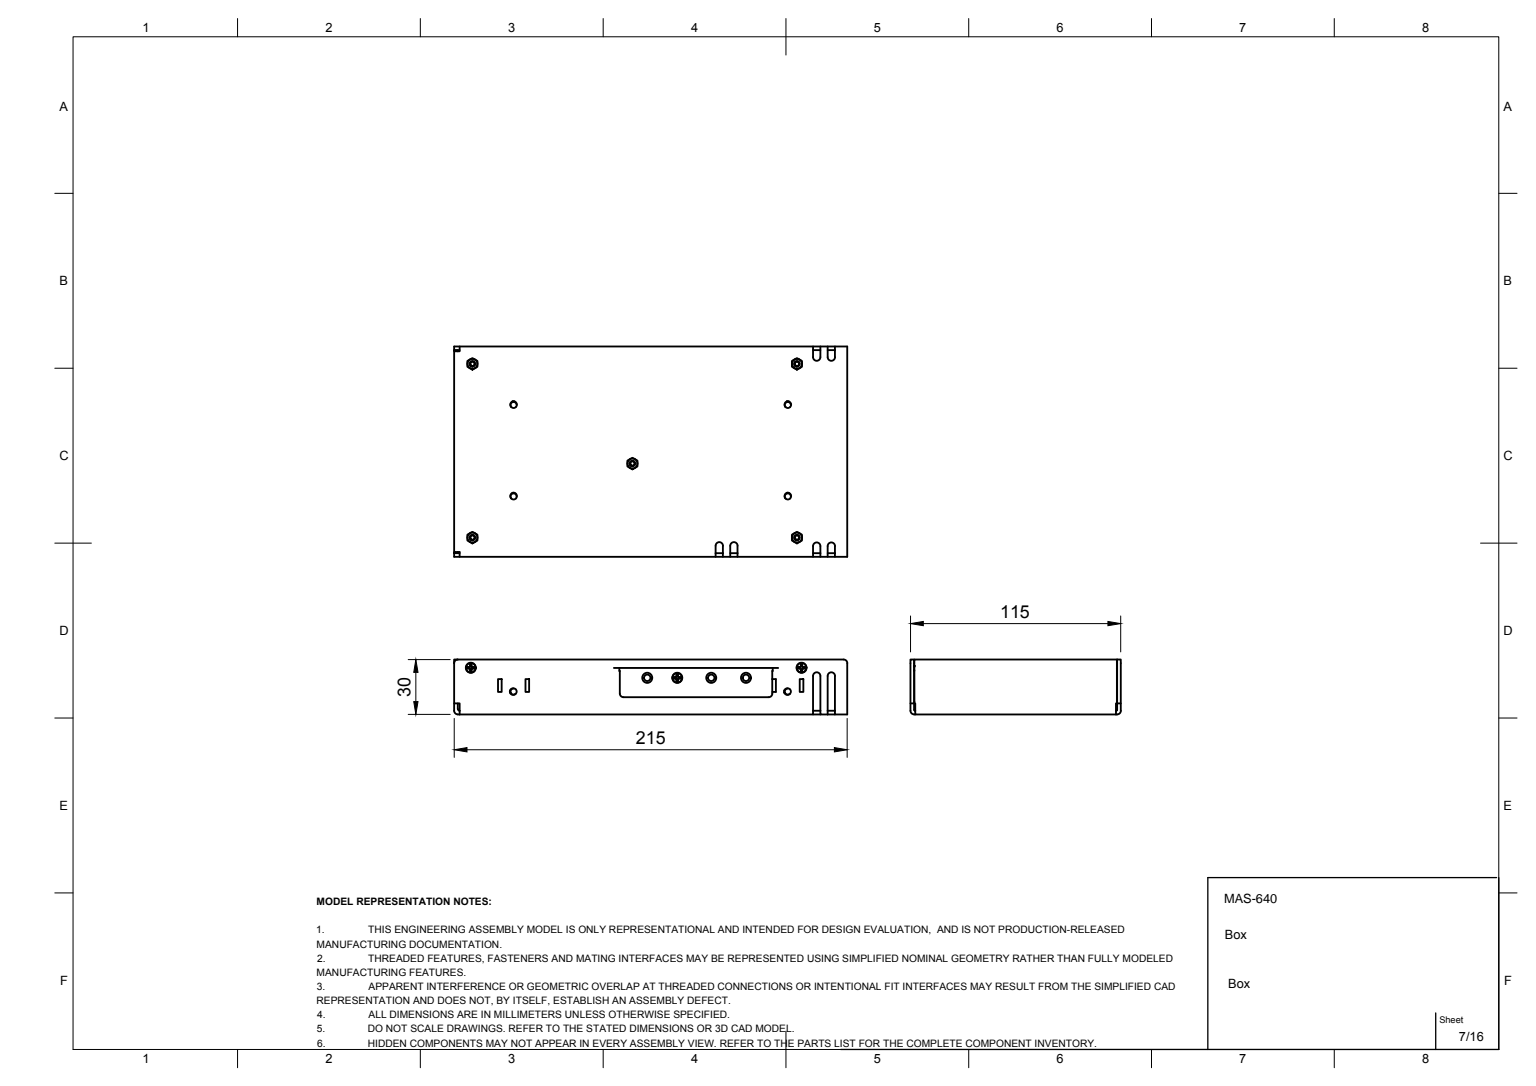
ISO-10303-21;
HEADER;
FILE_DESCRIPTION((''),'2;1');
FILE_NAME('Box.step','2026-10-09T10:33:02-07:00',(''),(''),'','','');
FILE_SCHEMA (('AUTOMOTIVE_DESIGN { 1 0 10303 214 3 1 1 }'));
ENDSEC;
DATA;
#10=MECHANICAL_DESIGN_GEOMETRIC_PRESENTATION_REPRESENTATION('',(#841),#86330);
#227=TOROIDAL_SURFACE('',#33403,5.,1.) ;
#228=TOROIDAL_SURFACE('',#33408,5.,1.) ;
#229=TOROIDAL_SURFACE('',#33423,5.,1.) ;
#230=TOROIDAL_SURFACE('',#33428,5.,1.) ;
#231=TOROIDAL_SURFACE('',#33506,5.25,3.25) ;
#232=TOROIDAL_SURFACE('',#33549,5.25,3.25) ;
#233=TOROIDAL_SURFACE('',#33614,5.25,3.25) ;
#234=TOROIDAL_SURFACE('',#33619,5.25,3.25) ;
#235=TOROIDAL_SURFACE('',#33657,0.250000000000004,0.124999999999957) ;
#236=TOROIDAL_SURFACE('',#33661,0.250000000000004,0.125000000000002) ;
#237=TOROIDAL_SURFACE('',#33662,0.250000000000004,0.125000000000002) ;
#238=TOROIDAL_SURFACE('',#33663,0.250000000000004,0.125000000000011) ;
#740=(
BOUNDED_SURFACE()
B_SPLINE_SURFACE(2,2,((#67035,#67036,#67037),(#67038,#67039,#67040),(#67041,
#67042,#67043)),.UNSPECIFIED.,.F.,.F.,.F.)
B_SPLINE_SURFACE_WITH_KNOTS((3,3),(3,3),(-1.5707963267962,1.31181440870059E-14),
(-1.57079632679766,2.95313754417746E-12),.UNSPECIFIED.)
GEOMETRIC_REPRESENTATION_ITEM()
RATIONAL_B_SPLINE_SURFACE(((1.,0.707106781184525,1.),(0.707106781186029,
0.499999999998204,0.707106781186029),(1.,0.707106781184525,1.)))
REPRESENTATION_ITEM('')
SURFACE()
) ;
#741=(
BOUNDED_SURFACE()
B_SPLINE_SURFACE(2,2,((#67047,#67048,#67049),(#67050,#67051,#67052),(#67053,
#67054,#67055)),.UNSPECIFIED.,.F.,.F.,.F.)
B_SPLINE_SURFACE_WITH_KNOTS((3,3),(3,3),(-1.38839876682605E-15,1.57079632679588),
(1.57079632679424,3.14159265359081),.UNSPECIFIED.)
GEOMETRIC_REPRESENTATION_ITEM()
RATIONAL_B_SPLINE_SURFACE(((1.,0.707106781185957,1.),(0.707106781186211,
0.499999999999345,0.707106781186211),(1.,0.707106781185957,1.)))
REPRESENTATION_ITEM('')
SURFACE()
) ;
#742=(
BOUNDED_SURFACE()
B_SPLINE_SURFACE(2,2,((#67066,#67067,#67068),(#67069,#67070,#67071),(#67072,
#67073,#67074)),.UNSPECIFIED.,.F.,.F.,.F.)
B_SPLINE_SURFACE_WITH_KNOTS((3,3),(3,3),(-3.21499456677232E-13,1.57079632679539),
(-7.36310365920222E-13,1.57079632679562),.UNSPECIFIED.)
GEOMETRIC_REPRESENTATION_ITEM()
RATIONAL_B_SPLINE_SURFACE(((1.,0.707106781186032,1.),(0.707106781186293,
0.499999999999455,0.707106781186293),(1.,0.707106781186032,1.)))
REPRESENTATION_ITEM('')
SURFACE()
) ;
#743=(
BOUNDED_SURFACE()
B_SPLINE_SURFACE(2,2,((#67078,#67079,#67080),(#67081,#67082,#67083),(#67084,
#67085,#67086)),.UNSPECIFIED.,.F.,.F.,.F.)
B_SPLINE_SURFACE_WITH_KNOTS((3,3),(3,3),(-1.57079632679451,6.78283756875461E-13),
(-3.14159265358933,-1.57079632679533),.UNSPECIFIED.)
GEOMETRIC_REPRESENTATION_ITEM()
RATIONAL_B_SPLINE_SURFACE(((1.,0.707106781186867,1.),(0.70710678118647,
0.500000000000171,0.70710678118647),(1.,0.707106781186867,1.)))
REPRESENTATION_ITEM('')
SURFACE()
) ;
#817=SHAPE_REPRESENTATION_RELATIONSHIP('SRR','None',#86454,#829) ;
#829=ADVANCED_BREP_SHAPE_REPRESENTATION('',(#853),#86308) ;
#841=STYLED_ITEM('',(#86581),#853) ;
#853=MANIFOLD_SOLID_BREP('Body1',#32640) ;
#883=CONICAL_SURFACE('',#33469,2.20000000000002,0.785398163397472) ;
#884=CONICAL_SURFACE('',#33472,2.2,0.78539816339745) ;
#885=CONICAL_SURFACE('',#33475,2.2,0.785398163397451) ;
#886=CONICAL_SURFACE('',#33486,2.25,0.785398163397448) ;
#887=CONICAL_SURFACE('',#33571,2.25,0.785398163397448) ;
#888=CONICAL_SURFACE('',#33576,2.25,0.785398163397448) ;
#889=CONICAL_SURFACE('',#33581,2.25,0.785398163397448) ;
#890=CONICAL_SURFACE('',#33586,2.25,0.785398163397448) ;
#891=CONICAL_SURFACE('',#33635,2.2,0.78539816339745) ;
#905=B_SPLINE_SURFACE_WITH_KNOTS('',3,1,((#65564,#65565),(#65566,#65567),
(#65568,#65569),(#65570,#65571),(#65572,#65573),(#65574,#65575),(#65576,
#65577),(#65578,#65579),(#65580,#65581),(#65582,#65583),(#65584,#65585),
(#65586,#65587),(#65588,#65589),(#65590,#65591),(#65592,#65593),(#65594,
#65595),(#65596,#65597),(#65598,#65599),(#65600,#65601),(#65602,#65603),
(#65604,#65605),(#65606,#65607)),.UNSPECIFIED.,.F.,.F.,.F.,(4,3,3,3,3,3,
3,4),(2,2),(0.136589431488165,0.1402592459748,0.143851356976514,0.2091154250925,
0.346827783328,0.4845401415634,0.990211404581674,0.997547219258416),(0.,
0.297000000002801),.UNSPECIFIED.) ;
#906=B_SPLINE_SURFACE_WITH_KNOTS('',3,3,((#66221,#66222,#66223,#66224,#66225,
#66226,#66227,#66228,#66229,#66230,#66231,#66232,#66233,#66234,#66235,#66236,
#66237,#66238,#66239,#66240,#66241,#66242,#66243),(#66244,#66245,#66246,
#66247,#66248,#66249,#66250,#66251,#66252,#66253,#66254,#66255,#66256,#66257,
#66258,#66259,#66260,#66261,#66262,#66263,#66264,#66265,#66266),(#66267,
#66268,#66269,#66270,#66271,#66272,#66273,#66274,#66275,#66276,#66277,#66278,
#66279,#66280,#66281,#66282,#66283,#66284,#66285,#66286,#66287,#66288,#66289),
(#66290,#66291,#66292,#66293,#66294,#66295,#66296,#66297,#66298,#66299,
#66300,#66301,#66302,#66303,#66304,#66305,#66306,#66307,#66308,#66309,#66310,
#66311,#66312)),.UNSPECIFIED.,.F.,.F.,.F.,(4,4),(4,1,1,1,1,1,1,1,1,1,1,
1,1,1,1,1,1,1,1,1,4),(-0.000643685928907995,0.0452738098722425),(14.3976860695295,
15.3964695570642,16.3947981013537,17.3931266456432,18.3914551899327,19.3897837342222,
20.3881122785118,21.3864408228013,22.3847693670908,23.3830979113803,24.3814264556698,
25.3797549999593,26.3780835442488,27.3764120885383,28.3747406328278,29.3730691771173,
30.3713977214068,31.3697262656963,32.3680548099858,33.3663833542754,34.3650967250075),
 .UNSPECIFIED.) ;
#907=B_SPLINE_SURFACE_WITH_KNOTS('',3,3,((#66313,#66314,#66315,#66316,#66317,
#66318,#66319,#66320,#66321,#66322,#66323,#66324,#66325,#66326,#66327,#66328,
#66329,#66330,#66331,#66332,#66333,#66334,#66335),(#66336,#66337,#66338,
#66339,#66340,#66341,#66342,#66343,#66344,#66345,#66346,#66347,#66348,#66349,
#66350,#66351,#66352,#66353,#66354,#66355,#66356,#66357,#66358),(#66359,
#66360,#66361,#66362,#66363,#66364,#66365,#66366,#66367,#66368,#66369,#66370,
#66371,#66372,#66373,#66374,#66375,#66376,#66377,#66378,#66379,#66380,#66381),
(#66382,#66383,#66384,#66385,#66386,#66387,#66388,#66389,#66390,#66391,
#66392,#66393,#66394,#66395,#66396,#66397,#66398,#66399,#66400,#66401,#66402,
#66403,#66404)),.UNSPECIFIED.,.F.,.F.,.F.,(4,4),(4,1,1,1,1,1,1,1,1,1,1,
1,1,1,1,1,1,1,1,1,4),(-0.000384825361838686,0.0458091503480694),(11.8611951788935,
12.8599085485448,13.8582370928343,14.8565656371238,15.8548941814133,16.8532227257028,
17.8515512699923,18.8498798142818,19.8482083585713,20.8465369028608,21.8448654471503,
22.8431939914399,23.8415225357294,24.8398510800189,25.8381796243084,26.8365081685979,
27.8348367128874,28.8331652571769,29.8314938014664,30.8298223457559,31.8285783647924),
 .UNSPECIFIED.) ;
#908=B_SPLINE_SURFACE_WITH_KNOTS('',3,3,((#66405,#66406,#66407,#66408,#66409,
#66410,#66411,#66412,#66413,#66414,#66415,#66416,#66417,#66418,#66419,#66420,
#66421,#66422,#66423,#66424,#66425,#66426,#66427),(#66428,#66429,#66430,
#66431,#66432,#66433,#66434,#66435,#66436,#66437,#66438,#66439,#66440,#66441,
#66442,#66443,#66444,#66445,#66446,#66447,#66448,#66449,#66450),(#66451,
#66452,#66453,#66454,#66455,#66456,#66457,#66458,#66459,#66460,#66461,#66462,
#66463,#66464,#66465,#66466,#66467,#66468,#66469,#66470,#66471,#66472,#66473),
(#66474,#66475,#66476,#66477,#66478,#66479,#66480,#66481,#66482,#66483,
#66484,#66485,#66486,#66487,#66488,#66489,#66490,#66491,#66492,#66493,#66494,
#66495,#66496)),.UNSPECIFIED.,.F.,.F.,.F.,(4,4),(4,1,1,1,1,1,1,1,1,1,1,
1,1,1,1,1,1,1,1,1,4),(-0.000647263935840991,0.0452759437895929),(14.3976836084423,
15.3964695570666,16.394798101356,17.3931266456453,18.3914551899347,19.389783734224,
20.3881122785134,21.3864408228027,22.384769367092,23.3830979113814,24.3814264556707,
25.3797549999601,26.3780835442494,27.3764120885388,28.3747406328281,29.3730691771175,
30.3713977214068,31.3697262656962,32.3680548099855,33.3663833542749,34.3650988589243),
 .UNSPECIFIED.) ;
#909=B_SPLINE_SURFACE_WITH_KNOTS('',3,3,((#66497,#66498,#66499,#66500,#66501,
#66502,#66503,#66504,#66505,#66506,#66507,#66508,#66509,#66510,#66511,#66512,
#66513,#66514,#66515,#66516,#66517,#66518,#66519),(#66520,#66521,#66522,
#66523,#66524,#66525,#66526,#66527,#66528,#66529,#66530,#66531,#66532,#66533,
#66534,#66535,#66536,#66537,#66538,#66539,#66540,#66541,#66542),(#66543,
#66544,#66545,#66546,#66547,#66548,#66549,#66550,#66551,#66552,#66553,#66554,
#66555,#66556,#66557,#66558,#66559,#66560,#66561,#66562,#66563,#66564,#66565),
(#66566,#66567,#66568,#66569,#66570,#66571,#66572,#66573,#66574,#66575,
#66576,#66577,#66578,#66579,#66580,#66581,#66582,#66583,#66584,#66585,#66586,
#66587,#66588)),.UNSPECIFIED.,.F.,.F.,.F.,(4,4),(4,1,1,1,1,1,1,1,1,1,1,
1,1,1,1,1,1,1,1,1,4),(-0.00038695950106726,0.0458188085461498),(11.8611930447567,
12.8599085485472,13.8582370928365,14.8565656371259,15.8548941814152,16.8532227257046,
17.8515512699939,18.8498798142833,19.8482083585726,20.846536902862,21.8448654471513,
22.8431939914407,23.84152253573,24.8398510800194,25.8381796243087,26.8365081685981,
27.8348367128874,28.8331652571768,29.8314938014661,30.8298223457555,31.8285876047897),
 .UNSPECIFIED.) ;
#910=B_SPLINE_SURFACE_WITH_KNOTS('',3,3,((#66589,#66590,#66591,#66592,#66593,
#66594,#66595,#66596,#66597,#66598,#66599,#66600,#66601,#66602,#66603,#66604,
#66605,#66606,#66607,#66608,#66609,#66610,#66611),(#66612,#66613,#66614,
#66615,#66616,#66617,#66618,#66619,#66620,#66621,#66622,#66623,#66624,#66625,
#66626,#66627,#66628,#66629,#66630,#66631,#66632,#66633,#66634),(#66635,
#66636,#66637,#66638,#66639,#66640,#66641,#66642,#66643,#66644,#66645,#66646,
#66647,#66648,#66649,#66650,#66651,#66652,#66653,#66654,#66655,#66656,#66657),
(#66658,#66659,#66660,#66661,#66662,#66663,#66664,#66665,#66666,#66667,
#66668,#66669,#66670,#66671,#66672,#66673,#66674,#66675,#66676,#66677,#66678,
#66679,#66680)),.UNSPECIFIED.,.F.,.F.,.F.,(4,4),(4,1,1,1,1,1,1,1,1,1,1,
1,1,1,1,1,1,1,1,1,4),(-0.000640464694106941,0.0452718121575805),(14.3976883946163,
15.3964695570665,16.394798101356,17.3931266456454,18.3914551899348,19.3897837342242,
20.3881122785137,21.3864408228031,22.3847693670925,23.3830979113819,24.3814264556714,
25.3797549999608,26.3780835442502,27.3764120885396,28.3747406328291,29.3730691771185,
30.3713977214079,31.3697262656973,32.3680548099868,33.3663833542762,34.3650947272934),
 .UNSPECIFIED.) ;
#911=B_SPLINE_SURFACE_WITH_KNOTS('',3,3,((#66681,#66682,#66683,#66684,#66685,
#66686,#66687,#66688,#66689,#66690,#66691,#66692,#66693,#66694,#66695,#66696,
#66697,#66698,#66699,#66700,#66701,#66702,#66703),(#66704,#66705,#66706,
#66707,#66708,#66709,#66710,#66711,#66712,#66713,#66714,#66715,#66716,#66717,
#66718,#66719,#66720,#66721,#66722,#66723,#66724,#66725,#66726),(#66727,
#66728,#66729,#66730,#66731,#66732,#66733,#66734,#66735,#66736,#66737,#66738,
#66739,#66740,#66741,#66742,#66743,#66744,#66745,#66746,#66747,#66748,#66749),
(#66750,#66751,#66752,#66753,#66754,#66755,#66756,#66757,#66758,#66759,
#66760,#66761,#66762,#66763,#66764,#66765,#66766,#66767,#66768,#66769,#66770,
#66771,#66772)),.UNSPECIFIED.,.F.,.F.,.F.,(4,4),(4,1,1,1,1,1,1,1,1,1,1,
1,1,1,1,1,1,1,1,1,4),(-0.000382830284004954,0.0458008767222032),(11.8611971739735,
12.8599085485469,13.8582370928364,14.8565656371258,15.8548941814152,16.8532227257047,
17.8515512699941,18.8498798142835,19.848208358573,20.8465369028624,21.8448654471518,
22.8431939914413,23.8415225357307,24.8398510800201,25.8381796243096,26.836508168599,
27.8348367128884,28.8331652571779,29.8314938014673,30.8298223457568,31.8285705594706),
 .UNSPECIFIED.) ;
#912=B_SPLINE_SURFACE_WITH_KNOTS('',3,3,((#66773,#66774,#66775,#66776,#66777,
#66778,#66779,#66780,#66781,#66782,#66783,#66784,#66785,#66786,#66787,#66788,
#66789,#66790,#66791,#66792,#66793,#66794,#66795),(#66796,#66797,#66798,
#66799,#66800,#66801,#66802,#66803,#66804,#66805,#66806,#66807,#66808,#66809,
#66810,#66811,#66812,#66813,#66814,#66815,#66816,#66817,#66818),(#66819,
#66820,#66821,#66822,#66823,#66824,#66825,#66826,#66827,#66828,#66829,#66830,
#66831,#66832,#66833,#66834,#66835,#66836,#66837,#66838,#66839,#66840,#66841),
(#66842,#66843,#66844,#66845,#66846,#66847,#66848,#66849,#66850,#66851,
#66852,#66853,#66854,#66855,#66856,#66857,#66858,#66859,#66860,#66861,#66862,
#66863,#66864)),.UNSPECIFIED.,.F.,.F.,.F.,(4,4),(4,1,1,1,1,1,1,1,1,1,1,
1,1,1,1,1,1,1,1,1,4),(-0.000644632360233455,0.0452743831442753),(14.3976854059706,
15.3964695570646,16.394798101354,17.3931266456435,18.3914551899329,19.3897837342223,
20.3881122785117,21.3864408228012,22.3847693670906,23.38309791138,24.3814264556694,
25.3797549999589,26.3780835442483,27.3764120885377,28.3747406328271,29.3730691771166,
30.371397721406,31.3697262656954,32.3680548099849,33.3663833542743,34.3650972982779),
 .UNSPECIFIED.) ;
#913=B_SPLINE_SURFACE_WITH_KNOTS('',3,3,((#66865,#66866,#66867,#66868,#66869,
#66870,#66871,#66872,#66873,#66874,#66875,#66876,#66877,#66878,#66879,#66880,
#66881,#66882,#66883,#66884,#66885,#66886,#66887),(#66888,#66889,#66890,
#66891,#66892,#66893,#66894,#66895,#66896,#66897,#66898,#66899,#66900,#66901,
#66902,#66903,#66904,#66905,#66906,#66907,#66908,#66909,#66910),(#66911,
#66912,#66913,#66914,#66915,#66916,#66917,#66918,#66919,#66920,#66921,#66922,
#66923,#66924,#66925,#66926,#66927,#66928,#66929,#66930,#66931,#66932,#66933),
(#66934,#66935,#66936,#66937,#66938,#66939,#66940,#66941,#66942,#66943,
#66944,#66945,#66946,#66947,#66948,#66949,#66950,#66951,#66952,#66953,#66954,
#66955,#66956)),.UNSPECIFIED.,.F.,.F.,.F.,(4,4),(4,1,1,1,1,1,1,1,1,1,1,
1,1,1,1,1,1,1,1,1,4),(-0.000385400908840022,0.045811671314961),(11.8611946033468,
12.859908548545,13.8582370928345,14.8565656371239,15.8548941814133,16.8532227257028,
17.8515512699922,18.8498798142816,19.8482083585711,20.8465369028605,21.8448654471499,
22.8431939914394,23.8415225357288,24.8398510800182,25.8381796243077,26.8365081685971,
27.8348367128865,28.833165257176,29.8314938014654,30.8298223457548,31.8285807653119),
 .UNSPECIFIED.) ;
#914=B_SPLINE_SURFACE_WITH_KNOTS('',3,3,((#67087,#67088,#67089,#67090,#67091,
#67092,#67093,#67094,#67095,#67096,#67097,#67098,#67099,#67100,#67101,#67102,
#67103,#67104,#67105,#67106,#67107,#67108,#67109),(#67110,#67111,#67112,
#67113,#67114,#67115,#67116,#67117,#67118,#67119,#67120,#67121,#67122,#67123,
#67124,#67125,#67126,#67127,#67128,#67129,#67130,#67131,#67132),(#67133,
#67134,#67135,#67136,#67137,#67138,#67139,#67140,#67141,#67142,#67143,#67144,
#67145,#67146,#67147,#67148,#67149,#67150,#67151,#67152,#67153,#67154,#67155),
(#67156,#67157,#67158,#67159,#67160,#67161,#67162,#67163,#67164,#67165,
#67166,#67167,#67168,#67169,#67170,#67171,#67172,#67173,#67174,#67175,#67176,
#67177,#67178)),.UNSPECIFIED.,.F.,.F.,.F.,(4,4),(4,1,1,1,1,1,1,1,1,1,1,
1,1,1,1,1,1,1,1,1,4),(-0.000645665255431383,0.0452750015650409),(14.3976846920928,
15.3964695570661,16.3947981013555,17.3931266456449,18.3914551899343,19.3897837342237,
20.3881122785131,21.3864408228024,22.3847693670918,23.3830979113812,24.3814264556706,
25.37975499996,26.3780835442494,27.3764120885388,28.3747406328282,29.3730691771176,
30.3713977214069,31.3697262656963,32.3680548099857,33.3663833542751,34.3650979167),
 .UNSPECIFIED.) ;
#915=B_SPLINE_SURFACE_WITH_KNOTS('',3,3,((#67354,#67355,#67356,#67357,#67358,
#67359,#67360,#67361,#67362,#67363,#67364,#67365,#67366,#67367,#67368,#67369,
#67370,#67371,#67372,#67373,#67374,#67375,#67376),(#67377,#67378,#67379,
#67380,#67381,#67382,#67383,#67384,#67385,#67386,#67387,#67388,#67389,#67390,
#67391,#67392,#67393,#67394,#67395,#67396,#67397,#67398,#67399),(#67400,
#67401,#67402,#67403,#67404,#67405,#67406,#67407,#67408,#67409,#67410,#67411,
#67412,#67413,#67414,#67415,#67416,#67417,#67418,#67419,#67420,#67421,#67422),
(#67423,#67424,#67425,#67426,#67427,#67428,#67429,#67430,#67431,#67432,
#67433,#67434,#67435,#67436,#67437,#67438,#67439,#67440,#67441,#67442,#67443,
#67444,#67445)),.UNSPECIFIED.,.F.,.F.,.F.,(4,4),(4,1,1,1,1,1,1,1,1,1,1,
1,1,1,1,1,1,1,1,1,4),(-0.000386017183284365,0.0458144387691291),(11.8611939870731,
12.8599085485457,13.8582370928351,14.8565656371245,15.8548941814139,16.8532227257033,
17.8515512699927,18.8498798142821,19.8482083585714,20.8465369028608,21.8448654471502,
22.8431939914396,23.841522535729,24.8398510800184,25.8381796243078,26.8365081685971,
27.8348367128865,28.8331652571759,29.8314938014653,30.8298223457547,31.8285834103066),
 .UNSPECIFIED.) ;
#916=B_SPLINE_SURFACE_WITH_KNOTS('',3,3,((#67621,#67622,#67623,#67624,#67625,
#67626,#67627,#67628,#67629,#67630,#67631,#67632,#67633,#67634,#67635,#67636,
#67637,#67638,#67639,#67640,#67641,#67642,#67643),(#67644,#67645,#67646,
#67647,#67648,#67649,#67650,#67651,#67652,#67653,#67654,#67655,#67656,#67657,
#67658,#67659,#67660,#67661,#67662,#67663,#67664,#67665,#67666),(#67667,
#67668,#67669,#67670,#67671,#67672,#67673,#67674,#67675,#67676,#67677,#67678,
#67679,#67680,#67681,#67682,#67683,#67684,#67685,#67686,#67687,#67688,#67689),
(#67690,#67691,#67692,#67693,#67694,#67695,#67696,#67697,#67698,#67699,
#67700,#67701,#67702,#67703,#67704,#67705,#67706,#67707,#67708,#67709,#67710,
#67711,#67712)),.UNSPECIFIED.,.F.,.F.,.F.,(4,4),(4,1,1,1,1,1,1,1,1,1,1,
1,1,1,1,1,1,1,1,1,4),(-0.000641741025930388,0.0452726121833519),(14.3976874611935,
15.3964695570662,16.3947981013556,17.393126645645,18.3914551899344,19.3897837342237,
20.3881122785131,21.3864408228025,22.3847693670919,23.3830979113813,24.3814264556707,
25.37975499996,26.3780835442494,27.3764120885388,28.3747406328282,29.3730691771176,
30.371397721407,31.3697262656963,32.3680548099857,33.3663833542751,34.3650955273184),
 .UNSPECIFIED.) ;
#917=B_SPLINE_SURFACE_WITH_KNOTS('',3,3,((#67888,#67889,#67890,#67891,#67892,
#67893,#67894,#67895,#67896,#67897,#67898,#67899,#67900,#67901,#67902,#67903,
#67904,#67905,#67906,#67907,#67908,#67909,#67910),(#67911,#67912,#67913,
#67914,#67915,#67916,#67917,#67918,#67919,#67920,#67921,#67922,#67923,#67924,
#67925,#67926,#67927,#67928,#67929,#67930,#67931,#67932,#67933),(#67934,
#67935,#67936,#67937,#67938,#67939,#67940,#67941,#67942,#67943,#67944,#67945,
#67946,#67947,#67948,#67949,#67950,#67951,#67952,#67953,#67954,#67955,#67956),
(#67957,#67958,#67959,#67960,#67961,#67962,#67963,#67964,#67965,#67966,
#67967,#67968,#67969,#67970,#67971,#67972,#67973,#67974,#67975,#67976,#67977,
#67978,#67979)),.UNSPECIFIED.,.F.,.F.,.F.,(4,4),(4,1,1,1,1,1,1,1,1,1,1,
1,1,1,1,1,1,1,1,1,4),(-0.000383627530710749,0.0458040974015815),(11.8611963767258,
12.8599085485459,13.8582370928353,14.8565656371247,15.8548941814141,16.8532227257035,
17.8515512699929,18.8498798142822,19.8482083585716,20.846536902861,21.8448654471504,
22.8431939914398,23.8415225357292,24.8398510800186,25.8381796243079,26.8365081685973,
27.8348367128867,28.8331652571761,29.8314938014655,30.8298223457549,31.8285735830159),
 .UNSPECIFIED.) ;
#918=B_SPLINE_SURFACE_WITH_KNOTS('',3,3,((#68155,#68156,#68157,#68158,#68159,
#68160,#68161,#68162,#68163,#68164,#68165,#68166,#68167,#68168,#68169,#68170,
#68171,#68172,#68173,#68174,#68175,#68176,#68177),(#68178,#68179,#68180,
#68181,#68182,#68183,#68184,#68185,#68186,#68187,#68188,#68189,#68190,#68191,
#68192,#68193,#68194,#68195,#68196,#68197,#68198,#68199,#68200),(#68201,
#68202,#68203,#68204,#68205,#68206,#68207,#68208,#68209,#68210,#68211,#68212,
#68213,#68214,#68215,#68216,#68217,#68218,#68219,#68220,#68221,#68222,#68223),
(#68224,#68225,#68226,#68227,#68228,#68229,#68230,#68231,#68232,#68233,
#68234,#68235,#68236,#68237,#68238,#68239,#68240,#68241,#68242,#68243,#68244,
#68245,#68246)),.UNSPECIFIED.,.F.,.F.,.F.,(4,4),(4,1,1,1,1,1,1,1,1,1,1,
1,1,1,1,1,1,1,1,1,4),(-0.000643140498361754,0.0452734766386899),(14.3976864560211,
15.3964695570662,16.3947981013556,17.3931266456449,18.3914551899343,19.3897837342237,
20.3881122785131,21.3864408228024,22.3847693670918,23.3830979113812,24.3814264556706,
25.3797549999599,26.3780835442493,27.3764120885387,28.3747406328281,29.3730691771174,
30.3713977214068,31.3697262656962,32.3680548099856,33.3663833542749,34.3650963917735),
 .UNSPECIFIED.) ;
#919=B_SPLINE_SURFACE_WITH_KNOTS('',3,3,((#68422,#68423,#68424,#68425,#68426,
#68427,#68428,#68429,#68430,#68431,#68432,#68433,#68434,#68435,#68436,#68437,
#68438,#68439,#68440,#68441,#68442,#68443,#68444),(#68445,#68446,#68447,
#68448,#68449,#68450,#68451,#68452,#68453,#68454,#68455,#68456,#68457,#68458,
#68459,#68460,#68461,#68462,#68463,#68464,#68465,#68466,#68467),(#68468,
#68469,#68470,#68471,#68472,#68473,#68474,#68475,#68476,#68477,#68478,#68479,
#68480,#68481,#68482,#68483,#68484,#68485,#68486,#68487,#68488,#68489,#68490),
(#68491,#68492,#68493,#68494,#68495,#68496,#68497,#68498,#68499,#68500,
#68501,#68502,#68503,#68504,#68505,#68506,#68507,#68508,#68509,#68510,#68511,
#68512,#68513)),.UNSPECIFIED.,.F.,.F.,.F.,(4,4),(4,1,1,1,1,1,1,1,1,1,1,
1,1,1,1,1,1,1,1,1,4),(-0.000384492090036841,0.0458077183624923),(11.8611955121666,
12.859908548546,13.8582370928354,14.8565656371247,15.8548941814141,16.8532227257035,
17.8515512699929,18.8498798142823,19.8482083585716,20.846536902861,21.8448654471504,
22.8431939914398,23.8415225357292,24.8398510800185,25.8381796243079,26.8365081685973,
27.8348367128867,28.833165257176,29.8314938014654,30.8298223457548,31.8285770053882),
 .UNSPECIFIED.) ;
#920=B_SPLINE_SURFACE_WITH_KNOTS('',3,3,((#68901,#68902,#68903,#68904,#68905,
#68906,#68907,#68908,#68909,#68910,#68911,#68912,#68913,#68914,#68915,#68916,
#68917,#68918,#68919,#68920,#68921,#68922,#68923),(#68924,#68925,#68926,
#68927,#68928,#68929,#68930,#68931,#68932,#68933,#68934,#68935,#68936,#68937,
#68938,#68939,#68940,#68941,#68942,#68943,#68944,#68945,#68946),(#68947,
#68948,#68949,#68950,#68951,#68952,#68953,#68954,#68955,#68956,#68957,#68958,
#68959,#68960,#68961,#68962,#68963,#68964,#68965,#68966,#68967,#68968,#68969),
(#68970,#68971,#68972,#68973,#68974,#68975,#68976,#68977,#68978,#68979,
#68980,#68981,#68982,#68983,#68984,#68985,#68986,#68987,#68988,#68989,#68990,
#68991,#68992)),.UNSPECIFIED.,.F.,.F.,.F.,(4,4),(4,1,1,1,1,1,1,1,1,1,1,
1,1,1,1,1,1,1,1,1,4),(-0.000646812714374105,0.0452756796923178),(14.3976839116802,
15.3964695570661,16.3947981013555,17.3931266456449,18.3914551899343,19.3897837342237,
20.3881122785131,21.3864408228024,22.3847693670918,23.3830979113812,24.3814264556706,
25.37975499996,26.3780835442494,27.3764120885387,28.3747406328281,29.3730691771175,
30.3713977214069,31.3697262656963,32.3680548099857,33.3663833542751,34.3650985948273),
 .UNSPECIFIED.) ;
#921=B_SPLINE_SURFACE_WITH_KNOTS('',3,3,((#69075,#69076,#69077,#69078,#69079,
#69080,#69081,#69082,#69083,#69084,#69085,#69086,#69087,#69088,#69089,#69090,
#69091,#69092,#69093,#69094,#69095,#69096,#69097),(#69098,#69099,#69100,
#69101,#69102,#69103,#69104,#69105,#69106,#69107,#69108,#69109,#69110,#69111,
#69112,#69113,#69114,#69115,#69116,#69117,#69118,#69119,#69120),(#69121,
#69122,#69123,#69124,#69125,#69126,#69127,#69128,#69129,#69130,#69131,#69132,
#69133,#69134,#69135,#69136,#69137,#69138,#69139,#69140,#69141,#69142,#69143),
(#69144,#69145,#69146,#69147,#69148,#69149,#69150,#69151,#69152,#69153,
#69154,#69155,#69156,#69157,#69158,#69159,#69160,#69161,#69162,#69163,#69164,
#69165,#69166)),.UNSPECIFIED.,.F.,.F.,.F.,(4,4),(4,1,1,1,1,1,1,1,1,1,1,
1,1,1,1,1,1,1,1,1,4),(-0.000386695378374584,0.0458175667348162),(11.861193308878,
12.8599085485458,13.8582370928352,14.8565656371246,15.854894181414,16.8532227257034,
17.8515512699928,18.8498798142822,19.8482083585716,20.846536902861,21.8448654471503,
22.8431939914397,23.8415225357291,24.8398510800185,25.8381796243079,26.8365081685973,
27.8348367128867,28.8331652571761,29.8314938014655,30.8298223457549,31.8285864107338),
 .UNSPECIFIED.) ;
#1051=FACE_BOUND('',#4491,.T.) ;
#1052=FACE_BOUND('',#4492,.T.) ;
#1053=FACE_BOUND('',#4493,.T.) ;
#1054=FACE_BOUND('',#4494,.T.) ;
#1055=FACE_BOUND('',#4495,.T.) ;
#1056=FACE_BOUND('',#4496,.T.) ;
#1057=FACE_BOUND('',#4497,.T.) ;
#1058=FACE_BOUND('',#4498,.T.) ;
#1059=FACE_BOUND('',#4501,.T.) ;
#1060=FACE_BOUND('',#4502,.T.) ;
#1061=FACE_BOUND('',#4503,.T.) ;
#1062=FACE_BOUND('',#4504,.T.) ;
#1063=FACE_BOUND('',#4505,.T.) ;
#1064=FACE_BOUND('',#4506,.T.) ;
#1065=FACE_BOUND('',#4507,.T.) ;
#1066=FACE_BOUND('',#4508,.T.) ;
#1067=FACE_BOUND('',#4509,.T.) ;
#1068=FACE_BOUND('',#4510,.T.) ;
#1069=FACE_BOUND('',#4512,.T.) ;
#1070=FACE_BOUND('',#4513,.T.) ;
#1071=FACE_BOUND('',#4514,.T.) ;
#1072=FACE_BOUND('',#4515,.T.) ;
#1073=FACE_BOUND('',#4516,.T.) ;
#1074=FACE_BOUND('',#4517,.T.) ;
#1075=FACE_BOUND('',#4518,.T.) ;
#1076=FACE_BOUND('',#4519,.T.) ;
#1077=FACE_BOUND('',#4521,.T.) ;
#1078=FACE_BOUND('',#4522,.T.) ;
#1079=FACE_BOUND('',#4523,.T.) ;
#1080=FACE_BOUND('',#4524,.T.) ;
#1081=FACE_BOUND('',#4525,.T.) ;
#1082=FACE_BOUND('',#4526,.T.) ;
#1083=FACE_BOUND('',#4527,.T.) ;
#1084=FACE_BOUND('',#4528,.T.) ;
#1085=FACE_BOUND('',#4529,.T.) ;
#1086=FACE_BOUND('',#4530,.T.) ;
#1087=FACE_BOUND('',#4644,.T.) ;
#1088=FACE_BOUND('',#4645,.T.) ;
#1089=FACE_BOUND('',#4646,.T.) ;
#1090=FACE_BOUND('',#4647,.T.) ;
#1091=FACE_BOUND('',#4689,.T.) ;
#1092=FACE_BOUND('',#4724,.T.) ;
#1093=FACE_BOUND('',#4725,.T.) ;
#1094=FACE_BOUND('',#4726,.T.) ;
#1095=FACE_BOUND('',#4727,.T.) ;
#1096=FACE_BOUND('',#4732,.T.) ;
#1097=FACE_BOUND('',#4744,.T.) ;
#1098=FACE_BOUND('',#4745,.T.) ;
#1099=FACE_BOUND('',#4746,.T.) ;
#1100=FACE_BOUND('',#4747,.T.) ;
#1101=FACE_BOUND('',#4748,.T.) ;
#1102=FACE_BOUND('',#4749,.T.) ;
#1103=FACE_BOUND('',#4750,.T.) ;
#1104=FACE_BOUND('',#4751,.T.) ;
#1105=FACE_BOUND('',#4752,.T.) ;
#1106=FACE_BOUND('',#4768,.T.) ;
#1107=FACE_BOUND('',#4769,.T.) ;
#1108=FACE_BOUND('',#4770,.T.) ;
#1109=FACE_BOUND('',#4771,.T.) ;
#1110=FACE_BOUND('',#4772,.T.) ;
#1111=FACE_BOUND('',#4773,.T.) ;
#1112=FACE_BOUND('',#4774,.T.) ;
#1113=FACE_BOUND('',#4775,.T.) ;
#1114=FACE_BOUND('',#4776,.T.) ;
#1256=B_SPLINE_CURVE_WITH_KNOTS('',3,(#50230,#50231,#50232,#50233,#50234,
#50235,#50236,#50237,#50238,#50239,#50240,#50241,#50242,#50243,#50244,#50245,
#50246,#50247,#50248,#50249,#50250,#50251,#50252,#50253,#50254,#50255,#50256,
#50257),.UNSPECIFIED.,.F.,.F.,(4,2,2,2,2,2,2,2,2,2,2,2,2,4),(0.459093916516044,
0.46455562735916,0.505821881594587,0.520988271639936,0.529970590367133,
0.542578350982259,0.575709939682203,0.614672647551458,0.632542444852366,
0.649281677754947,0.689464111786888,0.720032267469635,0.726902083818049,
0.732437476861398),.UNSPECIFIED.) ;
#1257=B_SPLINE_CURVE_WITH_KNOTS('',3,(#50260,#50261,#50262,#50263,#50264,
#50265,#50266,#50267,#50268,#50269,#50270,#50271,#50272,#50273,#50274,#50275,
#50276,#50277,#50278,#50279,#50280,#50281,#50282,#50283,#50284,#50285,#50286,
#50287,#50288,#50289,#50290,#50291,#50292,#50293,#50294,#50295),
 .UNSPECIFIED.,.F.,.F.,(4,2,2,2,2,2,2,2,2,2,2,2,2,2,2,2,2,4),(0.000332701134793292,
0.00532995658148356,0.0119825509393597,0.0487188803356833,0.0844089965964979,
0.100361879460944,0.116282468689568,0.149629266254007,0.178290336895723,
0.190733178272163,0.201074425783365,0.210399404436054,0.232074117560219,
0.28208000915706,0.30011450772679,0.315087246273823,0.336912777571983,0.381141457942968),
 .UNSPECIFIED.) ;
#1258=B_SPLINE_CURVE_WITH_KNOTS('',3,(#50301,#50302,#50303,#50304,#50305,
#50306,#50307,#50308,#50309,#50310,#50311,#50312,#50313,#50314,#50315,#50316,
#50317,#50318,#50319,#50320,#50321,#50322,#50323,#50324,#50325,#50326,#50327,
#50328,#50329,#50330,#50331,#50332,#50333,#50334,#50335,#50336,#50337,#50338,
#50339,#50340,#50341,#50342,#50343,#50344,#50345,#50346,#50347,#50348,#50349,
#50350,#50351,#50352,#50353,#50354,#50355,#50356,#50357,#50358,#50359,#50360,
#50361,#50362,#50363,#50364,#50365,#50366,#50367,#50368,#50369,#50370,#50371,
#50372,#50373,#50374,#50375,#50376,#50377,#50378),.UNSPECIFIED.,.F.,.F.,
(4,2,2,2,2,2,2,2,2,2,2,2,2,2,2,2,2,2,2,2,2,2,2,2,2,2,2,2,2,2,2,2,2,2,2,
2,2,2,4),(1.29365561641325,1.30113546894178,1.31756663056678,1.33312830280463,
1.36194319812924,1.40306001798898,1.41707239726473,1.42583345144023,1.438907235276,
1.4567472055773,1.50742443095404,1.52367565736048,1.53936823703037,1.57015419556187,
1.61065266245251,1.62355132522206,1.63233056992128,1.64662569486736,1.66730671714928,
1.71296324961579,1.72915479064639,1.74486354159992,1.77604692182362,1.81647765873443,
1.82921296125272,1.83797276770033,1.85234265187279,1.87321966665841,1.91832818857784,
1.93450511617934,1.95007856425548,1.97985222672331,2.02092117751393,2.03443886875799,
2.04322587270968,2.05689828304459,2.07604574726155,2.11487866906583,2.12885059658721),
 .UNSPECIFIED.) ;
#1259=B_SPLINE_CURVE_WITH_KNOTS('',3,(#50379,#50380,#50381,#50382,#50383,
#50384,#50385,#50386,#50387,#50388,#50389,#50390,#50391,#50392,#50393,#50394,
#50395,#50396,#50397,#50398,#50399,#50400,#50401,#50402,#50403,#50404,#50405,
#50406,#50407,#50408,#50409,#50410,#50411,#50412,#50413,#50414,#50415,#50416,
#50417,#50418,#50419,#50420),.UNSPECIFIED.,.F.,.F.,(4,2,2,2,2,2,2,2,2,2,
2,2,2,2,2,2,2,2,2,2,4),(0.000735163267886744,0.0138746955681923,0.0296423865919577,
0.0801063196227826,0.106649689626277,0.116363467174073,0.126486258322458,
0.164825866697053,0.201303399889853,0.217473147550887,0.233580681855967,
0.267585305229778,0.296202685786829,0.313253112284756,0.322102080649573,
0.33246197481545,0.366409709031667,0.408171648460054,0.424893469175312,
0.43988857479256,0.459093916516044),.UNSPECIFIED.) ;
#1260=B_SPLINE_CURVE_WITH_KNOTS('',3,(#50421,#50422,#50423,#50424,#50425,
#50426,#50427,#50428,#50429,#50430,#50431,#50432,#50433,#50434,#50435,#50436,
#50437,#50438,#50439,#50440,#50441,#50442,#50443,#50444,#50445,#50446,#50447,
#50448,#50449,#50450,#50451,#50452,#50453,#50454,#50455,#50456,#50457,#50458,
#50459,#50460,#50461,#50462,#50463,#50464,#50465,#50466,#50467,#50468,#50469,
#50470,#50471,#50472,#50473,#50474,#50475,#50476,#50477,#50478,#50479,#50480,
#50481,#50482,#50483,#50484,#50485,#50486,#50487,#50488,#50489,#50490,#50491,
#50492,#50493,#50494,#50495,#50496,#50497,#50498,#50499,#50500,#50501,#50502,
#50503,#50504,#50505,#50506,#50507,#50508,#50509,#50510,#50511,#50512,#50513,
#50514,#50515,#50516,#50517,#50518,#50519,#50520,#50521,#50522,#50523,#50524,
#50525,#50526,#50527,#50528,#50529,#50530,#50531,#50532,#50533,#50534),
 .UNSPECIFIED.,.F.,.F.,(4,2,2,2,2,2,2,2,2,2,2,2,2,2,2,2,2,2,2,2,2,2,2,2,
2,2,2,2,2,2,2,2,2,2,2,2,2,2,2,2,2,2,2,2,2,2,2,2,2,2,2,2,2,2,2,2,4),(9.99999991669717E-7,
0.0184447153223968,0.0263230505661795,0.036124778687421,0.0777207405050378,
0.102193231964045,0.121768138081197,0.136562874516093,0.155835590898569,
0.200176795636776,0.223236930617453,0.232676101620211,0.242768076763171,
0.281244235113264,0.318133316641436,0.334188540648712,0.349821365894987,
0.404181271018304,0.421248051626733,0.433948239560394,0.442676632303089,
0.45695402708308,0.498123802940828,0.526459180733287,0.541922825721667,
0.558274678127576,0.608828260701387,0.626375137247475,0.639298848005466,
0.648006132300929,0.661936527802842,0.702985516242036,0.731840841610424,
0.747335614023785,0.763614463819922,0.813238739648188,0.83939123519187,
0.849033315152608,0.858910393837397,0.899917598632736,0.935729657832649,
0.951576711293341,0.96742262672389,1.01680549308803,1.03610593709597,1.04980856829621,
1.05851147029703,1.07163514017831,1.11229204645002,1.14255802948317,1.1581480745398,
1.17429114011009,1.22532712172044,1.25069491457693,1.26029683909567,1.27022952044346,
1.29379821101641),.UNSPECIFIED.) ;
#1261=B_SPLINE_CURVE_WITH_KNOTS('',3,(#50540,#50541,#50542,#50543,#50544,
#50545,#50546,#50547,#50548,#50549,#50550,#50551,#50552,#50553,#50554,#50555,
#50556,#50557,#50558,#50559,#50560,#50561,#50562,#50563,#50564,#50565,#50566,
#50567,#50568,#50569,#50570,#50571,#50572,#50573,#50574,#50575,#50576,#50577,
#50578,#50579,#50580,#50581,#50582,#50583,#50584,#50585,#50586,#50587,#50588,
#50589,#50590,#50591,#50592,#50593,#50594,#50595,#50596,#50597,#50598,#50599,
#50600,#50601,#50602,#50603,#50604,#50605,#50606,#50607,#50608,#50609,#50610,
#50611,#50612,#50613,#50614,#50615,#50616,#50617,#50618,#50619,#50620,#50621,
#50622,#50623,#50624,#50625,#50626,#50627,#50628,#50629,#50630),
 .UNSPECIFIED.,.F.,.F.,(4,3,3,3,3,3,3,3,3,3,3,3,3,3,3,3,3,3,3,3,3,3,3,3,
3,3,3,3,3,3,4),(15.707963267949,15.8113162289403,15.9146430055769,16.0179789766908,
16.1214346358621,16.2249545823278,16.3224671580076,16.3286700874657,16.3947464669144,
16.3947981013555,16.489367670122,16.4989544967138,16.6029510560627,16.706819180176,
16.8106179355233,16.9143822485449,17.0181469982565,17.1220156832995,17.2259403207901,
17.3243464907781,17.3300437451009,17.3930767925987,17.3931266456449,17.488158788607,
17.4974450344715,17.6010532740212,17.606557916941,17.7106004897465,17.8145739596521,
17.9185190132978,17.9338965643494),.UNSPECIFIED.) ;
#1262=B_SPLINE_CURVE_WITH_KNOTS('',3,(#50632,#50633,#50634,#50635,#50636,
#50637,#50638,#50639,#50640,#50641,#50642,#50643,#50644,#50645,#50646,#50647,
#50648,#50649,#50650,#50651,#50652,#50653,#50654,#50655,#50656,#50657,#50658,
#50659,#50660,#50661,#50662,#50663,#50664,#50665,#50666,#50667,#50668,#50669,
#50670,#50671),.UNSPECIFIED.,.F.,.F.,(4,3,3,3,3,3,3,3,3,3,3,3,3,4),(14.3981410127767,
14.5041304628989,14.6100344213185,14.7159061169048,14.8217654368488,14.9276423442954,
15.0335668127656,15.1396478264459,15.2458169541302,15.3521882187467,15.3964695570661,
15.5190017212959,15.6402256956334,15.7079554188088),.UNSPECIFIED.) ;
#1263=B_SPLINE_CURVE_WITH_KNOTS('',3,(#50674,#50675,#50676,#50677,#50678,
#50679,#50680,#50681,#50682,#50683,#50684,#50685,#50686,#50687,#50688,#50689,
#50690,#50691,#50692,#50693,#50694,#50695,#50696,#50697,#50698,#50699,#50700,
#50701,#50702,#50703,#50704,#50705,#50706,#50707,#50708,#50709,#50710,#50711,
#50712,#50713,#50714,#50715,#50716,#50717,#50718,#50719,#50720,#50721,#50722,
#50723,#50724,#50725,#50726,#50727,#50728,#50729,#50730,#50731,#50732,#50733,
#50734,#50735,#50736,#50737,#50738,#50739,#50740,#50741,#50742,#50743,#50744,
#50745,#50746,#50747),.UNSPECIFIED.,.F.,.F.,(4,2,2,2,2,2,2,2,2,2,2,2,2,
2,2,2,2,2,2,2,2,2,2,2,2,2,2,2,2,2,2,2,2,2,2,2,4),(9.08164939039677E-5,0.00964446188066229,
0.0631727038946699,0.0833213424346721,0.0995270112478277,0.11521076241323,
0.168160574823218,0.192914913994012,0.202483681644903,0.212472572657854,
0.25229975169802,0.277505378195093,0.297440690943511,0.312324763000316,
0.331569412660729,0.375644072231997,0.398570725096213,0.408027582384325,
0.418068765141332,0.451392820401004,0.491734973859357,0.508171201472686,
0.52328080899074,0.548904583706971,0.592593255836169,0.607623400269449,
0.616321082217894,0.62824029431287,0.661333455958532,0.699795498757593,
0.715650850691533,0.731252650752003,0.763193487628226,0.808059994616459,
0.818142249781261,0.826085801679224,0.835754501023224),.UNSPECIFIED.) ;
#1264=B_SPLINE_CURVE_WITH_KNOTS('',3,(#50753,#50754,#50755,#50756,#50757,
#50758),.UNSPECIFIED.,.F.,.F.,(4,2,4),(0.688175935048327,0.722528389859189,
0.732483913740625),.UNSPECIFIED.) ;
#1265=B_SPLINE_CURVE_WITH_KNOTS('',3,(#50761,#50762,#50763,#50764,#50765,
#50766,#50767,#50768,#50769,#50770,#50771,#50772,#50773,#50774,#50775,#50776,
#50777,#50778),.UNSPECIFIED.,.F.,.F.,(4,2,2,2,2,2,2,2,4),(0.000326322779117739,
0.0053095587093796,0.0119345202360929,0.0491915472726964,0.0845062818898445,
0.100433841269843,0.116331511114054,0.149505453170145,0.152028373115396),
 .UNSPECIFIED.) ;
#1266=B_SPLINE_CURVE_WITH_KNOTS('',3,(#50784,#50785,#50786,#50787,#50788,
#50789,#50790,#50791,#50792,#50793,#50794,#50795,#50796,#50797,#50798,#50799,
#50800,#50801,#50802,#50803,#50804,#50805,#50806,#50807,#50808,#50809,#50810,
#50811,#50812,#50813,#50814,#50815,#50816,#50817,#50818,#50819,#50820,#50821,
#50822,#50823,#50824,#50825,#50826,#50827,#50828,#50829,#50830,#50831,#50832,
#50833,#50834,#50835,#50836,#50837,#50838,#50839),.UNSPECIFIED.,.F.,.F.,
(4,2,2,2,2,2,2,2,2,2,2,2,2,2,2,2,2,2,2,2,2,2,2,2,2,2,2,4),(1.98102711455768,
1.98958188275697,2.00867262502161,2.03197282727063,2.07443930051198,2.08480989656363,
2.09422631816803,2.11636340346817,2.16057507188391,2.18055526267638,2.19552374775884,
2.21498613387434,2.23909906769021,2.28155745479864,2.29133239102646,2.3011688929944,
2.33194922685791,2.37661912184551,2.39284432220525,2.40839273375275,2.43776671592168,
2.47890861126898,2.49264355354582,2.5014268582012,2.51487424116833,2.53350674094852,
2.5735412222785,2.58730157653673),.UNSPECIFIED.) ;
#1267=B_SPLINE_CURVE_WITH_KNOTS('',3,(#50840,#50841,#50842,#50843,#50844,
#50845,#50846,#50847,#50848,#50849,#50850,#50851,#50852,#50853,#50854,#50855,
#50856,#50857,#50858,#50859,#50860,#50861,#50862,#50863,#50864,#50865,#50866,
#50867,#50868,#50869,#50870,#50871,#50872,#50873,#50874,#50875,#50876,#50877,
#50878,#50879,#50880,#50881,#50882,#50883,#50884,#50885,#50886,#50887,#50888,
#50889,#50890,#50891,#50892,#50893,#50894,#50895,#50896,#50897,#50898,#50899,
#50900,#50901),.UNSPECIFIED.,.F.,.F.,(4,2,2,2,2,2,2,2,2,2,2,2,2,2,2,2,2,
2,2,2,2,2,2,2,2,2,2,2,2,2,4),(0.000740443363498194,0.0138349862975699,0.0295154725943613,
0.0790451299155813,0.106523846021425,0.116283064754404,0.126365470374231,
0.165172536751136,0.201324346128904,0.217457679525018,0.233551669346709,
0.267457400749719,0.296225634265475,0.313321898958139,0.322168521883493,
0.332525058471953,0.366431274633955,0.408017845899989,0.424714758522178,
0.439696860657482,0.4643168630784,0.505291340570378,0.520968983786635,0.529935246689459,
0.542398396489085,0.575204404091594,0.614943460595965,0.632807529475108,
0.649590886610583,0.66732217651446,0.688175935048327),.UNSPECIFIED.) ;
#1268=B_SPLINE_CURVE_WITH_KNOTS('',3,(#50903,#50904,#50905,#50906,#50907,
#50908,#50909,#50910,#50911,#50912,#50913,#50914,#50915,#50916,#50917,#50918,
#50919,#50920,#50921,#50922,#50923,#50924),.UNSPECIFIED.,.F.,.F.,(4,2,2,
2,2,2,2,2,2,2,4),(0.152028373115396,0.178271254198615,0.190732100705371,
0.201082878473419,0.210411761708287,0.232100824336856,0.282188910937535,
0.300143539111472,0.315112949643421,0.337038683452346,0.38114427299709),
 .UNSPECIFIED.) ;
#1269=B_SPLINE_CURVE_WITH_KNOTS('',3,(#50925,#50926,#50927,#50928,#50929,
#50930,#50931,#50932,#50933,#50934,#50935,#50936,#50937,#50938,#50939,#50940,
#50941,#50942,#50943,#50944,#50945,#50946,#50947,#50948,#50949,#50950,#50951,
#50952,#50953,#50954,#50955,#50956,#50957,#50958,#50959,#50960,#50961,#50962,
#50963,#50964,#50965,#50966,#50967,#50968,#50969,#50970,#50971,#50972,#50973,
#50974,#50975,#50976,#50977,#50978,#50979,#50980,#50981,#50982,#50983,#50984,
#50985,#50986,#50987,#50988,#50989,#50990,#50991,#50992,#50993,#50994,#50995,
#50996,#50997,#50998,#50999,#51000,#51001,#51002,#51003,#51004,#51005,#51006,
#51007,#51008,#51009,#51010,#51011,#51012,#51013,#51014,#51015,#51016,#51017,
#51018,#51019,#51020),.UNSPECIFIED.,.F.,.F.,(4,2,2,2,2,2,2,2,2,2,2,2,2,
2,2,2,2,2,2,2,2,2,2,2,2,2,2,2,2,2,2,2,2,2,2,2,2,2,2,2,2,2,2,2,2,2,2,4),
(9.99999998689338E-7,0.0174292635150208,0.0254334249445552,0.034789333326389,
0.0508440411265439,0.0912843741617236,0.111367032937248,0.127643504238079,
0.142995575497015,0.170701023554272,0.20580631807345,0.219337663136388,
0.230262195740999,0.239264644851289,0.257288082646908,0.297769585088541,
0.317929655952516,0.334037200357709,0.349643368751472,0.404845134658746,
0.428697831040931,0.438205956602896,0.448279237366973,0.487071365345615,
0.523692736645848,0.539737861694203,0.555412355415605,0.60929867965605,
0.634103560413446,0.643671473439017,0.653641438561538,0.69361372217156,
0.729510278592592,0.745504798507947,0.76120034152742,0.814297588916916,
0.839633215522294,0.849230500429995,0.859158345347323,0.899622697096617,
0.935800805641872,0.951658023515114,0.967490300857546,1.01703691034612,
1.03627966855327,1.04995760843149,1.05865975920911,1.06478356715028),
 .UNSPECIFIED.) ;
#1270=B_SPLINE_CURVE_WITH_KNOTS('',3,(#51026,#51027,#51028,#51029,#51030,
#51031,#51032,#51033,#51034,#51035,#51036,#51037,#51038,#51039,#51040,#51041,
#51042,#51043,#51044,#51045,#51046,#51047,#51048,#51049),.UNSPECIFIED.,
 .F.,.F.,(4,2,2,2,2,2,2,2,2,2,2,4),(2.35872509297639,2.36454743071151,2.38374966573916,
2.39854959804016,2.41821532462426,2.44290115786587,2.48383265586654,2.49371083602286,
2.50342578994992,2.52999234611409,2.57237232063052,2.58784193793521),
 .UNSPECIFIED.) ;
#1271=B_SPLINE_CURVE_WITH_KNOTS('',3,(#51051,#51052,#51053,#51054,#51055,
#51056,#51057,#51058,#51059,#51060,#51061,#51062,#51063,#51064,#51065,#51066,
#51067,#51068,#51069,#51070,#51071,#51072,#51073,#51074,#51075,#51076,#51077,
#51078,#51079,#51080,#51081,#51082,#51083,#51084,#51085,#51086,#51087,#51088,
#51089,#51090,#51091,#51092,#51093,#51094,#51095,#51096,#51097,#51098,#51099,
#51100,#51101,#51102,#51103,#51104,#51105,#51106,#51107,#51108,#51109,#51110,
#51111,#51112,#51113,#51114,#51115,#51116,#51117,#51118,#51119,#51120,#51121,
#51122,#51123,#51124,#51125,#51126,#51127,#51128,#51129,#51130,#51131,#51132,
#51133,#51134,#51135,#51136,#51137,#51138,#51139,#51140,#51141),
 .UNSPECIFIED.,.F.,.F.,(4,3,3,3,3,3,3,3,3,3,3,3,3,3,3,3,3,3,3,3,3,3,3,3,
3,3,3,3,3,3,4),(15.707963267949,15.8112952063224,15.9146002263953,16.0179137372553,
16.1213459971886,16.2248419869704,16.322362584987,16.3285328702908,16.394747429185,
16.3947981013556,16.4893602620961,16.4989462658854,16.6029345449639,16.7067943250266,
16.8105846969145,16.9143405893863,17.0180968837363,17.1219570901659,17.2258732220661,
17.3242843261941,17.3299681660503,17.3930783662191,17.3931266456449,17.4881614419572,
17.4974411081676,17.6010539690716,17.606553977256,17.710593186314,17.8145634851322,
17.9185056328178,17.9338925845213),.UNSPECIFIED.) ;
#1272=B_SPLINE_CURVE_WITH_KNOTS('',3,(#51143,#51144,#51145,#51146,#51147,
#51148,#51149,#51150,#51151,#51152,#51153,#51154,#51155,#51156,#51157,#51158,
#51159,#51160,#51161,#51162,#51163,#51164,#51165,#51166,#51167,#51168,#51169,
#51170,#51171,#51172,#51173,#51174,#51175,#51176,#51177,#51178,#51179,#51180,
#51181,#51182),.UNSPECIFIED.,.F.,.F.,(4,3,3,3,3,3,3,3,3,3,3,3,3,4),(14.3981410127768,
14.5041552849212,14.610085034542,14.7159837761904,14.8218708833437,14.9277762546341,
15.0337297999276,15.1398405743496,15.246039878247,15.3524416189491,15.3964695570662,
15.5190178529893,15.6402487977518,15.7079553869838),.UNSPECIFIED.) ;
#1273=B_SPLINE_CURVE_WITH_KNOTS('',3,(#51186,#51187,#51188,#51189,#51190,
#51191,#51192,#51193,#51194,#51195,#51196,#51197,#51198,#51199,#51200,#51201,
#51202,#51203,#51204,#51205,#51206,#51207,#51208,#51209,#51210,#51211,#51212,
#51213,#51214,#51215,#51216,#51217,#51218,#51219,#51220,#51221,#51222,#51223),
 .UNSPECIFIED.,.F.,.F.,(4,2,2,2,2,2,2,2,2,2,2,2,2,2,2,2,2,2,4),(0.000124769152405228,
0.00530283650978471,0.0119163883522527,0.0412949498779639,0.0805290761834309,
0.0975098147518704,0.112590970716538,0.1376147116016,0.175122950526936,
0.188971300360272,0.200067436032103,0.209050888113163,0.226868360620307,
0.258115591573283,0.289449081113609,0.305266632561115,0.321115120108506,
0.358122798341047,0.377579306682493),.UNSPECIFIED.) ;
#1274=B_SPLINE_CURVE_WITH_KNOTS('',3,(#51224,#51225,#51226,#51227,#51228,
#51229,#51230,#51231,#51232,#51233,#51234,#51235,#51236,#51237,#51238,#51239,
#51240,#51241,#51242,#51243,#51244,#51245,#51246,#51247,#51248,#51249,#51250,
#51251,#51252,#51253,#51254,#51255,#51256,#51257,#51258,#51259,#51260,#51261,
#51262,#51263,#51264,#51265,#51266,#51267,#51268,#51269,#51270,#51271,#51272,
#51273,#51274,#51275,#51276,#51277,#51278,#51279,#51280,#51281,#51282,#51283,
#51284,#51285),.UNSPECIFIED.,.F.,.F.,(4,2,2,2,2,2,2,2,2,2,2,2,2,2,2,2,2,
2,2,2,2,2,2,2,2,2,2,2,2,2,4),(9.999999931312E-7,0.0195843476304998,0.0296126220572481,
0.039313713778823,0.087896979280459,0.109292353934291,0.127460709263585,
0.142411374670944,0.163896663152293,0.207090939979833,0.227594924564628,
0.236857837595574,0.247394214498245,0.288505026781035,0.322917817070159,
0.338779331894746,0.354790271445652,0.392049970295044,0.427641430355377,
0.438989063679899,0.447877993643495,0.465017643283455,0.506415288618611,
0.526589770247727,0.542852862564029,0.558535544036832,0.614023558862245,
0.637818889649371,0.647353831033265,0.657516966897515,0.687313624506759),
 .UNSPECIFIED.) ;
#1275=B_SPLINE_CURVE_WITH_KNOTS('',3,(#51291,#51292,#51293,#51294,#51295,
#51296,#51297,#51298,#51299,#51300,#51301,#51302,#51303,#51304,#51305,#51306,
#51307,#51308,#51309,#51310,#51311,#51312,#51313,#51314,#51315,#51316,#51317,
#51318),.UNSPECIFIED.,.F.,.F.,(4,2,2,2,2,2,2,2,2,2,2,2,2,4),(0.459106433511841,
0.46421803988814,0.505059886921481,0.52089212016626,0.529860094088288,0.542206609381327,
0.57500566722291,0.615055906254151,0.632916344569532,0.649718573849782,
0.687670392249843,0.719981615275833,0.726884172836083,0.732443895036435),
 .UNSPECIFIED.) ;
#1276=B_SPLINE_CURVE_WITH_KNOTS('',3,(#51321,#51322,#51323,#51324,#51325,
#51326,#51327,#51328,#51329,#51330,#51331,#51332,#51333,#51334,#51335,#51336,
#51337,#51338,#51339,#51340,#51341,#51342,#51343,#51344,#51345,#51346,#51347,
#51348,#51349,#51350,#51351,#51352,#51353,#51354,#51355,#51356),
 .UNSPECIFIED.,.F.,.F.,(4,2,2,2,2,2,2,2,2,2,2,2,2,2,2,2,2,4),(0.000323627366430275,
0.00530468234356636,0.0119236929644194,0.0492443118740968,0.0845209544914468,
0.100443254054711,0.116328626559381,0.149319629535501,0.178221238025312,
0.190706602926174,0.2010706929436,0.210395000645647,0.232013989441357,0.281746612914986,
0.299850090908258,0.314796919879222,0.33640350897614,0.381145592574581),
 .UNSPECIFIED.) ;
#1277=B_SPLINE_CURVE_WITH_KNOTS('',3,(#51362,#51363,#51364,#51365,#51366,
#51367,#51368,#51369,#51370,#51371,#51372,#51373,#51374,#51375,#51376,#51377,
#51378,#51379,#51380,#51381,#51382,#51383,#51384,#51385,#51386,#51387,#51388,
#51389,#51390,#51391,#51392,#51393,#51394,#51395,#51396,#51397,#51398,#51399,
#51400,#51401,#51402,#51403,#51404,#51405,#51406,#51407,#51408,#51409,#51410,
#51411,#51412,#51413,#51414,#51415,#51416,#51417,#51418,#51419,#51420,#51421,
#51422,#51423,#51424,#51425,#51426,#51427,#51428,#51429,#51430,#51431,#51432,
#51433,#51434,#51435,#51436,#51437,#51438,#51439),.UNSPECIFIED.,.F.,.F.,
(4,2,2,2,2,2,2,2,2,2,2,2,2,2,2,2,2,2,2,2,2,2,2,2,2,2,2,2,2,2,2,2,2,2,2,
2,2,2,4),(0.458634629932413,0.468300840510139,0.484196861274041,0.50016509288339,
0.548723419503458,0.568340131710824,0.582191837596508,0.59094604609867,
0.604144741830108,0.64702296667436,0.675665519837222,0.691218868871637,
0.70767490065704,0.72781583866651,0.771167490136565,0.786448567224049,0.795305947097795,
0.807310050431355,0.840575503830774,0.87876863269993,0.894763994595969,
0.910638413268068,0.945390278369844,0.985953035480812,0.996560194075815,
1.0057826482125,1.0258531736437,1.06679615831433,1.08978974441653,1.1048418048654,
1.12234040877952,1.14239095099251,1.18372609071405,1.19842596399046,1.20722957825154,
1.21990039351384,1.23683119570789,1.28103441539912,1.29379172823382),
 .UNSPECIFIED.) ;
#1278=B_SPLINE_CURVE_WITH_KNOTS('',3,(#51440,#51441,#51442,#51443,#51444,
#51445,#51446,#51447,#51448,#51449,#51450,#51451,#51452,#51453,#51454,#51455,
#51456,#51457,#51458,#51459,#51460,#51461,#51462,#51463,#51464,#51465,#51466,
#51467,#51468,#51469,#51470,#51471,#51472,#51473,#51474,#51475,#51476,#51477,
#51478,#51479,#51480,#51481),.UNSPECIFIED.,.F.,.F.,(4,2,2,2,2,2,2,2,2,2,
2,2,2,2,2,2,2,2,2,2,4),(0.000743070825158928,0.0138183874138461,0.0294632506701812,
0.078638337800008,0.106479908835764,0.116255202249531,0.12632377121154,
0.165286117290309,0.201331912606227,0.217452660851885,0.233541178068994,
0.267395556774417,0.296229585496045,0.31334574782802,0.322192112681112,
0.332547173019449,0.366439965368885,0.407958097916761,0.424645227747565,
0.439621348066991,0.459106433511841),.UNSPECIFIED.) ;
#1279=B_SPLINE_CURVE_WITH_KNOTS('',3,(#51482,#51483,#51484,#51485,#51486,
#51487,#51488,#51489,#51490,#51491,#51492,#51493,#51494,#51495,#51496,#51497,
#51498,#51499,#51500,#51501,#51502,#51503,#51504,#51505,#51506,#51507,#51508,
#51509,#51510,#51511,#51512,#51513,#51514,#51515,#51516,#51517,#51518,#51519,
#51520,#51521,#51522,#51523,#51524,#51525,#51526,#51527,#51528,#51529,#51530,
#51531,#51532,#51533,#51534,#51535,#51536,#51537,#51538,#51539,#51540,#51541,
#51542,#51543,#51544,#51545,#51546,#51547,#51548,#51549,#51550,#51551,#51552,
#51553,#51554,#51555,#51556,#51557,#51558,#51559,#51560,#51561,#51562,#51563,
#51564,#51565,#51566,#51567,#51568,#51569,#51570,#51571,#51572,#51573,#51574,
#51575,#51576,#51577,#51578,#51579,#51580,#51581,#51582,#51583,#51584,#51585,
#51586,#51587,#51588,#51589,#51590,#51591,#51592,#51593,#51594,#51595,#51596,
#51597),.UNSPECIFIED.,.F.,.F.,(4,2,2,2,2,2,2,2,2,2,2,2,2,2,2,2,2,2,2,2,
2,2,2,2,2,2,2,2,2,2,2,2,2,2,2,2,2,2,2,2,2,2,2,2,2,2,2,2,2,2,2,2,2,2,2,2,
2,4),(1.00000002227832E-6,0.0112238415242,0.0192301303887427,0.0272771137891719,
0.0376302766663001,0.0801259453598099,0.103386439221757,0.122405930723958,
0.137206159944638,0.157073182616755,0.201283797023069,0.223466584261481,
0.232832546780453,0.243009558461636,0.286600593259539,0.319563822681232,
0.335294199052886,0.351238688388344,0.387813790697272,0.421429964250173,
0.433991334059334,0.442723428560765,0.457173786303744,0.499600153131827,
0.526857736851706,0.542239034458496,0.558729495818835,0.606205000027797,
0.625114473075408,0.638646897705653,0.647343441333917,0.660607608104126,
0.701332032884221,0.731305251402524,0.746867883638596,0.763022205076203,
0.813861763041297,0.839335603509961,0.848938126424361,0.858852205273181,
0.899417192833346,0.935509224651299,0.951358618903697,0.967186436715782,
1.01669943243797,1.03594198043776,1.04961797458601,1.05831696692786,1.07145231923964,
1.11210924043534,1.1423381118637,1.15792046651988,1.17405768397425,1.22508146764573,
1.25044280360822,1.26004140506794,1.26996816855601,1.29353464663662),
 .UNSPECIFIED.) ;
#1280=B_SPLINE_CURVE_WITH_KNOTS('',3,(#51603,#51604,#51605,#51606,#51607,
#51608,#51609,#51610,#51611,#51612,#51613,#51614,#51615,#51616,#51617,#51618,
#51619,#51620,#51621,#51622,#51623,#51624,#51625,#51626,#51627,#51628,#51629,
#51630,#51631,#51632,#51633,#51634,#51635,#51636,#51637,#51638,#51639,#51640,
#51641,#51642,#51643,#51644,#51645,#51646,#51647,#51648,#51649,#51650,#51651,
#51652,#51653,#51654,#51655,#51656,#51657,#51658,#51659,#51660,#51661,#51662,
#51663,#51664,#51665,#51666,#51667,#51668,#51669,#51670,#51671,#51672,#51673,
#51674,#51675,#51676,#51677,#51678,#51679,#51680,#51681,#51682,#51683,#51684,
#51685,#51686,#51687,#51688,#51689,#51690,#51691,#51692,#51693),
 .UNSPECIFIED.,.F.,.F.,(4,3,3,3,3,3,3,3,3,3,3,3,3,3,3,3,3,3,3,3,3,3,3,3,
3,3,3,3,3,3,4),(15.7079632679489,15.8112862145918,15.9145819569287,16.0178859166035,
16.1213082644554,16.2247941267765,16.3223176520483,16.328474632555,16.3947477954893,
16.3947981013556,16.489357726852,16.4989433816516,16.6029287721312,16.7067856596915,
16.8105731365216,16.9143261318643,17.0180795274943,17.1219368421535,17.2258500814329,
17.3242629549208,17.3299421537631,17.3930789381131,17.393126645645,17.4881627074684,
17.4974400050297,17.6010549229789,17.6065527859347,17.7105911054467,17.8145605873424,
17.9185020171076,17.9338911286497),.UNSPECIFIED.) ;
#1281=B_SPLINE_CURVE_WITH_KNOTS('',3,(#51695,#51696,#51697,#51698,#51699,
#51700,#51701,#51702,#51703,#51704,#51705,#51706,#51707,#51708,#51709,#51710,
#51711,#51712,#51713,#51714,#51715,#51716,#51717,#51718,#51719,#51720,#51721,
#51722,#51723,#51724,#51725,#51726,#51727,#51728,#51729,#51730,#51731,#51732,
#51733,#51734),.UNSPECIFIED.,.F.,.F.,(4,3,3,3,3,3,3,3,3,3,3,3,3,4),(14.3981410127768,
14.504165380809,14.6101056089343,14.716015321525,14.8219136896749,14.9278305855172,
15.0337958927558,15.1399186889816,15.2461301728942,15.3525441995258,15.3964695570662,
15.5190228063118,15.640255155241,15.7079553729118),.UNSPECIFIED.) ;
#1282=B_SPLINE_CURVE_WITH_KNOTS('',3,(#51738,#51739,#51740,#51741,#51742,
#51743,#51744,#51745,#51746,#51747,#51748,#51749,#51750,#51751,#51752,#51753,
#51754,#51755,#51756,#51757,#51758,#51759,#51760,#51761,#51762,#51763,#51764,
#51765,#51766,#51767,#51768,#51769,#51770,#51771,#51772,#51773,#51774,#51775),
 .UNSPECIFIED.,.F.,.F.,(4,2,2,2,2,2,2,2,2,2,2,2,2,2,2,2,2,2,4),(0.000123888491208429,
0.00530097158793175,0.0119135358149671,0.0413087913729525,0.0805378612701992,
0.0975159189419682,0.112586285557099,0.137553323954031,0.175117088689359,
0.188972222625648,0.200071653519827,0.209056561170478,0.22687817831067,
0.25814390936283,0.289431712038232,0.305242605840278,0.321088767321622,
0.358043788409661,0.377582389026477),.UNSPECIFIED.) ;
#1283=B_SPLINE_CURVE_WITH_KNOTS('',3,(#51776,#51777,#51778,#51779,#51780,
#51781,#51782,#51783,#51784,#51785,#51786,#51787,#51788,#51789,#51790,#51791,
#51792,#51793,#51794,#51795,#51796,#51797,#51798,#51799,#51800,#51801,#51802,
#51803,#51804,#51805,#51806,#51807,#51808,#51809,#51810,#51811,#51812,#51813,
#51814,#51815,#51816,#51817,#51818,#51819,#51820,#51821),.UNSPECIFIED.,
 .F.,.F.,(4,2,2,2,2,2,2,2,2,2,2,2,2,2,2,2,2,2,2,2,2,2,4),(9.62132622118833E-5,
0.0151686805222011,0.0250764405871821,0.0338681801368411,0.0468910424127618,
0.090942954515606,0.119087295147558,0.134543854258273,0.150904946987846,
0.199684592076087,0.218150734757442,0.231497901566788,0.240231336528935,
0.253830368051126,0.294788211242235,0.324295440911908,0.339901492363877,
0.356248065950247,0.405673464097533,0.423906443126347,0.437155718637114,
0.445919717201807,0.458255991027476),.UNSPECIFIED.) ;
#1284=B_SPLINE_CURVE_WITH_KNOTS('',3,(#51827,#51828,#51829,#51830,#51831,
#51832,#51833,#51834,#51835,#51836,#51837,#51838,#51839,#51840,#51841,#51842,
#51843,#51844,#51845,#51846,#51847,#51848,#51849,#51850,#51851,#51852),
 .UNSPECIFIED.,.F.,.F.,(4,2,2,2,2,2,2,2,2,2,2,2,4),(0.459096610162116,0.464484342986074,
0.505668080579649,0.520933833493707,0.529915992349492,0.54243499630205,
0.575250236487497,0.614798671012523,0.632654644680522,0.649413835000852,
0.667105487768125,0.722540336011944,0.73248042541764),.UNSPECIFIED.) ;
#1285=B_SPLINE_CURVE_WITH_KNOTS('',3,(#51855,#51856,#51857,#51858,#51859,
#51860,#51861,#51862,#51863,#51864,#51865,#51866,#51867,#51868,#51869,#51870,
#51871,#51872,#51873,#51874,#51875,#51876,#51877,#51878,#51879,#51880,#51881,
#51882,#51883,#51884,#51885,#51886,#51887,#51888,#51889,#51890),
 .UNSPECIFIED.,.F.,.F.,(4,2,2,2,2,2,2,2,2,2,2,2,2,2,2,2,2,4),(0.000330659804311743,
0.00532268279890478,0.0119652393155716,0.0489137712862508,0.0844466789380679,
0.100390177495993,0.116304718668483,0.149639300369354,0.178299187759877,
0.190741385079452,0.201082178857332,0.210410580183121,0.232117158451284,
0.282288937876845,0.300234024157747,0.315213791978961,0.337203182451053,
0.381142147507287),.UNSPECIFIED.) ;
#1286=B_SPLINE_CURVE_WITH_KNOTS('',3,(#51896,#51897,#51898,#51899,#51900,
#51901,#51902,#51903,#51904,#51905,#51906,#51907,#51908,#51909,#51910,#51911,
#51912,#51913,#51914,#51915,#51916,#51917,#51918,#51919,#51920,#51921,#51922,
#51923,#51924,#51925,#51926,#51927,#51928,#51929,#51930,#51931,#51932,#51933,
#51934,#51935,#51936,#51937,#51938,#51939,#51940,#51941,#51942,#51943,#51944,
#51945,#51946,#51947,#51948,#51949,#51950,#51951,#51952,#51953,#51954,#51955,
#51956,#51957,#51958,#51959,#51960,#51961,#51962,#51963,#51964,#51965,#51966,
#51967,#51968,#51969,#51970,#51971,#51972,#51973),.UNSPECIFIED.,.F.,.F.,
(4,2,2,2,2,2,2,2,2,2,2,2,2,2,2,2,2,2,2,2,2,2,2,2,2,2,2,2,2,2,2,2,2,2,2,
2,2,2,4),(1.29358094859399,1.30102621768796,1.31746349241148,1.33301830687605,
1.36175265660975,1.40289178715733,1.41695745330526,1.42571909490168,1.43874559827101,
1.4564822236342,1.50745376612977,1.52367647047814,1.53938760067812,1.57050924037248,
1.61088197490208,1.62361971586095,1.63240634535552,1.64691310392657,1.66812039125473,
1.71247092468887,1.72876553219963,1.74440242333882,1.77438578117767,1.81523711670643,
1.82858191899148,1.83732061561392,1.8509484004107,1.87005073834989,1.91688275202948,
1.93342514886333,1.94878576328709,1.97562922446084,2.02433805715359,2.035934070784,
2.04486283448474,2.0610646819781,2.08687744711799,2.11459664905666,2.12877604277013),
 .UNSPECIFIED.) ;
#1287=B_SPLINE_CURVE_WITH_KNOTS('',3,(#51974,#51975,#51976,#51977,#51978,
#51979,#51980,#51981,#51982,#51983,#51984,#51985,#51986,#51987,#51988,#51989,
#51990,#51991,#51992,#51993,#51994,#51995,#51996,#51997,#51998,#51999,#52000,
#52001,#52002,#52003,#52004,#52005,#52006,#52007,#52008,#52009,#52010,#52011,
#52012,#52013,#52014,#52015),.UNSPECIFIED.,.F.,.F.,(4,2,2,2,2,2,2,2,2,2,
2,2,2,2,2,2,2,2,2,2,4),(0.000736727244597652,0.0138630500639099,0.0296047208355221,
0.0797774319646349,0.10660912375222,0.116337527341353,0.12644712976289,
0.164941777871912,0.201310185331325,0.217468062584905,0.233571497463829,
0.267550915715147,0.296211966738743,0.313275697185141,0.322123670998576,
0.332482592175531,0.366416413504128,0.408124252474692,0.424838409521503,
0.439829856362813,0.459096610162116),.UNSPECIFIED.) ;
#1288=B_SPLINE_CURVE_WITH_KNOTS('',3,(#52016,#52017,#52018,#52019,#52020,
#52021,#52022,#52023,#52024,#52025,#52026,#52027,#52028,#52029,#52030,#52031,
#52032,#52033,#52034,#52035,#52036,#52037,#52038,#52039,#52040,#52041,#52042,
#52043,#52044,#52045,#52046,#52047,#52048,#52049,#52050,#52051,#52052,#52053,
#52054,#52055,#52056,#52057,#52058,#52059,#52060,#52061,#52062,#52063,#52064,
#52065,#52066,#52067,#52068,#52069,#52070,#52071,#52072,#52073,#52074,#52075,
#52076,#52077,#52078,#52079,#52080,#52081,#52082,#52083,#52084,#52085,#52086,
#52087,#52088,#52089,#52090,#52091,#52092,#52093,#52094,#52095,#52096,#52097,
#52098,#52099,#52100,#52101,#52102,#52103,#52104,#52105,#52106,#52107,#52108,
#52109,#52110,#52111,#52112,#52113,#52114,#52115,#52116,#52117,#52118,#52119,
#52120,#52121,#52122,#52123,#52124,#52125,#52126,#52127,#52128,#52129),
 .UNSPECIFIED.,.F.,.F.,(4,2,2,2,2,2,2,2,2,2,2,2,2,2,2,2,2,2,2,2,2,2,2,2,
2,2,2,2,2,2,2,2,2,2,2,2,2,2,2,2,2,2,2,2,2,2,2,2,2,2,2,2,2,2,2,2,4),(9.99999992887031E-7,
0.0186616073847396,0.0265145648287108,0.0364172205219696,0.0768552188462689,
0.101753994768879,0.121515268481445,0.136312633376872,0.155416829288432,
0.199810777329292,0.223169469646049,0.23262884996062,0.242689125040078,
0.281562678656109,0.31632308573852,0.33284556735728,0.348192875678435,0.375112560596473,
0.411072223212628,0.424735680902339,0.435735995351809,0.44475699666495,
0.462801730928076,0.503187277361918,0.523359270112846,0.53945352867169,
0.555087724667914,0.609993057856924,0.63412073326911,0.643643996789702,
0.653668525480734,0.702347086434316,0.731644458141428,0.747167476314061,
0.763395866290607,0.813517561529774,0.839394244676013,0.849020882378051,
0.858913106669476,0.899745295132745,0.935668108620726,0.951516768444482,
0.967356614754378,1.01678695434003,1.036066749431,1.04975998469544,1.05846175303386,
1.07159052398353,1.11224828740261,1.14249992235587,1.15808752367891,1.17422930654474,
1.22525639840622,1.25062473160401,1.26022582485268,1.27015675728782,1.29372477504308),
 .UNSPECIFIED.) ;
#1289=B_SPLINE_CURVE_WITH_KNOTS('',3,(#52135,#52136,#52137,#52138,#52139,
#52140,#52141,#52142,#52143,#52144,#52145,#52146,#52147,#52148,#52149,#52150,
#52151,#52152,#52153,#52154,#52155,#52156,#52157,#52158,#52159,#52160,#52161,
#52162,#52163,#52164,#52165,#52166,#52167,#52168,#52169,#52170,#52171,#52172,
#52173,#52174,#52175,#52176,#52177,#52178,#52179,#52180,#52181,#52182,#52183,
#52184,#52185,#52186,#52187,#52188,#52189,#52190,#52191,#52192,#52193,#52194,
#52195,#52196,#52197,#52198,#52199,#52200,#52201,#52202,#52203,#52204,#52205,
#52206,#52207,#52208,#52209,#52210,#52211,#52212,#52213,#52214,#52215,#52216,
#52217,#52218,#52219,#52220,#52221,#52222,#52223,#52224,#52225),
 .UNSPECIFIED.,.F.,.F.,(4,3,3,3,3,3,3,3,3,3,3,3,3,3,3,3,3,3,3,3,3,3,3,3,
3,3,3,3,3,3,4),(15.7079632679489,15.8113100481548,15.9146304174514,16.0179597637145,
16.121408506256,16.224921363305,16.3224364904957,16.3286295701974,16.3947467672854,
16.3947981013555,16.4893652458264,16.4989518365239,16.6029457144663,16.7068111290688,
16.8106071575924,16.9143687273476,17.0181307182028,17.1219966306611,17.2259184833068,
17.3243262425669,17.3300191259139,17.3930772951172,17.3931266456449,17.4881595111779,
17.4974436459181,17.6010532040285,17.6065565589844,17.7105979188205,17.8145702361085,
17.918514220579,17.9338952981833),.UNSPECIFIED.) ;
#1290=B_SPLINE_CURVE_WITH_KNOTS('',3,(#52227,#52228,#52229,#52230,#52231,
#52232,#52233,#52234,#52235,#52236,#52237,#52238,#52239,#52240,#52241,#52242,
#52243,#52244,#52245,#52246,#52247,#52248,#52249,#52250,#52251,#52252,#52253,
#52254,#52255,#52256,#52257,#52258,#52259,#52260,#52261,#52262,#52263,#52264,
#52265,#52266),.UNSPECIFIED.,.F.,.F.,(4,3,3,3,3,3,3,3,3,3,3,3,3,4),(14.3981410127767,
14.504137960918,14.61004971469,14.7159295917658,14.8217973215678,14.9276828478524,
15.0336161250156,15.1397061611793,15.2458844410812,15.3522649548022,15.3964695570661,
15.5190072170087,15.6402338511171,15.7079554096739),.UNSPECIFIED.) ;
#1291=B_SPLINE_CURVE_WITH_KNOTS('',3,(#52269,#52270,#52271,#52272,#52273,
#52274,#52275,#52276,#52277,#52278,#52279,#52280,#52281,#52282,#52283,#52284,
#52285,#52286,#52287,#52288,#52289,#52290,#52291,#52292,#52293,#52294,#52295,
#52296,#52297,#52298,#52299,#52300,#52301,#52302,#52303,#52304,#52305,#52306,
#52307,#52308,#52309,#52310,#52311,#52312,#52313,#52314,#52315,#52316,#52317,
#52318,#52319,#52320,#52321,#52322,#52323,#52324,#52325,#52326,#52327,#52328,
#52329,#52330,#52331,#52332,#52333,#52334,#52335,#52336,#52337,#52338,#52339,
#52340,#52341,#52342,#52343,#52344),.UNSPECIFIED.,.F.,.F.,(4,2,2,2,2,2,
2,2,2,2,2,2,2,2,2,2,2,2,2,2,2,2,2,2,2,2,2,2,2,2,2,2,2,2,2,2,2,4),(9.03212379660126E-5,
0.00957464539286387,0.063316634352145,0.083467899230563,0.0996371287737807,
0.115333995030373,0.167738796060251,0.192855728715468,0.202445810461218,
0.212412273542816,0.252486125819501,0.277582644409014,0.297467528730337,
0.312346809846427,0.331622833295928,0.375708714755005,0.39859634760076,
0.408047640128789,0.418091316914522,0.430056519706791,0.456400850306449,
0.494030306038328,0.509859880561215,0.525330099484413,0.555914229040669,
0.596369402008556,0.609242891445144,0.617871076698452,0.631503317897237,
0.65068604789205,0.700307170737338,0.716050896621134,0.731757816929863,
0.765959715718328,0.808239304508462,0.818258387720161,0.826154683199369,
0.835771767811734),.UNSPECIFIED.) ;
#1292=B_SPLINE_CURVE_WITH_KNOTS('',3,(#52351,#52352,#52353,#52354,#52355,
#52356,#52357,#52358,#52359,#52360,#52361,#52362,#52363,#52364,#52365,#52366,
#52367,#52368,#52369,#52370,#52371,#52372,#52373,#52374,#52375,#52376,#52377,
#52378,#52379,#52380,#52381,#52382,#52383,#52384,#52385,#52386,#52387,#52388,
#52389,#52390,#52391,#52392,#52393),.UNSPECIFIED.,.F.,.F.,(4,3,3,3,3,3,
3,3,3,3,3,3,3,3,4),(-17.9381921786934,-17.84255119842,-17.733347647525,
-17.6242554309927,-17.5152330417418,-17.4062390702213,-17.297153285934,
-17.1880265338616,-17.078692513265,-16.9804446462392,-16.9716447107412,
-16.9715852529195,-16.8695603658721,-16.8587108864595,-16.7648968801594),
 .UNSPECIFIED.) ;
#1293=B_SPLINE_CURVE_WITH_KNOTS('',3,(#52399,#52400,#52401,#52402,#52403,
#52404,#52405,#52406,#52407,#52408,#52409,#52410,#52411,#52412,#52413,#52414,
#52415,#52416,#52417,#52418,#52419,#52420,#52421,#52422,#52423,#52424,#52425,
#52426,#52427,#52428,#52429,#52430,#52431,#52432,#52433,#52434,#52435,#52436,
#52437,#52438,#52439,#52440,#52441,#52442,#52443,#52444,#52445,#52446,#52447,
#52448,#52449,#52450,#52451,#52452,#52453,#52454,#52455,#52456,#52457,#52458,
#52459,#52460,#52461,#52462,#52463,#52464,#52465,#52466,#52467,#52468,#52469,
#52470,#52471,#52472,#52473,#52474,#52475,#52476,#52477,#52478,#52479,#52480,
#52481,#52482,#52483,#52484,#52485,#52486,#52487,#52488,#52489,#52490,#52491,
#52492,#52493,#52494,#52495,#52496,#52497,#52498,#52499,#52500,#52501,#52502,
#52503,#52504,#52505,#52506,#52507,#52508,#52509,#52510,#52511,#52512,#52513,
#52514,#52515,#52516,#52517,#52518,#52519,#52520,#52521,#52522,#52523,#52524,
#52525,#52526,#52527,#52528,#52529,#52530,#52531,#52532,#52533,#52534,#52535,
#52536,#52537,#52538,#52539,#52540,#52541,#52542,#52543,#52544,#52545,#52546,
#52547,#52548,#52549,#52550,#52551,#52552,#52553,#52554,#52555,#52556,#52557,
#52558,#52559,#52560,#52561,#52562,#52563,#52564,#52565,#52566,#52567,#52568,
#52569,#52570,#52571,#52572,#52573,#52574,#52575,#52576,#52577,#52578,#52579,
#52580,#52581,#52582,#52583,#52584,#52585,#52586,#52587,#52588,#52589,#52590,
#52591,#52592,#52593,#52594,#52595,#52596,#52597),.UNSPECIFIED.,.F.,.F.,
(4,3,3,3,3,3,3,3,3,3,3,3,3,3,3,3,3,3,3,3,3,3,3,3,3,3,3,3,3,3,3,3,3,3,3,
3,3,3,3,3,3,3,3,3,3,3,3,3,3,3,3,3,3,3,3,3,3,3,3,3,3,3,3,3,3,3,4),(14.2294985582914,
14.3389460551526,14.4483384046449,14.5577163080432,14.6671996455868,14.7767350734239,
14.8864771704765,14.9748740828937,14.9749281643406,15.0752586873661,15.0846380345985,
15.1957153688525,15.3051222524056,15.414462240541,15.5237761597846,15.6361462969959,
15.7456017222214,15.8594292154257,15.9579697000886,15.9732013864772,15.97325670863,
16.0738005094969,16.0831956290521,16.1942443320355,16.3038817778961,16.4134522833054,
16.5229963245652,16.6351435566538,16.7448256020604,16.8582054274899,16.9568838883179,
16.9715259416915,16.9715852529194,17.0721629157137,17.0813044812162,17.1923806457152,
17.3018057577008,17.4111673178708,17.5205061818026,17.6328580856542,17.7423468637998,
17.8561303305043,17.9543267491162,17.9698505499765,17.9699137972087,18.0695586486444,
18.0792692192989,18.1903908595738,18.299435457365,18.4084113055606,18.5173598834856,
18.6300804979887,18.7391721543765,18.8537072479373,18.9524124448144,18.9682083299824,
18.9682423414981,19.0701276240468,19.0803889423434,19.1922977544505,19.3040678221704,
19.4157344265348,19.5273327084527,19.6389407654977,19.7505444309161,19.8622587312217,
19.9665708857875),.UNSPECIFIED.) ;
#1294=B_SPLINE_CURVE_WITH_KNOTS('',3,(#52599,#52600,#52601,#52602,#52603,
#52604,#52605,#52606,#52607,#52608,#52609,#52610,#52611,#52612,#52613,#52614,
#52615,#52616,#52617,#52618,#52619,#52620,#52621,#52622,#52623,#52624,#52625,
#52626,#52627,#52628,#52629,#52630,#52631,#52632,#52633,#52634,#52635,#52636,
#52637,#52638,#52639,#52640,#52641,#52642,#52643,#52644,#52645,#52646,#52647,
#52648,#52649,#52650,#52651,#52652,#52653,#52654,#52655,#52656,#52657,#52658,
#52659,#52660,#52661,#52662,#52663,#52664,#52665,#52666,#52667,#52668,#52669,
#52670,#52671,#52672,#52673,#52674,#52675,#52676,#52677,#52678,#52679,#52680,
#52681,#52682,#52683,#52684,#52685,#52686,#52687,#52688,#52689,#52690,#52691,
#52692,#52693,#52694,#52695,#52696,#52697,#52698,#52699,#52700,#52701,#52702),
 .UNSPECIFIED.,.F.,.F.,(4,2,2,2,2,2,2,2,2,2,2,2,2,2,2,2,2,2,2,2,2,2,2,2,
2,2,2,2,2,2,2,2,2,2,2,2,2,2,2,2,2,2,2,2,2,2,2,2,2,2,2,4),(1.10906469945444,
1.11644179379854,1.13767404484332,1.16925937097399,1.18614807304508,1.19521787211305,
1.2079746259431,1.22628467027725,1.26313703689709,1.27862570307869,1.29601903027109,
1.31662312511589,1.35083366981395,1.36044435318284,1.37150334131016,1.40310804188015,
1.4311789832774,1.44633688717477,1.46421088555474,1.4859701109504,1.5186366830229,
1.52796710429679,1.53967142713642,1.55546837692492,1.59652752283311,1.61207491358455,
1.62932310833252,1.64959144102805,1.68487769212845,1.69438184985283,1.70570010383403,
1.72064458309577,1.76585042140126,1.78102778991588,1.7996551503634,1.84829086317497,
1.85912184122804,1.86883008853204,1.88048923002279,1.90864659496912,1.93331757477378,
1.94837534891107,1.96720425580469,2.00360604212628,2.0205483517595,2.02963733862127,
2.04245354220867,2.06087185016348,2.0972058647788,2.11276529158488,2.13033849194594,
2.1591307752799),.UNSPECIFIED.) ;
#1295=B_SPLINE_CURVE_WITH_KNOTS('',3,(#52708,#52709,#52710,#52711,#52712,
#52713,#52714,#52715,#52716,#52717),.UNSPECIFIED.,.F.,.F.,(4,2,2,2,4),(0.000104814392196666,
0.0139942526189345,0.0233080874743996,0.0329393031166841,0.0589549240516137),
 .UNSPECIFIED.) ;
#1296=B_SPLINE_CURVE_WITH_KNOTS('',3,(#52719,#52720,#52721,#52722,#52723,
#52724,#52725,#52726,#52727,#52728,#52729,#52730,#52731,#52732,#52733,#52734,
#52735,#52736,#52737,#52738,#52739,#52740,#52741,#52742,#52743,#52744,#52745,
#52746,#52747,#52748,#52749,#52750,#52751,#52752,#52753,#52754,#52755,#52756,
#52757,#52758,#52759,#52760,#52761,#52762,#52763,#52764,#52765,#52766,#52767,
#52768,#52769,#52770,#52771,#52772,#52773,#52774,#52775,#52776,#52777,#52778,
#52779,#52780,#52781,#52782,#52783,#52784,#52785,#52786,#52787,#52788,#52789,
#52790,#52791,#52792,#52793,#52794,#52795,#52796,#52797,#52798,#52799,#52800,
#52801,#52802,#52803,#52804,#52805,#52806,#52807,#52808,#52809,#52810,#52811,
#52812,#52813,#52814,#52815,#52816,#52817,#52818,#52819,#52820,#52821,#52822,
#52823,#52824,#52825,#52826,#52827,#52828,#52829,#52830,#52831,#52832,#52833,
#52834,#52835,#52836,#52837,#52838,#52839,#52840,#52841,#52842,#52843,#52844,
#52845,#52846,#52847,#52848),.UNSPECIFIED.,.F.,.F.,(4,3,3,3,3,3,3,3,3,3,
3,3,3,3,3,3,3,3,3,3,3,3,3,3,3,3,3,3,3,3,3,3,3,3,3,3,3,3,3,3,3,3,3,4),(-3.84638257448865,
-3.73820981375279,-3.63015427375729,-3.52217346020946,-3.41422462150895,
-3.30618883650797,-3.19811283732308,-3.0898366058282,-2.99504494316089,
-2.99498563286816,-2.89440797106735,-2.88526640865405,-2.77419024364464,
-2.66476513576646,-2.55540357970902,-2.44606471989407,-2.33371281206525,
-2.22422403802765,-2.11044056330321,-2.01224414737772,-1.996720335184,-1.99665708857877,
-1.89701223877746,-1.887301676346,-1.77618003483892,-1.66713544615312,-1.55815960676097,
-1.44921103732509,-1.33649041406617,-1.22739876529517,-1.11286365479228,
-1.01415847169605,-0.998362556174536,-0.998328544289387,-0.896443265106951,
-0.886181926854384,-0.774273098472086,-0.662503014698027,-0.550836394538628,
-0.439238097123404,-0.327630025180105,-0.216026345188961,-0.10431203103316,
-1.15547111670624E-13),.UNSPECIFIED.) ;
#1297=B_SPLINE_CURVE_WITH_KNOTS('',3,(#52852,#52853,#52854,#52855,#52856,
#52857,#52858,#52859,#52860,#52861,#52862,#52863,#52864,#52865,#52866,#52867,
#52868,#52869,#52870,#52871,#52872,#52873,#52874,#52875,#52876,#52877,#52878,
#52879,#52880,#52881,#52882,#52883,#52884,#52885,#52886,#52887,#52888,#52889,
#52890,#52891,#52892,#52893,#52894,#52895,#52896,#52897,#52898,#52899,#52900,
#52901,#52902,#52903,#52904,#52905,#52906,#52907,#52908,#52909,#52910,#52911,
#52912,#52913,#52914,#52915,#52916,#52917,#52918,#52919,#52920,#52921,#52922,
#52923,#52924,#52925,#52926,#52927,#52928,#52929,#52930,#52931,#52932,#52933,
#52934,#52935,#52936,#52937,#52938,#52939,#52940,#52941,#52942,#52943,#52944,
#52945,#52946,#52947,#52948,#52949,#52950,#52951,#52952,#52953,#52954,#52955,
#52956,#52957,#52958,#52959,#52960,#52961,#52962,#52963,#52964,#52965,#52966,
#52967,#52968,#52969,#52970,#52971,#52972,#52973,#52974,#52975,#52976,#52977,
#52978,#52979,#52980,#52981,#52982,#52983,#52984,#52985,#52986,#52987,#52988,
#52989,#52990,#52991,#52992,#52993,#52994,#52995,#52996,#52997,#52998,#52999,
#53000,#53001,#53002,#53003,#53004,#53005,#53006,#53007,#53008,#53009,#53010,
#53011,#53012,#53013,#53014,#53015,#53016,#53017,#53018,#53019,#53020,#53021,
#53022,#53023,#53024,#53025,#53026,#53027,#53028,#53029,#53030,#53031,#53032,
#53033,#53034,#53035,#53036,#53037,#53038,#53039,#53040,#53041,#53042,#53043,
#53044,#53045,#53046,#53047,#53048,#53049,#53050),.UNSPECIFIED.,.F.,.F.,
(4,3,3,3,3,3,3,3,3,3,3,3,3,3,3,3,3,3,3,3,3,3,3,3,3,3,3,3,3,3,3,3,3,3,3,
3,3,3,3,3,3,3,3,3,3,3,3,3,3,3,3,3,3,3,3,3,3,3,3,3,3,3,3,3,3,3,4),(2.02837884434118,
2.1240196911459,2.23322324616186,2.34231546682411,2.45133786021298,2.56033183587889,
2.66941762430942,2.77854438053048,2.88787840524992,2.98612627157822,2.99492617411531,
2.99498563286811,3.095559170198,3.10492126614826,3.21597038002441,3.32560646520527,
3.43517633163416,3.54472045447418,3.65686888514501,3.76655278708082,3.87993348211915,
3.9785834862159,3.99325866988823,3.99331417715749,4.0937196533305,4.10302861870553,
4.2141053815482,4.32351415904549,4.43285503962457,4.54216885140771,4.6545373189175,
4.76399016764901,4.87781644454794,4.97628313139962,4.99158865070613,4.99164272144687,
5.09203035032617,5.10141775971842,5.21248694797065,5.32195859236235,5.43136300708735,
5.54074091187526,5.6530485003405,5.7625660676359,5.87626866668607,5.97482553317191,
5.98991776896683,5.98997126573624,6.09040645084578,6.09976781763968,6.21083431668792,
6.32032871950448,6.42975630058055,6.53915774670571,6.65144326253569,6.76098505495927,
6.87464243249244,6.97319341710015,6.98824593552854,6.98829981002562,7.08940621512439,
7.09951479840276,7.21054371655544,7.32140209163783,7.43216080950087,7.54286222160147,
7.59300756235177),.UNSPECIFIED.) ;
#1298=B_SPLINE_CURVE_WITH_KNOTS('',3,(#53051,#53052,#53053,#53054,#53055,
#53056,#53057,#53058),.UNSPECIFIED.,.F.,.F.,(4,2,2,4),(-1.10892786928915,
-1.08701579877003,-1.05545668530014,-1.05009726896819),.UNSPECIFIED.) ;
#1299=B_SPLINE_CURVE_WITH_KNOTS('',3,(#53065,#53066,#53067,#53068,#53069,
#53070,#53071,#53072,#53073,#53074,#53075,#53076,#53077,#53078,#53079,#53080,
#53081,#53082,#53083,#53084,#53085,#53086,#53087,#53088,#53089,#53090,#53091,
#53092,#53093,#53094,#53095,#53096,#53097,#53098,#53099,#53100,#53101,#53102,
#53103,#53104,#53105,#53106,#53107),.UNSPECIFIED.,.F.,.F.,(4,3,3,3,3,3,
3,3,3,3,3,3,3,3,4),(-17.9382970979382,-17.8425540308235,-17.7333535479141,
-17.6242644024251,-17.5152450868105,-17.4062541910623,-17.2971714758685,
-17.1880477943208,-17.0787168207789,-16.9804683437631,-16.9716440068398,
-16.9715852529196,-16.8695599004832,-16.8587139242793,-16.7649015929075),
 .UNSPECIFIED.) ;
#1300=B_SPLINE_CURVE_WITH_KNOTS('',3,(#53113,#53114,#53115,#53116,#53117,
#53118,#53119,#53120,#53121,#53122,#53123,#53124,#53125,#53126,#53127,#53128,
#53129,#53130,#53131,#53132,#53133,#53134,#53135,#53136,#53137,#53138,#53139,
#53140,#53141,#53142,#53143,#53144,#53145,#53146,#53147,#53148,#53149,#53150,
#53151,#53152,#53153,#53154,#53155,#53156,#53157,#53158,#53159,#53160,#53161,
#53162,#53163,#53164,#53165,#53166,#53167,#53168,#53169,#53170,#53171,#53172,
#53173,#53174,#53175,#53176,#53177,#53178,#53179,#53180,#53181,#53182,#53183,
#53184,#53185,#53186,#53187,#53188,#53189,#53190,#53191,#53192,#53193,#53194,
#53195,#53196,#53197,#53198,#53199,#53200,#53201,#53202,#53203,#53204,#53205,
#53206,#53207,#53208,#53209,#53210,#53211,#53212,#53213,#53214,#53215,#53216,
#53217,#53218,#53219,#53220,#53221,#53222,#53223,#53224,#53225,#53226,#53227,
#53228,#53229,#53230,#53231,#53232,#53233,#53234,#53235,#53236,#53237,#53238,
#53239,#53240,#53241,#53242,#53243,#53244,#53245,#53246,#53247,#53248,#53249,
#53250,#53251,#53252,#53253,#53254,#53255,#53256,#53257,#53258,#53259,#53260,
#53261,#53262,#53263,#53264,#53265,#53266,#53267,#53268,#53269,#53270,#53271,
#53272,#53273,#53274,#53275,#53276,#53277,#53278,#53279,#53280,#53281,#53282,
#53283,#53284,#53285,#53286,#53287,#53288,#53289,#53290,#53291,#53292,#53293,
#53294,#53295,#53296,#53297,#53298,#53299,#53300,#53301,#53302,#53303,#53304,
#53305,#53306,#53307,#53308,#53309,#53310,#53311),.UNSPECIFIED.,.F.,.F.,
(4,3,3,3,3,3,3,3,3,3,3,3,3,3,3,3,3,3,3,3,3,3,3,3,3,3,3,3,3,3,3,3,3,3,3,
3,3,3,3,3,3,3,3,3,3,3,3,3,3,3,3,3,3,3,3,3,3,3,3,3,3,3,3,3,3,3,4),(14.2295041962807,
14.3389527740686,14.4483462151971,14.5577252201524,14.6672096681762,14.7767462138682,
14.8864894271704,14.9748742139681,14.9749281643407,15.0752586275347,15.084638833907,
15.1957160682474,15.3051236621828,15.4144643261432,15.5237788860543,15.6361483416983,
15.7456043152617,15.8594305119459,15.9579714051649,15.973201766293,15.9732567086301,
16.0737983632465,16.0831953062282,16.1942440495646,16.303880929867,16.4134507779162,
16.5229940690511,16.6351418650182,16.744822928944,16.8582040909317,16.9568843065312,
16.9715266399014,16.9715852529195,17.07216214021,17.081301466679,17.1923780079952,
17.3018000786669,17.411158590375,17.5204943992678,17.6328492487531,17.7423349694877,
17.8561243833483,17.9543186908075,17.9698510293629,17.9699137972089,18.0695572552717,
18.0792613911935,18.1903840099816,18.2994213549179,18.4083901820114,18.5173319801007,
18.6300595704501,18.7391451195388,18.8536937305186,18.9523880995745,18.9682080461121,
18.9682423414983,19.0701250867853,19.080401850269,19.1923233312894,19.3041058992852,
19.415784805444,19.5273951605258,19.6390148289136,19.7506298546352,19.8623549565011,
19.9665708857876),.UNSPECIFIED.) ;
#1301=B_SPLINE_CURVE_WITH_KNOTS('',3,(#53313,#53314,#53315,#53316,#53317,
#53318,#53319,#53320,#53321,#53322,#53323,#53324,#53325,#53326,#53327,#53328,
#53329,#53330,#53331,#53332,#53333,#53334,#53335,#53336,#53337,#53338,#53339,
#53340,#53341,#53342,#53343,#53344,#53345,#53346,#53347,#53348,#53349,#53350,
#53351,#53352,#53353,#53354,#53355,#53356,#53357,#53358,#53359,#53360,#53361,
#53362,#53363,#53364,#53365,#53366,#53367,#53368,#53369,#53370,#53371,#53372,
#53373,#53374,#53375,#53376,#53377,#53378,#53379,#53380,#53381,#53382,#53383,
#53384,#53385,#53386,#53387,#53388,#53389,#53390,#53391,#53392,#53393,#53394,
#53395,#53396,#53397,#53398,#53399,#53400,#53401,#53402,#53403,#53404,#53405,
#53406,#53407,#53408,#53409,#53410,#53411,#53412,#53413,#53414,#53415,#53416),
 .UNSPECIFIED.,.F.,.F.,(4,2,2,2,2,2,2,2,2,2,2,2,2,2,2,2,2,2,2,2,2,2,2,2,
2,2,2,2,2,2,2,2,2,2,2,2,2,2,2,2,2,2,2,2,2,2,2,2,2,2,2,4),(1.10921089576887,
1.1165407497641,1.1377191197715,1.16909543804062,1.18618906391538,1.19528608214462,
1.20790932058952,1.22587909147871,1.26360125462676,1.2790532194091,1.29656844924673,
1.31745268685726,1.35276232031494,1.36183513301177,1.37401990875906,1.39092675320549,
1.43145123251076,1.44661521359877,1.46448147982816,1.48621574539827,1.5189855364488,
1.52831265082856,1.54003542102944,1.5558706418114,1.59684321214082,1.61240079929573,
1.62963855734371,1.64987657864815,1.68530409836741,1.69479824642061,1.70614484450102,
1.72114792974254,1.76623728942954,1.78142302429321,1.80004020942435,1.84859367092729,
1.85948803106446,1.86915885371709,1.88073863170467,1.9083848327913,1.93384705100083,
1.94890686995806,1.9677744135678,2.00274590059768,2.02036028629064,2.02949399608927,
2.04158020440638,2.05821101212464,2.09925252968438,2.11460315827409,2.13296303919467,
2.15968734072935),.UNSPECIFIED.) ;
#1302=B_SPLINE_CURVE_WITH_KNOTS('',3,(#53422,#53423,#53424,#53425,#53426,
#53427,#53428,#53429,#53430,#53431),.UNSPECIFIED.,.F.,.F.,(4,2,2,2,4),(0.000104517902925009,
0.0138899081821579,0.0231300525877348,0.0326747507448214,0.0589272293900401),
 .UNSPECIFIED.) ;
#1303=B_SPLINE_CURVE_WITH_KNOTS('',3,(#53433,#53434,#53435,#53436,#53437,
#53438,#53439,#53440,#53441,#53442,#53443,#53444,#53445,#53446,#53447,#53448,
#53449,#53450,#53451,#53452,#53453,#53454,#53455,#53456,#53457,#53458,#53459,
#53460,#53461,#53462,#53463,#53464,#53465,#53466,#53467,#53468,#53469,#53470,
#53471,#53472,#53473,#53474,#53475,#53476,#53477,#53478,#53479,#53480,#53481,
#53482,#53483,#53484,#53485,#53486,#53487,#53488,#53489,#53490,#53491,#53492,
#53493,#53494,#53495,#53496,#53497,#53498,#53499,#53500,#53501,#53502,#53503,
#53504,#53505,#53506,#53507,#53508,#53509,#53510,#53511,#53512,#53513,#53514,
#53515,#53516,#53517,#53518,#53519,#53520,#53521,#53522,#53523,#53524,#53525,
#53526,#53527,#53528,#53529,#53530,#53531,#53532,#53533,#53534,#53535,#53536,
#53537,#53538,#53539,#53540,#53541,#53542,#53543,#53544,#53545,#53546,#53547,
#53548,#53549,#53550,#53551,#53552,#53553,#53554,#53555,#53556,#53557,#53558,
#53559,#53560,#53561,#53562),.UNSPECIFIED.,.F.,.F.,(4,3,3,3,3,3,3,3,3,3,
3,3,3,3,3,3,3,3,3,3,3,3,3,3,3,3,3,3,3,3,3,3,3,3,3,3,3,3,3,3,3,3,3,4),(-3.84638258138888,
-3.73821081936309,-3.63015636590979,-3.52217672366053,-3.41422914122735,
-3.30619474264527,-3.19812020357506,-3.08984554459139,-2.99504424490879,
-2.99498563286818,-2.89440874631802,-2.88526942317335,-2.77419288134903,
-2.6647708147905,-2.55541230721001,-2.44607650245855,-2.33372164898861,
-2.22423593241171,-2.11044651049525,-2.01225220580641,-1.9967198557535,
-1.99665708857879,-1.89701363271621,-1.88730950597383,-1.77618688576327,
-1.66714955140073,-1.55818073455541,-1.44923894637485,-1.33651134585349,
-1.22742580572388,-1.11287717500664,-1.01418282151687,-0.998362840074688,
-0.998328544289396,-0.896445802515984,-0.886169017124272,-0.774247518042122,
-0.662464932220208,-0.550786008513675,-0.439175636205823,-0.327555951244137,
-0.215940909303158,-0.104215792009426,-1.01437695921273E-13),
 .UNSPECIFIED.) ;
#1304=B_SPLINE_CURVE_WITH_KNOTS('',3,(#53566,#53567,#53568,#53569,#53570,
#53571,#53572,#53573,#53574,#53575,#53576,#53577,#53578,#53579,#53580,#53581,
#53582,#53583,#53584,#53585,#53586,#53587,#53588,#53589,#53590,#53591,#53592,
#53593,#53594,#53595,#53596,#53597,#53598,#53599,#53600,#53601,#53602,#53603,
#53604,#53605,#53606,#53607,#53608,#53609,#53610,#53611,#53612,#53613,#53614,
#53615,#53616,#53617,#53618,#53619,#53620,#53621,#53622,#53623,#53624,#53625,
#53626,#53627,#53628,#53629,#53630,#53631,#53632,#53633,#53634,#53635,#53636,
#53637,#53638,#53639,#53640,#53641,#53642,#53643,#53644,#53645,#53646,#53647,
#53648,#53649,#53650,#53651,#53652,#53653,#53654,#53655,#53656,#53657,#53658,
#53659,#53660,#53661,#53662,#53663,#53664,#53665,#53666,#53667,#53668,#53669,
#53670,#53671,#53672,#53673,#53674,#53675,#53676,#53677,#53678,#53679,#53680,
#53681,#53682,#53683,#53684,#53685,#53686,#53687,#53688,#53689,#53690,#53691,
#53692,#53693,#53694,#53695,#53696,#53697,#53698,#53699,#53700,#53701,#53702,
#53703,#53704,#53705,#53706,#53707,#53708,#53709,#53710,#53711,#53712,#53713,
#53714,#53715,#53716,#53717,#53718,#53719,#53720,#53721,#53722,#53723,#53724,
#53725,#53726,#53727,#53728,#53729,#53730,#53731,#53732,#53733,#53734,#53735,
#53736,#53737,#53738,#53739,#53740,#53741,#53742,#53743,#53744,#53745,#53746,
#53747,#53748,#53749,#53750,#53751,#53752,#53753,#53754,#53755,#53756,#53757,
#53758,#53759,#53760,#53761,#53762,#53763,#53764),.UNSPECIFIED.,.F.,.F.,
(4,3,3,3,3,3,3,3,3,3,3,3,3,3,3,3,3,3,3,3,3,3,3,3,3,3,3,3,3,3,3,3,3,3,3,
3,3,3,3,3,3,3,3,3,3,3,3,3,3,3,3,3,3,3,3,3,3,3,3,3,3,3,3,3,3,3,4),(2.02827393470618,
2.12401685884403,2.2332173459281,2.34230649559061,2.45132581537725,2.5603167152955,
2.66939943464312,2.77852312034262,2.88785409799839,2.98610257413192,2.99492687797345,
2.99498563286815,3.09556048440326,3.10492009829771,3.21596935815519,3.32560452798313,
3.43517357277873,3.54471696644991,3.65686626912681,3.76654966682786,3.87993192199269,
3.97857994078247,3.9932590621024,3.99331417715753,4.09372001119541,4.10302908632675,
4.21410579071677,4.32351514116986,4.43285663280961,4.54217109304234,4.65453900014349,
4.76399258414707,4.877817652797,4.97628416232411,4.99158878638053,4.99164272144692,
5.09203073599517,5.10141887365017,5.21248792266094,5.32196067405111,5.43136619139733,
5.54074519366075,5.65305171167964,5.76257035608005,5.87627081090818,5.97482854624451,
5.98991786319383,5.9899712657363,6.0904065550125,6.09976804010903,6.21083451134862,
6.32032909358392,6.4297568381361,6.53915843204149,6.65144377653754,6.76098567858234,
6.87464274430401,6.97319398049008,6.9882460799675,6.98829981002569,7.08940605201705,
7.09951457708467,7.2105432634816,7.32140139284322,7.43215985716547,7.54286100567203,
7.59300756235177),.UNSPECIFIED.) ;
#1305=B_SPLINE_CURVE_WITH_KNOTS('',3,(#53765,#53766,#53767,#53768,#53769,
#53770,#53771,#53772),.UNSPECIFIED.,.F.,.F.,(4,2,2,4),(-1.10892889037454,
-1.08702947025092,-1.0554688082652,-1.05009743737373),.UNSPECIFIED.) ;
#1306=B_SPLINE_CURVE_WITH_KNOTS('',3,(#53779,#53780,#53781,#53782,#53783,
#53784,#53785,#53786,#53787,#53788,#53789,#53790,#53791,#53792,#53793,#53794,
#53795,#53796,#53797,#53798,#53799,#53800,#53801,#53802,#53803,#53804,#53805,
#53806,#53807,#53808,#53809,#53810,#53811,#53812,#53813,#53814,#53815,#53816,
#53817,#53818,#53819,#53820,#53821),.UNSPECIFIED.,.F.,.F.,(4,3,3,3,3,3,
3,3,3,3,3,3,3,3,4),(-17.9379151410847,-17.8425432679218,-17.7333309013929,
-17.6242298257075,-17.5151985361325,-17.4061956253956,-17.29710087273,-17.1879651215466,
-17.0786221284184,-16.9803757539028,-16.9716466477506,-16.9715852529197,
-16.8695608598858,-16.8587017272605,-16.7648831157624),.UNSPECIFIED.) ;
#1307=B_SPLINE_CURVE_WITH_KNOTS('',3,(#53827,#53828,#53829,#53830,#53831,
#53832,#53833,#53834,#53835,#53836,#53837,#53838,#53839,#53840,#53841,#53842,
#53843,#53844,#53845,#53846,#53847,#53848,#53849,#53850,#53851,#53852,#53853,
#53854,#53855,#53856,#53857,#53858,#53859,#53860,#53861,#53862,#53863,#53864,
#53865,#53866,#53867,#53868,#53869,#53870,#53871,#53872,#53873,#53874,#53875,
#53876,#53877,#53878,#53879,#53880,#53881,#53882,#53883,#53884,#53885,#53886,
#53887,#53888,#53889,#53890,#53891,#53892,#53893,#53894,#53895,#53896,#53897,
#53898,#53899,#53900,#53901,#53902,#53903,#53904,#53905,#53906,#53907,#53908,
#53909,#53910,#53911,#53912,#53913,#53914,#53915,#53916,#53917,#53918,#53919,
#53920,#53921,#53922,#53923,#53924,#53925,#53926,#53927,#53928,#53929,#53930,
#53931,#53932,#53933,#53934,#53935,#53936,#53937,#53938,#53939,#53940,#53941,
#53942,#53943,#53944,#53945,#53946,#53947,#53948,#53949,#53950,#53951,#53952,
#53953,#53954,#53955,#53956,#53957,#53958,#53959,#53960,#53961,#53962,#53963,
#53964,#53965,#53966,#53967,#53968,#53969,#53970,#53971,#53972,#53973,#53974,
#53975,#53976,#53977,#53978,#53979,#53980,#53981,#53982,#53983,#53984,#53985,
#53986,#53987,#53988,#53989,#53990,#53991,#53992,#53993,#53994,#53995,#53996,
#53997,#53998,#53999,#54000,#54001,#54002,#54003,#54004,#54005,#54006,#54007,
#54008,#54009,#54010,#54011,#54012,#54013,#54014,#54015,#54016,#54017,#54018,
#54019,#54020,#54021,#54022,#54023,#54024,#54025),.UNSPECIFIED.,.F.,.F.,
(4,3,3,3,3,3,3,3,3,3,3,3,3,3,3,3,3,3,3,3,3,3,3,3,3,3,3,3,3,3,3,3,3,3,3,
3,3,3,3,3,3,3,3,3,3,3,3,3,3,3,3,3,3,3,3,3,3,3,3,3,3,3,3,3,3,3,4),(14.2294810629657,
14.3389251840774,14.4483141319448,14.5576886102697,14.6671685063617,14.77670047614,
14.8864391301828,14.9748737855452,14.9749281643408,15.075258940077,15.0846355867601,
15.1957132269939,15.3051179526876,15.414455895575,15.523767884172,15.6361400902866,
15.745593885446,15.8594252970381,15.9579642345869,15.9732003327611,15.9732567086302,
16.0738069045067,16.0831975064353,16.1942459747458,16.3038859647742,16.413459264328,
16.523006351189,16.6351510766217,16.7448367857224,16.858211019321,16.9568853997338,
16.9715240189252,16.9715852529196,17.0721654154571,17.0813133909945,17.1923884417713,
17.3018224587493,17.4111929125193,17.520540656044,17.6328839413352,17.742381519234,
17.8561476582214,17.9543503381828,17.9698492848388,17.9699137972089,18.0695607358278,
18.0792872295431,18.1904066185375,18.2994677125777,18.408459452567,18.5174232958139,
18.630128057235,18.7392332550938,18.853737798296,18.9524694433536,18.9682090697805,
18.9682423414983,19.0701346353313,19.0803569178244,19.1922343498211,19.3039734858659,
19.4156096794738,19.5271781448262,19.6387575696301,19.7503332460084,19.8620209741044,
19.9665708857877),.UNSPECIFIED.) ;
#1308=B_SPLINE_CURVE_WITH_KNOTS('',3,(#54027,#54028,#54029,#54030,#54031,
#54032,#54033,#54034,#54035,#54036,#54037,#54038,#54039,#54040,#54041,#54042,
#54043,#54044,#54045,#54046,#54047,#54048,#54049,#54050,#54051,#54052,#54053,
#54054,#54055,#54056,#54057,#54058,#54059,#54060,#54061,#54062,#54063,#54064,
#54065,#54066,#54067,#54068,#54069,#54070,#54071,#54072,#54073,#54074,#54075,
#54076,#54077,#54078,#54079,#54080,#54081,#54082,#54083,#54084,#54085,#54086,
#54087,#54088,#54089,#54090,#54091,#54092,#54093,#54094,#54095,#54096,#54097,
#54098,#54099,#54100,#54101,#54102,#54103,#54104,#54105,#54106,#54107,#54108,
#54109,#54110,#54111,#54112,#54113,#54114,#54115,#54116,#54117,#54118,#54119,
#54120,#54121,#54122,#54123,#54124,#54125,#54126,#54127,#54128,#54129,#54130),
 .UNSPECIFIED.,.F.,.F.,(4,2,2,2,2,2,2,2,2,2,2,2,2,2,2,2,2,2,2,2,2,2,2,2,
2,2,2,2,2,2,2,2,2,2,2,2,2,2,2,2,2,2,2,2,2,2,2,2,2,2,2,4),(1.10923317368641,
1.11666256443331,1.13796698671944,1.16979398628159,1.18648633306866,1.1955363052136,
1.20845641506686,1.2271779298195,1.26308344394781,1.27862643423749,1.29591470288027,
1.31626339855425,1.35135219608917,1.36087907748399,1.37211876799907,1.40422601455767,
1.43154479013796,1.44684981283533,1.46488734764193,1.48703666194828,1.51867416145164,
1.52807467181166,1.53961320413495,1.55503553052287,1.59723041441357,1.61272025648597,
1.63014776357057,1.65082730757719,1.68477650100827,1.69442112195966,1.70548341908458,
1.73711202265563,1.76510278197234,1.78025690052183,1.79814050897969,1.81991228390051,
1.85264425634999,1.86196800051899,1.87362972720979,1.88934043318008,1.93049967303983,
1.94596068848039,1.9630644315494,1.98305552649924,2.01952385790263,2.02892042589877,
2.04057198294345,2.05620240023131,2.09741648348771,2.11299416773319,2.13056123103445,
2.15945093591691),.UNSPECIFIED.) ;
#1309=B_SPLINE_CURVE_WITH_KNOTS('',3,(#54136,#54137,#54138,#54139,#54140,
#54141,#54142,#54143,#54144,#54145),.UNSPECIFIED.,.F.,.F.,(4,2,2,2,4),(0.000105573133753892,
0.0138955038549731,0.0231490164641212,0.0327225726684864,0.0589305428466179),
 .UNSPECIFIED.) ;
#1310=B_SPLINE_CURVE_WITH_KNOTS('',3,(#54147,#54148,#54149,#54150,#54151,
#54152,#54153,#54154,#54155,#54156,#54157,#54158,#54159,#54160,#54161,#54162,
#54163,#54164,#54165,#54166,#54167,#54168,#54169,#54170,#54171,#54172,#54173,
#54174,#54175,#54176,#54177,#54178,#54179,#54180,#54181,#54182,#54183,#54184,
#54185,#54186,#54187,#54188,#54189,#54190,#54191,#54192,#54193,#54194,#54195,
#54196,#54197,#54198,#54199,#54200,#54201,#54202,#54203,#54204,#54205,#54206,
#54207,#54208,#54209,#54210,#54211,#54212,#54213,#54214,#54215,#54216,#54217,
#54218,#54219,#54220,#54221,#54222,#54223,#54224,#54225,#54226,#54227,#54228,
#54229,#54230,#54231,#54232,#54233,#54234,#54235,#54236,#54237,#54238,#54239,
#54240,#54241,#54242,#54243,#54244,#54245,#54246,#54247,#54248,#54249,#54250,
#54251,#54252,#54253,#54254,#54255,#54256,#54257,#54258,#54259,#54260,#54261,
#54262,#54263,#54264,#54265,#54266,#54267,#54268,#54269,#54270,#54271,#54272,
#54273,#54274,#54275,#54276),.UNSPECIFIED.,.F.,.F.,(4,3,3,3,3,3,3,3,3,3,
3,3,3,3,3,3,3,3,3,3,3,3,3,3,3,3,3,3,3,3,3,3,3,3,3,3,3,3,3,3,3,3,3,4),(-3.84638255852685,
-3.73820615619476,-3.63014673992374,-3.5221618213571,-3.41420864885417,
-3.30616818381397,-3.19808730684748,-3.08980590461576,-2.99504686603603,
-2.99498563286819,-2.8944054715389,-2.88525749870731,-2.77418244744124,
-2.66474843435285,-2.55537798445871,-2.44603024479486,-2.33368695574084,
-2.22418938164505,-2.11042323511192,-2.01222055801228,-1.99672160042913,
-1.99665708857879,-1.89701015027871,-1.88728366291615,-1.7761642730878,
-1.66710318509831,-1.55811145091343,-1.4491476132164,-1.33644284598465,
-1.22733765298158,-1.11283309863549,-1.01410146365423,-0.998361816309247,
-0.998328544289396,-0.89643625326683,-0.886213955367558,-0.774336511044062,
-0.662597362857677,-0.550961157321703,-0.439392680283066,-0.327813244270253,
-0.21623755694208,-0.104549818462726,-8.74178244858098E-13),
 .UNSPECIFIED.) ;
#1311=B_SPLINE_CURVE_WITH_KNOTS('',3,(#54280,#54281,#54282,#54283,#54284,
#54285,#54286,#54287,#54288,#54289,#54290,#54291,#54292,#54293,#54294,#54295,
#54296,#54297,#54298,#54299,#54300,#54301,#54302,#54303,#54304,#54305,#54306,
#54307,#54308,#54309,#54310,#54311,#54312,#54313,#54314,#54315,#54316,#54317,
#54318,#54319,#54320,#54321,#54322,#54323,#54324,#54325,#54326,#54327,#54328,
#54329,#54330,#54331,#54332,#54333,#54334,#54335,#54336,#54337,#54338,#54339,
#54340,#54341,#54342,#54343,#54344,#54345,#54346,#54347,#54348,#54349,#54350,
#54351,#54352,#54353,#54354,#54355,#54356,#54357,#54358,#54359,#54360,#54361,
#54362,#54363,#54364,#54365,#54366,#54367,#54368,#54369,#54370,#54371,#54372,
#54373,#54374,#54375,#54376,#54377,#54378,#54379,#54380,#54381,#54382,#54383,
#54384,#54385,#54386,#54387,#54388,#54389,#54390,#54391,#54392,#54393,#54394,
#54395,#54396,#54397,#54398,#54399,#54400,#54401,#54402,#54403,#54404,#54405,
#54406,#54407,#54408,#54409,#54410,#54411,#54412,#54413,#54414,#54415,#54416,
#54417,#54418,#54419,#54420,#54421,#54422,#54423,#54424,#54425,#54426,#54427,
#54428,#54429,#54430,#54431,#54432,#54433,#54434,#54435,#54436,#54437,#54438,
#54439,#54440,#54441,#54442,#54443,#54444,#54445,#54446,#54447,#54448,#54449,
#54450,#54451,#54452,#54453,#54454,#54455,#54456,#54457,#54458,#54459,#54460,
#54461,#54462,#54463,#54464,#54465,#54466,#54467,#54468,#54469,#54470,#54471,
#54472,#54473,#54474,#54475,#54476,#54477,#54478),.UNSPECIFIED.,.F.,.F.,
(4,3,3,3,3,3,3,3,3,3,3,3,3,3,3,3,3,3,3,3,3,3,3,3,3,3,3,3,3,3,3,3,3,3,3,
3,3,3,3,3,3,3,3,3,3,3,3,3,3,3,3,3,3,3,3,3,3,3,3,3,3,3,3,3,3,3,4),(2.02865585856489,
2.12402762122252,2.23323999155846,2.34234107107911,2.45137236451629,2.56037527914099,
2.66947003572026,2.77860579083783,2.88794878790004,2.9861951620001,2.99492423721753,
2.99498563286815,3.09555643554825,3.10492541786507,3.21597401277663,3.32561358356885,
3.43518668625693,3.54473379827187,3.65687889299329,3.76656517412907,3.8799396756433,
3.97859548600955,3.99325757945939,3.99331417715754,4.09371825155224,4.10302725066695,
4.21410418451445,4.32351125154536,4.43285029772412,4.54216215354018,4.65453229551687,
4.76398290563599,4.87781281354146,4.97628013227034,4.9915883385075,4.99164272144692,
5.09202893482422,5.10141432669419,5.21248394407445,5.32195215739788,5.43135314730772,
5.54072763591608,5.65303854337114,5.76255273957561,5.87626200265596,5.97481642665783,
5.98991760907827,5.98997126573631,6.09040615425878,6.09976697233783,6.21083357704881,
6.32032727182328,6.42975419592545,6.53915503546805,6.65144122910747,6.76098253848876,
6.87464117425723,6.97319126496119,6.98824561473473,6.9882998100257,7.08940671165733,
7.09951538805716,7.21054493226041,7.32140398308574,7.43216340464187,7.54286555752923,
7.59300756235177),.UNSPECIFIED.) ;
#1312=B_SPLINE_CURVE_WITH_KNOTS('',3,(#54479,#54480,#54481,#54482,#54483,
#54484,#54485,#54486),.UNSPECIFIED.,.F.,.F.,(4,2,2,4),(-1.10884496276699,
-1.08689879128658,-1.05535201010488,-1.05003008412879),.UNSPECIFIED.) ;
#1313=B_SPLINE_CURVE_WITH_KNOTS('',3,(#54493,#54494,#54495,#54496,#54497,
#54498,#54499,#54500,#54501,#54502,#54503,#54504,#54505,#54506,#54507,#54508,
#54509,#54510,#54511,#54512,#54513,#54514,#54515,#54516,#54517,#54518,#54519,
#54520,#54521,#54522,#54523,#54524,#54525,#54526,#54527,#54528,#54529,#54530,
#54531,#54532,#54533,#54534,#54535),.UNSPECIFIED.,.F.,.F.,(4,3,3,3,3,3,
3,3,3,3,3,3,3,3,4),(-17.9380018385438,-17.8425458057697,-17.7333362973642,
-17.6242380988214,-17.5152097045172,-17.4062097063169,-17.2971178825619,
-17.1879850740603,-17.0786450208909,-16.9803981893995,-16.9716460291613,
-16.9715852529196,-16.8695608211846,-16.8587047742622,-16.7648876345291),
 .UNSPECIFIED.) ;
#1314=B_SPLINE_CURVE_WITH_KNOTS('',3,(#54541,#54542,#54543,#54544,#54545,
#54546,#54547,#54548,#54549,#54550,#54551,#54552,#54553,#54554,#54555,#54556,
#54557,#54558,#54559,#54560,#54561,#54562,#54563,#54564,#54565,#54566,#54567,
#54568,#54569,#54570,#54571,#54572,#54573,#54574,#54575,#54576,#54577,#54578,
#54579,#54580,#54581,#54582,#54583,#54584,#54585,#54586,#54587,#54588,#54589,
#54590,#54591,#54592,#54593,#54594,#54595,#54596,#54597,#54598,#54599,#54600,
#54601,#54602,#54603,#54604,#54605,#54606,#54607,#54608,#54609,#54610,#54611,
#54612,#54613,#54614,#54615,#54616,#54617,#54618,#54619,#54620,#54621,#54622,
#54623,#54624,#54625,#54626,#54627,#54628,#54629,#54630,#54631,#54632,#54633,
#54634,#54635,#54636,#54637,#54638,#54639,#54640,#54641,#54642,#54643,#54644,
#54645,#54646,#54647,#54648,#54649,#54650,#54651,#54652,#54653,#54654,#54655,
#54656,#54657,#54658,#54659,#54660,#54661,#54662,#54663,#54664,#54665,#54666,
#54667,#54668,#54669,#54670,#54671,#54672,#54673,#54674,#54675,#54676,#54677,
#54678,#54679,#54680,#54681,#54682,#54683,#54684,#54685,#54686,#54687,#54688,
#54689,#54690,#54691,#54692,#54693,#54694,#54695,#54696,#54697,#54698,#54699,
#54700,#54701,#54702,#54703,#54704,#54705,#54706,#54707,#54708,#54709,#54710,
#54711,#54712,#54713,#54714,#54715,#54716,#54717,#54718,#54719,#54720,#54721,
#54722,#54723,#54724,#54725,#54726,#54727,#54728,#54729,#54730,#54731,#54732,
#54733,#54734,#54735,#54736,#54737,#54738,#54739),.UNSPECIFIED.,.F.,.F.,
(4,3,3,3,3,3,3,3,3,3,3,3,3,3,3,3,3,3,3,3,3,3,3,3,3,3,3,3,3,3,3,3,3,3,3,
3,3,3,3,3,3,3,3,3,3,3,3,3,3,3,3,3,3,3,3,3,3,3,3,3,3,3,3,3,3,3,4),(14.2294869669467,
14.3389322308676,14.4483223291313,14.5576979646225,14.6671790216403,14.7767121569683,
14.8864519699031,14.9748738708372,14.9749281643408,15.0752588397667,15.0846363989758,
15.1957139376826,15.3051193758575,15.4144579925258,15.5237706155259,15.636142138802,
15.7455964652154,15.8594265869228,15.9579660798332,15.9732006708539,15.9732567086302,
16.0738047882785,16.0831967562974,16.1942453183752,16.3038843458098,16.4134566034534,
16.5230025687912,16.6351482398233,16.744832633098,16.8582089430088,16.9568845136797,
16.9715246332023,16.9715852529196,17.0721645754056,17.081310467377,17.192385883606,
17.3018169902679,17.4111845419844,17.5205293926883,17.6328754938185,17.742370217053,
17.856142007131,17.9543426244737,17.9698496806575,17.969913797209,18.0695603136759,
18.0792819826719,18.1904020275252,18.299458347709,18.4084455018845,18.5174049537962,
18.6301143007217,18.7392156390599,18.8537289902791,18.9524526707438,18.968208839462,
18.9682423414984,19.0701323904312,19.0803666377335,19.192253585914,19.3040020972769,
19.4156475035808,19.5272249970061,19.6388130843005,19.7503972247079,19.8620929819371,
19.9665708857877),.UNSPECIFIED.) ;
#1315=B_SPLINE_CURVE_WITH_KNOTS('',3,(#54741,#54742,#54743,#54744,#54745,
#54746,#54747,#54748,#54749,#54750,#54751,#54752,#54753,#54754,#54755,#54756,
#54757,#54758,#54759,#54760,#54761,#54762,#54763,#54764,#54765,#54766,#54767,
#54768,#54769,#54770,#54771,#54772,#54773,#54774,#54775,#54776,#54777,#54778,
#54779,#54780,#54781,#54782,#54783,#54784,#54785,#54786,#54787,#54788,#54789,
#54790,#54791,#54792,#54793,#54794,#54795,#54796,#54797,#54798,#54799,#54800,
#54801,#54802,#54803,#54804,#54805,#54806,#54807,#54808,#54809,#54810,#54811,
#54812,#54813,#54814,#54815,#54816,#54817,#54818,#54819,#54820,#54821,#54822,
#54823,#54824,#54825,#54826,#54827,#54828,#54829,#54830,#54831,#54832,#54833,
#54834,#54835,#54836,#54837,#54838,#54839,#54840,#54841,#54842,#54843,#54844),
 .UNSPECIFIED.,.F.,.F.,(4,2,2,2,2,2,2,2,2,2,2,2,2,2,2,2,2,2,2,2,2,2,2,2,
2,2,2,2,2,2,2,2,2,2,2,2,2,2,2,2,2,2,2,2,2,2,2,2,2,2,2,4),(1.10920453594835,
1.1166320815093,1.13793450121648,1.16974966156749,1.18645799264353,1.19551033122356,
1.20841878766804,1.22710875477439,1.26309690717015,1.27863717849374,1.29593413862243,
1.31630153851001,1.35134179362724,1.36087497196007,1.3721034776389,1.40414323734612,
1.43154792730153,1.4467050506917,1.46463919801635,1.48653286711609,1.51886748686928,
1.52822543273842,1.53987769753952,1.5555523588918,1.59701777933286,1.61255121200086,
1.62986742642601,1.65028403353202,1.68511285067916,1.69466952558485,1.70590048122777,
1.73794741238401,1.76525899060161,1.78040499829536,1.79833960200703,1.82023252238522,
1.85263795723406,1.86198361343096,1.87358284299029,1.88915308158601,1.93075092780285,
1.94618976202995,1.96335684506068,1.98349276395793,2.01944550510397,2.0288905106591,
2.04041875376629,2.05577463402855,2.09782802978038,2.11336056920194,2.13105185822123,
2.15957942398687),.UNSPECIFIED.) ;
#1316=B_SPLINE_CURVE_WITH_KNOTS('',3,(#54850,#54851,#54852,#54853,#54854,
#54855,#54856,#54857,#54858,#54859),.UNSPECIFIED.,.F.,.F.,(4,2,2,2,4),(0.00010533907809324,
0.013377535183783,0.022284006867853,0.0315331293986908,0.0589297775460328),
 .UNSPECIFIED.) ;
#1317=B_SPLINE_CURVE_WITH_KNOTS('',3,(#54861,#54862,#54863,#54864,#54865,
#54866,#54867,#54868,#54869,#54870,#54871,#54872,#54873,#54874,#54875,#54876,
#54877,#54878,#54879,#54880,#54881,#54882,#54883,#54884,#54885,#54886,#54887,
#54888,#54889,#54890,#54891,#54892,#54893,#54894,#54895,#54896,#54897,#54898,
#54899,#54900,#54901,#54902,#54903,#54904,#54905,#54906,#54907,#54908,#54909,
#54910,#54911,#54912,#54913,#54914,#54915,#54916,#54917,#54918,#54919,#54920,
#54921,#54922,#54923,#54924,#54925,#54926,#54927,#54928,#54929,#54930,#54931,
#54932,#54933,#54934,#54935,#54936,#54937,#54938,#54939,#54940,#54941,#54942,
#54943,#54944,#54945,#54946,#54947,#54948,#54949,#54950,#54951,#54952,#54953,
#54954,#54955,#54956,#54957,#54958,#54959,#54960,#54961,#54962,#54963,#54964,
#54965,#54966,#54967,#54968,#54969,#54970,#54971,#54972,#54973,#54974,#54975,
#54976,#54977,#54978,#54979,#54980,#54981,#54982,#54983,#54984,#54985,#54986,
#54987,#54988,#54989,#54990),.UNSPECIFIED.,.F.,.F.,(4,3,3,3,3,3,3,3,3,3,
3,3,3,3,3,3,3,3,3,3,3,3,3,3,3,3,3,3,3,3,3,3,3,3,3,3,3,3,3,3,3,3,3,4),(-3.84638256364261,
-3.73820745978248,-3.63014941624604,-3.52216594268968,-3.41421428740373,
-3.30617544820113,-3.19809625937625,-3.08981663623424,-2.99504625172493,
-2.99498563286813,-2.89440631145632,-2.88526042240579,-2.77418500567741,
-2.66475390299952,-2.55538635525859,-2.44604150852038,-2.33369540353497,
-2.22420068422119,-2.11042888639997,-2.0122282719807,-1.99672120457837,
-1.99665708857875,-1.89701057277755,-1.88728891067,-1.77616886487242,-1.66711255158284,
-1.55812540403875,-1.44916595848633,-1.33645660493709,-1.22735527221197,
-1.11284190825067,-1.01411823893781,-0.998362046647454,-0.99832854428937,
-0.896438498507768,-0.886204234316478,-0.77431727268097,-0.662568748059076,
-0.550923328723212,-0.43934582252413,-0.327757722968657,-0.216173570578685,
-0.104477801978497,-5.02812373608076E-13),.UNSPECIFIED.) ;
#1318=B_SPLINE_CURVE_WITH_KNOTS('',3,(#54994,#54995,#54996,#54997,#54998,
#54999,#55000,#55001,#55002,#55003,#55004,#55005,#55006,#55007,#55008,#55009,
#55010,#55011,#55012,#55013,#55014,#55015,#55016,#55017,#55018,#55019,#55020,
#55021,#55022,#55023,#55024,#55025,#55026,#55027,#55028,#55029,#55030,#55031,
#55032,#55033,#55034,#55035,#55036,#55037,#55038,#55039,#55040,#55041,#55042,
#55043,#55044,#55045,#55046,#55047,#55048,#55049,#55050,#55051,#55052,#55053,
#55054,#55055,#55056,#55057,#55058,#55059,#55060,#55061,#55062,#55063,#55064,
#55065,#55066,#55067,#55068,#55069,#55070,#55071,#55072,#55073,#55074,#55075,
#55076,#55077,#55078,#55079,#55080,#55081,#55082,#55083,#55084,#55085,#55086,
#55087,#55088,#55089,#55090,#55091,#55092,#55093,#55094,#55095,#55096,#55097,
#55098,#55099,#55100,#55101,#55102,#55103,#55104,#55105,#55106,#55107,#55108,
#55109,#55110,#55111,#55112,#55113,#55114,#55115,#55116,#55117,#55118,#55119,
#55120,#55121,#55122,#55123,#55124,#55125,#55126,#55127,#55128,#55129,#55130,
#55131,#55132,#55133,#55134,#55135,#55136,#55137,#55138,#55139,#55140,#55141,
#55142,#55143,#55144,#55145,#55146,#55147,#55148,#55149,#55150,#55151,#55152,
#55153,#55154,#55155,#55156,#55157,#55158,#55159,#55160,#55161,#55162,#55163,
#55164,#55165,#55166,#55167,#55168,#55169,#55170,#55171,#55172,#55173,#55174,
#55175,#55176,#55177,#55178,#55179,#55180,#55181,#55182,#55183,#55184,#55185,
#55186,#55187,#55188,#55189,#55190,#55191,#55192),.UNSPECIFIED.,.F.,.F.,
(4,3,3,3,3,3,3,3,3,3,3,3,3,3,3,3,3,3,3,3,3,3,3,3,3,3,3,3,3,3,3,3,3,3,3,
3,3,3,3,3,3,3,3,3,3,3,3,3,3,3,3,3,3,3,3,3,3,3,3,3,3,3,3,3,3,3,4),(2.02856916811818,
2.12402508352432,2.23323459585707,2.3423327983503,2.45136119662696,2.56036119882055,
2.66945302658712,2.77858583911685,2.88792589630695,2.98617272709135,2.99492485577242,
2.99498563286816,3.09555717591128,3.10492395017402,3.21597272854696,3.32561103972279,
3.43518296101929,3.54472896932239,3.65687527128118,3.76656064185824,3.87993740950789,
3.97859131455151,3.99325792967966,3.99331417715755,4.09371875826342,4.10302769217917,
4.21410457083764,4.32351219675406,4.43285184432446,4.54216434323133,4.65453393778523,
4.76398528807051,4.87781400475873,4.97628109455529,4.99158842889737,4.99164272144694,
5.09202944416287,5.1014154817733,5.21248495476868,5.32195432557387,5.43135647200078,
5.54073211535619,5.65304190295122,5.76255724150614,5.87626425362123,5.97481946627002,
5.98991764446527,5.98997126573632,6.09040625393766,6.09976728300663,6.21083384888401,
6.32032780763715,6.4297549783069,6.53915604721805,6.65144198791996,6.76098348433243,
6.87464164717906,6.9731920566554,6.98824570503598,6.9882998100257,7.08940654529792,
7.09951520459782,7.21054455240904,7.32140338904543,7.4321625863856,7.54286450158988,
7.59300756235177),.UNSPECIFIED.) ;
#1319=B_SPLINE_CURVE_WITH_KNOTS('',3,(#55193,#55194,#55195,#55196,#55197,
#55198,#55199,#55200),.UNSPECIFIED.,.F.,.F.,(4,2,2,4),(-1.10884009192702,
-1.08690736009366,-1.05535892792443,-1.05002476366986),.UNSPECIFIED.) ;
#1320=B_SPLINE_CURVE_WITH_KNOTS('',3,(#55206,#55207,#55208,#55209,#55210,
#55211,#55212,#55213,#55214,#55215,#55216,#55217,#55218,#55219,#55220,#55221,
#55222,#55223,#55224,#55225,#55226,#55227,#55228,#55229,#55230,#55231,#55232,
#55233),.UNSPECIFIED.,.F.,.F.,(4,2,2,2,2,2,2,2,2,2,2,2,2,4),(0.459098935875569,
0.464417734433904,0.505520800153837,0.520882111108831,0.52986479302885,
0.5423026928859,0.575113037158553,0.614875876244612,0.632729769250043,0.649501533827279,
0.687496632532719,0.719965224203154,0.726875831338429,0.732438471583609),
 .UNSPECIFIED.) ;
#1321=B_SPLINE_CURVE_WITH_KNOTS('',3,(#55236,#55237,#55238,#55239,#55240,
#55241,#55242,#55243,#55244,#55245,#55246,#55247,#55248,#55249,#55250,#55251,
#55252,#55253,#55254,#55255,#55256,#55257,#55258,#55259,#55260,#55261,#55262,
#55263,#55264,#55265,#55266,#55267,#55268,#55269,#55270,#55271),
 .UNSPECIFIED.,.F.,.F.,(4,2,2,2,2,2,2,2,2,2,2,2,2,2,2,2,2,4),(0.0003284355859769,
0.00531767720044407,0.0119536835984835,0.0490121209748348,0.0844681757214455,
0.100405765516477,0.11631259325507,0.149557305146467,0.178278962167049,
0.190732222627568,0.201079007639284,0.210406505179939,0.232092261470985,
0.282159926353324,0.300140818751553,0.315111986607238,0.33700779754842,
0.381142777041596),.UNSPECIFIED.) ;
#1322=B_SPLINE_CURVE_WITH_KNOTS('',3,(#55277,#55278,#55279,#55280,#55281,
#55282,#55283,#55284,#55285,#55286,#55287,#55288,#55289,#55290,#55291,#55292,
#55293,#55294,#55295,#55296,#55297,#55298,#55299,#55300,#55301,#55302,#55303,
#55304,#55305,#55306,#55307,#55308,#55309,#55310,#55311,#55312,#55313,#55314,
#55315,#55316,#55317,#55318,#55319,#55320,#55321,#55322,#55323,#55324,#55325,
#55326,#55327,#55328,#55329,#55330,#55331,#55332,#55333,#55334,#55335,#55336,
#55337,#55338,#55339,#55340,#55341,#55342,#55343,#55344,#55345,#55346,#55347,
#55348,#55349,#55350),.UNSPECIFIED.,.F.,.F.,(4,2,2,2,2,2,2,2,2,2,2,2,2,
2,2,2,2,2,2,2,2,2,2,2,2,2,2,2,2,2,2,2,2,2,2,2,4),(1.29359998411323,1.30095406668721,
1.31741432341847,1.33295482268895,1.36148535680912,1.40267840562338,1.4168827682256,
1.42564857009657,1.43856307377589,1.45605514494036,1.50897620000202,1.52485836063247,
1.54087322196961,1.57757886415223,1.61688912127807,1.62695610494123,1.63658903940002,
1.66191828021951,1.71494369390444,1.73069937007811,1.74683327998757,1.78395462238556,
1.82219256849362,1.832340258941,1.84185095546442,1.86546888373326,1.92105272943006,
1.93665099692755,1.95279196240484,1.97294420449489,2.01346271879964,2.03165906133175,
2.04072270747648,2.05190736557107,2.06584925450052,2.11923314491368,2.12891857368306),
 .UNSPECIFIED.) ;
#1323=B_SPLINE_CURVE_WITH_KNOTS('',3,(#55351,#55352,#55353,#55354,#55355,
#55356,#55357,#55358,#55359,#55360,#55361,#55362,#55363,#55364,#55365,#55366,
#55367,#55368,#55369,#55370,#55371,#55372,#55373,#55374,#55375,#55376,#55377,
#55378,#55379,#55380,#55381,#55382,#55383,#55384,#55385,#55386,#55387,#55388,
#55389,#55390,#55391,#55392),.UNSPECIFIED.,.F.,.F.,(4,2,2,2,2,2,2,2,2,2,
2,2,2,2,2,2,2,2,2,2,4),(0.000738082385943926,0.0138519484644011,0.0295692425710776,
0.0794798266889706,0.106573518509978,0.116314733841013,0.126412928211499,
0.165039800973681,0.201315998205497,0.217463598449292,0.233563252041158,
0.267515628887756,0.296218550217051,0.313295008909005,0.322142293471645,
0.332500284255174,0.366422341235642,0.408081104489123,0.424788295102322,
0.439776151822035,0.459098935875569),.UNSPECIFIED.) ;
#1324=B_SPLINE_CURVE_WITH_KNOTS('',3,(#55393,#55394,#55395,#55396,#55397,
#55398,#55399,#55400,#55401,#55402,#55403,#55404,#55405,#55406,#55407,#55408,
#55409,#55410,#55411,#55412,#55413,#55414,#55415,#55416,#55417,#55418,#55419,
#55420,#55421,#55422,#55423,#55424,#55425,#55426,#55427,#55428,#55429,#55430,
#55431,#55432,#55433,#55434,#55435,#55436,#55437,#55438,#55439,#55440,#55441,
#55442,#55443,#55444,#55445,#55446,#55447,#55448,#55449,#55450,#55451,#55452,
#55453,#55454,#55455,#55456,#55457,#55458,#55459,#55460,#55461,#55462,#55463,
#55464,#55465,#55466,#55467,#55468,#55469,#55470,#55471,#55472,#55473,#55474,
#55475,#55476,#55477,#55478,#55479,#55480,#55481,#55482,#55483,#55484,#55485,
#55486,#55487,#55488,#55489,#55490,#55491,#55492,#55493,#55494,#55495,#55496,
#55497,#55498,#55499,#55500,#55501,#55502,#55503,#55504,#55505,#55506),
 .UNSPECIFIED.,.F.,.F.,(4,2,2,2,2,2,2,2,2,2,2,2,2,2,2,2,2,2,2,2,2,2,2,2,
2,2,2,2,2,2,2,2,2,2,2,2,2,2,2,2,2,2,2,2,2,2,2,2,2,2,2,2,2,2,2,2,4),(9.9999999911049E-7,
0.0181412579621644,0.0260517011858928,0.03569506804886,0.0856389271588889,
0.114970951918313,0.130443396223946,0.146521745286428,0.197472647378066,
0.222831685352658,0.23242000657169,0.242317758348657,0.28307583406927,0.318816335082925,
0.334727678149403,0.350487394344637,0.404321518915359,0.421345075068166,
0.434025097613039,0.442753508335243,0.457052499386952,0.501754765373651,
0.527684940848551,0.542966732260761,0.559688778480777,0.595876018588788,
0.629041013088632,0.64065417101676,0.649497725865986,0.665641909499553,
0.708103849070844,0.728232473019738,0.744532529259699,0.760012287632047,
0.788626677992194,0.82285658068839,0.841440446077428,0.850502880244777,
0.861330836969597,0.911157653131982,0.938261616252987,0.953631128251108,
0.970141586102395,1.01737241808675,1.03635678173686,1.04992207666676,1.05862155682344,
1.07186549350823,1.11259380862868,1.142628458096,1.15820158179272,1.17436083719213,
1.22518214710482,1.25065900116484,1.2602658284382,1.2701883131198,1.29377606271217),
 .UNSPECIFIED.) ;
#1325=B_SPLINE_CURVE_WITH_KNOTS('',3,(#55512,#55513,#55514,#55515,#55516,
#55517,#55518,#55519,#55520,#55521,#55522,#55523,#55524,#55525,#55526,#55527,
#55528,#55529,#55530,#55531,#55532,#55533,#55534,#55535,#55536,#55537,#55538,
#55539,#55540,#55541,#55542,#55543,#55544,#55545,#55546,#55547,#55548,#55549,
#55550,#55551,#55552,#55553,#55554,#55555,#55556,#55557,#55558,#55559,#55560,
#55561,#55562,#55563,#55564,#55565,#55566,#55567,#55568,#55569,#55570,#55571,
#55572,#55573,#55574,#55575,#55576,#55577,#55578,#55579,#55580,#55581,#55582,
#55583,#55584,#55585,#55586,#55587,#55588,#55589,#55590,#55591,#55592,#55593,
#55594,#55595,#55596,#55597,#55598,#55599,#55600,#55601,#55602),
 .UNSPECIFIED.,.F.,.F.,(4,3,3,3,3,3,3,3,3,3,3,3,3,3,3,3,3,3,3,3,3,3,3,3,
3,3,3,3,3,3,4),(15.7079632679487,15.8113041863724,15.9146184877327,16.0179415683624,
16.1213837812541,16.2248899519759,16.3224073436296,16.3285912852237,16.3947470380404,
16.394798101354,16.4893631462319,16.4989495063346,16.6029410394302,16.7068040901932,
16.8105977431501,16.9143569262867,17.0181165201345,17.1219800282497,17.2258994684857,
17.3243086209598,17.3299977052375,17.3930777392184,17.3931266456435,17.488160245186,
17.4974425219354,17.6010533657214,17.6065554326192,17.7105958268345,17.8145672327603,
17.9185103805803,17.9338941646706),.UNSPECIFIED.) ;
#1326=B_SPLINE_CURVE_WITH_KNOTS('',3,(#55604,#55605,#55606,#55607,#55608,
#55609,#55610,#55611,#55612,#55613,#55614,#55615,#55616,#55617,#55618,#55619,
#55620,#55621,#55622,#55623,#55624,#55625,#55626,#55627,#55628,#55629,#55630,
#55631,#55632,#55633,#55634,#55635,#55636,#55637,#55638,#55639,#55640,#55641,
#55642,#55643),.UNSPECIFIED.,.F.,.F.,(4,3,3,3,3,3,3,3,3,3,3,3,3,4),(14.3981410127754,
14.5041449103233,14.6100638854506,14.7159513361487,14.8218268476716,14.9277203457283,
15.033661766908,15.1397601395315,15.245946872782,15.3523359246553,15.3964695570646,
15.5190118197687,15.6402404822583,15.7079554008178),.UNSPECIFIED.) ;
#1327=B_SPLINE_CURVE_WITH_KNOTS('',3,(#55646,#55647,#55648,#55649,#55650,
#55651,#55652,#55653,#55654,#55655,#55656,#55657,#55658,#55659,#55660,#55661,
#55662,#55663,#55664,#55665,#55666,#55667,#55668,#55669,#55670,#55671,#55672,
#55673,#55674,#55675,#55676,#55677,#55678,#55679,#55680,#55681,#55682,#55683,
#55684,#55685,#55686,#55687,#55688,#55689,#55690,#55691,#55692,#55693,#55694,
#55695,#55696,#55697,#55698,#55699,#55700,#55701,#55702,#55703,#55704,#55705,
#55706,#55707,#55708,#55709,#55710,#55711,#55712,#55713,#55714,#55715,#55716,
#55717,#55718,#55719),.UNSPECIFIED.,.F.,.F.,(4,2,2,2,2,2,2,2,2,2,2,2,2,
2,2,2,2,2,2,2,2,2,2,2,2,2,2,2,2,2,2,2,2,2,2,2,4),(8.98756407565875E-5,0.00958673476959858,
0.0632031336255092,0.0833445098038401,0.0995431819327776,0.115206036663946,
0.168389320176256,0.192964400571718,0.202521587597258,0.212531919880494,
0.252085336041996,0.277375924344348,0.29734241960763,0.31221965819781,0.33141213917936,
0.375535701000085,0.398575768451147,0.408036346243251,0.418062919419705,
0.451131415410438,0.491791764285841,0.508201330943047,0.523322593889842,
0.549083529179824,0.593368985045316,0.607943154443325,0.616608600447831,
0.628783684406638,0.661898827321747,0.699758037739072,0.715623109939765,
0.731218812619801,0.763029012118359,0.808061561073486,0.818144105240131,
0.826091049587224,0.835764201608868),.UNSPECIFIED.) ;
#1328=B_SPLINE_CURVE_WITH_KNOTS('',3,(#55725,#55726,#55727,#55728,#55729,
#55730,#55731,#55732,#55733,#55734,#55735,#55736,#55737,#55738,#55739,#55740,
#55741,#55742,#55743,#55744,#55745,#55746,#55747,#55748,#55749,#55750,#55751,
#55752),.UNSPECIFIED.,.F.,.F.,(4,2,2,2,2,2,2,2,2,2,2,2,2,4),(0.45910898550012,
0.464123317728498,0.504834291857946,0.520817723021585,0.529788408837737,
0.542027898291406,0.574819933375454,0.615161849610536,0.633018213721076,
0.649838699815419,0.687975160352418,0.719992757768681,0.726888844299736,
0.732445412692217),.UNSPECIFIED.) ;
#1329=B_SPLINE_CURVE_WITH_KNOTS('',3,(#55755,#55756,#55757,#55758,#55759,
#55760,#55761,#55762,#55763,#55764,#55765,#55766,#55767,#55768,#55769,#55770,
#55771,#55772,#55773,#55774,#55775,#55776,#55777,#55778,#55779,#55780,#55781,
#55782,#55783,#55784,#55785,#55786,#55787,#55788,#55789,#55790),
 .UNSPECIFIED.,.F.,.F.,(4,2,2,2,2,2,2,2,2,2,2,2,2,2,2,2,2,4),(0.000321553292874637,
0.00529579930759916,0.0119020171496447,0.0494611338648065,0.0845644657484785,
0.100475323375435,0.116356578470903,0.149389590129435,0.178249519548127,
0.190726728454751,0.201086130709088,0.210416304464164,0.232095757180373,
0.282140266304572,0.300085602459823,0.315048158012112,0.336954443421903,
0.381146228182771),.UNSPECIFIED.) ;
#1330=B_SPLINE_CURVE_WITH_KNOTS('',3,(#55796,#55797,#55798,#55799,#55800,
#55801,#55802,#55803,#55804,#55805,#55806,#55807,#55808,#55809,#55810,#55811,
#55812,#55813,#55814,#55815,#55816,#55817,#55818,#55819,#55820,#55821,#55822,
#55823,#55824,#55825,#55826,#55827,#55828,#55829,#55830,#55831,#55832,#55833,
#55834,#55835,#55836,#55837,#55838,#55839,#55840,#55841,#55842,#55843,#55844,
#55845,#55846,#55847,#55848,#55849,#55850,#55851,#55852,#55853,#55854,#55855,
#55856,#55857,#55858,#55859,#55860,#55861,#55862,#55863,#55864,#55865,#55866,
#55867,#55868,#55869,#55870,#55871,#55872,#55873),.UNSPECIFIED.,.F.,.F.,
(4,2,2,2,2,2,2,2,2,2,2,2,2,2,2,2,2,2,2,2,2,2,2,2,2,2,2,2,2,2,2,2,2,2,2,
2,2,2,4),(0.458614805141202,0.468276334293724,0.484172078983711,0.500138368708875,
0.548722523717207,0.568332719679477,0.582181641216813,0.590935448093863,
0.604134706231622,0.647012452574512,0.675653447701051,0.691206326288677,
0.707661678880968,0.727803084519804,0.771146082241682,0.786438447891096,
0.795296281120897,0.807292273622826,0.840558191000508,0.878772863383274,
0.894768757920461,0.910644605195344,0.94542027431542,0.985939907421154,
0.99655236593802,1.00576978002281,1.02579542812151,1.06650639499888,1.08968052587657,
1.10474702453885,1.12218254242584,1.14210899514003,1.18334736526887,1.19827456080035,
1.20708809368799,1.21960615721636,1.25306240072434,1.2797654071498,1.29379501408075),
 .UNSPECIFIED.) ;
#1331=B_SPLINE_CURVE_WITH_KNOTS('',3,(#55874,#55875,#55876,#55877,#55878,
#55879,#55880,#55881,#55882,#55883,#55884,#55885,#55886,#55887,#55888,#55889,
#55890,#55891,#55892,#55893,#55894,#55895,#55896,#55897,#55898,#55899,#55900,
#55901,#55902,#55903,#55904,#55905,#55906,#55907,#55908,#55909,#55910,#55911,
#55912,#55913,#55914,#55915),.UNSPECIFIED.,.F.,.F.,(4,2,2,2,2,2,2,2,2,2,
2,2,2,2,2,2,2,2,2,2,4),(0.00074538786090497,0.0138027418242267,0.0294144634151981,
0.078270908564491,0.106441999089265,0.11623114716668,0.126288013383736,
0.165379768164886,0.201338030985534,0.217448030072118,0.233531439200502,
0.26733290588678,0.296230510522788,0.313365850679765,0.322212279066863,
0.332565896103022,0.36644770944264,0.407902212188932,0.424580316139229,
0.439550483908069,0.45910898550012),.UNSPECIFIED.) ;
#1332=B_SPLINE_CURVE_WITH_KNOTS('',3,(#55916,#55917,#55918,#55919,#55920,
#55921,#55922,#55923,#55924,#55925,#55926,#55927,#55928,#55929,#55930,#55931,
#55932,#55933,#55934,#55935,#55936,#55937,#55938,#55939,#55940,#55941,#55942,
#55943,#55944,#55945,#55946,#55947,#55948,#55949,#55950,#55951,#55952,#55953,
#55954,#55955,#55956,#55957,#55958,#55959,#55960,#55961,#55962,#55963,#55964,
#55965,#55966,#55967,#55968,#55969,#55970,#55971,#55972,#55973,#55974,#55975,
#55976,#55977,#55978,#55979,#55980,#55981,#55982,#55983,#55984,#55985,#55986,
#55987,#55988,#55989,#55990,#55991,#55992,#55993,#55994,#55995,#55996,#55997,
#55998,#55999,#56000,#56001,#56002,#56003,#56004,#56005,#56006,#56007,#56008,
#56009,#56010,#56011,#56012,#56013,#56014,#56015,#56016,#56017,#56018,#56019,
#56020,#56021,#56022,#56023,#56024,#56025,#56026,#56027,#56028,#56029,#56030,
#56031),.UNSPECIFIED.,.F.,.F.,(4,2,2,2,2,2,2,2,2,2,2,2,2,2,2,2,2,2,2,2,
2,2,2,2,2,2,2,2,2,2,2,2,2,2,2,2,2,2,2,2,2,2,2,2,2,2,2,2,2,2,2,2,2,2,2,2,
2,4),(1.00000001892163E-6,0.0125988430125637,0.0214541379866562,0.030189816183294,
0.0430833350666729,0.0868476702733789,0.115249975074114,0.130656050971666,
0.146839979433289,0.196767185511196,0.21481261268838,0.227955380941075,
0.236633839533386,0.250201735758349,0.29112270602314,0.32059920547237,0.336134579367343,
0.352340352688741,0.404741003149359,0.42865449581047,0.43816468646413,0.448226683737091,
0.48711735581692,0.521799384735325,0.538317185364559,0.553685912926676,
0.58074739823862,0.616635941990185,0.630291683837093,0.641287517650734,
0.65029001640104,0.668227485523075,0.708737595010008,0.728900958505633,
0.745001307548107,0.760605312967583,0.815946752036598,0.839765022519998,
0.849264640463107,0.859307773470979,0.898409307993087,0.935515748610904,
0.951393430137624,0.967197254334127,1.01705271376006,1.03617851658254,1.04980500103518,
1.05850438042598,1.07168754742342,1.11238036824938,1.14252866008741,1.158107881077,
1.17425428651828,1.22521120025375,1.25061763376755,1.26022001215864,1.27014486204402,
1.29372393529934),.UNSPECIFIED.) ;
#1333=B_SPLINE_CURVE_WITH_KNOTS('',3,(#56037,#56038,#56039,#56040,#56041,
#56042,#56043,#56044,#56045,#56046,#56047,#56048,#56049,#56050,#56051,#56052,
#56053,#56054,#56055,#56056,#56057,#56058,#56059,#56060,#56061,#56062,#56063,
#56064,#56065,#56066,#56067,#56068,#56069,#56070,#56071,#56072,#56073,#56074,
#56075,#56076,#56077,#56078,#56079,#56080,#56081,#56082,#56083,#56084,#56085,
#56086,#56087,#56088,#56089,#56090,#56091,#56092,#56093,#56094,#56095,#56096,
#56097,#56098,#56099,#56100,#56101,#56102,#56103,#56104,#56105,#56106,#56107,
#56108,#56109,#56110,#56111,#56112,#56113,#56114,#56115,#56116,#56117,#56118,
#56119,#56120,#56121,#56122,#56123,#56124,#56125,#56126,#56127),
 .UNSPECIFIED.,.F.,.F.,(4,3,3,3,3,3,3,3,3,3,3,3,3,3,3,3,3,3,3,3,3,3,3,3,
3,3,3,3,3,3,4),(15.7079632679487,15.811277521818,15.9145643079774,16.0178590600282,
16.1212718704572,16.2247479979436,16.3222741136381,16.3284185432556,16.3947481283565,
16.394798101356,16.4893555683339,16.4989409022619,16.6029238165732,16.7067782344606,
16.8105632454197,16.9143137789071,17.0180647169156,17.1219195878195,17.2258303871081,
17.3242448251247,17.3299200437246,17.3930794452619,17.3931266456454,17.4881639775743,
17.4974391842717,17.6010561100227,17.6065518441373,17.7105895362785,17.8145584563115,
17.9184994130691,17.9338898237342),.UNSPECIFIED.) ;
#1334=B_SPLINE_CURVE_WITH_KNOTS('',3,(#56129,#56130,#56131,#56132,#56133,
#56134,#56135,#56136,#56137,#56138,#56139,#56140,#56141,#56142,#56143,#56144,
#56145,#56146,#56147,#56148,#56149,#56150,#56151,#56152,#56153,#56154,#56155,
#56156,#56157,#56158,#56159,#56160,#56161,#56162,#56163,#56164,#56165,#56166,
#56167,#56168),.UNSPECIFIED.,.F.,.F.,(4,3,3,3,3,3,3,3,3,3,3,3,3,4),(14.3981410127773,
14.5041748950571,14.610124992509,14.7160450299549,14.8219539908772,14.9278817223058,
15.0338580831529,15.1399921691173,15.2462150867062,15.3526406391366,15.3964695570665,
15.5190266859576,15.6402596565994,15.7079553591874),.UNSPECIFIED.) ;
#1335=B_SPLINE_CURVE_WITH_KNOTS('',3,(#56172,#56173,#56174,#56175,#56176,
#56177,#56178,#56179,#56180,#56181,#56182,#56183,#56184,#56185,#56186,#56187,
#56188,#56189,#56190,#56191,#56192,#56193,#56194,#56195,#56196,#56197,#56198,
#56199,#56200,#56201,#56202,#56203,#56204,#56205,#56206,#56207,#56208,#56209),
 .UNSPECIFIED.,.F.,.F.,(4,2,2,2,2,2,2,2,2,2,2,2,2,2,2,2,2,2,4),(0.000123090557559488,
0.00529923882504241,0.0119107487871958,0.0413163072992257,0.0805438068736347,
0.097519789031416,0.112580594592888,0.137496734407516,0.175111623725341,
0.188973027739506,0.200075494695848,0.20906163629957,0.226886150571072,
0.258165447247631,0.289415603200177,0.305220905766297,0.321065189093378,
0.357976300969813,0.377585064672507),.UNSPECIFIED.) ;
#1336=B_SPLINE_CURVE_WITH_KNOTS('',3,(#56210,#56211,#56212,#56213,#56214,
#56215,#56216,#56217,#56218,#56219,#56220,#56221,#56222,#56223,#56224,#56225,
#56226,#56227,#56228,#56229,#56230,#56231,#56232,#56233,#56234,#56235,#56236,
#56237,#56238,#56239,#56240,#56241,#56242,#56243,#56244,#56245,#56246,#56247,
#56248,#56249,#56250,#56251,#56252,#56253,#56254,#56255),.UNSPECIFIED.,
 .F.,.F.,(4,2,2,2,2,2,2,2,2,2,2,2,2,2,2,2,2,2,2,2,2,2,4),(9.56198978167309E-5,
0.0155193550344561,0.0256373012228276,0.0344142215086527,0.0480745154991777,
0.0898821437212078,0.11876831069995,0.134277603293621,0.15055282867365,
0.200251947837585,0.218411629353159,0.231621827313627,0.240355829566199,
0.25409557288221,0.295119188869773,0.32439106078887,0.339982215933523,0.356354956915731,
0.405519961437129,0.423843305304581,0.437133033790102,0.445895732161899,
0.458271301746286),.UNSPECIFIED.) ;
#1337=B_SPLINE_CURVE_WITH_KNOTS('',3,(#56262,#56263,#56264,#56265,#56266,
#56267,#56268,#56269,#56270,#56271,#56272,#56273,#56274,#56275,#56276,#56277,
#56278,#56279,#56280,#56281,#56282,#56283,#56284,#56285,#56286,#56287,#56288,
#56289,#56290,#56291,#56292,#56293,#56294,#56295,#56296,#56297,#56298,#56299,
#56300,#56301,#56302,#56303,#56304),.UNSPECIFIED.,.F.,.F.,(4,3,3,3,3,3,
3,3,3,3,3,3,3,3,4),(-17.9383918421104,-17.842556478735,-17.7333586134708,
-17.6242720817764,-17.515255375924,-17.4062670857227,-17.2971869615572,
-17.1880658673982,-17.0787374538633,-16.9804883875736,-16.9716433848556,
-16.9715852529204,-16.8695593508381,-16.8587164708144,-16.7649056225393),
 .UNSPECIFIED.) ;
#1338=B_SPLINE_CURVE_WITH_KNOTS('',3,(#56310,#56311,#56312,#56313,#56314,
#56315,#56316,#56317,#56318,#56319,#56320,#56321,#56322,#56323,#56324,#56325,
#56326,#56327,#56328,#56329,#56330,#56331,#56332,#56333,#56334,#56335,#56336,
#56337,#56338,#56339,#56340,#56341,#56342,#56343,#56344,#56345,#56346,#56347,
#56348,#56349,#56350,#56351,#56352,#56353,#56354,#56355,#56356,#56357,#56358,
#56359,#56360,#56361,#56362,#56363,#56364,#56365,#56366,#56367,#56368,#56369,
#56370,#56371,#56372,#56373,#56374,#56375,#56376,#56377,#56378,#56379,#56380,
#56381,#56382,#56383,#56384,#56385,#56386,#56387,#56388,#56389,#56390,#56391,
#56392,#56393,#56394,#56395,#56396,#56397,#56398,#56399,#56400,#56401,#56402,
#56403,#56404,#56405,#56406,#56407,#56408,#56409,#56410,#56411,#56412,#56413,
#56414,#56415,#56416,#56417,#56418,#56419,#56420,#56421,#56422,#56423,#56424,
#56425,#56426,#56427,#56428,#56429,#56430,#56431,#56432,#56433,#56434,#56435,
#56436,#56437,#56438,#56439,#56440,#56441,#56442,#56443,#56444,#56445,#56446,
#56447,#56448,#56449,#56450,#56451,#56452,#56453,#56454,#56455,#56456,#56457,
#56458,#56459,#56460,#56461,#56462,#56463,#56464,#56465,#56466,#56467,#56468,
#56469,#56470,#56471,#56472,#56473,#56474,#56475,#56476,#56477,#56478,#56479,
#56480,#56481,#56482,#56483,#56484,#56485,#56486,#56487,#56488,#56489,#56490,
#56491,#56492,#56493,#56494,#56495,#56496,#56497,#56498,#56499,#56500,#56501,
#56502,#56503,#56504,#56505,#56506,#56507,#56508),.UNSPECIFIED.,.F.,.F.,
(4,3,3,3,3,3,3,3,3,3,3,3,3,3,3,3,3,3,3,3,3,3,3,3,3,3,3,3,3,3,3,3,3,3,3,
3,3,3,3,3,3,3,3,3,3,3,3,3,3,3,3,3,3,3,3,3,3,3,3,3,3,3,3,3,3,3,4),(14.2295088655003,
14.3389583388931,14.4483526855265,14.5577326052243,14.6672179769316,14.7767554532794,
14.8864995972602,14.9748743412368,14.9749281643414,15.0752585779058,15.0846394854706,
15.1957166383656,15.3051248124756,15.4144660288951,15.5237811130958,15.6361500119795,
15.7456064359459,15.8594315722883,15.9579727480213,15.9732021021314,15.9732567086308,
16.0737965463703,16.0831951929036,16.1942439504057,16.30388050249,16.4134499406568,
16.522992739184,16.635140867618,16.7448212310155,16.8582032419678,16.9568851477706,
16.9715272588334,16.9715852529202,17.0721615462789,17.081298932139,17.1923757902729,
17.3017952886031,17.4111512159923,17.5204844288647,17.6328417709509,17.7423248774763,
17.856119337343,17.9543118630367,17.9698514639413,17.9699137972097,18.0695556702309,
18.0792537650142,18.1903773370748,18.299407578028,18.4083695126169,18.5173046389224,
18.6300390645666,18.7391185616584,18.8536804515787,18.9523645764336,18.968207786416,
18.9682423414991,19.070122838832,19.0804139585051,19.1923473335779,19.3041416432842,
19.4158321105052,19.5274538174148,19.6390844118875,19.7507101321439,19.8624454103262,
19.9665708857883),.UNSPECIFIED.) ;
#1339=B_SPLINE_CURVE_WITH_KNOTS('',3,(#56510,#56511,#56512,#56513,#56514,
#56515,#56516,#56517,#56518,#56519,#56520,#56521,#56522,#56523,#56524,#56525,
#56526,#56527,#56528,#56529,#56530,#56531,#56532,#56533,#56534,#56535,#56536,
#56537,#56538,#56539,#56540,#56541,#56542,#56543,#56544,#56545,#56546,#56547,
#56548,#56549,#56550,#56551,#56552,#56553,#56554,#56555,#56556,#56557,#56558,
#56559,#56560,#56561,#56562,#56563,#56564,#56565,#56566,#56567,#56568,#56569,
#56570,#56571,#56572,#56573,#56574,#56575,#56576,#56577,#56578,#56579,#56580,
#56581,#56582,#56583,#56584,#56585,#56586,#56587,#56588,#56589,#56590,#56591,
#56592,#56593,#56594,#56595,#56596,#56597,#56598,#56599,#56600,#56601,#56602,
#56603,#56604,#56605,#56606,#56607,#56608,#56609,#56610,#56611,#56612,#56613),
 .UNSPECIFIED.,.F.,.F.,(4,2,2,2,2,2,2,2,2,2,2,2,2,2,2,2,2,2,2,2,2,2,2,2,
2,2,2,2,2,2,2,2,2,2,2,2,2,2,2,2,2,2,2,2,2,2,2,2,2,2,2,4),(1.10920986980175,
1.11653740164681,1.13771123831766,1.16907366933029,1.18617897538512,1.19527680512883,
1.20788932723244,1.22583306009734,1.26361823026631,1.27906578579854,1.29658710580061,
1.31748720980365,1.35274550512533,1.36182087986681,1.3739898364051,1.39085974376577,
1.43148096289359,1.44663902389709,1.46451981315105,1.48629077793157,1.51895929967274,
1.52829235454364,1.53999383830962,1.55578141362031,1.59688701040672,1.61243501408099,
1.62969110733505,1.64997265934366,1.68525287030369,1.69476096474687,1.70607270300085,
1.7210004004899,1.76627501983604,1.78145697493476,1.80010059834877,1.84881182401862,
1.85960372224137,1.86933452340368,1.8810400885696,1.90948454784739,1.93419108950702,
1.94922498732281,1.96834389747161,1.99335689267842,2.01853610278449,2.02826757682473,
2.03921222740924,2.07090038355154,2.09901082443907,2.11438713698595,2.13260513630923,
2.15965741239705),.UNSPECIFIED.) ;
#1340=B_SPLINE_CURVE_WITH_KNOTS('',3,(#56619,#56620,#56621,#56622,#56623,
#56624,#56625,#56626,#56627,#56628),.UNSPECIFIED.,.F.,.F.,(4,2,2,2,4),(0.000104245096920715,
0.0139017618315296,0.0231479761800173,0.0326957883926925,0.0589262539191868),
 .UNSPECIFIED.) ;
#1341=B_SPLINE_CURVE_WITH_KNOTS('',3,(#56630,#56631,#56632,#56633,#56634,
#56635,#56636,#56637,#56638,#56639,#56640,#56641,#56642,#56643,#56644,#56645,
#56646,#56647,#56648,#56649,#56650,#56651,#56652,#56653,#56654,#56655,#56656,
#56657,#56658,#56659,#56660,#56661,#56662,#56663,#56664,#56665,#56666,#56667,
#56668,#56669,#56670,#56671,#56672,#56673,#56674,#56675,#56676,#56677,#56678,
#56679,#56680,#56681,#56682,#56683,#56684,#56685,#56686,#56687,#56688,#56689,
#56690,#56691,#56692,#56693,#56694,#56695,#56696,#56697,#56698,#56699,#56700,
#56701,#56702,#56703,#56704,#56705,#56706,#56707,#56708,#56709,#56710,#56711,
#56712,#56713,#56714,#56715,#56716,#56717,#56718,#56719,#56720,#56721,#56722,
#56723,#56724,#56725,#56726,#56727,#56728,#56729,#56730,#56731,#56732,#56733,
#56734,#56735,#56736,#56737,#56738,#56739,#56740,#56741,#56742,#56743,#56744,
#56745,#56746,#56747,#56748,#56749,#56750,#56751,#56752,#56753,#56754,#56755,
#56756,#56757,#56758,#56759),.UNSPECIFIED.,.F.,.F.,(4,3,3,3,3,3,3,3,3,3,
3,3,3,3,3,3,3,3,3,3,3,3,3,3,3,3,3,3,3,3,3,3,3,3,3,3,3,3,3,3,3,3,3,4),(-3.84638258862878,
-3.73821155326556,-3.63015790575673,-3.52217914496424,-3.41423251978327,
-3.30619919528476,-3.19812579616014,-3.08985237906168,-2.9950436281227,
-2.9949856328683,-2.89440933850989,-2.88527194896355,-2.77419509141547,
-2.66477558831422,-2.55541965612589,-2.4460864384266,-2.33372910096467,
-2.22424598956245,-2.11045153907066,-2.01225901005051,-1.99671942268382,
-1.99665708857887,-1.89701521204593,-1.8873171055871,-1.77619353542489,
-1.66716328029021,-1.55820133192825,-1.44926619227649,-1.33653178027973,
-1.22745227104431,-1.11289040766687,-1.01420626267801,-0.998363098870108,
-0.998328544289432,-0.896448042701214,-0.886156950979831,-0.774223599193483,
-0.662429312480799,-0.550738867904862,-0.439117183235771,-0.327486610177047,
-0.215860910885113,-0.104125652658588,-2.11597950287882E-13),
 .UNSPECIFIED.) ;
#1342=B_SPLINE_CURVE_WITH_KNOTS('',3,(#56763,#56764,#56765,#56766,#56767,
#56768,#56769,#56770,#56771,#56772,#56773,#56774,#56775,#56776,#56777,#56778,
#56779,#56780,#56781,#56782,#56783,#56784,#56785,#56786,#56787,#56788,#56789,
#56790,#56791,#56792,#56793,#56794,#56795,#56796,#56797,#56798,#56799,#56800,
#56801,#56802,#56803,#56804,#56805,#56806,#56807,#56808,#56809,#56810,#56811,
#56812,#56813,#56814,#56815,#56816,#56817,#56818,#56819,#56820,#56821,#56822,
#56823,#56824,#56825,#56826,#56827,#56828,#56829,#56830,#56831,#56832,#56833,
#56834,#56835,#56836,#56837,#56838,#56839,#56840,#56841,#56842,#56843,#56844,
#56845,#56846,#56847,#56848,#56849,#56850,#56851,#56852,#56853,#56854,#56855,
#56856,#56857,#56858,#56859,#56860,#56861,#56862,#56863,#56864,#56865,#56866,
#56867,#56868,#56869,#56870,#56871,#56872,#56873,#56874,#56875,#56876,#56877,
#56878,#56879,#56880,#56881,#56882,#56883,#56884,#56885,#56886,#56887,#56888,
#56889,#56890,#56891,#56892,#56893,#56894,#56895,#56896,#56897,#56898,#56899,
#56900,#56901,#56902,#56903,#56904,#56905,#56906,#56907,#56908,#56909,#56910,
#56911,#56912,#56913,#56914,#56915,#56916,#56917,#56918,#56919,#56920,#56921,
#56922,#56923,#56924,#56925,#56926,#56927,#56928,#56929,#56930,#56931,#56932,
#56933,#56934,#56935,#56936,#56937,#56938,#56939,#56940,#56941,#56942,#56943,
#56944,#56945,#56946,#56947,#56948,#56949,#56950,#56951,#56952,#56953,#56954,
#56955,#56956,#56957,#56958,#56959,#56960,#56961),.UNSPECIFIED.,.F.,.F.,
(4,3,3,3,3,3,3,3,3,3,3,3,3,3,3,3,3,3,3,3,3,3,3,3,3,3,3,3,3,3,3,3,3,3,3,
3,3,3,3,3,3,3,3,3,3,3,3,3,3,3,3,3,3,3,3,3,3,3,3,3,3,3,3,3,3,3,4),(2.02817886070011,
2.12401440243833,2.23321226279834,2.34229878960224,2.45131549057795,2.56030377591627,
2.66938389525482,2.77850498459844,2.88783339337641,2.98608246080593,2.99492750212187,
2.99498563286828,3.09556180779865,3.10491922853353,3.21596859711155,3.32560312559594,
3.43517161345578,3.54471453327594,3.65686444424638,3.76654756863079,3.87993087289425,
3.97857719176355,3.99325940849771,3.9933141771577,4.09372024726719,4.10302947216521,
4.21410612832545,4.32351594885692,4.43285794107218,4.54217293183031,4.65454037923451,
4.7639945634008,4.87781864242396,4.97628500966465,4.9915889173842,4.99164272144712,
5.09203102228959,5.10141980278939,5.21248873565778,5.32196240779199,5.43136884125333,
5.5407487543607,5.65305438220467,5.76257391804421,5.87627259189038,5.97483109049847,
5.98991796320581,5.98997126573655,6.09040665155374,6.09976820578768,6.21083465631747,
6.32032936931871,6.42975723173439,6.53915893081329,6.65144415061646,6.7609861270978,
6.87464296856189,6.9731943976366,6.98824622069259,6.98829981002598,7.08940591454106,
7.09951438005358,7.21054286125676,7.32140077463895,7.43215901695895,7.54285993587725,
7.59300756235165),.UNSPECIFIED.) ;
#1343=B_SPLINE_CURVE_WITH_KNOTS('',3,(#56962,#56963,#56964,#56965,#56966,
#56967,#56968,#56969),.UNSPECIFIED.,.F.,.F.,(4,2,2,4),(-1.10885368045049,
-1.08696980493825,-1.05541474700099,-1.05003427160778),.UNSPECIFIED.) ;
#1344=B_SPLINE_CURVE_WITH_KNOTS('',3,(#56976,#56977,#56978,#56979,#56980,
#56981,#56982,#56983,#56984,#56985,#56986,#56987,#56988,#56989,#56990,#56991,
#56992,#56993,#56994,#56995,#56996,#56997,#56998,#56999,#57000,#57001,#57002,
#57003,#57004,#57005,#57006,#57007,#57008,#57009,#57010,#57011,#57012,#57013,
#57014,#57015,#57016,#57017,#57018),.UNSPECIFIED.,.F.,.F.,(4,3,3,3,3,3,
3,3,3,3,3,3,3,3,4),(-17.938079539449,-17.8425480409392,-17.7333410205706,
-17.6242453229645,-17.5152194418143,-17.4062219683227,-17.2971326783531,
-17.188002412777,-17.0786648957393,-16.9804176491229,-16.9716454844279,
-16.9715852529204,-16.8695606965042,-16.8587073643271,-16.7648915192752),
 .UNSPECIFIED.) ;
#1345=B_SPLINE_CURVE_WITH_KNOTS('',3,(#57024,#57025,#57026,#57027,#57028,
#57029,#57030,#57031,#57032,#57033,#57034,#57035,#57036,#57037,#57038,#57039,
#57040,#57041,#57042,#57043,#57044,#57045,#57046,#57047,#57048,#57049,#57050,
#57051,#57052,#57053,#57054,#57055,#57056,#57057,#57058,#57059,#57060,#57061,
#57062,#57063,#57064,#57065,#57066,#57067,#57068,#57069,#57070,#57071,#57072,
#57073,#57074,#57075,#57076,#57077,#57078,#57079,#57080,#57081,#57082,#57083,
#57084,#57085,#57086,#57087,#57088,#57089,#57090,#57091,#57092,#57093,#57094,
#57095,#57096,#57097,#57098,#57099,#57100,#57101,#57102,#57103,#57104,#57105,
#57106,#57107,#57108,#57109,#57110,#57111,#57112,#57113,#57114,#57115,#57116,
#57117,#57118,#57119,#57120,#57121,#57122,#57123,#57124,#57125,#57126,#57127,
#57128,#57129,#57130,#57131,#57132,#57133,#57134,#57135,#57136,#57137,#57138,
#57139,#57140,#57141,#57142,#57143,#57144,#57145,#57146,#57147,#57148,#57149,
#57150,#57151,#57152,#57153,#57154,#57155,#57156,#57157,#57158,#57159,#57160,
#57161,#57162,#57163,#57164,#57165,#57166,#57167,#57168,#57169,#57170,#57171,
#57172,#57173,#57174,#57175,#57176,#57177,#57178,#57179,#57180,#57181,#57182,
#57183,#57184,#57185,#57186,#57187,#57188,#57189,#57190,#57191,#57192,#57193,
#57194,#57195,#57196,#57197,#57198,#57199,#57200,#57201,#57202,#57203,#57204,
#57205,#57206,#57207,#57208,#57209,#57210,#57211,#57212,#57213,#57214,#57215,
#57216,#57217,#57218,#57219,#57220,#57221,#57222),.UNSPECIFIED.,.F.,.F.,
(4,3,3,3,3,3,3,3,3,3,3,3,3,3,3,3,3,3,3,3,3,3,3,3,3,3,3,3,3,3,3,3,3,3,3,
3,3,3,3,3,3,3,3,3,3,3,3,3,3,3,3,3,3,3,3,3,3,3,3,3,3,3,3,3,3,3,4),(14.2294919259517,
14.3389381490702,14.4483292137904,14.5577058223085,14.6671878568696,14.776721974381,
14.8864627651101,14.9748739536409,14.9749281643414,15.0752587674523,15.0846370954552,
15.1957145471022,15.3051205991587,15.4144597976302,15.5237729697857,15.636143904497,
15.7455986944277,15.8594277015293,15.9579676391285,15.9732009683324,15.9732567086308,
16.0738029748843,16.0831962089879,16.1942448394794,16.3038831313914,16.4134545829914,
16.5229996713677,16.6351460667559,16.7448294089135,16.8582073309168,16.9568840398618,
16.9715251758643,16.9715852529202,17.0721638612044,17.0813079395613,17.1923836717674,
17.3018122533801,17.411177283829,17.520519617807,17.6328681626577,17.7423603933053,
17.8561370952575,17.9543359365701,17.9698500367431,17.9699137972097,18.0695597591183,
18.0792769675553,18.1903976392982,18.2994493704183,18.4084321055174,18.5173873144738,
18.6301010712301,18.7391986507741,18.8537204961366,18.9524367761661,18.9682086314664,
18.9682423414991,19.0701304113359,19.0803756098126,19.1922713484363,19.3040285239676,
19.415682447892,19.5272682918946,19.6388643971447,19.7504563748751,19.8621595718363,
19.9665708857883),.UNSPECIFIED.) ;
#1346=B_SPLINE_CURVE_WITH_KNOTS('',3,(#57224,#57225,#57226,#57227,#57228,
#57229,#57230,#57231,#57232,#57233,#57234,#57235,#57236,#57237,#57238,#57239,
#57240,#57241,#57242,#57243,#57244,#57245,#57246,#57247,#57248,#57249,#57250,
#57251,#57252,#57253,#57254,#57255,#57256,#57257,#57258,#57259,#57260,#57261,
#57262,#57263,#57264,#57265,#57266,#57267,#57268,#57269,#57270,#57271,#57272,
#57273,#57274,#57275,#57276,#57277,#57278,#57279,#57280,#57281,#57282,#57283,
#57284,#57285,#57286,#57287,#57288,#57289,#57290,#57291,#57292,#57293,#57294,
#57295,#57296,#57297,#57298,#57299,#57300,#57301,#57302,#57303,#57304,#57305,
#57306,#57307,#57308,#57309,#57310,#57311,#57312,#57313,#57314,#57315,#57316,
#57317,#57318,#57319,#57320,#57321,#57322,#57323,#57324,#57325),
 .UNSPECIFIED.,.F.,.F.,(4,2,2,2,2,2,2,2,2,2,2,2,2,2,2,2,2,2,2,2,2,2,2,2,
2,2,2,2,2,2,2,2,2,2,2,2,2,2,2,2,2,2,2,2,2,2,2,2,2,2,4),(1.10894604130966,
1.11627336363691,1.13744845361287,1.16882272821857,1.18590494333013,1.19499960459813,
1.20762946026794,1.22561879302956,1.26326981320216,1.27872261588766,1.29623077539129,
1.31710179780014,1.3524222080599,1.36149198082141,1.37368390575001,1.39061053417187,
1.43106308715466,1.44622844891658,1.46408529560854,1.4858009244646,1.51858805580375,
1.52791156434614,1.53964154921547,1.55549588654148,1.59639725374685,1.6119563226357,
1.62918243733498,1.64939828671883,1.68486297139135,1.69435047401396,1.70571168392109,
1.72074904504411,1.7652272488211,1.78046325505563,1.79874084752736,1.85028822390102,
1.86025453118219,1.87073306078469,1.90215593343046,1.93149459367087,1.94659576105821,
1.96424361239819,1.98550925177549,2.01975587604291,2.02890229557161,2.04093901561324,
2.05745505594631,2.09872531277398,2.11406288297816,2.13250330112224,2.15906108059027),
 .UNSPECIFIED.) ;
#1347=B_SPLINE_CURVE_WITH_KNOTS('',3,(#57331,#57332,#57333,#57334,#57335,
#57336,#57337,#57338,#57339,#57340),.UNSPECIFIED.,.F.,.F.,(4,2,2,2,4),(0.000105126802572485,
0.014031716210766,0.0233742014449894,0.0330434563056765,0.0589148629143721),
 .UNSPECIFIED.) ;
#1348=B_SPLINE_CURVE_WITH_KNOTS('',3,(#57342,#57343,#57344,#57345,#57346,
#57347,#57348,#57349,#57350,#57351,#57352,#57353,#57354,#57355,#57356,#57357,
#57358,#57359,#57360,#57361,#57362,#57363,#57364,#57365,#57366,#57367,#57368,
#57369,#57370,#57371,#57372,#57373,#57374,#57375,#57376,#57377,#57378,#57379,
#57380,#57381,#57382,#57383,#57384,#57385,#57386,#57387,#57388,#57389,#57390,
#57391,#57392,#57393,#57394,#57395,#57396,#57397,#57398,#57399,#57400,#57401,
#57402,#57403,#57404,#57405,#57406,#57407,#57408,#57409,#57410,#57411,#57412,
#57413,#57414,#57415,#57416,#57417,#57418,#57419,#57420,#57421,#57422,#57423,
#57424,#57425,#57426,#57427,#57428,#57429,#57430,#57431,#57432,#57433,#57434,
#57435,#57436,#57437,#57438,#57439,#57440,#57441,#57442,#57443,#57444,#57445,
#57446,#57447,#57448,#57449,#57450,#57451,#57452,#57453,#57454,#57455,#57456,
#57457,#57458,#57459,#57460,#57461,#57462,#57463,#57464,#57465,#57466,#57467,
#57468,#57469,#57470,#57471),.UNSPECIFIED.,.F.,.F.,(4,3,3,3,3,3,3,3,3,3,
3,3,3,3,3,3,3,3,3,3,3,3,3,3,3,3,3,3,3,3,3,3,3,3,3,3,3,3,3,3,3,3,3,4),(-3.84638256813386,
-3.73820850425281,-3.63015156663993,-3.52216926327145,-3.41421884243916,
-3.30618133487243,-3.19810353321684,-3.08982537936042,-2.99504571094475,
-2.9949856328683,-2.89440702304788,-2.88526294147605,-2.77418720986391,
-2.66475862349703,-2.55539358829796,-2.44605124957496,-2.33370270932594,
-2.22421047397042,-2.11043378127464,-2.01223493666377,-1.99672084972804,
-1.99665708857887,-1.89701112545988,-1.88729390833867,-1.77617323783252,
-1.66712149763544,-1.5581387537861,-1.44918353641828,-1.33646978838607,
-1.22737220136461,-1.11285037282702,-1.01413407829555,-0.998362253922141,
-0.998328544289434,-0.896440470790495,-0.886195293396442,-0.774299571846485,
-0.662542413147004,-0.550888505773211,-0.439302677999796,-0.327706588337476,
-0.216114625846442,-0.104411443356276,-5.31522163870105E-13),
 .UNSPECIFIED.) ;
#1349=B_SPLINE_CURVE_WITH_KNOTS('',3,(#57475,#57476,#57477,#57478,#57479,
#57480,#57481,#57482,#57483,#57484,#57485,#57486,#57487,#57488,#57489,#57490,
#57491,#57492,#57493,#57494,#57495,#57496,#57497,#57498,#57499,#57500,#57501,
#57502,#57503,#57504,#57505,#57506,#57507,#57508,#57509,#57510,#57511,#57512,
#57513,#57514,#57515,#57516,#57517,#57518,#57519,#57520,#57521,#57522,#57523,
#57524,#57525,#57526,#57527,#57528,#57529,#57530,#57531,#57532,#57533,#57534,
#57535,#57536,#57537,#57538,#57539,#57540,#57541,#57542,#57543,#57544,#57545,
#57546,#57547,#57548,#57549,#57550,#57551,#57552,#57553,#57554,#57555,#57556,
#57557,#57558,#57559,#57560,#57561,#57562,#57563,#57564,#57565,#57566,#57567,
#57568,#57569,#57570,#57571,#57572,#57573,#57574,#57575,#57576,#57577,#57578,
#57579,#57580,#57581,#57582,#57583,#57584,#57585,#57586,#57587,#57588,#57589,
#57590,#57591,#57592,#57593,#57594,#57595,#57596,#57597,#57598,#57599,#57600,
#57601,#57602,#57603,#57604,#57605,#57606,#57607,#57608,#57609,#57610,#57611,
#57612,#57613,#57614,#57615,#57616,#57617,#57618,#57619,#57620,#57621,#57622,
#57623,#57624,#57625,#57626,#57627,#57628,#57629,#57630,#57631,#57632,#57633,
#57634,#57635,#57636,#57637,#57638,#57639,#57640,#57641,#57642,#57643,#57644,
#57645,#57646,#57647,#57648,#57649,#57650,#57651,#57652,#57653,#57654,#57655,
#57656,#57657,#57658,#57659,#57660,#57661,#57662,#57663,#57664,#57665,#57666,
#57667,#57668,#57669,#57670,#57671,#57672,#57673),.UNSPECIFIED.,.F.,.F.,
(4,3,3,3,3,3,3,3,3,3,3,3,3,3,3,3,3,3,3,3,3,3,3,3,3,3,3,3,3,3,3,3,3,3,3,
3,3,3,3,3,3,3,3,3,3,3,3,3,3,3,3,3,3,3,3,3,3,3,3,3,3,3,3,3,3,3,4),(2.02849119681895,
2.12402284058456,2.23322985623704,2.34232554910588,2.45135142549916,2.56034889421509,
2.66943817939672,2.77856844017022,2.8879059524223,2.98615319978999,2.99492540240048,
2.99498563286828,3.09555793178458,3.1049227617298,3.21597168865829,3.32560899891808,
3.43517998953789,3.54472513678483,3.65687239687805,3.76655707843461,3.87993562779616,
3.97858788803385,3.99325823756284,3.99331417715771,4.09371916216987,4.10302808104315,
4.21410491109365,4.32351302343983,4.43285319274963,4.54216624802883,4.65453536638341,
4.76398735355505,4.87781503750109,4.97628194727701,4.99158851592506,4.99164272144713,
5.09202984908505,5.10141645669967,5.21248580782928,5.32195615323443,5.43135927257129,
5.5407358864701,5.65304473128672,5.76256102779188,5.87626614676422,5.97482204959029,
5.98991768793335,5.98997126573656,6.0904063371316,6.0997675247197,6.21083406038298,
6.32032822177535,6.42975558054475,6.53915682320765,6.65144256991223,6.76098420489217,
6.87464200745908,6.97319267264661,6.98824579430711,6.98829981002598,7.0894064044638,
7.099515038111,7.21054420905378,7.32140285463792,7.43216185294655,7.54286355851905,
7.59300756235355),.UNSPECIFIED.) ;
#1350=B_SPLINE_CURVE_WITH_KNOTS('',3,(#57674,#57675,#57676,#57677,#57678,
#57679,#57680,#57681),.UNSPECIFIED.,.F.,.F.,(4,2,2,4),(-1.10883530707003,
-1.08691376692716,-1.0553640497396,-1.05001965519088),.UNSPECIFIED.) ;
#1351=B_SPLINE_CURVE_WITH_KNOTS('',3,(#57687,#57688,#57689,#57690,#57691,
#57692,#57693,#57694,#57695,#57696,#57697,#57698,#57699,#57700,#57701,#57702,
#57703,#57704,#57705,#57706,#57707,#57708,#57709,#57710,#57711,#57712),
 .UNSPECIFIED.,.F.,.F.,(4,2,2,2,2,2,2,2,2,2,2,2,4),(0.459092828659847,0.46458280938324,
0.505879393319841,0.521008735046651,0.529991319325623,0.542633449959227,
0.575929685166336,0.614621897851766,0.632497588871837,0.649228900547743,
0.666866115107942,0.722578742135439,0.732479068875876),.UNSPECIFIED.) ;
#1352=B_SPLINE_CURVE_WITH_KNOTS('',3,(#57715,#57716,#57717,#57718,#57719,
#57720,#57721,#57722,#57723,#57724,#57725,#57726,#57727,#57728,#57729,#57730,
#57731,#57732,#57733,#57734,#57735,#57736,#57737,#57738,#57739,#57740,#57741,
#57742,#57743,#57744,#57745,#57746,#57747,#57748,#57749,#57750),
 .UNSPECIFIED.,.F.,.F.,(4,2,2,2,2,2,2,2,2,2,2,2,2,2,2,2,2,4),(0.000333295488794572,
0.00533169420316919,0.0119863859187359,0.048691939483201,0.0844017923136275,
0.100356581500467,0.116281319030886,0.149692705305946,0.1783076015109,0.190742024534847,
0.201078659920755,0.210405171548014,0.232103074145979,0.282226565630108,
0.300212219360226,0.315193011616712,0.337127704802259,0.381140802024926),
 .UNSPECIFIED.) ;
#1353=B_SPLINE_CURVE_WITH_KNOTS('',3,(#57756,#57757,#57758,#57759,#57760,
#57761,#57762,#57763,#57764,#57765,#57766,#57767,#57768,#57769,#57770,#57771,
#57772,#57773,#57774,#57775,#57776,#57777,#57778,#57779,#57780,#57781,#57782,
#57783,#57784,#57785,#57786,#57787,#57788,#57789,#57790,#57791,#57792,#57793,
#57794,#57795,#57796,#57797,#57798,#57799,#57800,#57801,#57802,#57803,#57804,
#57805,#57806,#57807,#57808,#57809,#57810,#57811,#57812,#57813,#57814,#57815,
#57816,#57817,#57818,#57819,#57820,#57821,#57822,#57823,#57824,#57825,#57826,
#57827,#57828,#57829,#57830,#57831,#57832,#57833),.UNSPECIFIED.,.F.,.F.,
(4,2,2,2,2,2,2,2,2,2,2,2,2,2,2,2,2,2,2,2,2,2,2,2,2,2,2,2,2,2,2,2,2,2,2,
2,2,2,4),(1.29359361912601,1.30106987292448,1.31750403155353,1.33306635135568,
1.36187428370035,1.40299397077918,1.41701197002479,1.42577387270662,1.43884531163003,
1.45667948572154,1.50738242336099,1.52363298492541,1.53932799920826,1.57014056486922,
1.61063065145667,1.623517366373,1.63229811331715,1.64661281546571,1.66734113986291,
1.71288214330797,1.7290835487098,1.74478576388706,1.77584413634624,1.81632835476311,
1.82912521118274,1.83788291242882,1.85217474358337,1.87285804431839,1.9184471776329,
1.93458554047298,1.95018735587936,1.9803875670598,2.02133212904445,2.03461501728283,
2.04340752395374,2.05733245183337,2.07707132400357,2.11467829361035,2.12882907516074),
 .UNSPECIFIED.) ;
#1354=B_SPLINE_CURVE_WITH_KNOTS('',3,(#57834,#57835,#57836,#57837,#57838,
#57839,#57840,#57841,#57842,#57843,#57844,#57845,#57846,#57847,#57848,#57849,
#57850,#57851,#57852,#57853,#57854,#57855,#57856,#57857,#57858,#57859,#57860,
#57861,#57862,#57863,#57864,#57865,#57866,#57867,#57868,#57869,#57870,#57871,
#57872,#57873,#57874,#57875),.UNSPECIFIED.,.F.,.F.,(4,2,2,2,2,2,2,2,2,2,
2,2,2,2,2,2,2,2,2,2,4),(0.000734533073629474,0.0138790511024117,0.0296566148513827,
0.0802346251044167,0.106665857315606,0.116373796810632,0.126501899960165,
0.164778388123386,0.201300657865272,0.217475187060577,0.233584299088167,
0.267597394367349,0.296198479539202,0.313243933653704,0.322093358567795,
0.332453617478739,0.366407046245808,0.408190077661704,0.424914882262875,
0.439911329919575,0.459092828659847),.UNSPECIFIED.) ;
#1355=B_SPLINE_CURVE_WITH_KNOTS('',3,(#57876,#57877,#57878,#57879,#57880,
#57881,#57882,#57883,#57884,#57885,#57886,#57887,#57888,#57889,#57890,#57891,
#57892,#57893,#57894,#57895,#57896,#57897,#57898,#57899,#57900,#57901,#57902,
#57903,#57904,#57905,#57906,#57907,#57908,#57909,#57910,#57911,#57912,#57913,
#57914,#57915,#57916,#57917,#57918,#57919,#57920,#57921,#57922,#57923,#57924,
#57925,#57926,#57927,#57928,#57929,#57930,#57931,#57932,#57933,#57934,#57935,
#57936,#57937,#57938,#57939,#57940,#57941,#57942,#57943,#57944,#57945,#57946,
#57947,#57948,#57949,#57950,#57951,#57952,#57953,#57954,#57955,#57956,#57957,
#57958,#57959,#57960,#57961,#57962,#57963,#57964,#57965,#57966,#57967,#57968,
#57969,#57970,#57971,#57972,#57973,#57974,#57975,#57976,#57977,#57978,#57979,
#57980,#57981,#57982,#57983,#57984,#57985,#57986,#57987,#57988,#57989,#57990,
#57991,#57992,#57993),.UNSPECIFIED.,.F.,.F.,(4,2,2,2,2,2,2,2,2,2,2,2,2,
2,2,2,2,2,2,2,2,2,2,2,2,2,2,2,2,2,2,2,2,2,2,2,2,2,2,2,2,2,2,2,2,2,2,2,2,
2,2,2,2,2,2,2,2,2,4),(9.9999999739413E-7,0.0160738874198969,0.0243015288141959,
0.0331995744590351,0.0509725032934508,0.0913818065799422,0.111457641442597,
0.127727564529213,0.143078744774428,0.170817330016844,0.20581943179008,
0.219335709806031,0.230254102060281,0.239265195718039,0.257369449100544,
0.297791259046865,0.317949924898833,0.334051303539227,0.349654113706522,
0.404856472005175,0.428706238735585,0.438214816383149,0.448294410421727,
0.48701762271562,0.521794091712671,0.53832480323903,0.553696441310369,0.580724198831505,
0.616695673361533,0.630366418165186,0.641370973970987,0.650377376883583,
0.668310842685775,0.708820817694532,0.72899296528574,0.745097716403503,
0.760716399539172,0.815957566093128,0.839872655156268,0.849381354834161,
0.85942268120762,0.89860037183343,0.935662834432564,0.951546389770785,0.967363065175678,
1.01717070951904,1.03632569817519,1.04996676214464,1.05867044847102,1.0718550912914,
1.11255678435931,1.14271858391255,1.15830493726752,1.17446102876239,1.22539811312515,
1.25082901670304,1.26043620180714,1.270367123206,1.29395065554619),
 .UNSPECIFIED.) ;
#1356=B_SPLINE_CURVE_WITH_KNOTS('',3,(#57999,#58000,#58001,#58002,#58003,
#58004,#58005,#58006,#58007,#58008,#58009,#58010,#58011,#58012,#58013,#58014,
#58015,#58016,#58017,#58018,#58019,#58020,#58021,#58022,#58023,#58024,#58025,
#58026,#58027,#58028,#58029,#58030,#58031,#58032,#58033,#58034,#58035,#58036,
#58037,#58038,#58039,#58040,#58041,#58042,#58043,#58044,#58045,#58046,#58047,
#58048,#58049,#58050,#58051,#58052,#58053,#58054,#58055,#58056,#58057,#58058,
#58059,#58060,#58061,#58062,#58063,#58064,#58065,#58066,#58067,#58068,#58069,
#58070,#58071,#58072,#58073,#58074,#58075,#58076,#58077,#58078,#58079,#58080,
#58081,#58082,#58083,#58084,#58085,#58086,#58087,#58088,#58089),
 .UNSPECIFIED.,.F.,.F.,(4,3,3,3,3,3,3,3,3,3,3,3,3,3,3,3,3,3,3,3,3,3,3,3,
3,3,3,3,3,3,4),(15.7079632679487,15.8113185661092,15.9146477682657,16.0179862497935,
16.1214445336244,16.2249671723021,16.3224787353659,16.3286854519248,16.3947463489873,
16.394798101356,16.4893686487847,16.4989555611429,16.6029531946589,16.7068224059803,
16.8106222565616,16.9143876724686,17.0181535323515,17.122023334568,17.2259490949981,
17.3243546278831,17.3300536422211,17.3930765924381,17.3931266456453,17.4881585315426,
17.4974456208808,17.6010533743386,17.6065584824799,17.7106015728288,17.8145755365523,
17.9185210511146,17.9338970672771),.UNSPECIFIED.) ;
#1357=B_SPLINE_CURVE_WITH_KNOTS('',3,(#58091,#58092,#58093,#58094,#58095,
#58096,#58097,#58098,#58099,#58100,#58101,#58102,#58103,#58104,#58105,#58106,
#58107,#58108,#58109,#58110,#58111,#58112,#58113,#58114,#58115,#58116,#58117,
#58118,#58119,#58120,#58121,#58122,#58123,#58124,#58125,#58126,#58127,#58128,
#58129,#58130),.UNSPECIFIED.,.F.,.F.,(4,3,3,3,3,3,3,3,3,3,3,3,3,4),(14.3981410127773,
14.5041275779632,14.6100285359095,14.7158970806972,14.8217531608633,14.9276267469892,
15.0335478199294,15.1396253540428,15.2457909511983,15.3521586464516,15.3964695570666,
15.5189994551258,15.6402222711559,15.7079554221965),.UNSPECIFIED.) ;
#1358=B_SPLINE_CURVE_WITH_KNOTS('',3,(#58133,#58134,#58135,#58136,#58137,
#58138,#58139,#58140,#58141,#58142,#58143,#58144,#58145,#58146,#58147,#58148,
#58149,#58150,#58151,#58152,#58153,#58154,#58155,#58156,#58157,#58158,#58159,
#58160,#58161,#58162,#58163,#58164,#58165,#58166,#58167,#58168,#58169,#58170,
#58171,#58172,#58173,#58174,#58175,#58176,#58177,#58178,#58179,#58180,#58181,
#58182,#58183,#58184,#58185,#58186,#58187,#58188,#58189,#58190,#58191,#58192,
#58193,#58194,#58195,#58196,#58197,#58198,#58199,#58200,#58201,#58202,#58203,
#58204,#58205,#58206,#58207,#58208,#58209,#58210),.UNSPECIFIED.,.F.,.F.,
(4,2,2,2,2,2,2,2,2,2,2,2,2,2,2,2,2,2,2,2,2,2,2,2,2,2,2,2,2,2,2,2,2,2,2,
2,2,2,4),(9.11640338329011E-5,0.0051025466412606,0.0113875670523336,0.0548470562170383,
0.0857482806918087,0.101417815155263,0.117653019630782,0.166957731175739,
0.192706981078215,0.202333248824673,0.212252232765116,0.252876439023877,
0.277779339804877,0.297584062449989,0.312468457507578,0.331838238059752,
0.375873450570578,0.398590164456944,0.408032189351106,0.418096415804966,
0.430099242590052,0.456627998374622,0.494015251410843,0.5098507658762,0.525317201277499,
0.55584552958573,0.596302274316993,0.609196791407187,0.617827198975333,
0.631448481288996,0.650604889682355,0.700320208050008,0.716058185493827,
0.731770099253375,0.766102498367211,0.808240308785967,0.818255737119278,
0.826146810363654,0.835757597382848),.UNSPECIFIED.) ;
#1359=B_SPLINE_CURVE_WITH_KNOTS('',3,(#58216,#58217,#58218,#58219,#58220,
#58221,#58222,#58223,#58224,#58225,#58226,#58227,#58228,#58229,#58230,#58231,
#58232,#58233,#58234,#58235,#58236,#58237,#58238,#58239,#58240,#58241),
 .UNSPECIFIED.,.F.,.F.,(4,2,2,2,2,2,2,2,2,2,2,2,4),(0.459101110943174,0.464354084783774,
0.505377027644394,0.520997705906278,0.529963645940253,0.542471817233919,
0.575280333026665,0.614901030815203,0.632766276068313,0.649542615135927,
0.667261331011091,0.72253469686435,0.732483173568347),.UNSPECIFIED.) ;
#1360=B_SPLINE_CURVE_WITH_KNOTS('',3,(#58244,#58245,#58246,#58247,#58248,
#58249,#58250,#58251,#58252,#58253,#58254,#58255,#58256,#58257,#58258,#58259,
#58260,#58261,#58262,#58263,#58264,#58265,#58266,#58267,#58268,#58269,#58270,
#58271,#58272,#58273,#58274,#58275,#58276,#58277,#58278,#58279),
 .UNSPECIFIED.,.F.,.F.,(4,2,2,2,2,2,2,2,2,2,2,2,2,2,2,2,2,4),(0.000327211641307999,
0.00531276958370105,0.011942178793651,0.0491171206788442,0.0844907768687678,
0.100422340388374,0.116322911773884,0.149510046624113,0.178269548979332,
0.190729453077571,0.201079787432153,0.210407580488322,0.232088112343222,
0.282131222632167,0.300112650559163,0.315080422309398,0.336959281230109,
0.381143861704028),.UNSPECIFIED.) ;
#1361=B_SPLINE_CURVE_WITH_KNOTS('',3,(#58285,#58286,#58287,#58288,#58289,
#58290,#58291,#58292,#58293,#58294,#58295,#58296,#58297,#58298,#58299,#58300,
#58301,#58302,#58303,#58304,#58305,#58306,#58307,#58308,#58309,#58310,#58311,
#58312,#58313,#58314,#58315,#58316,#58317,#58318,#58319,#58320,#58321,#58322,
#58323,#58324,#58325,#58326,#58327,#58328,#58329,#58330,#58331,#58332,#58333,
#58334,#58335,#58336,#58337,#58338,#58339,#58340,#58341,#58342,#58343,#58344,
#58345,#58346,#58347,#58348,#58349,#58350,#58351,#58352,#58353,#58354,#58355,
#58356,#58357,#58358,#58359,#58360,#58361,#58362),.UNSPECIFIED.,.F.,.F.,
(4,2,2,2,2,2,2,2,2,2,2,2,2,2,2,2,2,2,2,2,2,2,2,2,2,2,2,2,2,2,2,2,2,2,2,
2,2,2,4),(1.29362987758487,1.30089907076155,1.31737875058471,1.3329043258506,
1.36124830246446,1.40248211826036,1.41681275265866,1.42558201814846,1.43839619816745,
1.45567241916341,1.5097097437419,1.52544352982289,1.54163064892364,1.56182405576991,
1.60248744352981,1.62033145379943,1.62928220105769,1.64040671981978,1.65427714699489,
1.69156480647918,1.71735948797143,1.73253846774084,1.74936390666995,1.76804611359679,
1.81102421322096,1.82682871782048,1.83567257446723,1.84753935964157,1.88074677457094,
1.91928590673729,1.93521642888214,1.9509776165905,1.98422212626801,2.02765785097719,
2.03789161381674,2.04743919730058,2.0707566216888,2.1163762040201,2.12870581412763),
 .UNSPECIFIED.) ;
#1362=B_SPLINE_CURVE_WITH_KNOTS('',3,(#58363,#58364,#58365,#58366,#58367,
#58368,#58369,#58370,#58371,#58372,#58373,#58374,#58375,#58376,#58377,#58378,
#58379,#58380,#58381,#58382,#58383,#58384,#58385,#58386,#58387,#58388,#58389,
#58390,#58391,#58392,#58393,#58394,#58395,#58396,#58397,#58398,#58399,#58400,
#58401,#58402,#58403,#58404),.UNSPECIFIED.,.F.,.F.,(4,2,2,2,2,2,2,2,2,2,
2,2,2,2,2,2,2,2,2,2,4),(0.000739397909415687,0.0138412325044495,0.0295352759641673,
0.0792037035965399,0.106541526696309,0.116294270869245,0.126382320725574,
0.165125340584505,0.201321192902339,0.217459634847154,0.233555712978872,
0.267479454618907,0.296223261584647,0.313312125494654,0.322158943272101,
0.332516024622701,0.366427842431594,0.408040859835102,0.424741542140745,
0.439725818137328,0.459101110943174),.UNSPECIFIED.) ;
#1363=B_SPLINE_CURVE_WITH_KNOTS('',3,(#58405,#58406,#58407,#58408,#58409,
#58410,#58411,#58412,#58413,#58414,#58415,#58416,#58417,#58418,#58419,#58420,
#58421,#58422,#58423,#58424,#58425,#58426,#58427,#58428,#58429,#58430,#58431,
#58432,#58433,#58434,#58435,#58436,#58437,#58438,#58439,#58440,#58441,#58442,
#58443,#58444,#58445,#58446,#58447,#58448,#58449,#58450,#58451,#58452,#58453,
#58454,#58455,#58456,#58457,#58458,#58459,#58460,#58461,#58462,#58463,#58464,
#58465,#58466,#58467,#58468,#58469,#58470,#58471,#58472,#58473,#58474,#58475,
#58476,#58477,#58478,#58479,#58480,#58481,#58482,#58483,#58484,#58485,#58486,
#58487,#58488,#58489,#58490,#58491,#58492,#58493,#58494,#58495,#58496,#58497,
#58498,#58499,#58500,#58501,#58502,#58503,#58504,#58505,#58506,#58507,#58508,
#58509,#58510,#58511,#58512,#58513,#58514,#58515,#58516,#58517,#58518,#58519,
#58520),.UNSPECIFIED.,.F.,.F.,(4,2,2,2,2,2,2,2,2,2,2,2,2,2,2,2,2,2,2,2,
2,2,2,2,2,2,2,2,2,2,2,2,2,2,2,2,2,2,2,2,2,2,2,2,2,2,2,2,2,2,2,2,2,2,2,2,
2,4),(1.0000000227918E-6,0.016150234256278,0.0243635252181724,0.0333737690104111,
0.0514110440662363,0.0918108935996449,0.111922267913714,0.128057346526151,
0.143494986960628,0.172393810303427,0.206237998757624,0.219576650432681,
0.23039822943815,0.239439859401816,0.257874384261227,0.297938597922265,
0.318067340872359,0.334141819533777,0.3497721960782,0.40436017980479,0.428614839934304,
0.438149900351881,0.448189395863537,0.487401859487926,0.523758810157126,
0.53978852569054,0.555476142512416,0.609030315051042,0.634063864344299,
0.643645826385148,0.653599569332248,0.693758198031548,0.730119447399353,
0.745976834881271,0.761797529179021,0.791625082917581,0.823689745585661,
0.841721547803439,0.850732235107347,0.861699880985403,0.911297282661011,
0.938339273537299,0.953703949654931,0.970223302942397,1.01736770922379,
1.03638319681025,1.04996207192976,1.05866165389312,1.07189242424699,1.11261372824132,
1.14267376817757,1.15824847834276,1.17440513574077,1.22525734750247,1.25071900847628,
1.26032500820491,1.27024816493027,1.2938343569962),.UNSPECIFIED.) ;
#1364=B_SPLINE_CURVE_WITH_KNOTS('',3,(#58526,#58527,#58528,#58529,#58530,
#58531,#58532,#58533,#58534,#58535,#58536,#58537,#58538,#58539,#58540,#58541,
#58542,#58543,#58544,#58545,#58546,#58547,#58548,#58549,#58550,#58551,#58552,
#58553,#58554,#58555,#58556,#58557,#58558,#58559,#58560,#58561,#58562,#58563,
#58564,#58565,#58566,#58567,#58568,#58569,#58570,#58571,#58572,#58573,#58574,
#58575,#58576,#58577,#58578,#58579,#58580,#58581,#58582,#58583,#58584,#58585,
#58586,#58587,#58588,#58589,#58590,#58591,#58592,#58593,#58594,#58595,#58596,
#58597,#58598,#58599,#58600,#58601,#58602,#58603,#58604,#58605,#58606,#58607,
#58608,#58609,#58610,#58611,#58612,#58613,#58614,#58615,#58616),
 .UNSPECIFIED.,.F.,.F.,(4,3,3,3,3,3,3,3,3,3,3,3,3,3,3,3,3,3,3,3,3,3,3,3,
3,3,3,3,3,3,4),(15.7079632679487,15.811298560919,15.9146070461799,16.0179241280816,
16.1213600993717,16.2248598840742,16.3223793192546,16.3285546604084,16.3947472862124,
16.3947981013537,16.4893612956316,16.4989474321208,16.6029368813412,16.7067978361585,
16.8105893856834,16.9143464584217,17.0181039354167,17.1219653241399,17.2258826400782,
17.3242930388564,17.3299787615837,17.3930781390119,17.3931266456432,17.4881609860694,
17.4974415964232,17.6010536984685,17.6065544877355,17.7105941015318,17.814564776613,
17.9185072616035,17.9338931616724),.UNSPECIFIED.) ;
#1365=B_SPLINE_CURVE_WITH_KNOTS('',3,(#58618,#58619,#58620,#58621,#58622,
#58623,#58624,#58625,#58626,#58627,#58628,#58629,#58630,#58631,#58632,#58633,
#58634,#58635,#58636,#58637,#58638,#58639,#58640,#58641,#58642,#58643,#58644,
#58645,#58646,#58647,#58648,#58649,#58650,#58651,#58652,#58653,#58654,#58655,
#58656,#58657),.UNSPECIFIED.,.F.,.F.,(4,3,3,3,3,3,3,3,3,3,3,3,3,4),(14.3981410127747,
14.5041514455698,14.6100772086715,14.7159717739477,14.8218545927831,14.9277555738488,
15.0337046369196,15.1398108276545,15.2460054861428,15.3524025388386,15.3964695570642,
15.519015734404,15.6402459361385,15.7079553921828),.UNSPECIFIED.) ;
#1366=B_SPLINE_CURVE_WITH_KNOTS('',3,(#58660,#58661,#58662,#58663,#58664,
#58665,#58666,#58667,#58668,#58669,#58670,#58671,#58672,#58673,#58674,#58675,
#58676,#58677,#58678,#58679,#58680,#58681,#58682,#58683,#58684,#58685,#58686,
#58687,#58688,#58689,#58690,#58691,#58692,#58693,#58694,#58695,#58696,#58697,
#58698,#58699,#58700,#58701,#58702,#58703,#58704,#58705,#58706,#58707,#58708,
#58709,#58710,#58711,#58712,#58713,#58714,#58715,#58716,#58717,#58718,#58719,
#58720,#58721,#58722,#58723,#58724,#58725,#58726,#58727,#58728,#58729,#58730,
#58731,#58732,#58733),.UNSPECIFIED.,.F.,.F.,(4,2,2,2,2,2,2,2,2,2,2,2,2,
2,2,2,2,2,2,2,2,2,2,2,2,2,2,2,2,2,2,2,2,2,2,2,4),(8.9593587986984E-5,0.00952093609751188,
0.0633488659849307,0.0834941189489905,0.099655415189997,0.115334705893301,
0.167927086572246,0.192896620540458,0.202477430415909,0.212461292430139,
0.252316259026952,0.277477254805576,0.297385234412671,0.312258519839811,
0.331492489948905,0.375621279613763,0.398601940600346,0.408056006597219,
0.418087133787787,0.451228293324594,0.491755232729443,0.508170422783087,
0.523289133651666,0.549016933433626,0.593139017551487,0.607852077954839,
0.616524557735506,0.628609638320433,0.661720602807763,0.699769801191,0.715631535074734,
0.731230302036858,0.763097776354719,0.808060373537215,0.818141454642955,
0.826088585101868,0.835762250436862),.UNSPECIFIED.) ;
#1367=B_SPLINE_CURVE_WITH_KNOTS('',3,(#58740,#58741,#58742,#58743,#58744,
#58745,#58746,#58747,#58748,#58749,#58750,#58751,#58752,#58753,#58754,#58755,
#58756,#58757,#58758,#58759,#58760,#58761,#58762,#58763,#58764,#58765,#58766,
#58767,#58768,#58769,#58770,#58771,#58772,#58773,#58774,#58775,#58776,#58777,
#58778,#58779,#58780,#58781,#58782),.UNSPECIFIED.,.F.,.F.,(4,3,3,3,3,3,
3,3,3,3,3,3,3,3,4),(-17.9381511473345,-17.8425500608732,-17.7333452660566,
-17.6242518023618,-17.5152281629583,-17.4062329385398,-17.2971459013018,
-17.188017894178,-17.0786826257273,-16.9804349880921,-16.9716449904015,
-16.9715852529217,-16.8695605066972,-16.8587096350255,-16.7648949639448),
 .UNSPECIFIED.) ;
#1368=B_SPLINE_CURVE_WITH_KNOTS('',3,(#58788,#58789,#58790,#58791,#58792,
#58793,#58794,#58795,#58796,#58797,#58798,#58799,#58800,#58801,#58802,#58803,
#58804,#58805,#58806,#58807,#58808,#58809,#58810,#58811,#58812,#58813,#58814,
#58815,#58816,#58817,#58818,#58819,#58820,#58821,#58822,#58823,#58824,#58825,
#58826,#58827,#58828,#58829,#58830,#58831,#58832,#58833,#58834,#58835,#58836,
#58837,#58838,#58839,#58840,#58841,#58842,#58843,#58844,#58845,#58846,#58847,
#58848,#58849,#58850,#58851,#58852,#58853,#58854,#58855,#58856,#58857,#58858,
#58859,#58860,#58861,#58862,#58863,#58864,#58865,#58866,#58867,#58868,#58869,
#58870,#58871,#58872,#58873,#58874,#58875,#58876,#58877,#58878,#58879,#58880,
#58881,#58882,#58883,#58884,#58885,#58886,#58887,#58888,#58889,#58890,#58891,
#58892,#58893,#58894,#58895,#58896,#58897,#58898,#58899,#58900,#58901,#58902,
#58903,#58904,#58905,#58906,#58907,#58908,#58909,#58910,#58911,#58912,#58913,
#58914,#58915,#58916,#58917,#58918,#58919,#58920,#58921,#58922,#58923,#58924,
#58925,#58926,#58927,#58928,#58929,#58930,#58931,#58932,#58933,#58934,#58935,
#58936,#58937,#58938,#58939,#58940,#58941,#58942,#58943,#58944,#58945,#58946,
#58947,#58948,#58949,#58950,#58951,#58952,#58953,#58954,#58955,#58956,#58957,
#58958,#58959,#58960,#58961,#58962,#58963,#58964,#58965,#58966,#58967,#58968,
#58969,#58970,#58971,#58972,#58973,#58974,#58975,#58976,#58977,#58978,#58979,
#58980,#58981,#58982,#58983,#58984,#58985,#58986),.UNSPECIFIED.,.F.,.F.,
(4,3,3,3,3,3,3,3,3,3,3,3,3,3,3,3,3,3,3,3,3,3,3,3,3,3,3,3,3,3,3,3,3,3,3,
3,3,3,3,3,3,3,3,3,3,3,3,3,3,3,3,3,3,3,3,3,3,3,3,3,3,3,3,3,3,3,4),(14.22949621209,
14.3389432582009,14.4483351528519,14.5577125976453,14.667195473431,14.7767304367527,
14.8864720704545,14.9748740343502,14.9749281643426,15.0752587140259,15.0846377010481,
15.1957150769961,15.3051216647848,15.4144613718424,15.5237750249548,15.6361454458741,
15.7456006442242,15.8594286764281,15.9579689742753,15.9732012351861,15.9732567086321,
16.0738013897155,16.0831958125145,16.1942444925654,16.303882218346,16.4134530400326,
16.5229974342433,16.6351443889129,16.7448268782272,16.8582060655744,16.956883871392,
16.9715256642228,16.9715852529216,17.0721632484324,17.0813057177578,17.1923817276894,
17.3018080824215,17.4111708864129,17.5205109949489,17.6328616955145,17.7423517142398,
17.8561327557255,17.954330039963,17.9698503625424,17.9699137972111,18.0695590982029,
18.0792721224164,18.190393399802,18.2994406760192,18.4084191124463,18.5173701848731,
18.63008822403,18.7391821149852,18.8537122282429,18.9524215317913,18.9682084403491,
18.9682423415007,19.0701286333108,19.0803840166759,19.1922879973418,19.304053299737,
19.4157152161891,19.5273088990212,19.6389125354701,19.7505118772813,19.8622220689861,
19.96657088579),.UNSPECIFIED.) ;
#1369=B_SPLINE_CURVE_WITH_KNOTS('',3,(#58988,#58989,#58990,#58991,#58992,
#58993,#58994,#58995,#58996,#58997,#58998,#58999,#59000,#59001,#59002,#59003,
#59004,#59005,#59006,#59007,#59008,#59009,#59010,#59011,#59012,#59013,#59014,
#59015,#59016,#59017,#59018,#59019,#59020,#59021,#59022,#59023,#59024,#59025,
#59026,#59027,#59028,#59029,#59030,#59031,#59032,#59033,#59034,#59035,#59036,
#59037,#59038,#59039,#59040,#59041,#59042,#59043,#59044,#59045,#59046,#59047,
#59048,#59049,#59050,#59051,#59052,#59053,#59054,#59055,#59056,#59057,#59058,
#59059,#59060,#59061,#59062,#59063,#59064,#59065,#59066,#59067,#59068,#59069,
#59070,#59071,#59072,#59073,#59074,#59075,#59076,#59077,#59078,#59079,#59080,
#59081,#59082,#59083,#59084,#59085,#59086,#59087,#59088,#59089,#59090,#59091),
 .UNSPECIFIED.,.F.,.F.,(4,2,2,2,2,2,2,2,2,2,2,2,2,2,2,2,2,2,2,2,2,2,2,2,
2,2,2,2,2,2,2,2,2,2,2,2,2,2,2,2,2,2,2,2,2,2,2,2,2,2,2,4),(1.10915693870482,
1.11653647298846,1.13777455317558,1.16937210321511,1.18625815048209,1.19532910777744,
1.20809347272472,1.22642008117511,1.2632474552953,1.2787409213987,1.29613448763331,
1.3167350062781,1.35097542441865,1.36058555646715,1.37165177568789,1.40326323007923,
1.43132946312879,1.4464905459374,1.46436978353603,1.48613741210746,1.51879622492545,
1.52812939115584,1.53983435924038,1.55563078244551,1.59670910640585,1.61225905008095,
1.62951253261758,1.64978938441473,1.68506412274503,1.69457193167923,1.70588981021872,
1.72083164811916,1.76605846754896,1.78123805415975,1.79986981076746,1.84852087613937,
1.85935080091146,1.86906430813207,1.88073228386662,1.90893636218579,1.93356771082283,
1.94862623505778,1.96747335279999,2.00244608157891,2.01999222969602,2.02924579125722,
2.04132595857289,2.05794208021421,2.0989728229684,2.11432310360108,2.13270315491108,
2.15940621679325),.UNSPECIFIED.) ;
#1370=B_SPLINE_CURVE_WITH_KNOTS('',3,(#59097,#59098,#59099,#59100,#59101,
#59102,#59103,#59104,#59105,#59106),.UNSPECIFIED.,.F.,.F.,(4,2,2,2,4),(0.000104928857968991,
0.0136473364548126,0.0227277261700891,0.0321175737869646,0.0589236362380934),
 .UNSPECIFIED.) ;
#1371=B_SPLINE_CURVE_WITH_KNOTS('',3,(#59108,#59109,#59110,#59111,#59112,
#59113,#59114,#59115,#59116,#59117,#59118,#59119,#59120,#59121,#59122,#59123,
#59124,#59125,#59126,#59127,#59128,#59129,#59130,#59131,#59132,#59133,#59134,
#59135,#59136,#59137,#59138,#59139,#59140,#59141,#59142,#59143,#59144,#59145,
#59146,#59147,#59148,#59149,#59150,#59151,#59152,#59153,#59154,#59155,#59156,
#59157,#59158,#59159,#59160,#59161,#59162,#59163,#59164,#59165,#59166,#59167,
#59168,#59169,#59170,#59171,#59172,#59173,#59174,#59175,#59176,#59177,#59178,
#59179,#59180,#59181,#59182,#59183,#59184,#59185,#59186,#59187,#59188,#59189,
#59190,#59191,#59192,#59193,#59194,#59195,#59196,#59197,#59198,#59199,#59200,
#59201,#59202,#59203,#59204,#59205,#59206,#59207,#59208,#59209,#59210,#59211,
#59212,#59213,#59214,#59215,#59216,#59217,#59218,#59219,#59220,#59221,#59222,
#59223,#59224,#59225,#59226,#59227,#59228,#59229,#59230,#59231,#59232,#59233,
#59234,#59235,#59236,#59237),.UNSPECIFIED.,.F.,.F.,(4,3,3,3,3,3,3,3,3,3,
3,3,3,3,3,3,3,3,3,3,3,3,3,3,3,3,3,3,3,3,3,3,3,3,3,3,3,3,3,3,3,3,3,4),(-3.84638257219504,
-3.73820936453911,-3.63015334337089,-3.52217201520158,-3.41422262837725,
-3.30618624416936,-3.19810961675877,-3.0898327132607,-2.99504522064809,
-2.99498563286853,-2.8944076385451,-2.88526517210916,-2.77418916166789,
-2.664762811029,-2.55540001113266,-2.44605990669266,-2.33370920216425,-2.22421918751735,
-2.11043813804818,-2.01224085665499,-1.99672052263736,-1.99665708857902,
-1.89701178895675,-1.88729877268755,-1.7761774941378,-1.66713022650311,
-1.55815179836512,-1.44920073392293,-1.33648268651457,-1.22738880270019,
-1.11285867349485,-1.01414938328435,-0.998362445800008,-0.99832854428951,
-0.896442255853368,-0.886186853182638,-0.774282856892657,-0.662517539088778,
-0.550855607479958,-0.439261909779892,-0.32765825904241,-0.216058903257302,
-0.10434869827575,0.),.UNSPECIFIED.) ;
#1372=B_SPLINE_CURVE_WITH_KNOTS('',3,(#59241,#59242,#59243,#59244,#59245,
#59246,#59247,#59248,#59249,#59250,#59251,#59252,#59253,#59254,#59255,#59256,
#59257,#59258,#59259,#59260,#59261,#59262,#59263,#59264,#59265,#59266,#59267,
#59268,#59269,#59270,#59271,#59272,#59273,#59274,#59275,#59276,#59277,#59278,
#59279,#59280,#59281,#59282,#59283,#59284,#59285,#59286,#59287,#59288,#59289,
#59290,#59291,#59292,#59293,#59294,#59295,#59296,#59297,#59298,#59299,#59300,
#59301,#59302,#59303,#59304,#59305,#59306,#59307,#59308,#59309,#59310,#59311,
#59312,#59313,#59314,#59315,#59316,#59317,#59318,#59319,#59320,#59321,#59322,
#59323,#59324,#59325,#59326,#59327,#59328,#59329,#59330,#59331,#59332,#59333,
#59334,#59335,#59336,#59337,#59338,#59339,#59340,#59341,#59342,#59343,#59344,
#59345,#59346,#59347,#59348,#59349,#59350,#59351,#59352,#59353,#59354,#59355,
#59356,#59357,#59358,#59359,#59360,#59361,#59362,#59363,#59364,#59365,#59366,
#59367,#59368,#59369,#59370,#59371,#59372,#59373,#59374,#59375,#59376,#59377,
#59378,#59379,#59380,#59381,#59382,#59383,#59384,#59385,#59386,#59387,#59388,
#59389,#59390,#59391,#59392,#59393,#59394,#59395,#59396,#59397,#59398,#59399,
#59400,#59401,#59402,#59403,#59404,#59405,#59406,#59407,#59408,#59409,#59410,
#59411,#59412,#59413,#59414,#59415,#59416,#59417,#59418,#59419,#59420,#59421,
#59422,#59423,#59424,#59425,#59426,#59427,#59428,#59429,#59430,#59431,#59432,
#59433,#59434,#59435,#59436,#59437,#59438,#59439),.UNSPECIFIED.,.F.,.F.,
(4,3,3,3,3,3,3,3,3,3,3,3,3,3,3,3,3,3,3,3,3,3,3,3,3,3,3,3,3,3,3,3,3,3,3,
3,3,3,3,3,3,3,3,3,3,3,3,3,3,3,3,3,3,3,3,3,3,3,3,3,3,3,3,3,3,3,4),(2.02841987206312,
2.12402082864211,2.23322562754713,2.34231909534285,2.45134273885873,2.56033796740028,
2.66942500876404,2.77855302002171,2.88788829258475,2.98613592948803,2.99492589447402,
2.99498563286853,3.0955586975681,3.1049217827746,3.21597083207253,3.32560733508656,
3.43517758256086,3.5447220500906,3.65687008185746,3.766554239541,3.87993420834952,
3.97858502075132,3.99325851352659,3.99331417715804,4.09371948668603,4.10302842613273,
4.21410521304708,4.32351375319195,4.43285438022156,4.54216792256757,4.65453662228756,
4.76398916469203,4.87781594306978,4.97628270692179,4.99158860021678,4.99164272144754,
5.09203017823468,5.10141729746262,5.21248654349692,5.32195772755063,5.4313616833961,
5.5407391310821,5.65304716474584,5.76256428251417,5.87626777412561,5.97482429279774,
5.98991773692861,5.98997126573705,6.09040640986076,6.09976771772371,6.21083422926157,
6.32032855031362,6.42975605635821,6.53915743408588,6.65144302807105,6.76098476827248,
6.87464228914952,6.97319316334142,6.98824588229396,6.98829981002656,7.08940628246248,
7.09951488574536,7.21054389577484,7.32140236885079,7.4321611881387,7.54286270613221,
7.59300756235356),.UNSPECIFIED.) ;
#1373=B_SPLINE_CURVE_WITH_KNOTS('',3,(#59440,#59441,#59442,#59443,#59444,
#59445,#59446,#59447),.UNSPECIFIED.,.F.,.F.,(4,2,2,4),(-1.10892742733099,
-1.0870101516285,-1.05545170465039,-1.05009718249423),.UNSPECIFIED.) ;
#1374=B_SPLINE_CURVE_WITH_KNOTS('',3,(#59454,#59455,#59456,#59457,#59458,
#59459,#59460,#59461,#59462,#59463,#59464,#59465,#59466,#59467,#59468,#59469,
#59470,#59471,#59472,#59473,#59474,#59475,#59476,#59477,#59478,#59479,#59480,
#59481,#59482,#59483,#59484,#59485,#59486,#59487,#59488,#59489,#59490,#59491,
#59492,#59493,#59494,#59495,#59496),.UNSPECIFIED.,.F.,.F.,(4,3,3,3,3,3,
3,3,3,3,3,3,3,3,4),(-17.9378810482228,-17.8425422594294,-17.7333287470564,
-17.6242265167285,-17.5151940640977,-17.4061899822639,-17.297094050263,
-17.1879571133028,-17.0786129340523,-16.9803667380989,-16.9716468941508,
-16.971585252919,-16.8695608459483,-16.8587004832189,-16.7648812846952),
 .UNSPECIFIED.) ;
#1375=B_SPLINE_CURVE_WITH_KNOTS('',3,(#59502,#59503,#59504,#59505,#59506,
#59507,#59508,#59509,#59510,#59511,#59512,#59513,#59514,#59515,#59516,#59517,
#59518,#59519,#59520,#59521,#59522,#59523,#59524,#59525,#59526,#59527,#59528,
#59529,#59530,#59531,#59532,#59533,#59534,#59535,#59536,#59537,#59538,#59539,
#59540,#59541,#59542,#59543,#59544,#59545,#59546,#59547,#59548,#59549,#59550,
#59551,#59552,#59553,#59554,#59555,#59556,#59557,#59558,#59559,#59560,#59561,
#59562,#59563,#59564,#59565,#59566,#59567,#59568,#59569,#59570,#59571,#59572,
#59573,#59574,#59575,#59576,#59577,#59578,#59579,#59580,#59581,#59582,#59583,
#59584,#59585,#59586,#59587,#59588,#59589,#59590,#59591,#59592,#59593,#59594,
#59595,#59596,#59597,#59598,#59599,#59600,#59601,#59602,#59603,#59604,#59605,
#59606,#59607,#59608,#59609,#59610,#59611,#59612,#59613,#59614,#59615,#59616,
#59617,#59618,#59619,#59620,#59621,#59622,#59623,#59624,#59625,#59626,#59627,
#59628,#59629,#59630,#59631,#59632,#59633,#59634,#59635,#59636,#59637,#59638,
#59639,#59640,#59641,#59642,#59643,#59644,#59645,#59646,#59647,#59648,#59649,
#59650,#59651,#59652,#59653,#59654,#59655,#59656,#59657,#59658,#59659,#59660,
#59661,#59662,#59663,#59664,#59665,#59666,#59667,#59668,#59669,#59670,#59671,
#59672,#59673,#59674,#59675,#59676,#59677,#59678,#59679,#59680,#59681,#59682,
#59683,#59684,#59685,#59686,#59687,#59688,#59689,#59690,#59691,#59692,#59693,
#59694,#59695,#59696,#59697,#59698,#59699,#59700),.UNSPECIFIED.,.F.,.F.,
(4,3,3,3,3,3,3,3,3,3,3,3,3,3,3,3,3,3,3,3,3,3,3,3,3,3,3,3,3,3,3,3,3,3,3,
3,3,3,3,3,3,3,3,3,3,3,3,3,3,3,3,3,3,3,3,3,3,3,3,3,3,3,3,3,3,3,4),(14.2294786280813,
14.338922276967,14.4483107497908,14.557684750591,14.6671641680892,14.7766956576339,
14.8864338346194,14.9748737539835,14.9749281643402,15.0752589866694,15.0846352575163,
15.1957129389055,15.3051173769189,15.4144550482415,15.523766781667,15.6361392634077,
15.7455928462855,15.8594247774576,15.9579634795709,15.9732001976188,15.9732567086296,
16.0738077652168,16.0831978427548,16.1942462690253,16.3038866797998,16.413460431536,
16.5230080020905,16.6351523147976,16.7448385841499,16.8582119185344,16.9568858525924,
16.9715237741764,16.9715852529189,17.0721657571332,17.081314571444,17.1923894746645,
17.3018246639043,17.4111962855185,17.5205451920549,17.6328873433433,17.7423860660186,
17.8561499316134,17.9543534474692,17.9698491292093,17.9699137972083,18.0695608481754,
18.079289201519,18.1904083440163,18.2994712242243,18.4084646767039,18.5174301563394,
18.630133202629,18.7392398295538,18.8537410855257,18.9524757897826,18.9682091601267,
18.9682423414976,19.0701355316434,19.0803531665545,19.1922269279062,19.3039624488416,
19.4155950912131,19.5271600776355,19.6387361661106,19.7503085835541,19.8619932217595,
19.9665708857868),.UNSPECIFIED.) ;
#1376=B_SPLINE_CURVE_WITH_KNOTS('',3,(#59702,#59703,#59704,#59705,#59706,
#59707,#59708,#59709,#59710,#59711,#59712,#59713,#59714,#59715,#59716,#59717,
#59718,#59719,#59720,#59721,#59722,#59723,#59724,#59725,#59726,#59727,#59728,
#59729,#59730,#59731,#59732,#59733,#59734,#59735,#59736,#59737,#59738,#59739,
#59740,#59741,#59742,#59743,#59744,#59745,#59746,#59747,#59748,#59749,#59750,
#59751,#59752,#59753,#59754,#59755,#59756,#59757,#59758,#59759,#59760,#59761,
#59762,#59763,#59764,#59765,#59766,#59767,#59768,#59769,#59770,#59771,#59772,
#59773,#59774,#59775,#59776,#59777,#59778,#59779,#59780,#59781,#59782,#59783,
#59784,#59785,#59786,#59787,#59788,#59789,#59790,#59791,#59792,#59793,#59794,
#59795,#59796,#59797,#59798,#59799,#59800,#59801,#59802,#59803,#59804,#59805),
 .UNSPECIFIED.,.F.,.F.,(4,2,2,2,2,2,2,2,2,2,2,2,2,2,2,2,2,2,2,2,2,2,2,2,
2,2,2,2,2,2,2,2,2,2,2,2,2,2,2,2,2,2,2,2,2,2,2,2,2,2,2,4),(1.10923445814272,
1.11666497858643,1.13797140915878,1.16980477676763,1.18649199766935,1.19554160045309,
1.20846695437517,1.22720172171421,1.26307764714478,1.27862260987191,1.29590862498156,
1.31625148391788,1.35136039511481,1.36088547756677,1.37213003076759,1.40426460938443,
1.4315528060664,1.44670778896382,1.46465320683135,1.48657603571803,1.51881468477099,
1.52817783896307,1.53981594437058,1.55546005225205,1.59701085189892,1.61253832989724,
1.6298665872769,1.65031352546849,1.68502329566247,1.69459082162201,1.70580180457738,
1.73773773559284,1.76517201833841,1.7803173091195,1.79823685726372,1.82009585491647,
1.85259182246046,1.86193134040701,1.87355251831195,1.88917171818081,1.93059177790007,
1.94603630598094,1.96317990033113,1.98326148971095,2.0194272706928,2.02885251398158,
2.04043217677661,2.05590113240821,2.09758105669224,2.11313303528988,2.13078190515427,
2.15945489884343),.UNSPECIFIED.) ;
#1377=B_SPLINE_CURVE_WITH_KNOTS('',3,(#59811,#59812,#59813,#59814,#59815,
#59816,#59817,#59818,#59819,#59820),.UNSPECIFIED.,.F.,.F.,(4,2,2,2,4),(0.000105664403462806,
0.013888256199573,0.0231378033575992,0.0327082927549276,0.0589309959070275),
 .UNSPECIFIED.) ;
#1378=B_SPLINE_CURVE_WITH_KNOTS('',3,(#59822,#59823,#59824,#59825,#59826,
#59827,#59828,#59829,#59830,#59831,#59832,#59833,#59834,#59835,#59836,#59837,
#59838,#59839,#59840,#59841,#59842,#59843,#59844,#59845,#59846,#59847,#59848,
#59849,#59850,#59851,#59852,#59853,#59854,#59855,#59856,#59857,#59858,#59859,
#59860,#59861,#59862,#59863,#59864,#59865,#59866,#59867,#59868,#59869,#59870,
#59871,#59872,#59873,#59874,#59875,#59876,#59877,#59878,#59879,#59880,#59881,
#59882,#59883,#59884,#59885,#59886,#59887,#59888,#59889,#59890,#59891,#59892,
#59893,#59894,#59895,#59896,#59897,#59898,#59899,#59900,#59901,#59902,#59903,
#59904,#59905,#59906,#59907,#59908,#59909,#59910,#59911,#59912,#59913,#59914,
#59915,#59916,#59917,#59918,#59919,#59920,#59921,#59922,#59923,#59924,#59925,
#59926,#59927,#59928,#59929,#59930,#59931,#59932,#59933,#59934,#59935,#59936,
#59937,#59938,#59939,#59940,#59941,#59942,#59943,#59944,#59945,#59946,#59947,
#59948,#59949,#59950,#59951),.UNSPECIFIED.,.F.,.F.,(4,3,3,3,3,3,3,3,3,3,
3,3,3,3,3,3,3,3,3,3,3,3,3,3,3,3,3,3,3,3,3,3,3,3,3,3,3,3,3,3,3,3,3,4),(-3.84638255648223,
-3.7382056031972,-3.63014560658662,-3.52216007910798,-3.41420626916828,
-3.30616512394713,-3.19808354221321,-3.08980139966837,-2.99504711079657,
-2.99498563286806,-2.89440512981233,-2.88525631822079,-2.77418141451553,
-2.66474622912418,-2.55537461134289,-2.44602570862247,-2.33368355361152,
-2.22418483468985,-2.11042096163427,-2.0122174484571,-1.99672175606977,
-1.9966570885787,-1.89701003804244,-1.88728169061728,-1.77616254732629,
-1.66709967286179,-1.55810622588554,-1.44914075150563,-1.33643769970156,
-1.22733107735769,-1.11282981082352,-1.01409511633373,-0.998361725954698,
-0.998328544289352,-0.89643535725085,-0.886217707062147,-0.774343933803599,
-0.662608401142561,-0.550975747253691,-0.439410749549519,-0.327834650256548,
-0.216262222247108,-0.104577574025189,0.),.UNSPECIFIED.) ;
#1379=B_SPLINE_CURVE_WITH_KNOTS('',3,(#59955,#59956,#59957,#59958,#59959,
#59960,#59961,#59962,#59963,#59964,#59965,#59966,#59967,#59968,#59969,#59970,
#59971,#59972,#59973,#59974,#59975,#59976,#59977,#59978,#59979,#59980,#59981,
#59982,#59983,#59984,#59985,#59986,#59987,#59988,#59989,#59990,#59991,#59992,
#59993,#59994,#59995,#59996,#59997,#59998,#59999,#60000,#60001,#60002,#60003,
#60004,#60005,#60006,#60007,#60008,#60009,#60010,#60011,#60012,#60013,#60014,
#60015,#60016,#60017,#60018,#60019,#60020,#60021,#60022,#60023,#60024,#60025,
#60026,#60027,#60028,#60029,#60030,#60031,#60032,#60033,#60034,#60035,#60036,
#60037,#60038,#60039,#60040,#60041,#60042,#60043,#60044,#60045,#60046,#60047,
#60048,#60049,#60050,#60051,#60052,#60053,#60054,#60055,#60056,#60057,#60058,
#60059,#60060,#60061,#60062,#60063,#60064,#60065,#60066,#60067,#60068,#60069,
#60070,#60071,#60072,#60073,#60074,#60075,#60076,#60077,#60078,#60079,#60080,
#60081,#60082,#60083,#60084,#60085,#60086,#60087,#60088,#60089,#60090,#60091,
#60092,#60093,#60094,#60095,#60096,#60097,#60098,#60099,#60100,#60101,#60102,
#60103,#60104,#60105,#60106,#60107,#60108,#60109,#60110,#60111,#60112,#60113,
#60114,#60115,#60116,#60117,#60118,#60119,#60120,#60121,#60122,#60123,#60124,
#60125,#60126,#60127,#60128,#60129,#60130,#60131,#60132,#60133,#60134,#60135,
#60136,#60137,#60138,#60139,#60140,#60141,#60142,#60143,#60144,#60145,#60146,
#60147,#60148,#60149,#60150,#60151,#60152,#60153),.UNSPECIFIED.,.F.,.F.,
(4,3,3,3,3,3,3,3,3,3,3,3,3,3,3,3,3,3,3,3,3,3,3,3,3,3,3,3,3,3,3,3,3,3,3,
3,3,3,3,3,3,3,3,3,3,3,3,3,3,3,3,3,3,3,3,3,3,3,3,3,3,3,3,3,3,3,4),(2.02868994874317,
2.12402862965265,2.23324214578185,2.34234437989576,2.4513768363412,2.56038092201705,
2.66947685788854,2.77861379874124,2.88795798188678,2.98620417724028,2.99492399082981,
2.99498563286805,3.09555617348582,3.10492603756324,3.21597455501251,3.32561466385153,
3.43518827380549,3.54473586247821,3.65688044114801,3.76656712248518,3.87994064982129,
3.97859723168738,3.99325743938423,3.9933141771574,4.09371803583068,4.10302707563617,
4.21410403136249,4.32351087460842,4.43284967933567,4.54216127636544,4.65453163763577,
4.76398194856462,4.87781233500568,4.97627975308706,4.99158830482236,4.99164272144675,
5.09202871645766,5.1014138513281,5.2124835281291,5.32195126426091,5.431351777065,
5.54072578898615,5.65303715817364,5.76255088203706,5.87626107388658,5.9748151813961,
5.98991759903774,5.9899712657361,6.09040611229201,6.09976683700301,6.21083345863081,
6.32032703737286,6.42975385265224,6.5391545904993,6.65144089538084,6.76098212066125,
6.87464096534335,6.97319091957135,6.98824558193009,6.98829981002545,7.089406779752,
7.09951545927819,7.21054508021919,7.32140421541049,7.43216372563492,7.54286597301087,
7.593007562351),.UNSPECIFIED.) ;
#1380=B_SPLINE_CURVE_WITH_KNOTS('',3,(#60154,#60155,#60156,#60157,#60158,
#60159,#60160,#60161),.UNSPECIFIED.,.F.,.F.,(4,2,2,4),(-1.10884682316275,
-1.08689503526884,-1.05534897114704,-1.05003214208722),.UNSPECIFIED.) ;
#1381=B_SPLINE_CURVE_WITH_KNOTS('',3,(#60163,#60164,#60165,#60166,#60167,
#60168,#60169,#60170,#60171,#60172,#60173,#60174,#60175,#60176,#60177,#60178,
#60179,#60180,#60181,#60182,#60183,#60184,#60185,#60186,#60187,#60188,#60189,
#60190,#60191,#60192,#60193,#60194,#60195,#60196,#60197,#60198,#60199,#60200,
#60201,#60202,#60203,#60204,#60205,#60206,#60207,#60208,#60209,#60210,#60211,
#60212,#60213,#60214,#60215,#60216,#60217,#60218,#60219,#60220,#60221,#60222,
#60223,#60224,#60225,#60226,#60227,#60228,#60229,#60230,#60231,#60232,#60233,
#60234,#60235,#60236,#60237,#60238,#60239,#60240,#60241,#60242,#60243,#60244,
#60245,#60246,#60247,#60248,#60249,#60250,#60251,#60252,#60253,#60254,#60255,
#60256,#60257,#60258,#60259,#60260,#60261,#60262,#60263,#60264,#60265,#60266),
 .UNSPECIFIED.,.F.,.F.,(4,2,2,2,2,2,2,2,2,2,2,2,2,2,2,2,2,2,2,2,2,2,2,2,
2,2,2,2,2,2,2,2,2,2,2,2,2,2,2,2,2,2,2,2,2,2,2,2,2,2,2,4),(-1.05003214208722,
-1.04431790606983,-1.03481094545539,-1.00003759698371,-0.979677257209173,
-0.962430901614528,-0.947036722863476,-0.904868645028897,-0.889517257790306,
-0.878029357298292,-0.86871841066293,-0.831920651739553,-0.812142554503174,
-0.795148484116817,-0.779653060990973,-0.739156076372092,-0.723227683493391,
-0.711482092797267,-0.702260210393523,-0.668597701106728,-0.647240311786537,
-0.629569615001816,-0.614483019326602,-0.586107260480668,-0.554586077874824,
-0.543725444409351,-0.534110794360145,-0.522617749546019,-0.495427129208312,
-0.470333279145638,-0.455188297948145,-0.436976322937294,-0.385563849403027,
-0.375618860991466,-0.36523374758677,-0.33385290221376,-0.304245283135888,
-0.289146936842405,-0.271518785459582,-0.250261593351171,-0.21639347451471,
-0.207186878728247,-0.195386560398939,-0.1793331484783,-0.139082756965759,
-0.123556325726735,-0.106601404037852,-0.0869187355250082,-0.0498664571300566,
-0.0405757086686247,-0.0289749179513464,-0.000105736955589282),
 .UNSPECIFIED.) ;
#1382=B_SPLINE_CURVE_WITH_KNOTS('',3,(#60267,#60268,#60269,#60270,#60271,
#60272,#60273,#60274,#60275,#60276,#60277,#60278,#60279,#60280,#60281,#60282,
#60283,#60284,#60285,#60286,#60287,#60288,#60289,#60290,#60291,#60292,#60293,
#60294,#60295,#60296,#60297,#60298,#60299,#60300,#60301,#60302,#60303,#60304,
#60305,#60306,#60307,#60308,#60309,#60310,#60311,#60312,#60313,#60314,#60315,
#60316,#60317,#60318,#60319,#60320,#60321,#60322,#60323,#60324,#60325,#60326,
#60327,#60328,#60329,#60330,#60331,#60332,#60333,#60334,#60335,#60336,#60337,
#60338,#60339,#60340,#60341,#60342,#60343,#60344,#60345,#60346,#60347,#60348,
#60349,#60350,#60351,#60352,#60353,#60354,#60355,#60356,#60357,#60358,#60359,
#60360,#60361,#60362,#60363,#60364,#60365,#60366,#60367,#60368,#60369,#60370),
 .UNSPECIFIED.,.F.,.F.,(4,2,2,2,2,2,2,2,2,2,2,2,2,2,2,2,2,2,2,2,2,2,2,2,
2,2,2,2,2,2,2,2,2,2,2,2,2,2,2,2,2,2,2,2,2,2,2,2,2,2,2,4),(0.0589309959070275,
0.0673105367891647,0.0878341697386557,0.105168713875815,0.120538545156185,
0.163277448753101,0.17845889663062,0.189880980338227,0.199296845798575,
0.235398156440507,0.255440965567746,0.272592461106828,0.288162209074821,
0.328658023811127,0.344638658922391,0.35642349567249,0.365753075913841,
0.398554535466949,0.420249228806342,0.438102775994272,0.453287441577484,
0.482604518844649,0.514080146699166,0.524638787758827,0.534591712082898,
0.586106633858573,0.604383068624081,0.61963489171561,0.664163839882258,
0.679244465726587,0.690625320536653,0.700085867517545,0.735796022663253,
0.755940679691749,0.773141156071703,0.788719090741103,0.829419033780146,
0.845359343849969,0.857128308161983,0.866447839550388,0.899377133437613,
0.921049672023105,0.938896990836141,0.954081508026912,0.984436791901902,
1.0075127403737,1.02196478051473,1.03088118671146,1.04712733482288,1.08003058740821,
1.10162173533867,1.10923445814272),.UNSPECIFIED.) ;
#1383=B_SPLINE_CURVE_WITH_KNOTS('',3,(#60372,#60373,#60374,#60375,#60376,
#60377,#60378,#60379,#60380,#60381,#60382,#60383,#60384,#60385,#60386,#60387,
#60388,#60389,#60390,#60391,#60392,#60393,#60394,#60395,#60396,#60397,#60398,
#60399,#60400,#60401,#60402,#60403,#60404,#60405,#60406,#60407,#60408,#60409,
#60410,#60411,#60412,#60413,#60414,#60415,#60416,#60417,#60418,#60419,#60420,
#60421,#60422,#60423,#60424,#60425,#60426,#60427,#60428,#60429,#60430,#60431,
#60432,#60433,#60434,#60435,#60436,#60437,#60438,#60439,#60440,#60441,#60442,
#60443,#60444,#60445,#60446,#60447,#60448,#60449,#60450,#60451,#60452,#60453,
#60454,#60455,#60456,#60457,#60458,#60459,#60460,#60461,#60462,#60463,#60464,
#60465,#60466,#60467,#60468,#60469,#60470,#60471,#60472,#60473,#60474,#60475,
#60476,#60477),.UNSPECIFIED.,.F.,.F.,(4,2,2,2,2,2,2,2,2,2,2,2,2,2,2,2,2,
2,2,2,2,2,2,2,2,2,2,2,2,2,2,2,2,2,2,2,2,2,2,2,2,2,2,2,2,2,2,2,2,2,2,2,4),
(-1.05009718249423,-1.04440384069162,-1.03490404059468,-1.00003925538964,
-0.979699394704859,-0.9624609922212,-0.947063577815217,-0.90492974045796,
-0.889561950214529,-0.87806598790377,-0.868757119523483,-0.8319166108485,
-0.8121451658037,-0.79515310473938,-0.779655329980471,-0.739161316490995,
-0.723226287841405,-0.711477106871101,-0.702255796851051,-0.668562333963969,
-0.647209575251974,-0.629539800290398,-0.614451716572985,-0.58607026667325,
-0.554543131940902,-0.543680915499547,-0.534066041098232,-0.522573554312757,
-0.495392626353674,-0.470323986373885,-0.455172730104426,-0.436992966401846,
-0.414397046252215,-0.384057785509152,-0.374628212069828,-0.363426593882055,
-0.331397695516476,-0.304073226126729,-0.28900212031638,-0.271284376210517,
-0.249810927369898,-0.216556601359796,-0.207310013978551,-0.195641197707316,
-0.179886111662056,-0.138787884050401,-0.123317797916446,-0.106240021436115,
-0.086275842155076,-0.0502059381847442,-0.0408239803117995,-0.0294675766559434,
-0.000104999262269449),.UNSPECIFIED.) ;
#1384=B_SPLINE_CURVE_WITH_KNOTS('',3,(#60478,#60479,#60480,#60481,#60482,
#60483,#60484,#60485,#60486,#60487,#60488,#60489,#60490,#60491,#60492,#60493,
#60494,#60495,#60496,#60497,#60498,#60499,#60500,#60501,#60502,#60503,#60504,
#60505,#60506,#60507,#60508,#60509,#60510,#60511,#60512,#60513,#60514,#60515,
#60516,#60517,#60518,#60519,#60520,#60521,#60522,#60523,#60524,#60525,#60526,
#60527,#60528,#60529,#60530,#60531,#60532,#60533,#60534,#60535,#60536,#60537,
#60538,#60539,#60540,#60541,#60542,#60543,#60544,#60545,#60546,#60547,#60548,
#60549,#60550,#60551,#60552,#60553,#60554,#60555,#60556,#60557,#60558,#60559,
#60560,#60561,#60562,#60563,#60564,#60565,#60566,#60567,#60568,#60569,#60570,
#60571,#60572,#60573,#60574,#60575,#60576,#60577,#60578,#60579,#60580,#60581,
#60582,#60583),.UNSPECIFIED.,.F.,.F.,(4,2,2,2,2,2,2,2,2,2,2,2,2,2,2,2,2,
2,2,2,2,2,2,2,2,2,2,2,2,2,2,2,2,2,2,2,2,2,2,2,2,2,2,2,2,2,2,2,2,2,2,2,4),
(0.0589236362380934,0.0635158185275896,0.0858196264570916,0.103894607137741,
0.119066674557036,0.163592372683235,0.178616439360702,0.189965040437009,
0.199403587897761,0.230190402340796,0.252671422661968,0.27084276731401,
0.286105385067266,0.327666480543899,0.344180445075028,0.356196540140646,
0.365448975000031,0.391370214599746,0.416825269071937,0.436124283029981,
0.451244414490889,0.475409609913047,0.504250489047926,0.516029893130278,
0.525802523841248,0.536603275814354,0.585229402586121,0.603855483269689,
0.619039288280215,0.664396476118038,0.679334919830258,0.690649514845529,
0.70013435020136,0.735569547448692,0.755790762571726,0.773021648641629,
0.788576830600346,0.829547704455815,0.845389112552175,0.857113299376208,
0.866442959077371,0.899173315808385,0.920911931681626,0.938783952092706,
0.953954915089721,0.982337188402188,1.00677377473397,1.02164504182984,1.03054546711717,
1.04675751171221,1.07985896645351,1.10149884302173,1.10915693870482),
 .UNSPECIFIED.) ;
#1385=B_SPLINE_CURVE_WITH_KNOTS('',3,(#60585,#60586,#60587,#60588,#60589,
#60590,#60591,#60592,#60593,#60594,#60595,#60596,#60597,#60598,#60599,#60600,
#60601,#60602,#60603,#60604,#60605,#60606,#60607,#60608,#60609,#60610,#60611,
#60612,#60613,#60614,#60615,#60616,#60617,#60618,#60619,#60620,#60621,#60622,
#60623,#60624,#60625,#60626,#60627,#60628,#60629,#60630,#60631,#60632,#60633,
#60634,#60635,#60636,#60637,#60638,#60639,#60640,#60641,#60642,#60643,#60644,
#60645,#60646,#60647,#60648,#60649,#60650,#60651,#60652,#60653,#60654,#60655,
#60656,#60657,#60658,#60659,#60660,#60661,#60662,#60663,#60664,#60665,#60666,
#60667,#60668,#60669,#60670,#60671,#60672,#60673,#60674,#60675,#60676,#60677,
#60678,#60679,#60680,#60681,#60682,#60683,#60684,#60685,#60686,#60687,#60688,
#60689,#60690,#60691,#60692,#60693,#60694),.UNSPECIFIED.,.F.,.F.,(4,2,2,
2,2,2,2,2,2,2,2,2,2,2,2,2,2,2,2,2,2,2,2,2,2,2,2,2,2,2,2,2,2,2,2,2,2,2,2,
2,2,2,2,2,2,2,2,2,2,2,2,2,2,2,4),(1.00000006361678E-6,0.0403383732114231,
0.0710490831136922,0.0867357356300736,0.102991445296282,0.153634238618413,
0.171497745854947,0.184581571030169,0.193340939594793,0.207334580300476,
0.248434086191359,0.277268820022062,0.292829275133986,0.309253163863494,
0.358041871857424,0.384682999262059,0.394382470861302,0.404335350906858,
0.444894402162554,0.469642610349295,0.489384110315505,0.50435428197641,
0.524055829842245,0.568418671704122,0.591013749967294,0.600462010919991,
0.610750427743009,0.653783778641295,0.676896139556732,0.695899514262901,
0.710880679088112,0.731418553902633,0.776255216756211,0.797065187062705,
0.806367710856781,0.816895594993979,0.858066414896168,0.881774919635306,
0.901050994782059,0.916022397211022,0.936215694056919,0.980397646718051,
1.00227270642186,1.01166355421563,1.02203884108323,1.06439103413832,1.09744727041259,
1.11340959527833,1.12932874960038,1.16537276803491,1.20613695542018,1.21607213983233,
1.2257852226005,1.2527447650388,1.29362987758487),.UNSPECIFIED.) ;
#1386=B_SPLINE_CURVE_WITH_KNOTS('',3,(#60695,#60696,#60697,#60698,#60699,
#60700,#60701,#60702,#60703,#60704,#60705,#60706,#60707,#60708,#60709,#60710,
#60711,#60712,#60713,#60714,#60715,#60716,#60717,#60718,#60719,#60720,#60721,
#60722,#60723,#60724,#60725,#60726,#60727,#60728,#60729,#60730,#60731,#60732,
#60733,#60734,#60735,#60736,#60737,#60738,#60739,#60740,#60741,#60742,#60743,
#60744,#60745,#60746,#60747,#60748,#60749,#60750,#60751,#60752,#60753,#60754,
#60755,#60756,#60757,#60758,#60759,#60760,#60761,#60762,#60763,#60764,#60765,
#60766,#60767,#60768,#60769,#60770,#60771,#60772,#60773,#60774,#60775,#60776,
#60777,#60778,#60779,#60780,#60781,#60782,#60783,#60784,#60785,#60786,#60787,
#60788,#60789,#60790,#60791,#60792,#60793,#60794,#60795,#60796,#60797,#60798,
#60799,#60800,#60801,#60802,#60803,#60804),.UNSPECIFIED.,.F.,.F.,(4,2,2,
2,2,2,2,2,2,2,2,2,2,2,2,2,2,2,2,2,2,2,2,2,2,2,2,2,2,2,2,2,2,2,2,2,2,2,2,
2,2,2,2,2,2,2,2,2,2,2,2,2,2,2,4),(1.2938343569962,1.29398644728992,1.34783545812506,
1.36349764754707,1.37953598958877,1.41609269887716,1.45505304576164,1.46511091332811,
1.47460836802503,1.49835596884893,1.55374208105197,1.5693454850041,1.58546726978071,
1.60563639211527,1.64628913244785,1.66412627491977,1.67311923424172,1.68413580579912,
1.69783089178063,1.73402395581065,1.76078590541362,1.77612431867759,1.7926753326203,
1.82773843505827,1.86601644822502,1.87612478810658,1.88558195322214,1.90877340853656,
1.95321180938884,1.97248661377819,1.98737303650753,2.00727513183119,2.03247215463915,
2.07178122202493,2.08181336623754,2.09135166230483,2.11568099593797,2.16947189389525,
2.18523202350263,2.2011463073406,2.23690321446718,2.27767661820716,2.28757639189183,
2.29716180922901,2.32248742106138,2.37545195516269,2.39108242253067,2.40695936596739,
2.44285289843246,2.48359334606267,2.49348873341424,2.50318828476119,2.52944381027782,
2.57223691900561,2.5876387803254),.UNSPECIFIED.) ;
#1387=B_SPLINE_CURVE_WITH_KNOTS('',3,(#60806,#60807,#60808,#60809,#60810,
#60811,#60812,#60813,#60814,#60815,#60816,#60817,#60818,#60819,#60820,#60821,
#60822,#60823,#60824,#60825,#60826,#60827,#60828,#60829,#60830,#60831,#60832,
#60833,#60834,#60835,#60836,#60837,#60838,#60839,#60840,#60841,#60842,#60843,
#60844,#60845,#60846,#60847,#60848,#60849,#60850,#60851,#60852,#60853,#60854,
#60855,#60856,#60857,#60858,#60859,#60860,#60861,#60862,#60863,#60864,#60865,
#60866,#60867,#60868,#60869,#60870,#60871,#60872,#60873,#60874,#60875,#60876,
#60877,#60878,#60879,#60880,#60881,#60882,#60883,#60884,#60885,#60886,#60887,
#60888,#60889,#60890,#60891,#60892,#60893,#60894,#60895,#60896,#60897,#60898,
#60899,#60900,#60901,#60902,#60903,#60904,#60905,#60906,#60907,#60908,#60909,
#60910,#60911,#60912,#60913,#60914,#60915),.UNSPECIFIED.,.F.,.F.,(4,2,2,
2,2,2,2,2,2,2,2,2,2,2,2,2,2,2,2,2,2,2,2,2,2,2,2,2,2,2,2,2,2,2,2,2,2,2,2,
2,2,2,2,2,2,2,2,2,2,2,2,2,2,2,4),(9.99999998185342E-7,0.0393714830762708,
0.0614236531788015,0.0799292118101189,0.0949519681806495,0.116270989140045,
0.159883898289276,0.180479303284034,0.189763590677115,0.20033136580239,
0.241164152569101,0.275664123794416,0.291528803690653,0.307548732072641,
0.345030200504205,0.378312653339943,0.390714015177875,0.399512834452093,
0.414445222726917,0.45574206941328,0.483324276412407,0.498802954998541,
0.515405335642074,0.562420894589255,0.581517250452164,0.59514795180082,
0.603903959020001,0.617325670303496,0.658170984699609,0.687970130931299,
0.703599983395622,0.719931630249499,0.76967450999556,0.795778492662367,
0.805454247909864,0.815447969538123,0.855566785240905,0.880484772404275,
0.900301104785482,0.915272635873529,0.934904310459233,0.980299415569464,
1.00221168927269,1.0116075141433,1.02198370292319,1.06434990025255,1.09740580169878,
1.11337285036377,1.12929989543337,1.16547076629152,1.20604506774957,1.2159999821617,
1.22570125360452,1.25238244100321,1.29359361912601),.UNSPECIFIED.) ;
#1388=B_SPLINE_CURVE_WITH_KNOTS('',3,(#60916,#60917,#60918,#60919,#60920,
#60921,#60922,#60923,#60924,#60925,#60926,#60927,#60928,#60929,#60930,#60931,
#60932,#60933,#60934,#60935,#60936,#60937,#60938,#60939,#60940,#60941,#60942,
#60943,#60944,#60945,#60946,#60947,#60948,#60949,#60950,#60951,#60952,#60953,
#60954,#60955,#60956,#60957,#60958,#60959,#60960,#60961,#60962,#60963,#60964,
#60965,#60966,#60967,#60968,#60969,#60970,#60971,#60972,#60973,#60974,#60975,
#60976,#60977,#60978,#60979,#60980,#60981,#60982,#60983,#60984,#60985,#60986,
#60987,#60988,#60989,#60990,#60991,#60992,#60993,#60994,#60995,#60996,#60997,
#60998,#60999,#61000,#61001,#61002,#61003,#61004,#61005,#61006,#61007,#61008,
#61009,#61010,#61011,#61012,#61013,#61014,#61015,#61016,#61017,#61018,#61019,
#61020,#61021,#61022,#61023,#61024,#61025,#61026,#61027,#61028,#61029,#61030,
#61031),.UNSPECIFIED.,.F.,.F.,(4,2,2,2,2,2,2,2,2,2,2,2,2,2,2,2,2,2,2,2,
2,2,2,2,2,2,2,2,2,2,2,2,2,2,2,2,2,2,2,2,2,2,2,2,2,2,2,2,2,2,2,2,2,2,2,2,
2,4),(1.29395065554619,1.29412647113177,1.34795804332071,1.36362730258072,
1.37967165797811,1.41624234391851,1.45520805147782,1.46526976129763,1.47477123977964,
1.49853687016536,1.55392487778237,1.56953545477562,1.5856648617973,1.60584013193459,
1.64652189029532,1.66434295951244,1.6732490038614,1.68420760483371,1.69779163750427,
1.73320528500144,1.76069411255744,1.77609419629443,1.79254509788095,1.81268172166021,
1.8567235700942,1.87156474690353,1.88031423644406,1.8925944261694,1.92580139257715,
1.96350669917209,1.97946235972831,1.99521499737111,2.02843530105521,2.07150917094093,
2.08176608365818,2.09115063374276,2.11331061581725,2.15749481019505,2.17739473887451,
2.1922709953139,2.2115115535979,2.23520582028204,2.27649462642989,2.28698612839726,
2.29618617478099,2.31630502514474,2.35761391596731,2.38024673649518,2.39519879687926,
2.41264245577691,2.43263755004155,2.4737413512898,2.48868791950007,2.49746205768953,
2.50981633664026,2.54328067721221,2.57241596901025,2.58798484160242),
 .UNSPECIFIED.) ;
#1389=B_SPLINE_CURVE_WITH_KNOTS('',3,(#61033,#61034,#61035,#61036,#61037,
#61038,#61039,#61040,#61041,#61042,#61043,#61044,#61045,#61046,#61047,#61048,
#61049,#61050,#61051,#61052,#61053,#61054,#61055,#61056,#61057,#61058,#61059,
#61060,#61061,#61062,#61063,#61064,#61065,#61066,#61067,#61068,#61069,#61070,
#61071,#61072,#61073,#61074,#61075,#61076,#61077,#61078,#61079,#61080,#61081,
#61082,#61083,#61084,#61085,#61086,#61087,#61088,#61089,#61090,#61091,#61092,
#61093,#61094,#61095,#61096,#61097,#61098,#61099,#61100,#61101,#61102,#61103,
#61104,#61105,#61106,#61107,#61108,#61109,#61110,#61111,#61112,#61113,#61114,
#61115,#61116,#61117,#61118,#61119,#61120,#61121,#61122,#61123,#61124,#61125,
#61126,#61127,#61128,#61129,#61130,#61131,#61132,#61133,#61134,#61135,#61136),
 .UNSPECIFIED.,.F.,.F.,(4,2,2,2,2,2,2,2,2,2,2,2,2,2,2,2,2,2,2,2,2,2,2,2,
2,2,2,2,2,2,2,2,2,2,2,2,2,2,2,2,2,2,2,2,2,2,2,2,2,2,2,4),(-1.05001965519088,
-1.04432229220903,-1.03482244015609,-0.999986602611031,-0.979645339017254,
-0.962408079697338,-0.947014267261727,-0.904879744379389,-0.889518808648716,
-0.878026928319333,-0.868719204200551,-0.831896248184208,-0.812126667939335,
-0.795137154664959,-0.77964276881305,-0.739155410492211,-0.72322492607398,
-0.711478769469322,-0.70225896360659,-0.668579624151552,-0.647229501402792,
-0.629562664283716,-0.614477677909573,-0.586102822255114,-0.554582908261496,
-0.543723031213306,-0.53410993118934,-0.522619347725069,-0.49544069022844,
-0.470370427488178,-0.455223536809314,-0.437038830035277,-0.385789447446468,
-0.375756530464295,-0.365474424583251,-0.334289141005716,-0.304256187657895,
-0.289159638986684,-0.27153775255282,-0.250294373321025,-0.216377731948496,
-0.207174965230979,-0.195367424126632,-0.179297432410926,-0.13910749793898,
-0.123578808245063,-0.106631042130916,-0.0869649081841599,-0.0498455866748933,
-0.0405616460688914,-0.0289500608303166,-0.000105196980790777),
 .UNSPECIFIED.) ;
#1390=B_SPLINE_CURVE_WITH_KNOTS('',3,(#61137,#61138,#61139,#61140,#61141,
#61142,#61143,#61144,#61145,#61146,#61147,#61148,#61149,#61150,#61151,#61152,
#61153,#61154,#61155,#61156,#61157,#61158,#61159,#61160,#61161,#61162,#61163,
#61164,#61165,#61166,#61167,#61168,#61169,#61170,#61171,#61172,#61173,#61174,
#61175,#61176,#61177,#61178,#61179,#61180,#61181,#61182,#61183,#61184,#61185,
#61186,#61187,#61188,#61189,#61190,#61191,#61192,#61193,#61194,#61195,#61196,
#61197,#61198,#61199,#61200,#61201,#61202,#61203,#61204,#61205,#61206,#61207,
#61208,#61209,#61210,#61211,#61212,#61213,#61214,#61215,#61216,#61217,#61218,
#61219,#61220,#61221,#61222,#61223,#61224,#61225,#61226,#61227,#61228,#61229,
#61230,#61231,#61232,#61233,#61234,#61235,#61236,#61237,#61238,#61239,#61240,
#61241,#61242),.UNSPECIFIED.,.F.,.F.,(4,2,2,2,2,2,2,2,2,2,2,2,2,2,2,2,2,
2,2,2,2,2,2,2,2,2,2,2,2,2,2,2,2,2,2,2,2,2,2,2,2,2,2,2,2,2,2,2,2,2,2,2,4),
(0.0589148629143721,0.0590186788227545,0.0836761261735466,0.10266362385716,
0.11770045310667,0.142731334957056,0.170798172465959,0.182445136240436,
0.192146244794664,0.202991157601695,0.251571998328379,0.270187004540828,
0.285363261691562,0.330569697155811,0.345527115094681,0.356849783314103,
0.366352722562126,0.401610304980716,0.421865590172558,0.439108591303875,
0.454658352339863,0.495729706689891,0.511539689650347,0.52324851840138,
0.532578071094702,0.565222290830694,0.586966370475972,0.604834760960242,
0.61999608870806,0.648144808479112,0.679759751805539,0.690793721242204,
0.700419500266837,0.734452537107621,0.75509311217183,0.772503489209045,
0.787989107541598,0.830126108597528,0.845565484279735,0.857109903499478,
0.866505825827409,0.898184038219147,0.920310094295822,0.938340224985504,
0.953646219623509,0.98103141025493,1.00622467106084,1.02131892231489,1.03021556836862,
1.04615682168103,1.0795269050592,1.10123582673028,1.10894604130966),
 .UNSPECIFIED.) ;
#1391=B_SPLINE_CURVE_WITH_KNOTS('',3,(#61244,#61245,#61246,#61247,#61248,
#61249,#61250,#61251,#61252,#61253,#61254,#61255,#61256,#61257,#61258,#61259,
#61260,#61261,#61262,#61263,#61264,#61265,#61266,#61267,#61268,#61269,#61270,
#61271,#61272,#61273,#61274,#61275,#61276,#61277,#61278,#61279,#61280,#61281,
#61282,#61283,#61284,#61285,#61286,#61287,#61288,#61289,#61290,#61291,#61292,
#61293,#61294,#61295,#61296,#61297,#61298,#61299,#61300,#61301,#61302,#61303,
#61304,#61305,#61306,#61307,#61308,#61309,#61310,#61311,#61312,#61313,#61314,
#61315,#61316,#61317,#61318,#61319,#61320,#61321,#61322,#61323,#61324,#61325,
#61326,#61327,#61328,#61329,#61330,#61331,#61332,#61333,#61334,#61335,#61336,
#61337,#61338,#61339,#61340,#61341,#61342,#61343,#61344,#61345,#61346,#61347),
 .UNSPECIFIED.,.F.,.F.,(4,2,2,2,2,2,2,2,2,2,2,2,2,2,2,2,2,2,2,2,2,2,2,2,
2,2,2,2,2,2,2,2,2,2,2,2,2,2,2,2,2,2,2,2,2,2,2,2,2,2,2,4),(-1.05003427160778,
-1.04435856196008,-1.03486818366525,-0.999945685105154,-0.979630166743616,
-0.962404972765004,-0.947011042222545,-0.90492026072272,-0.889545514766985,
-0.878047724810931,-0.868744437208028,-0.831882697078646,-0.812124960359172,
-0.795141543650289,-0.779648118856279,-0.739172494515501,-0.723238453872111,
-0.711491071959062,-0.702274075222173,-0.668567244734658,-0.647227292105553,
-0.62956556934539,-0.614482386638978,-0.586107510929279,-0.554588074280767,
-0.543729090856765,-0.534118059507347,-0.522630917087615,-0.495470415892834,
-0.47030772509645,-0.455171105694208,-0.436950734071715,-0.385470085972787,
-0.375561409040591,-0.365137513394907,-0.333740001661664,-0.304258370282471,
-0.289166007387783,-0.271547832939874,-0.250311065427103,-0.216367816106483,
-0.207167837468608,-0.195359300860494,-0.179286661749316,-0.139120348630675,
-0.123592900897117,-0.106648729599607,-0.0869901536427567,-0.0498352677481177,
-0.0405556676512946,-0.0289429427664708,-0.000104312699258312),
 .UNSPECIFIED.) ;
#1392=B_SPLINE_CURVE_WITH_KNOTS('',3,(#61348,#61349,#61350,#61351,#61352,
#61353,#61354,#61355,#61356,#61357,#61358,#61359,#61360,#61361,#61362,#61363,
#61364,#61365,#61366,#61367,#61368,#61369,#61370,#61371,#61372,#61373,#61374,
#61375,#61376,#61377,#61378,#61379,#61380,#61381,#61382,#61383,#61384,#61385,
#61386,#61387,#61388,#61389,#61390,#61391,#61392,#61393,#61394,#61395,#61396,
#61397,#61398,#61399,#61400,#61401,#61402,#61403,#61404,#61405,#61406,#61407,
#61408,#61409,#61410,#61411,#61412,#61413,#61414,#61415,#61416,#61417,#61418,
#61419,#61420,#61421,#61422,#61423,#61424,#61425,#61426,#61427,#61428,#61429,
#61430,#61431,#61432,#61433,#61434,#61435,#61436,#61437,#61438,#61439,#61440,
#61441,#61442,#61443,#61444,#61445,#61446,#61447,#61448,#61449,#61450,#61451,
#61452,#61453),.UNSPECIFIED.,.F.,.F.,(4,2,2,2,2,2,2,2,2,2,2,2,2,2,2,2,2,
2,2,2,2,2,2,2,2,2,2,2,2,2,2,2,2,2,2,2,2,2,2,2,2,2,2,2,2,2,2,2,2,2,2,2,4),
(0.0589262539191868,0.0674589489708446,0.0878852571293232,0.105172489890227,
0.12056093050769,0.163102704451498,0.178378182981949,0.189840085832997,
0.199222968064391,0.230895882994569,0.253023047339911,0.271050725853291,
0.286344983340089,0.313636635725664,0.34571657438274,0.356950670003054,
0.366493554486396,0.40137455207624,0.421753053350218,0.439050689179136,
0.454579718139182,0.496016837231611,0.511704630651829,0.523360210578599,
0.532708319661394,0.565093236046014,0.586944265165279,0.604857738723409,
0.620006820866124,0.647380229141851,0.679455188035899,0.69068762666048,
0.700210850991282,0.735277934835015,0.755613916385321,0.772894683574981,
0.788428618510123,0.829762639212868,0.845484365887109,0.85715598102644,
0.866503864136571,0.898970769041028,0.920811093617175,0.938725579502742,
0.953886202071171,0.981483984745242,1.00652350405074,1.02157450004231,1.03047164643318,
1.04645508624164,1.07979589234157,1.10149951924504,1.10920986980175),
 .UNSPECIFIED.) ;
#1393=B_SPLINE_CURVE_WITH_KNOTS('',3,(#61456,#61457,#61458,#61459,#61460,
#61461,#61462,#61463,#61464,#61465,#61466,#61467,#61468,#61469,#61470,#61471,
#61472,#61473,#61474,#61475,#61476,#61477,#61478,#61479,#61480,#61481,#61482,
#61483,#61484,#61485,#61486,#61487,#61488,#61489,#61490,#61491,#61492,#61493,
#61494,#61495,#61496,#61497,#61498,#61499,#61500,#61501,#61502,#61503,#61504,
#61505,#61506,#61507,#61508,#61509,#61510,#61511,#61512,#61513,#61514,#61515,
#61516,#61517,#61518,#61519,#61520,#61521,#61522,#61523,#61524,#61525,#61526,
#61527,#61528,#61529),.UNSPECIFIED.,.F.,.F.,(4,2,2,2,2,2,2,2,2,2,2,2,2,
2,2,2,2,2,2,2,2,2,2,2,2,2,2,2,2,2,2,2,2,2,2,2,4),(0.458271301746286,0.459696961893322,
0.50071918436547,0.529866039232826,0.545453324099051,0.561854599946403,
0.605115484680842,0.636907063955616,0.646775116783392,0.656555485465506,
0.68508855298933,0.733440945751511,0.749423771495339,0.765306871599009,
0.800337081203133,0.842743224519512,0.852520067962606,0.862384999107365,
0.894120906034862,0.937386088170665,0.953775264351649,0.969360379418854,
0.998517034301751,1.03957160201334,1.05338169136163,1.06213617398809,1.07537553769902,
1.09358430461608,1.1431151311845,1.15945817017287,1.17506808487596,1.2046248561194,
1.24707412640119,1.25983807041739,1.26860932330893,1.2784677893318,1.29350131041376),
 .UNSPECIFIED.) ;
#1394=B_SPLINE_CURVE_WITH_KNOTS('',3,(#61530,#61531,#61532,#61533,#61534,
#61535,#61536,#61537,#61538,#61539,#61540,#61541,#61542,#61543,#61544,#61545,
#61546,#61547,#61548,#61549,#61550,#61551,#61552,#61553,#61554,#61555,#61556,
#61557,#61558,#61559,#61560,#61561,#61562,#61563,#61564,#61565,#61566,#61567,
#61568,#61569),.UNSPECIFIED.,.F.,.F.,(4,2,2,2,2,2,2,2,2,2,2,2,2,2,2,2,2,
2,2,4),(0.00015657270929297,0.0264102910096243,0.0485396520684821,0.0670798630069268,
0.0820848444237249,0.103290341817068,0.14701667650591,0.167626528888988,
0.176910384667272,0.187467114579088,0.228394169883757,0.262867798966582,
0.278730545736736,0.294744744645573,0.342796479572657,0.371534998513901,
0.381323072066321,0.391174076235,0.432782250961712,0.458614805141202),
 .UNSPECIFIED.) ;
#1395=B_SPLINE_CURVE_WITH_KNOTS('',3,(#61570,#61571,#61572,#61573,#61574,
#61575,#61576,#61577,#61578,#61579,#61580,#61581,#61582,#61583,#61584,#61585,
#61586,#61587,#61588,#61589,#61590,#61591,#61592,#61593,#61594,#61595,#61596,
#61597,#61598,#61599,#61600,#61601,#61602,#61603,#61604,#61605,#61606,#61607,
#61608,#61609,#61610,#61611,#61612,#61613,#61614,#61615,#61616,#61617,#61618,
#61619,#61620,#61621,#61622,#61623,#61624,#61625,#61626,#61627,#61628,#61629,
#61630,#61631,#61632,#61633,#61634,#61635,#61636,#61637,#61638,#61639,#61640,
#61641,#61642,#61643,#61644,#61645,#61646,#61647,#61648,#61649,#61650,#61651,
#61652,#61653,#61654,#61655,#61656,#61657,#61658,#61659,#61660,#61661,#61662,
#61663,#61664,#61665,#61666,#61667,#61668,#61669,#61670,#61671,#61672,#61673,
#61674,#61675,#61676,#61677,#61678,#61679,#61680,#61681,#61682,#61683),
 .UNSPECIFIED.,.F.,.F.,(4,2,2,2,2,2,2,2,2,2,2,2,2,2,2,2,2,2,2,2,2,2,2,2,
2,2,2,2,2,2,2,2,2,2,2,2,2,2,2,2,2,2,2,2,2,2,2,2,2,2,2,2,2,2,2,2,4),(1.29372393529934,
1.29389165145828,1.3477247698968,1.36338665343711,1.37942178206577,1.41593890161886,
1.45496340266735,1.46501581980054,1.47451571088236,1.49830469099948,1.55362642680886,
1.56923105143439,1.58534631717237,1.60551642460622,1.64611486918859,1.66400744466805,
1.67300503360996,1.68400464949734,1.69766791991536,1.73364309516177,1.76059251207417,
1.7759435724897,1.79246065053425,1.82718944538032,1.86605176840251,1.87611448862571,
1.88560409335675,1.90924819107751,1.96483131168275,1.9804314858423,1.99656502026702,
2.01673445888671,2.05750711527526,2.07521596593425,2.08411509894518,2.09513299955481,
2.10882816573146,2.14503183083195,2.17171024741712,2.1870413249484,2.20361151984989,
2.23883311592371,2.27693116894822,2.28705230069124,2.2964556708009,2.31912953096445,
2.36344520140104,2.38298311665709,2.39778152172152,2.41710519578955,2.44103323028988,
2.48166690739291,2.49222908946604,2.50146856752791,2.52151851403579,2.574412876524,
2.58747754236347),.UNSPECIFIED.) ;
#1396=B_SPLINE_CURVE_WITH_KNOTS('',3,(#61685,#61686,#61687,#61688,#61689,
#61690,#61691,#61692,#61693,#61694,#61695,#61696,#61697,#61698,#61699,#61700,
#61701,#61702,#61703,#61704,#61705,#61706,#61707,#61708,#61709,#61710,#61711,
#61712,#61713,#61714,#61715,#61716,#61717,#61718,#61719,#61720,#61721,#61722,
#61723,#61724,#61725,#61726,#61727,#61728,#61729,#61730,#61731,#61732,#61733,
#61734,#61735,#61736,#61737,#61738,#61739,#61740,#61741,#61742,#61743,#61744,
#61745,#61746,#61747,#61748,#61749,#61750,#61751,#61752,#61753,#61754,#61755,
#61756,#61757,#61758,#61759,#61760,#61761,#61762,#61763,#61764,#61765,#61766,
#61767,#61768,#61769,#61770,#61771,#61772,#61773,#61774,#61775,#61776,#61777,
#61778,#61779,#61780,#61781,#61782,#61783,#61784,#61785,#61786,#61787,#61788,
#61789,#61790,#61791,#61792,#61793,#61794),.UNSPECIFIED.,.F.,.F.,(4,2,2,
2,2,2,2,2,2,2,2,2,2,2,2,2,2,2,2,2,2,2,2,2,2,2,2,2,2,2,2,2,2,2,2,2,2,2,2,
2,2,2,2,2,2,2,2,2,2,2,2,2,2,2,4),(9.99999998198343E-7,0.0378677308412848,
0.0606088389240463,0.0794397917309287,0.0944374645074597,0.115242832303476,
0.159678588171962,0.180421250368242,0.189717841754718,0.20025712450469,
0.241313725536981,0.275691031872575,0.291548808371455,0.307567579574782,
0.344798028502518,0.378087372069843,0.390600235981472,0.399387436423962,
0.414136507208067,0.455477455001117,0.483241979914481,0.498731328275587,
0.515301196188564,0.562607862053707,0.581599441470349,0.59518414720667,
0.60393825112704,0.617397357754011,0.658262856211241,0.687993752682849,
0.703616937221341,0.719950329799739,0.769651031232493,0.795776575367118,
0.805452368229739,0.815441140145354,0.855603025458804,0.880503336598619,
0.900310866404954,0.915279375543088,0.934909706911577,0.980303960619791,
1.00221521240317,1.01160984773296,1.02198258948594,1.06436558015494,1.09740872360189,
1.11337248517989,1.12929494759968,1.16539062845426,1.20608183630062,1.21602500675469,
1.22573336956587,1.25257572330547,1.29359998411323),.UNSPECIFIED.) ;
#1397=B_SPLINE_CURVE_WITH_KNOTS('',3,(#61795,#61796,#61797,#61798,#61799,
#61800,#61801,#61802,#61803,#61804,#61805,#61806,#61807,#61808,#61809,#61810,
#61811,#61812,#61813,#61814,#61815,#61816,#61817,#61818,#61819,#61820,#61821,
#61822,#61823,#61824,#61825,#61826,#61827,#61828,#61829,#61830,#61831,#61832,
#61833,#61834,#61835,#61836,#61837,#61838,#61839,#61840,#61841,#61842,#61843,
#61844,#61845,#61846,#61847,#61848,#61849,#61850,#61851,#61852,#61853,#61854,
#61855,#61856,#61857,#61858,#61859,#61860,#61861,#61862,#61863,#61864,#61865,
#61866,#61867,#61868,#61869,#61870,#61871,#61872,#61873,#61874,#61875,#61876,
#61877,#61878,#61879,#61880,#61881,#61882,#61883,#61884,#61885,#61886,#61887,
#61888,#61889,#61890,#61891,#61892,#61893,#61894,#61895,#61896,#61897,#61898,
#61899,#61900,#61901,#61902,#61903,#61904,#61905,#61906,#61907,#61908,#61909,
#61910),.UNSPECIFIED.,.F.,.F.,(4,2,2,2,2,2,2,2,2,2,2,2,2,2,2,2,2,2,2,2,
2,2,2,2,2,2,2,2,2,2,2,2,2,2,2,2,2,2,2,2,2,2,2,2,2,2,2,2,2,2,2,2,2,2,2,2,
2,4),(1.29377606271217,1.29392351502004,1.34777604763363,1.36343799978644,
1.37947695175275,1.41604465257822,1.45498511301125,1.46504437813709,1.47454088905445,
1.49827556414381,1.5536800943017,1.56928282945217,1.58540627245887,1.6055747008952,
1.64624343008846,1.66406282706303,1.6729658822995,1.68391911069071,1.69749525559918,
1.73287541645481,1.76036773521383,1.7757621088021,1.79220268332038,1.81232231140674,
1.85626750477301,1.87117857076983,1.87992907867113,1.89215835918365,1.92535646145756,
1.96313340070119,1.97908169110938,1.99483064261501,2.02806592004094,2.07109458732773,
2.08135259644495,2.09072853025411,2.1128140568377,2.15696991938091,2.17691336389267,
2.19178871196546,2.21099013704729,2.23460408242267,2.27607538771201,2.28653736585331,
2.29574252189067,2.31597627275637,2.35788951162614,2.38012594925297,2.39504701479166,
2.41264503530438,2.43295434217051,2.47429677095681,2.48857756112717,2.49731826701906,
2.51009738568464,2.52728843814934,2.57252021960535,2.587449001183),
 .UNSPECIFIED.) ;
#1398=B_SPLINE_CURVE_WITH_KNOTS('',3,(#61912,#61913,#61914,#61915,#61916,
#61917,#61918,#61919,#61920,#61921,#61922,#61923,#61924,#61925,#61926,#61927,
#61928,#61929,#61930,#61931,#61932,#61933,#61934,#61935,#61936,#61937,#61938,
#61939,#61940,#61941,#61942,#61943,#61944,#61945,#61946,#61947,#61948,#61949,
#61950,#61951,#61952,#61953,#61954,#61955,#61956,#61957,#61958,#61959,#61960,
#61961,#61962,#61963,#61964,#61965,#61966,#61967,#61968,#61969,#61970,#61971,
#61972,#61973,#61974,#61975,#61976,#61977,#61978,#61979,#61980,#61981,#61982,
#61983,#61984,#61985,#61986,#61987,#61988,#61989,#61990,#61991,#61992,#61993,
#61994,#61995,#61996,#61997,#61998,#61999,#62000,#62001,#62002,#62003,#62004,
#62005,#62006,#62007,#62008,#62009,#62010,#62011,#62012,#62013,#62014,#62015),
 .UNSPECIFIED.,.F.,.F.,(4,2,2,2,2,2,2,2,2,2,2,2,2,2,2,2,2,2,2,2,2,2,2,2,
2,2,2,2,2,2,2,2,2,2,2,2,2,2,2,2,2,2,2,2,2,2,2,2,2,2,2,4),(-1.05002476366986,
-1.0443211325236,-1.03481859349597,-1.00000617019621,-0.979657693011989,
-0.962416978791812,-0.947023007851114,-0.904875942109422,-0.889518566018222,
-0.87802815988194,-0.868719190779288,-0.831905832730221,-0.812132972524423,
-0.795141696024252,-0.77964689262054,-0.739155899933678,-0.723226180474464,
-0.71148021956807,-0.702259600028155,-0.668586779268195,-0.647233829327134,
-0.629565487276017,-0.614479867209571,-0.586104652776703,-0.554584234200954,
-0.54372403980417,-0.534110324425165,-0.522618767533955,-0.495435388023178,
-0.470356062419595,-0.455209933462259,-0.43701462918738,-0.385701707579139,
-0.375703277640384,-0.365381682155171,-0.334024036953984,-0.30425235752251,
-0.289155087271841,-0.271530862722873,-0.250282382749226,-0.216383491377353,
-0.207179303012565,-0.195374357598536,-0.179310344845435,-0.139098457746932,
-0.123570529204034,-0.106620051208684,-0.0869477113173263,-0.0498534596826706,
-0.040566965275065,-0.0289594292659833,-0.000105410653251608),
 .UNSPECIFIED.) ;
#1399=B_SPLINE_CURVE_WITH_KNOTS('',3,(#62016,#62017,#62018,#62019,#62020,
#62021,#62022,#62023,#62024,#62025,#62026,#62027,#62028,#62029,#62030,#62031,
#62032,#62033,#62034,#62035,#62036,#62037,#62038,#62039,#62040,#62041,#62042,
#62043,#62044,#62045,#62046,#62047,#62048,#62049,#62050,#62051,#62052,#62053,
#62054,#62055,#62056,#62057,#62058,#62059,#62060,#62061,#62062,#62063,#62064,
#62065,#62066,#62067,#62068,#62069,#62070,#62071,#62072,#62073,#62074,#62075,
#62076,#62077,#62078,#62079,#62080,#62081,#62082,#62083,#62084,#62085,#62086,
#62087,#62088,#62089,#62090,#62091,#62092,#62093,#62094,#62095,#62096,#62097,
#62098,#62099,#62100,#62101,#62102,#62103,#62104,#62105,#62106,#62107,#62108,
#62109,#62110,#62111,#62112,#62113,#62114,#62115,#62116,#62117,#62118,#62119,
#62120,#62121),.UNSPECIFIED.,.F.,.F.,(4,2,2,2,2,2,2,2,2,2,2,2,2,2,2,2,2,
2,2,2,2,2,2,2,2,2,2,2,2,2,2,2,2,2,2,2,2,2,2,2,2,2,2,2,2,2,2,2,2,2,2,2,4),
(0.0589297775460328,0.0652894712739869,0.0867420242877471,0.104468805486226,
0.119547855356985,0.146949856125031,0.178893239915403,0.190095662433324,
0.199605936431439,0.234732066332288,0.255055236302571,0.272327573690126,
0.287848119587509,0.329144758396892,0.344849153091511,0.356511468726538,
0.365881017427153,0.398040119826413,0.419969302454997,0.437918608740246,
0.453078159402929,0.480393408602737,0.512533638082787,0.523779103299443,
0.533305107312649,0.568336299464638,0.588669247427223,0.60594654111988,
0.621480015828052,0.664040370741232,0.679135999295418,0.690524147030703,
0.699981851612583,0.735733289664909,0.755870022630079,0.773067461583054,
0.788646363490021,0.829341590851685,0.845286548425108,0.857057941006012,
0.866376791841605,0.899329554935797,0.920997560296477,0.938843512856045,
0.954028607693655,0.984413321031502,1.00747521618607,1.02192342342242,1.03084004932114,
1.04708845541304,1.07999538023816,1.10158853164967,1.10920453594835),
 .UNSPECIFIED.) ;
#1400=B_SPLINE_CURVE_WITH_KNOTS('',3,(#62123,#62124,#62125,#62126,#62127,
#62128,#62129,#62130,#62131,#62132,#62133,#62134,#62135,#62136,#62137,#62138,
#62139,#62140,#62141,#62142,#62143,#62144,#62145,#62146,#62147,#62148,#62149,
#62150,#62151,#62152,#62153,#62154,#62155,#62156,#62157,#62158,#62159,#62160,
#62161,#62162,#62163,#62164,#62165,#62166,#62167,#62168,#62169,#62170,#62171,
#62172,#62173,#62174,#62175,#62176,#62177,#62178,#62179,#62180,#62181,#62182,
#62183,#62184,#62185,#62186,#62187,#62188,#62189,#62190,#62191,#62192,#62193,
#62194,#62195,#62196,#62197,#62198,#62199,#62200,#62201,#62202,#62203,#62204,
#62205,#62206,#62207,#62208,#62209,#62210,#62211,#62212,#62213,#62214,#62215,
#62216,#62217,#62218,#62219,#62220,#62221,#62222,#62223,#62224,#62225,#62226),
 .UNSPECIFIED.,.F.,.F.,(4,2,2,2,2,2,2,2,2,2,2,2,2,2,2,2,2,2,2,2,2,2,2,2,
2,2,2,2,2,2,2,2,2,2,2,2,2,2,2,2,2,2,2,2,2,2,2,2,2,2,2,4),(-1.05003008412879,
-1.04431896404847,-1.03481328881548,-1.00002851916316,-0.979671626744206,
-0.962426905678517,-0.947032780484766,-0.90487086648857,-0.889517720277496,
-0.878029080838536,-0.868718700745103,-0.831916430753326,-0.812139837211625,
-0.795146566431792,-0.779651315447274,-0.739156080255804,-0.723227292799457,
-0.71148158843511,-0.702260063727722,-0.668594613438749,-0.647238488275157,
-0.629568461293717,-0.614482141385646,-0.586106536452459,-0.554585569414328,
-0.543725053222038,-0.534110665469483,-0.522618039398998,-0.495429458990086,
-0.47033973122144,-0.455194435549932,-0.436987176613918,-0.385602805275799,
-0.375642806311598,-0.36527583333481,-0.333901495841986,-0.304247482853878,
-0.289149427153854,-0.271522452069984,-0.250267892143036,-0.216390464090898,
-0.207184587899735,-0.195382843131259,-0.179326169847952,-0.139087503231474,
-0.123560589981618,-0.106606992543605,-0.086927419905541,-0.0498625771347933,
-0.0405730962597217,-0.028970261341665,-0.000105645403308168),
 .UNSPECIFIED.) ;
#1401=B_SPLINE_CURVE_WITH_KNOTS('',3,(#62227,#62228,#62229,#62230,#62231,
#62232,#62233,#62234,#62235,#62236,#62237,#62238,#62239,#62240,#62241,#62242,
#62243,#62244,#62245,#62246,#62247,#62248,#62249,#62250,#62251,#62252,#62253,
#62254,#62255,#62256,#62257,#62258,#62259,#62260,#62261,#62262,#62263,#62264,
#62265,#62266,#62267,#62268,#62269,#62270,#62271,#62272,#62273,#62274,#62275,
#62276,#62277,#62278,#62279,#62280,#62281,#62282,#62283,#62284,#62285,#62286,
#62287,#62288,#62289,#62290,#62291,#62292,#62293,#62294,#62295,#62296,#62297,
#62298,#62299,#62300,#62301,#62302,#62303,#62304,#62305,#62306,#62307,#62308,
#62309,#62310,#62311,#62312,#62313,#62314,#62315,#62316,#62317,#62318,#62319,
#62320,#62321,#62322,#62323,#62324,#62325,#62326,#62327,#62328,#62329,#62330),
 .UNSPECIFIED.,.F.,.F.,(4,2,2,2,2,2,2,2,2,2,2,2,2,2,2,2,2,2,2,2,2,2,2,2,
2,2,2,2,2,2,2,2,2,2,2,2,2,2,2,2,2,2,2,2,2,2,2,2,2,2,2,4),(0.0589305428466179,
0.0672845159977873,0.0878174041535288,0.105155502442307,0.120524223180403,
0.163295642882688,0.178468096249972,0.189885861115552,0.199302354612582,
0.235392943926774,0.255437742804592,0.272590091372826,0.288159982715115,
0.328657569317303,0.344637669732123,0.356422205311361,0.365751083807702,
0.398559148128537,0.420251806610186,0.43810445199171,0.453288864247402,
0.482630270258008,0.514102600365068,0.524650646116702,0.534611151253447,
0.586112101532517,0.604385950945008,0.619637337659203,0.664154967711524,
0.679239299425177,0.69062178060246,0.700081096373092,0.735801621662722,
0.755943121607322,0.77314197730984,0.78871951163143,0.829416287168497,0.845357242850418,
0.857126395520116,0.866445333001415,0.899379873989889,0.921050193673692,
0.938896356258789,0.954080380361352,0.984443454819893,1.00751392957382,
1.02196410313733,1.03088019431753,1.04712650694432,1.08002915852087,1.10161988420202,
1.10923317368641),.UNSPECIFIED.) ;
#1402=B_SPLINE_CURVE_WITH_KNOTS('',3,(#62332,#62333,#62334,#62335,#62336,
#62337,#62338,#62339,#62340,#62341,#62342,#62343,#62344,#62345,#62346,#62347,
#62348,#62349,#62350,#62351,#62352,#62353,#62354,#62355,#62356,#62357,#62358,
#62359,#62360,#62361,#62362,#62363,#62364,#62365,#62366,#62367,#62368,#62369,
#62370,#62371,#62372,#62373,#62374,#62375,#62376,#62377,#62378,#62379,#62380,
#62381,#62382,#62383,#62384,#62385,#62386,#62387,#62388,#62389,#62390,#62391,
#62392,#62393,#62394,#62395,#62396,#62397,#62398,#62399,#62400,#62401,#62402,
#62403,#62404,#62405,#62406,#62407,#62408,#62409,#62410,#62411,#62412,#62413,
#62414,#62415,#62416,#62417,#62418,#62419,#62420,#62421,#62422,#62423,#62424,
#62425,#62426,#62427,#62428,#62429,#62430,#62431,#62432,#62433,#62434,#62435,
#62436,#62437),.UNSPECIFIED.,.F.,.F.,(4,2,2,2,2,2,2,2,2,2,2,2,2,2,2,2,2,
2,2,2,2,2,2,2,2,2,2,2,2,2,2,2,2,2,2,2,2,2,2,2,2,2,2,2,2,2,2,2,2,2,2,2,4),
(-1.05009743737373,-1.0444142954407,-1.03491901187677,-1.00001404596187,
-0.979686405976698,-0.962453803642405,-0.947056484787095,-0.904943448966669,
-0.889569365922612,-0.878070757400633,-0.868764044760531,-0.831905808769755,
-0.812140071074282,-0.79515101259579,-0.779653833199217,-0.739165661846125,
-0.723229129130369,-0.711479489481218,-0.702259576976015,-0.668553609235896,
-0.647205795595896,-0.629538572785096,-0.614451472915272,-0.58607028319706,
-0.55454366833602,-0.543681971177213,-0.534068151231903,-0.522577375586239,
-0.495405157151037,-0.470348621534463,-0.455196052630545,-0.437033285757907,
-0.414478636632468,-0.384038960855417,-0.374615326660911,-0.363403168420454,
-0.331313186786754,-0.304066188094179,-0.288998088171465,-0.27127773942017,
-0.249796997202879,-0.21655996628468,-0.207312682283666,-0.195649433482483,
-0.179906744369181,-0.13877991492888,-0.123312887067026,-0.106230980957928,
-0.0862570340744459,-0.0502170126684645,-0.0408326493672609,-0.0294865495056169,
-0.00010458719840716),.UNSPECIFIED.) ;
#1403=B_SPLINE_CURVE_WITH_KNOTS('',3,(#62438,#62439,#62440,#62441,#62442,
#62443,#62444,#62445,#62446,#62447,#62448,#62449,#62450,#62451,#62452,#62453,
#62454,#62455,#62456,#62457,#62458,#62459,#62460,#62461,#62462,#62463,#62464,
#62465,#62466,#62467,#62468,#62469,#62470,#62471,#62472,#62473,#62474,#62475,
#62476,#62477,#62478,#62479,#62480,#62481,#62482,#62483,#62484,#62485,#62486,
#62487,#62488,#62489,#62490,#62491,#62492,#62493,#62494,#62495,#62496,#62497,
#62498,#62499,#62500,#62501,#62502,#62503,#62504,#62505,#62506,#62507,#62508,
#62509,#62510,#62511,#62512,#62513,#62514,#62515,#62516,#62517,#62518,#62519,
#62520,#62521,#62522,#62523,#62524,#62525,#62526,#62527,#62528,#62529,#62530,
#62531,#62532,#62533,#62534,#62535,#62536,#62537,#62538,#62539,#62540,#62541,
#62542,#62543),.UNSPECIFIED.,.F.,.F.,(4,2,2,2,2,2,2,2,2,2,2,2,2,2,2,2,2,
2,2,2,2,2,2,2,2,2,2,2,2,2,2,2,2,2,2,2,2,2,2,2,2,2,2,2,2,2,2,2,2,2,2,2,4),
(0.0589272293900401,0.067488527546277,0.0879063949391725,0.105190876153072,
0.120580062603249,0.163086583564848,0.178370124455571,0.189836172480497,
0.199220285299566,0.230888475691084,0.253019666091311,0.271049193657553,
0.286342783191366,0.313603294782333,0.34571001824462,0.356949024196235,
0.366491537998796,0.40138208509266,0.421757515981374,0.43905423508961,0.454585623739544,
0.496006631946285,0.511701765732417,0.523360784388823,0.532709138807078,
0.565099812285689,0.586948556420365,0.604861666564845,0.620013213321861,
0.647439325735318,0.679473081914327,0.690698573057144,0.700226682596672,
0.735250884255282,0.75560024473867,0.772887397615669,0.788421292124127,
0.829778469040536,0.845493086314554,0.857161780545748,0.866512173995915,
0.898950068658538,0.920801877962503,0.938721682216242,0.953882995774727,
0.981451106708084,1.00651465352988,1.02157299203097,1.03047098559634,1.04645179889171,
1.0797962414394,1.10150145357039,1.10921089576887),.UNSPECIFIED.) ;
#1404=B_SPLINE_CURVE_WITH_KNOTS('',3,(#62545,#62546,#62547,#62548,#62549,
#62550,#62551,#62552,#62553,#62554,#62555,#62556,#62557,#62558,#62559,#62560,
#62561,#62562,#62563,#62564,#62565,#62566,#62567,#62568,#62569,#62570,#62571,
#62572,#62573,#62574,#62575,#62576,#62577,#62578,#62579,#62580,#62581,#62582,
#62583,#62584,#62585,#62586,#62587,#62588,#62589,#62590,#62591,#62592,#62593,
#62594,#62595,#62596,#62597,#62598,#62599,#62600,#62601,#62602,#62603,#62604,
#62605,#62606,#62607,#62608,#62609,#62610,#62611,#62612,#62613,#62614,#62615,
#62616,#62617,#62618,#62619,#62620,#62621,#62622,#62623,#62624,#62625,#62626,
#62627,#62628,#62629,#62630,#62631,#62632,#62633,#62634,#62635,#62636,#62637,
#62638,#62639,#62640,#62641,#62642,#62643,#62644,#62645,#62646,#62647,#62648,
#62649,#62650),.UNSPECIFIED.,.F.,.F.,(4,2,2,2,2,2,2,2,2,2,2,2,2,2,2,2,2,
2,2,2,2,2,2,2,2,2,2,2,2,2,2,2,2,2,2,2,2,2,2,2,2,2,2,2,2,2,2,2,2,2,2,2,4),
(-1.05009726896819,-1.04440689227039,-1.03490838516155,-1.00003204688939,
-0.979695682343558,-0.962458936406225,-0.947061549754477,-0.904933676652856,
-0.889564086487481,-0.878067365688205,-0.868759104476544,-0.831913581237844,
-0.812143746083211,-0.795152530839052,-0.779654921673552,-0.739162567398497,
-0.723227109103028,-0.711477795798406,-0.702256877846236,-0.668559896246528,
-0.647208528123987,-0.629539470444578,-0.614451662430445,-0.586070287160119,
-0.55454329746179,-0.543681222134124,-0.534066641030603,-0.52257463065588,
-0.495396126215626,-0.470331462097326,-0.455179785820508,-0.43700513146238,
-0.414421650912579,-0.384052129926698,-0.374624326885522,-0.36341951780383,
-0.331372181117148,-0.304071121534662,-0.289000893687606,-0.271282309783265,
-0.249806563201047,-0.216557673856157,-0.207310849350346,-0.195643719865775,
-0.179892400381864,-0.138785413988915,-0.123316229615429,-0.106237128833854,
-0.0862698516545277,-0.0502094735454203,-0.0408267314315204,-0.0294735284731143,
-0.000104884473885925),.UNSPECIFIED.) ;
#1405=B_SPLINE_CURVE_WITH_KNOTS('',3,(#62651,#62652,#62653,#62654,#62655,
#62656,#62657,#62658,#62659,#62660,#62661,#62662,#62663,#62664,#62665,#62666,
#62667,#62668,#62669,#62670,#62671,#62672,#62673,#62674,#62675,#62676,#62677,
#62678,#62679,#62680,#62681,#62682,#62683,#62684,#62685,#62686,#62687,#62688,
#62689,#62690,#62691,#62692,#62693,#62694,#62695,#62696,#62697,#62698,#62699,
#62700,#62701,#62702,#62703,#62704,#62705,#62706,#62707,#62708,#62709,#62710,
#62711,#62712,#62713,#62714,#62715,#62716,#62717,#62718,#62719,#62720,#62721,
#62722,#62723,#62724,#62725,#62726,#62727,#62728,#62729,#62730,#62731,#62732,
#62733,#62734,#62735,#62736,#62737,#62738,#62739,#62740,#62741,#62742,#62743,
#62744,#62745,#62746,#62747,#62748,#62749,#62750,#62751,#62752,#62753,#62754),
 .UNSPECIFIED.,.F.,.F.,(4,2,2,2,2,2,2,2,2,2,2,2,2,2,2,2,2,2,2,2,2,2,2,2,
2,2,2,2,2,2,2,2,2,2,2,2,2,2,2,2,2,2,2,2,2,2,2,2,2,2,2,4),(0.0589549240516137,
0.0851958477970781,0.103550850472164,0.118668784507955,0.163514220667212,
0.178609712524909,0.189990117089629,0.199411350087213,0.235404136686533,
0.2554656216767,0.272623939957196,0.288191317490099,0.328713719397892,0.344681365607318,
0.356459305376491,0.365782713816312,0.390581005212486,0.416498591395869,
0.435959052999002,0.451062007752223,0.475597303193304,0.504307905591082,
0.516065863436386,0.525827296003839,0.536639628375923,0.585236274830679,
0.603855211162292,0.61903599680304,0.664368619002719,0.679310380176029,
0.690625651735391,0.700107017687091,0.735552088727983,0.755764892071041,
0.772990398066607,0.788542736619561,0.829499046965055,0.845339896149365,
0.857062914604454,0.866390041503749,0.899124586325224,0.92085552352727,
0.938722574775654,0.953890511976325,0.982278565287995,1.00670264296543,
1.0215687162022,1.03046723474578,1.04667705716277,1.07977179153917,1.10140738512334,
1.10906469945444),.UNSPECIFIED.) ;
#1406=B_SPLINE_CURVE_WITH_KNOTS('',3,(#62756,#62757,#62758,#62759,#62760,
#62761,#62762,#62763,#62764,#62765,#62766,#62767,#62768,#62769,#62770,#62771,
#62772,#62773,#62774,#62775,#62776,#62777,#62778,#62779,#62780,#62781,#62782,
#62783,#62784,#62785,#62786,#62787,#62788,#62789,#62790,#62791,#62792,#62793,
#62794,#62795,#62796,#62797,#62798,#62799,#62800,#62801,#62802,#62803,#62804,
#62805,#62806,#62807,#62808,#62809,#62810,#62811,#62812,#62813,#62814,#62815,
#62816,#62817,#62818,#62819,#62820,#62821,#62822,#62823,#62824,#62825,#62826,
#62827,#62828,#62829,#62830,#62831,#62832,#62833,#62834,#62835,#62836,#62837,
#62838,#62839,#62840,#62841,#62842,#62843,#62844,#62845,#62846,#62847,#62848,
#62849,#62850,#62851,#62852,#62853,#62854,#62855,#62856,#62857,#62858,#62859,
#62860,#62861,#62862,#62863,#62864,#62865,#62866,#62867),.UNSPECIFIED.,
 .F.,.F.,(4,2,2,2,2,2,2,2,2,2,2,2,2,2,2,2,2,2,2,2,2,2,2,2,2,2,2,2,2,2,2,
2,2,2,2,2,2,2,2,2,2,2,2,2,2,2,2,2,2,2,2,2,2,2,2,4),(9.99999995666184E-7,
0.0356604468915954,0.070133267113053,0.0860029358249983,0.102035258196422,
0.138479242783618,0.172338809078127,0.184971208474476,0.193753965955692,
0.208347154612707,0.249637057802738,0.277597724849303,0.293098631733098,
0.309636799854698,0.357306543037373,0.37618928683413,0.389726264706006,
0.398478041709008,0.411971492751561,0.452852617873533,0.48252321909239,
0.498145991493354,0.514493440612958,0.558427122283655,0.579863109805348,
0.594462050137506,0.603245437648757,0.615877543116213,0.656167568986894,
0.678164181503244,0.696643297064956,0.711660116607348,0.732993373069633,
0.776520196897853,0.797095232053959,0.806378324128922,0.816947486375974,
0.857796463240435,0.881613343056727,0.900939343464071,0.915911945969393,
0.936054711457947,0.980258017814283,1.00220505651952,1.01160250446526,1.02197120600625,
1.06438132506819,1.09740639518348,1.11336964497618,1.12929361424787,1.16544165924478,
1.20604664522996,1.21599727173067,1.22569914880269,1.2524117708616,1.29358094859399),
 .UNSPECIFIED.) ;
#1407=B_SPLINE_CURVE_WITH_KNOTS('',3,(#62868,#62869,#62870,#62871,#62872,
#62873,#62874,#62875,#62876,#62877,#62878,#62879,#62880,#62881,#62882,#62883,
#62884,#62885,#62886,#62887,#62888,#62889,#62890,#62891,#62892,#62893,#62894,
#62895,#62896,#62897,#62898,#62899,#62900,#62901,#62902,#62903,#62904,#62905,
#62906,#62907,#62908,#62909,#62910,#62911,#62912,#62913,#62914,#62915,#62916,
#62917,#62918,#62919,#62920,#62921,#62922,#62923,#62924,#62925,#62926,#62927,
#62928,#62929,#62930,#62931,#62932,#62933,#62934,#62935,#62936,#62937,#62938,
#62939,#62940,#62941,#62942,#62943,#62944,#62945,#62946,#62947,#62948,#62949,
#62950,#62951,#62952,#62953,#62954,#62955,#62956,#62957,#62958,#62959,#62960,
#62961,#62962,#62963,#62964,#62965,#62966,#62967,#62968,#62969,#62970,#62971,
#62972,#62973,#62974,#62975,#62976,#62977,#62978,#62979),.UNSPECIFIED.,
 .F.,.F.,(4,2,2,2,2,2,2,2,2,2,2,2,2,2,2,2,2,2,2,2,2,2,2,2,2,2,2,2,2,2,2,
2,2,2,2,2,2,2,2,2,2,2,2,2,2,2,2,2,2,2,2,2,2,2,2,4),(1.29372477504308,1.29392078486775,
1.34771417135715,1.36337948433266,1.37941702445609,1.41594491724888,1.45495248269729,
1.4650070265992,1.47450844368933,1.49830749219453,1.55361694431632,1.56922485042015,
1.58534467078816,1.60551503339217,1.64613979410088,1.66400243912571,1.67299833222239,
1.68400882395125,1.69769229140463,1.73380226128087,1.76064384945758,1.77598994206369,
1.79253106836518,1.82748552452238,1.86593840949346,1.87603382421201,1.88550173505765,
1.90884295174587,1.953307274162,1.97249844204928,1.9873870874903,2.00738698304974,
2.06018929708678,2.07611514395467,2.08494812909607,2.09669278149997,2.12988195170081,
2.16863710080455,2.18455246760019,2.20030743542534,2.2337567200133,2.27655125126105,
2.28684273706431,2.29614776549758,2.31751585780158,2.36591766411947,2.38439846426727,
2.39922231412712,2.41979440095639,2.45845623747862,2.48257741921665,2.49281856811981,
2.50225778233022,2.52451208356163,2.5734104755075,2.58752750405949),
 .UNSPECIFIED.) ;
#1408=B_SPLINE_CURVE_WITH_KNOTS('',3,(#62982,#62983,#62984,#62985,#62986,
#62987,#62988,#62989,#62990,#62991,#62992,#62993,#62994,#62995,#62996,#62997,
#62998,#62999,#63000,#63001,#63002,#63003,#63004,#63005,#63006,#63007,#63008,
#63009,#63010,#63011,#63012,#63013,#63014,#63015,#63016,#63017,#63018,#63019,
#63020,#63021,#63022,#63023,#63024,#63025,#63026,#63027,#63028,#63029,#63030,
#63031,#63032,#63033,#63034,#63035,#63036,#63037,#63038,#63039,#63040,#63041,
#63042,#63043,#63044,#63045,#63046,#63047,#63048,#63049,#63050,#63051,#63052,
#63053),.UNSPECIFIED.,.F.,.F.,(4,2,2,2,2,2,2,2,2,2,2,2,2,2,2,2,2,2,2,2,
2,2,2,2,2,2,2,2,2,2,2,2,2,2,2,4),(0.458255991027476,0.459769175149047,0.500809246661114,
0.52987537666172,0.54545746136114,0.561868843971101,0.605000429750257,0.636881854988211,
0.646751201848579,0.65653133861299,0.685049665674218,0.733419643225896,
0.749401028417448,0.765287692550303,0.800400729865581,0.842672430761068,
0.852462666429538,0.862314719448503,0.893347021290769,0.937660583205908,
0.953970312708293,0.969607854792279,0.999561963597051,1.04037794907665,
1.05372007222468,1.06247360622918,1.07617407775912,1.0954328549492,1.1449737191145,
1.16086909755882,1.1768498703973,1.21266798211965,1.25342411010337,1.26334590831044,
1.27307733955482,1.29346035014047),.UNSPECIFIED.) ;
#1409=B_SPLINE_CURVE_WITH_KNOTS('',3,(#63054,#63055,#63056,#63057,#63058,
#63059,#63060,#63061,#63062,#63063,#63064,#63065,#63066,#63067,#63068,#63069,
#63070,#63071,#63072,#63073,#63074,#63075,#63076,#63077,#63078,#63079,#63080,
#63081,#63082,#63083,#63084,#63085,#63086,#63087,#63088,#63089,#63090,#63091),
 .UNSPECIFIED.,.F.,.F.,(4,2,2,2,2,2,2,2,2,2,2,2,2,2,2,2,2,2,4),(0.000157521932395551,
0.0468596001704785,0.0661006226859243,0.0810704747273422,0.101297244207578,
0.146666255253819,0.167568294536989,0.176877493818213,0.187388572022809,
0.228675693240133,0.262938074258254,0.278793151198754,0.294817688832346,
0.342740512631854,0.37155204865316,0.38134278249533,0.39119193768519,0.432818454349516,
0.458634629932413),.UNSPECIFIED.) ;
#1410=B_SPLINE_CURVE_WITH_KNOTS('',3,(#63092,#63093,#63094,#63095,#63096,
#63097,#63098,#63099,#63100,#63101,#63102,#63103,#63104,#63105,#63106,#63107,
#63108,#63109,#63110,#63111,#63112,#63113,#63114,#63115,#63116,#63117,#63118,
#63119,#63120,#63121,#63122,#63123,#63124,#63125,#63126,#63127,#63128,#63129,
#63130,#63131,#63132,#63133,#63134,#63135,#63136,#63137,#63138,#63139,#63140,
#63141,#63142,#63143,#63144,#63145,#63146,#63147,#63148,#63149,#63150,#63151,
#63152,#63153,#63154,#63155,#63156,#63157,#63158,#63159,#63160,#63161,#63162,
#63163,#63164,#63165,#63166,#63167,#63168,#63169,#63170,#63171,#63172,#63173,
#63174,#63175,#63176,#63177,#63178,#63179,#63180,#63181,#63182,#63183,#63184,
#63185,#63186,#63187,#63188,#63189,#63190,#63191,#63192,#63193,#63194,#63195,
#63196,#63197,#63198,#63199,#63200,#63201,#63202,#63203,#63204,#63205),
 .UNSPECIFIED.,.F.,.F.,(4,2,2,2,2,2,2,2,2,2,2,2,2,2,2,2,2,2,2,2,2,2,2,2,
2,2,2,2,2,2,2,2,2,2,2,2,2,2,2,2,2,2,2,2,2,2,2,2,2,2,2,2,2,2,2,2,4),(1.29353464663662,
1.29372323750481,1.3475200935386,1.36318078637633,1.3792129271178,1.4157123566257,
1.45474845020589,1.46479785145263,1.47429790587587,1.49810584329248,1.55338296284456,
1.56898695054761,1.58509875748223,1.60526577596705,1.64584584633556,1.66374549430997,
1.67274276260631,1.68373842464409,1.69739536328701,1.73333585412455,1.76030822097165,
1.77565954125108,1.79217111565895,1.82686267755522,1.86576778396304,1.87582498390098,
1.88531655585195,1.90900852615565,1.96450623220877,1.98010753845972,1.99623433804176,
2.01640149277719,2.05712850439889,2.0748684940139,2.083769679733,2.09477725393964,
2.10845413999575,2.14454097979264,2.17131164699336,2.18664689472732,2.20319667803955,
2.23823665944315,2.27663031234181,2.28672721931645,2.29614763773492,2.31905107458434,
2.36339129187136,2.3827724850076,2.39756729629176,2.41703584670838,2.44128701126702,
2.48333346315426,2.49309918628749,2.50291126105775,2.53199399121754,2.57116295231783,
2.58701551590747),.UNSPECIFIED.) ;
#1411=B_SPLINE_CURVE_WITH_KNOTS('',3,(#63207,#63208,#63209,#63210,#63211,
#63212,#63213,#63214,#63215,#63216,#63217,#63218,#63219,#63220,#63221,#63222,
#63223,#63224,#63225,#63226,#63227,#63228,#63229,#63230,#63231,#63232,#63233,
#63234,#63235,#63236,#63237,#63238,#63239,#63240,#63241,#63242,#63243,#63244,
#63245,#63246,#63247,#63248,#63249,#63250,#63251,#63252,#63253,#63254,#63255,
#63256,#63257,#63258,#63259,#63260,#63261,#63262,#63263,#63264,#63265,#63266,
#63267,#63268,#63269,#63270,#63271,#63272,#63273,#63274,#63275,#63276,#63277,
#63278,#63279,#63280,#63281,#63282,#63283,#63284,#63285,#63286,#63287,#63288,
#63289,#63290,#63291,#63292,#63293,#63294,#63295,#63296,#63297,#63298,#63299,
#63300,#63301,#63302,#63303,#63304,#63305,#63306,#63307,#63308,#63309,#63310,
#63311,#63312,#63313,#63314,#63315,#63316,#63317,#63318),.UNSPECIFIED.,
 .F.,.F.,(4,2,2,2,2,2,2,2,2,2,2,2,2,2,2,2,2,2,2,2,2,2,2,2,2,2,2,2,2,2,2,
2,2,2,2,2,2,2,2,2,2,2,2,2,2,2,2,2,2,2,2,2,2,2,2,4),(0.687313624506759,0.701487328335802,
0.734261479337814,0.750051238807075,0.766148089620778,0.81322549738789,
0.842574340968868,0.852382433439021,0.862219315435964,0.904004889536085,
0.92830389317549,0.947846979049493,0.962817779763856,0.982722800982418,
1.02701784679081,1.04930750026651,1.0587322877403,1.06905631150427,1.11181989420872,
1.14526522935246,1.16108870200738,1.17715297117741,1.22461845419938,1.25371347403238,
1.2635155650422,1.27336541533369,1.29364526539605,1.3389703542264,1.35871221493386,
1.37367940451246,1.39336987329903,1.41800449057946,1.45892736397017,1.46884990288418,
1.47858448850023,1.50593422863064,1.55335686814451,1.56991071464222,1.58540750930348,
1.61326782805456,1.65461961511933,1.6693127286257,1.67809689378171,1.69064592279205,
1.72409721773405,1.76105117914191,1.77706975302792,1.79292690452481,1.82724216113084,
1.86846855252021,1.87899235408722,1.88829788557021,1.90913766874792,1.95414060546348,
1.97459517707942,1.98102711455768),.UNSPECIFIED.) ;
#1412=B_SPLINE_CURVE_WITH_KNOTS('',3,(#63319,#63320,#63321,#63322,#63323,
#63324,#63325,#63326,#63327,#63328,#63329,#63330,#63331,#63332,#63333,#63334,
#63335,#63336,#63337,#63338,#63339,#63340,#63341,#63342,#63343,#63344,#63345,
#63346,#63347,#63348,#63349,#63350,#63351,#63352,#63353,#63354,#63355,#63356,
#63357,#63358,#63359,#63360,#63361,#63362,#63363,#63364,#63365,#63366,#63367,
#63368,#63369,#63370,#63371,#63372,#63373,#63374,#63375,#63376,#63377,#63378,
#63379,#63380,#63381,#63382,#63383,#63384,#63385,#63386,#63387,#63388,#63389,
#63390,#63391,#63392,#63393,#63394,#63395,#63396,#63397,#63398,#63399,#63400,
#63401,#63402,#63403,#63404,#63405,#63406,#63407,#63408,#63409,#63410,#63411,
#63412,#63413,#63414,#63415,#63416,#63417,#63418,#63419,#63420,#63421,#63422,
#63423,#63424,#63425,#63426,#63427,#63428,#63429,#63430),.UNSPECIFIED.,
 .F.,.F.,(4,2,2,2,2,2,2,2,2,2,2,2,2,2,2,2,2,2,2,2,2,2,2,2,2,2,2,2,2,2,2,
2,2,2,2,2,2,2,2,2,2,2,2,2,2,2,2,2,2,2,2,2,2,2,2,4),(1.06478356715028,1.07180327287809,
1.11247574840424,1.14270741058747,1.15829491714819,1.17443915661351,1.22546484370874,
1.25084218307447,1.26044459806911,1.27037500521748,1.29413790167027,1.34795120278219,
1.36361751705694,1.37965595762295,1.41617789572498,1.45520969852429,1.46526393074012,
1.47476671412784,1.49857395341122,1.55388273738589,1.5694919492235,1.58561111503344,
1.6057845335696,1.64639377285377,1.66428268995742,1.67328161761124,1.68428615114499,
1.69795741869486,1.73397654054865,1.76090093670943,1.7762537542395,1.79278143882586,
1.82758785260108,1.86632141360382,1.87639668433993,1.88588088324249,1.90943173426611,
1.96518601904047,1.98078348737423,1.99692903713025,2.01710053753758,2.05797545704317,
2.07539889105169,2.08441862376016,2.09541973305932,2.10908212808277,2.14504995500031,
2.17194393727841,2.18729207683965,2.20382663615556,2.23867415361913,2.27743584746603,
2.28750870492712,2.29695511804877,2.32016061345587,2.35872509297639),
 .UNSPECIFIED.) ;
#1413=B_SPLINE_CURVE_WITH_KNOTS('',3,(#63432,#63433,#63434,#63435,#63436,
#63437,#63438,#63439,#63440,#63441,#63442,#63443,#63444,#63445,#63446,#63447,
#63448,#63449,#63450,#63451,#63452,#63453,#63454,#63455,#63456,#63457,#63458,
#63459,#63460,#63461,#63462,#63463,#63464,#63465,#63466,#63467,#63468,#63469,
#63470,#63471,#63472,#63473,#63474,#63475,#63476,#63477,#63478,#63479,#63480,
#63481,#63482,#63483,#63484,#63485,#63486,#63487,#63488,#63489,#63490,#63491,
#63492,#63493,#63494,#63495,#63496,#63497,#63498,#63499,#63500,#63501,#63502,
#63503,#63504,#63505,#63506,#63507,#63508,#63509,#63510,#63511,#63512,#63513,
#63514,#63515,#63516,#63517,#63518,#63519,#63520,#63521,#63522,#63523,#63524,
#63525,#63526,#63527,#63528,#63529,#63530,#63531,#63532,#63533,#63534,#63535,
#63536,#63537,#63538,#63539),.UNSPECIFIED.,.F.,.F.,(4,2,2,2,2,2,2,2,2,2,
2,2,2,2,2,2,2,2,2,2,2,2,2,2,2,2,2,2,2,2,2,2,2,2,2,2,2,2,2,2,2,2,2,2,2,2,
2,2,2,2,2,2,2,4),(1.00000007181855E-6,0.04310229809024,0.0717672045422332,
0.08732439453051,0.103789024716376,0.152286090776099,0.17089027468351,0.184306167100127,
0.193061495476943,0.206693618374769,0.247627785375472,0.277039577271946,
0.29264137290383,0.309009459026135,0.35841804016586,0.384729351107226,0.39441285665854,
0.404387843685088,0.44471198748948,0.481024551681036,0.496954337073038,
0.512918819493949,0.561699672081028,0.590022275536263,0.599798646286373,
0.609681813849166,0.655828673281404,0.67800925118522,0.696576734116657,
0.711587951794427,0.73278117752412,0.776535005070598,0.797151998635442,
0.806439356836159,0.817003621720242,0.857897183765614,0.881700127370489,
0.90102041460234,0.915994706807118,0.936149449285819,0.980349387386379,
1.00228158178055,1.01167842912849,1.02205077680465,1.06443874400431,1.0974786836724,
1.11344391614396,1.12936979350977,1.16554051541397,1.20611103437312,1.21606544033483,
1.22576567221527,1.25243626665452,1.29365561641325),.UNSPECIFIED.) ;
#1414=B_SPLINE_CURVE_WITH_KNOTS('',3,(#63540,#63541,#63542,#63543,#63544,
#63545,#63546,#63547,#63548,#63549,#63550,#63551,#63552,#63553,#63554,#63555,
#63556,#63557,#63558,#63559,#63560,#63561,#63562,#63563,#63564,#63565,#63566,
#63567,#63568,#63569,#63570,#63571,#63572,#63573,#63574,#63575,#63576,#63577,
#63578,#63579,#63580,#63581,#63582,#63583,#63584,#63585,#63586,#63587,#63588,
#63589,#63590,#63591,#63592,#63593,#63594,#63595,#63596,#63597,#63598,#63599,
#63600,#63601,#63602,#63603,#63604,#63605,#63606,#63607,#63608,#63609,#63610,
#63611,#63612,#63613,#63614,#63615,#63616,#63617,#63618,#63619,#63620,#63621,
#63622,#63623,#63624,#63625,#63626,#63627,#63628,#63629,#63630,#63631,#63632,
#63633,#63634,#63635,#63636,#63637,#63638,#63639,#63640,#63641,#63642,#63643,
#63644,#63645,#63646,#63647,#63648,#63649,#63650,#63651,#63652,#63653,#63654,
#63655),.UNSPECIFIED.,.F.,.F.,(4,2,2,2,2,2,2,2,2,2,2,2,2,2,2,2,2,2,2,2,
2,2,2,2,2,2,2,2,2,2,2,2,2,2,2,2,2,2,2,2,2,2,2,2,2,2,2,2,2,2,2,2,2,2,2,2,
2,4),(1.29379821101641,1.29399768775507,1.34779007049791,1.36345729999771,
1.37949685755168,1.41603312542794,1.45503519551955,1.46509141930463,1.47459359649869,
1.49839194456128,1.55371126551867,1.56932094490488,1.58544360588411,1.60561564754221,
1.6462548501808,1.6641066737258,1.67310240150238,1.68411759843942,1.69780934608688,
1.73397078218191,1.76077543185893,1.77612055038952,1.79267091237169,1.82770495891532,
1.8660237806458,1.87613061406909,1.88559207883374,1.90883701585102,1.95329571087948,
1.97254754275993,1.98743643684044,2.00737058109388,2.03264141988664,2.0717603407041,
2.08180971648824,2.09133976928329,2.11552667077626,2.17017172158935,2.18579355255731,
2.20186872193732,2.22200592038068,2.26209434447167,2.28054700882681,2.28959063495702,
2.30041802100384,2.31376315994981,2.34766677696385,2.37642573705158,2.3918495327552,
2.4079984449846,2.42810851253555,2.46928473134019,2.48665829153025,2.49566329786108,
2.50677095702138,2.52059062840577,2.5749061863343,2.58760867156725),
 .UNSPECIFIED.) ;
#1415=B_SPLINE_CURVE_WITH_KNOTS('',3,(#63789,#63790,#63791,#63792,#63793,
#63794,#63795,#63796,#63797,#63798,#63799,#63800,#63801,#63802,#63803,#63804,
#63805,#63806,#63807,#63808,#63809,#63810,#63811,#63812,#63813,#63814,#63815,
#63816,#63817,#63818,#63819,#63820,#63821,#63822,#63823,#63824,#63825,#63826,
#63827,#63828,#63829,#63830,#63831,#63832,#63833,#63834,#63835,#63836,#63837,
#63838,#63839,#63840,#63841,#63842,#63843,#63844,#63845,#63846,#63847,#63848,
#63849,#63850,#63851,#63852,#63853,#63854,#63855,#63856,#63857,#63858,#63859,
#63860,#63861,#63862,#63863,#63864,#63865,#63866,#63867,#63868,#63869,#63870,
#63871,#63872,#63873,#63874,#63875,#63876),.UNSPECIFIED.,.F.,.F.,(4,3,3,
3,3,3,3,3,3,3,3,3,3,3,3,3,3,3,3,3,3,3,3,3,3,3,3,3,3,4),(1.00729736670009E-13,
0.0221235299431287,0.0446174963640137,0.0671263177453645,0.0720884332894729,
0.076729319300931,0.0810427188638101,0.102988755137381,0.124600311552118,
0.142904081042321,0.150434907716478,0.153947638893036,0.15757063756295,
0.178344943855092,0.19730630612935,0.219592370862223,0.224536090126318,
0.229375759206846,0.250039152971169,0.270700034753772,0.285804623298588,
0.292050600364105,0.29668581086518,0.300587021381912,0.320363777276505,
0.334366308076049,0.338839275887222,0.357867994143732,0.375594823992338,
0.378621596831646),.UNSPECIFIED.) ;
#1416=B_SPLINE_CURVE_WITH_KNOTS('',3,(#63877,#63878,#63879,#63880),
 .UNSPECIFIED.,.F.,.F.,(4,4),(-0.0138074141789072,0.),.UNSPECIFIED.) ;
#1417=B_SPLINE_CURVE_WITH_KNOTS('',3,(#63881,#63882,#63883,#63884,#63885,
#63886,#63887,#63888,#63889,#63890,#63891,#63892,#63893,#63894,#63895,#63896,
#63897,#63898,#63899,#63900,#63901,#63902,#63903,#63904,#63905,#63906,#63907,
#63908,#63909,#63910,#63911,#63912,#63913,#63914,#63915,#63916,#63917,#63918,
#63919,#63920,#63921,#63922,#63923,#63924,#63925,#63926,#63927,#63928,#63929,
#63930,#63931,#63932,#63933,#63934,#63935,#63936,#63937,#63938,#63939,#63940,
#63941,#63942,#63943,#63944,#63945,#63946,#63947,#63948,#63949,#63950,#63951,
#63952,#63953,#63954,#63955,#63956,#63957,#63958,#63959,#63960,#63961,#63962),
 .UNSPECIFIED.,.F.,.F.,(4,3,3,3,3,3,3,3,3,3,3,3,3,3,3,3,3,3,3,3,3,3,3,3,
3,3,3,4),(0.,0.0192100399714304,0.0384200799428608,0.055785952962528,0.0645126646314185,
0.0684606658468628,0.0884975138119028,0.108898824373168,0.126010884304925,
0.133916812365884,0.137322332661616,0.158397233054311,0.177347064100198,
0.197886036319214,0.205726140874419,0.209179108299885,0.230195957097379,
0.251694413295706,0.267939703341714,0.278006548808323,0.281855553762351,
0.304704589038728,0.321841365496011,0.327921806975797,0.332526964769193,
0.355052364906858,0.373251694867859,0.376839357608217),.UNSPECIFIED.) ;
#1418=B_SPLINE_CURVE_WITH_KNOTS('',3,(#63964,#63965,#63966,#63967,#63968,
#63969,#63970,#63971,#63972,#63973,#63974,#63975,#63976,#63977,#63978,#63979,
#63980,#63981,#63982,#63983,#63984,#63985,#63986,#63987,#63988,#63989,#63990,
#63991,#63992,#63993,#63994,#63995,#63996,#63997,#63998,#63999,#64000,#64001,
#64002,#64003,#64004,#64005,#64006,#64007,#64008,#64009,#64010,#64011,#64012,
#64013,#64014,#64015,#64016,#64017,#64018,#64019,#64020,#64021,#64022,#64023,
#64024,#64025,#64026,#64027,#64028,#64029,#64030,#64031,#64032,#64033,#64034,
#64035,#64036,#64037,#64038,#64039,#64040,#64041,#64042,#64043,#64044,#64045,
#64046,#64047,#64048,#64049,#64050,#64051),.UNSPECIFIED.,.F.,.F.,(4,3,3,
3,3,3,3,3,3,3,3,3,3,3,3,3,3,3,3,3,3,3,3,3,3,3,3,3,3,4),(5.34946170487962E-14,
0.0220613291570655,0.0446321217778821,0.0636200746038394,0.0720889029016907,
0.0767303357960608,0.0810429822369568,0.102989201024467,0.124600515521827,
0.142904269786994,0.150435349014095,0.153949373757925,0.15757105346863,
0.178345139325078,0.197306306129323,0.218627577357312,0.22453625458675,
0.229375801300445,0.250064043909956,0.270695862024059,0.285804876280239,
0.292050902532932,0.296684879018388,0.30058685343006,0.32036361603869,0.334365964016229,
0.342126630243114,0.361105414329871,0.375594823991594,0.378621596831076),
 .UNSPECIFIED.) ;
#1419=B_SPLINE_CURVE_WITH_KNOTS('',3,(#64052,#64053,#64054,#64055),
 .UNSPECIFIED.,.F.,.F.,(4,4),(-0.0134973973772337,0.),.UNSPECIFIED.) ;
#1420=B_SPLINE_CURVE_WITH_KNOTS('',3,(#64056,#64057,#64058,#64059,#64060,
#64061,#64062,#64063,#64064,#64065,#64066,#64067,#64068,#64069,#64070,#64071,
#64072,#64073,#64074,#64075,#64076,#64077,#64078,#64079,#64080,#64081,#64082,
#64083,#64084,#64085,#64086,#64087,#64088,#64089,#64090,#64091,#64092,#64093,
#64094,#64095,#64096,#64097,#64098,#64099,#64100,#64101,#64102,#64103,#64104,
#64105,#64106,#64107,#64108,#64109,#64110,#64111,#64112,#64113,#64114,#64115,
#64116,#64117,#64118,#64119,#64120,#64121,#64122,#64123,#64124,#64125,#64126,
#64127,#64128,#64129,#64130,#64131,#64132,#64133,#64134,#64135,#64136,#64137),
 .UNSPECIFIED.,.F.,.F.,(4,3,3,3,3,3,3,3,3,3,3,3,3,3,3,3,3,3,3,3,3,3,3,3,
3,3,3,4),(3.17409362789655E-14,0.0186663984199296,0.0380218662608163,0.0557872186169466,
0.0645149005559747,0.0684613229714192,0.0884994930860193,0.108901579487709,
0.126012950640826,0.133920158377381,0.13732459125606,0.158399696136409,
0.177347064100177,0.197885577244719,0.205726115616592,0.209179162683429,
0.230011587728157,0.251527757213882,0.267940059171801,0.278007542448308,
0.281856177051311,0.304705056505491,0.321841716096126,0.327925912502187,
0.332533113463834,0.355058546105816,0.37325169486803,0.376841786571624),
 .UNSPECIFIED.) ;
#1421=B_SPLINE_CURVE_WITH_KNOTS('',3,(#64248,#64249,#64250,#64251,#64252,
#64253,#64254,#64255,#64256,#64257,#64258,#64259,#64260,#64261,#64262,#64263,
#64264,#64265,#64266,#64267,#64268,#64269,#64270,#64271,#64272,#64273,#64274,
#64275,#64276,#64277,#64278,#64279,#64280,#64281,#64282,#64283,#64284,#64285,
#64286,#64287,#64288,#64289,#64290,#64291,#64292,#64293,#64294,#64295,#64296,
#64297,#64298,#64299,#64300,#64301,#64302,#64303,#64304,#64305,#64306,#64307,
#64308,#64309,#64310,#64311,#64312,#64313,#64314,#64315,#64316,#64317,#64318,
#64319,#64320,#64321,#64322,#64323,#64324,#64325,#64326,#64327,#64328,#64329,
#64330,#64331,#64332,#64333,#64334,#64335),.UNSPECIFIED.,.F.,.F.,(4,3,3,
3,3,3,3,3,3,3,3,3,3,3,3,3,3,3,3,3,3,3,3,3,3,3,3,3,3,4),(3.89216075304479E-14,
0.0220602863195691,0.0446307899041969,0.0636188651664292,0.0720885386670094,
0.0767295469819096,0.0810427777397907,0.102989666982509,0.124601161044241,
0.142904125735975,0.15043500853201,0.153948033803229,0.157570731855551,
0.17834498986759,0.197306306129356,0.219592370862149,0.224536128779729,
0.229375769171433,0.249977950539616,0.270610274779213,0.285804685006822,
0.292050674378722,0.296685588060879,0.300586982663982,0.320363742140175,
0.334366234094961,0.338839181965638,0.357867873624408,0.375594823991698,
0.378621596831146),.UNSPECIFIED.) ;
#1422=B_SPLINE_CURVE_WITH_KNOTS('',3,(#64336,#64337,#64338,#64339),
 .UNSPECIFIED.,.F.,.F.,(4,4),(-0.013736327206518,0.),.UNSPECIFIED.) ;
#1423=B_SPLINE_CURVE_WITH_KNOTS('',3,(#64340,#64341,#64342,#64343,#64344,
#64345,#64346,#64347,#64348,#64349,#64350,#64351,#64352,#64353,#64354,#64355,
#64356,#64357,#64358,#64359,#64360,#64361,#64362,#64363,#64364,#64365,#64366,
#64367,#64368,#64369,#64370,#64371,#64372,#64373,#64374,#64375,#64376,#64377,
#64378,#64379,#64380,#64381,#64382,#64383,#64384,#64385,#64386,#64387,#64388,
#64389,#64390,#64391,#64392,#64393,#64394,#64395,#64396,#64397,#64398,#64399,
#64400,#64401,#64402,#64403,#64404,#64405,#64406,#64407,#64408,#64409,#64410,
#64411,#64412,#64413,#64414,#64415,#64416,#64417,#64418,#64419,#64420,#64421),
 .UNSPECIFIED.,.F.,.F.,(4,3,3,3,3,3,3,3,3,3,3,3,3,3,3,3,3,3,3,3,3,3,3,3,
3,3,3,4),(0.,0.0192102002368296,0.0384204004736592,0.0580717225209105,0.0645131601572585,
0.0684608111803333,0.0885193531365119,0.108980282713294,0.126011344795134,
0.133917558241526,0.137322834176858,0.158397782796061,0.177347064100205,
0.19793323080713,0.205726138478045,0.209179123689474,0.230012007766502,
0.25152839500007,0.267939779531672,0.278006763196592,0.281855688543813,
0.304103277722834,0.321841441310683,0.327922698413653,0.332528297341932,
0.355053704892794,0.373251694868088,0.376839994115088),.UNSPECIFIED.) ;
#1424=B_SPLINE_CURVE_WITH_KNOTS('',3,(#64423,#64424,#64425,#64426,#64427,
#64428,#64429,#64430,#64431,#64432,#64433,#64434,#64435,#64436,#64437,#64438,
#64439,#64440,#64441,#64442,#64443,#64444,#64445,#64446,#64447,#64448,#64449,
#64450,#64451,#64452,#64453,#64454,#64455,#64456,#64457,#64458,#64459,#64460,
#64461,#64462,#64463,#64464,#64465,#64466,#64467,#64468,#64469,#64470,#64471,
#64472,#64473,#64474,#64475,#64476,#64477,#64478,#64479,#64480,#64481,#64482,
#64483,#64484,#64485,#64486,#64487,#64488,#64489,#64490,#64491,#64492,#64493,
#64494,#64495,#64496,#64497,#64498,#64499,#64500,#64501,#64502,#64503,#64504,
#64505,#64506,#64507,#64508,#64509,#64510),.UNSPECIFIED.,.F.,.F.,(4,3,3,
3,3,3,3,3,3,3,3,3,3,3,3,3,3,3,3,3,3,3,3,3,3,3,3,3,3,4),(1.00729736669584E-13,
0.0222595867875412,0.0445191735749817,0.0670286285400456,0.0720881472512565,
0.0767287027071146,0.0810425597515141,0.10298847612419,0.124769835483849,
0.142903953145218,0.150434629214208,0.153946551955451,0.157570379123684,
0.178344813275407,0.197306306129324,0.219592370862128,0.224535980326332,
0.229375730713216,0.250039050954983,0.270699830372278,0.285804444287051,
0.292050384204472,0.296686448092421,0.300587128415665,0.320363869220581,
0.334366498947699,0.338839516680554,0.357868298713684,0.375594823991754,
0.378621596831215),.UNSPECIFIED.) ;
#1425=B_SPLINE_CURVE_WITH_KNOTS('',3,(#64511,#64512,#64513,#64514),
 .UNSPECIFIED.,.F.,.F.,(4,4),(-0.0140044709886694,0.),.UNSPECIFIED.) ;
#1426=B_SPLINE_CURVE_WITH_KNOTS('',3,(#64515,#64516,#64517,#64518,#64519,
#64520,#64521,#64522,#64523,#64524,#64525,#64526,#64527,#64528,#64529,#64530,
#64531,#64532,#64533,#64534,#64535,#64536,#64537,#64538,#64539,#64540,#64541,
#64542,#64543,#64544,#64545,#64546,#64547,#64548,#64549,#64550,#64551,#64552,
#64553,#64554,#64555,#64556,#64557,#64558,#64559,#64560,#64561,#64562,#64563,
#64564,#64565,#64566,#64567,#64568,#64569,#64570,#64571,#64572,#64573,#64574,
#64575,#64576,#64577,#64578,#64579,#64580,#64581,#64582,#64583,#64584,#64585,
#64586,#64587,#64588,#64589,#64590,#64591,#64592,#64593,#64594,#64595,#64596),
 .UNSPECIFIED.,.F.,.F.,(4,3,3,3,3,3,3,3,3,3,3,3,3,3,3,3,3,3,3,3,3,3,3,3,
3,3,3,4),(0.,0.0185723777350143,0.0384192135306582,0.0580697119410092,0.0645113251116958,
0.0684602738285915,0.0884963219684918,0.10889715448173,0.126009631886339,
0.133914783248957,0.137320974046069,0.158395735620463,0.177347064100166,
0.197886298886923,0.20572613840078,0.209179057335835,0.230196205898824,
0.251694832634604,0.267939505072923,0.278005985924277,0.281855198662189,
0.30470432271361,0.321841165752176,0.327919447372899,0.332523443571899,
0.355048823266237,0.373251694867873,0.376837924097267),.UNSPECIFIED.) ;
#1427=B_SPLINE_CURVE_WITH_KNOTS('',3,(#64698,#64699,#64700,#64701,#64702,
#64703,#64704,#64705,#64706,#64707,#64708,#64709,#64710,#64711,#64712,#64713,
#64714,#64715,#64716,#64717,#64718,#64719,#64720,#64721,#64722,#64723,#64724,
#64725,#64726,#64727,#64728,#64729,#64730,#64731,#64732,#64733,#64734,#64735,
#64736,#64737,#64738,#64739,#64740,#64741,#64742,#64743,#64744,#64745,#64746,
#64747,#64748,#64749,#64750,#64751,#64752,#64753,#64754,#64755,#64756,#64757,
#64758,#64759,#64760,#64761,#64762,#64763,#64764,#64765,#64766,#64767,#64768,
#64769,#64770,#64771,#64772,#64773,#64774,#64775,#64776,#64777,#64778,#64779),
 .UNSPECIFIED.,.F.,.F.,(4,3,3,3,3,3,3,3,3,3,3,3,3,3,3,3,3,3,3,3,3,3,3,3,
3,3,3,4),(8.24698146814812E-14,0.0185733671595044,0.0384200792770817,0.0580711800398123,
0.0645126636019183,0.068460665561335,0.088497512914447,0.10895830285563,
0.126010883358896,0.133916810832616,0.137322331620615,0.158397231988687,
0.177347064100123,0.197886036524632,0.20572614087733,0.209179108308654,
0.230195957342159,0.251694413674633,0.267939703154651,0.278006548277264,
0.28185555342019,0.304704588782137,0.321841365303597,0.327921804787657,
0.332526961499993,0.355052361625049,0.373251694867978,0.376636436824541),
 .UNSPECIFIED.) ;
#1428=B_SPLINE_CURVE_WITH_KNOTS('',3,(#64781,#64782,#64783,#64784,#64785,
#64786,#64787,#64788,#64789,#64790,#64791,#64792,#64793,#64794,#64795,#64796,
#64797,#64798,#64799,#64800,#64801,#64802,#64803,#64804,#64805,#64806,#64807,
#64808,#64809,#64810,#64811,#64812,#64813,#64814,#64815,#64816,#64817,#64818,
#64819,#64820,#64821,#64822,#64823,#64824,#64825,#64826,#64827,#64828,#64829,
#64830,#64831,#64832,#64833,#64834,#64835,#64836,#64837,#64838,#64839,#64840,
#64841,#64842,#64843,#64844,#64845,#64846,#64847,#64848,#64849,#64850,#64851,
#64852,#64853,#64854,#64855,#64856,#64857,#64858,#64859,#64860,#64861,#64862,
#64863,#64864,#64865,#64866,#64867,#64868),.UNSPECIFIED.,.F.,.F.,(4,3,3,
3,3,3,3,3,3,3,3,3,3,3,3,3,3,3,3,3,3,3,3,3,3,3,3,3,3,4),(5.76922506808559E-14,
0.0219456891822088,0.0445202601827566,0.0636185159260876,0.0720884335083992,
0.076729319773797,0.0810427189711626,0.102988755333381,0.124770006124255,
0.142904081125542,0.150434907918552,0.1539476396971,0.157570637756284,0.17834494394397,
0.197306306129405,0.219592370862145,0.224536090207257,0.229375759240474,
0.250063857568636,0.270700034922499,0.285804623459792,0.292050600549566,
0.296685810329238,0.300587021291056,0.320363777194857,0.334366307920816,
0.338839275713723,0.357867993938263,0.375594823991326,0.378621596830935),
 .UNSPECIFIED.) ;
#1429=B_SPLINE_CURVE_WITH_KNOTS('',3,(#64869,#64870,#64871,#64872),
 .UNSPECIFIED.,.F.,.F.,(4,4),(-0.0138072657414553,0.),.UNSPECIFIED.) ;
#1430=B_SPLINE_CURVE_WITH_KNOTS('',3,(#64873,#64874,#64875,#64876,#64877,
#64878,#64879,#64880,#64881,#64882,#64883,#64884,#64885,#64886,#64887,#64888,
#64889,#64890,#64891,#64892,#64893,#64894,#64895,#64896,#64897,#64898,#64899,
#64900,#64901,#64902,#64903,#64904,#64905,#64906,#64907,#64908,#64909,#64910,
#64911,#64912,#64913,#64914,#64915,#64916,#64917,#64918,#64919,#64920,#64921,
#64922,#64923,#64924,#64925,#64926,#64927,#64928,#64929,#64930,#64931,#64932,
#64933,#64934,#64935,#64936,#64937,#64938,#64939,#64940,#64941,#64942,#64943,
#64944,#64945,#64946,#64947,#64948,#64949,#64950,#64951,#64952,#64953,#64954),
 .UNSPECIFIED.,.F.,.F.,(4,3,3,3,3,3,3,3,3,3,3,3,3,3,3,3,3,3,3,3,3,3,3,3,
3,3,3,4),(3.4584468016288E-14,0.0186663974215186,0.0380218644258986,0.0557872178449611,
0.0645148991924529,0.0684613225756388,0.0885208853153824,0.108982177034512,
0.12601294939485,0.133920156360152,0.137324589860616,0.158399694620118,
0.17734706410018,0.197885577533013,0.205726115643369,0.209179162646155,
0.230436403891952,0.251693645137749,0.267940058956061,0.278007541853836,
0.281856176673541,0.304103707162294,0.321841715883582,0.327925910083578,
0.332533109824159,0.355058542437522,0.37325169486792,0.376642568111857),
 .UNSPECIFIED.) ;
#1431=B_SPLINE_CURVE_WITH_KNOTS('',3,(#64956,#64957,#64958,#64959,#64960,
#64961,#64962,#64963,#64964,#64965,#64966,#64967,#64968,#64969,#64970,#64971,
#64972,#64973,#64974,#64975,#64976,#64977,#64978,#64979,#64980,#64981,#64982,
#64983,#64984,#64985,#64986,#64987,#64988,#64989,#64990,#64991,#64992,#64993,
#64994,#64995,#64996,#64997,#64998,#64999,#65000,#65001,#65002,#65003,#65004,
#65005,#65006,#65007,#65008,#65009,#65010,#65011,#65012,#65013,#65014,#65015,
#65016,#65017,#65018,#65019,#65020,#65021,#65022,#65023,#65024,#65025,#65026,
#65027,#65028,#65029,#65030,#65031,#65032,#65033,#65034,#65035,#65036,#65037,
#65038,#65039,#65040,#65041,#65042,#65043),.UNSPECIFIED.,.F.,.F.,(4,3,3,
3,3,3,3,3,3,3,3,3,3,3,3,3,3,3,3,3,3,3,3,3,3,3,3,3,3,4),(5.01899537219355E-14,
0.022261021302217,0.0445220426043838,0.063620075545003,0.0720889031852736,
0.0767303364111753,0.081042982385457,0.102989991413452,0.124601296415552,
0.142904269884553,0.150435349267875,0.153949374744116,0.157571053709541,
0.178345139423612,0.197306306129337,0.219592370862122,0.224536254679833,
0.229375801326243,0.249978049553714,0.270610495293834,0.285804876420835,
0.292050902697761,0.296684878486927,0.300586853329895,0.320363615935058,
0.334365963793087,0.338838836352753,0.357867421790014,0.375594823991614,
0.378621596831099),.UNSPECIFIED.) ;
#1432=B_SPLINE_CURVE_WITH_KNOTS('',3,(#65044,#65045,#65046,#65047),
 .UNSPECIFIED.,.F.,.F.,(4,4),(-0.0134972157492807,0.),.UNSPECIFIED.) ;
#1433=B_SPLINE_CURVE_WITH_KNOTS('',3,(#65105,#65106,#65107,#65108,#65109,
#65110,#65111,#65112,#65113,#65114,#65115,#65116,#65117,#65118,#65119,#65120,
#65121,#65122,#65123,#65124,#65125,#65126,#65127,#65128,#65129,#65130,#65131,
#65132,#65133,#65134,#65135,#65136,#65137,#65138,#65139,#65140,#65141,#65142,
#65143,#65144,#65145,#65146,#65147,#65148,#65149,#65150,#65151,#65152,#65153,
#65154,#65155,#65156,#65157,#65158,#65159,#65160,#65161,#65162,#65163,#65164,
#65165,#65166,#65167,#65168,#65169,#65170,#65171,#65172,#65173,#65174,#65175,
#65176,#65177,#65178,#65179,#65180,#65181,#65182,#65183,#65184,#65185,#65186),
 .UNSPECIFIED.,.F.,.F.,(4,3,3,3,3,3,3,3,3,3,3,3,3,3,3,3,3,3,3,3,3,3,3,3,
3,3,3,4),(0.,0.0190097553505953,0.0380195107011905,0.0557862339567285,0.06451316109333,
0.0684608114710175,0.0884979543611649,0.108958851497587,0.12601134567694,
0.133917559668794,0.137322835116023,0.15839778382808,0.177347064100199,
0.19788593667367,0.205726138471509,0.209179123708651,0.230195858569767,
0.251694250143536,0.273404722411164,0.278006763619963,0.281855688822625,
0.304103277964979,0.321841441467572,0.327922700231332,0.332528300050647,
0.355053707620067,0.373251694868217,0.376638067983665),.UNSPECIFIED.) ;
#1434=B_SPLINE_CURVE_WITH_KNOTS('',3,(#65188,#65189,#65190,#65191,#65192,
#65193,#65194,#65195,#65196,#65197,#65198,#65199,#65200,#65201,#65202,#65203,
#65204,#65205,#65206,#65207,#65208,#65209,#65210,#65211,#65212,#65213,#65214,
#65215,#65216,#65217,#65218,#65219,#65220,#65221,#65222,#65223,#65224,#65225,
#65226,#65227,#65228,#65229,#65230,#65231,#65232,#65233,#65234,#65235,#65236,
#65237,#65238,#65239,#65240,#65241,#65242,#65243,#65244,#65245,#65246,#65247,
#65248,#65249,#65250,#65251,#65252,#65253,#65254,#65255,#65256,#65257,#65258,
#65259,#65260,#65261,#65262,#65263,#65264,#65265,#65266,#65267,#65268,#65269,
#65270,#65271,#65272,#65273,#65274,#65275),.UNSPECIFIED.,.F.,.F.,(4,3,3,
3,3,3,3,3,3,3,3,3,3,3,3,3,3,3,3,3,3,3,3,3,3,3,3,3,3,4),(9.162090914368E-15,
0.0220602857583224,0.0446307891766625,0.0636188645106495,0.0720885384695292,
0.0767295465548163,0.0810427776264755,0.102988856337251,0.124600360073992,
0.142904125650606,0.150435008341509,0.153948033057643,0.157570731677898,
0.17834498979002,0.197306306129364,0.219592370862108,0.224536128708099,
0.229375769148714,0.250063899389668,0.27070010984115,0.285804684882141,
0.292050674233032,0.296685588486541,0.300586982738274,0.320363742208751,
0.334366234242714,0.338839182158917,0.357867873880841,0.375594823991314,
0.378621596830874),.UNSPECIFIED.) ;
#1435=B_SPLINE_CURVE_WITH_KNOTS('',3,(#65276,#65277,#65278,#65279),
 .UNSPECIFIED.,.F.,.F.,(4,4),(-0.0137364598392755,0.),.UNSPECIFIED.) ;
#1436=B_SPLINE_CURVE_WITH_KNOTS('',3,(#65280,#65281,#65282,#65283,#65284,
#65285,#65286,#65287,#65288,#65289,#65290,#65291,#65292,#65293,#65294,#65295,
#65296,#65297,#65298,#65299,#65300,#65301,#65302,#65303,#65304,#65305,#65306,
#65307,#65308,#65309,#65310,#65311,#65312,#65313,#65314,#65315,#65316,#65317,
#65318,#65319,#65320,#65321,#65322,#65323,#65324,#65325,#65326,#65327,#65328,
#65329,#65330,#65331,#65332,#65333,#65334,#65335,#65336,#65337,#65338,#65339,
#65340,#65341,#65342,#65343,#65344,#65345,#65346,#65347,#65348,#65349,#65350,
#65351,#65352,#65353,#65354,#65355,#65356,#65357,#65358,#65359,#65360,#65361),
 .UNSPECIFIED.,.F.,.F.,(4,3,3,3,3,3,3,3,3,3,3,3,3,3,3,3,3,3,3,3,3,3,3,3,
3,3,3,4),(0.,0.0185723782769974,0.0384192140048957,0.0557851952668067,0.0645113258447557,
0.0684602740353268,0.0884963226141113,0.108897155391316,0.126009632568533,
0.133914784354806,0.137320974779134,0.158395736535551,0.177347064100184,
0.19788629874665,0.205726138406649,0.209179057380608,0.230196205783086,
0.251694832427267,0.267939505171459,0.278005986203941,0.281855198863098,
0.304704322864273,0.321841165865154,0.327919448698485,0.332523445539268,
0.355048825232304,0.373251694867799,0.376632014560555),.UNSPECIFIED.) ;
#1437=B_SPLINE_CURVE_WITH_KNOTS('',3,(#65363,#65364,#65365,#65366,#65367,
#65368,#65369,#65370,#65371,#65372,#65373,#65374,#65375,#65376,#65377,#65378,
#65379,#65380,#65381,#65382,#65383,#65384,#65385,#65386,#65387,#65388,#65389,
#65390,#65391,#65392,#65393,#65394,#65395,#65396,#65397,#65398,#65399,#65400,
#65401,#65402,#65403,#65404,#65405,#65406,#65407,#65408,#65409,#65410,#65411,
#65412,#65413,#65414,#65415,#65416,#65417,#65418,#65419,#65420,#65421,#65422,
#65423,#65424,#65425,#65426,#65427,#65428,#65429,#65430,#65431,#65432,#65433,
#65434,#65435,#65436,#65437,#65438,#65439,#65440,#65441,#65442,#65443,#65444,
#65445,#65446,#65447,#65448,#65449,#65450),.UNSPECIFIED.,.F.,.F.,(4,3,3,
3,3,3,3,3,3,3,3,3,3,3,3,3,3,3,3,3,3,3,3,3,3,3,3,3,3,4),(9.16209091435299E-15,
0.0219448159624867,0.0445191729753408,0.0636175646195905,0.0720881470932013,
0.0767287023669779,0.0810425596539183,0.102969490401943,0.124769835375746,
0.142903953064144,0.150434629052655,0.15394655131555,0.157570378974426,
0.178344813208512,0.197306306129339,0.219592370862245,0.22453598026394,
0.229375730702232,0.250063743644679,0.270695308858957,0.285804444199926,
0.29205038409226,0.296686448479134,0.300587128478452,0.320363869272083,
0.334366499045275,0.338839516795851,0.357868298847846,0.375594823992585,
0.378621596831857),.UNSPECIFIED.) ;
#1438=B_SPLINE_CURVE_WITH_KNOTS('',3,(#65451,#65452,#65453,#65454),
 .UNSPECIFIED.,.F.,.F.,(4,4),(-0.0140045813698995,0.),.UNSPECIFIED.) ;
#1439=B_SPLINE_CURVE_WITH_KNOTS('',3,(#65519,#65520,#65521,#65522,#65523,
#65524,#65525,#65526,#65527,#65528),.UNSPECIFIED.,.F.,.F.,(4,2,2,2,4),(-1.45697727039821,
-1.34636560256276,-1.11265580623236,-0.878946009902128,-0.0207808841702046),
 .UNSPECIFIED.) ;
#1440=B_SPLINE_CURVE_WITH_KNOTS('',3,(#65610,#65611,#65612,#65613,#65614,
#65615,#65616,#65617,#65618,#65619),.UNSPECIFIED.,.F.,.F.,(4,2,2,2,4),(-0.99020975865206,
-0.4845401415634,-0.346827783328,-0.2091154250925,-0.143938039021296),
 .UNSPECIFIED.) ;
#1441=B_SPLINE_CURVE_WITH_KNOTS('',3,(#67179,#67180,#67181,#67182,#67183,
#67184,#67185,#67186,#67187,#67188,#67189,#67190,#67191,#67192,#67193,#67194,
#67195,#67196,#67197,#67198,#67199,#67200,#67201,#67202,#67203,#67204,#67205,
#67206,#67207,#67208,#67209,#67210,#67211,#67212,#67213,#67214,#67215,#67216,
#67217,#67218,#67219,#67220,#67221,#67222,#67223,#67224,#67225,#67226,#67227,
#67228,#67229,#67230,#67231,#67232,#67233,#67234,#67235,#67236,#67237,#67238,
#67239,#67240,#67241,#67242,#67243,#67244,#67245,#67246,#67247,#67248,#67249,
#67250,#67251,#67252,#67253,#67254,#67255,#67256,#67257,#67258,#67259,#67260),
 .UNSPECIFIED.,.F.,.F.,(4,3,3,3,3,3,3,3,3,3,3,3,3,3,3,3,3,3,3,3,3,3,3,3,
3,3,3,4),(0.,0.0192098677598375,0.038419735519675,0.0557856515922359,0.0645121321462078,
0.0684605097531964,0.0884970404929436,0.108898162240786,0.12601038770563,
0.133916007890461,0.137321792996603,0.15839663960389,0.177347064100162,
0.19788614178249,0.205726141447246,0.209179089705576,0.230196058990523,
0.251694583642526,0.267939623149047,0.278006322053237,0.28185541093348,
0.304704481917046,0.321841285154721,0.32792085991946,0.33252555045799,0.355050942519894,
0.373251694867745,0.376838869958313),.UNSPECIFIED.) ;
#1442=B_SPLINE_CURVE_WITH_KNOTS('',3,(#67262,#67263,#67264,#67265),
 .UNSPECIFIED.,.F.,.F.,(4,4),(-0.0138846719219583,0.),.UNSPECIFIED.) ;
#1443=B_SPLINE_CURVE_WITH_KNOTS('',3,(#67266,#67267,#67268,#67269,#67270,
#67271,#67272,#67273,#67274,#67275,#67276,#67277,#67278,#67279,#67280,#67281,
#67282,#67283,#67284,#67285,#67286,#67287,#67288,#67289,#67290,#67291,#67292,
#67293,#67294,#67295,#67296,#67297,#67298,#67299,#67300,#67301,#67302,#67303,
#67304,#67305,#67306,#67307,#67308,#67309,#67310,#67311,#67312,#67313,#67314,
#67315,#67316,#67317,#67318,#67319,#67320,#67321,#67322,#67323,#67324,#67325,
#67326,#67327,#67328,#67329,#67330,#67331,#67332,#67333,#67334,#67335,#67336,
#67337,#67338,#67339,#67340,#67341,#67342,#67343,#67344,#67345,#67346,#67347,
#67348,#67349,#67350,#67351,#67352,#67353),.UNSPECIFIED.,.F.,.F.,(4,3,3,
3,3,3,3,3,3,3,3,3,3,3,3,3,3,3,3,3,3,3,3,3,3,3,3,3,3,4),(0.,0.0219453428433969,
0.0445198298319151,0.0636181393690862,0.0720883201313736,0.0767290751133605,
0.0810426557911561,0.102988645412413,0.124769940064907,0.142904031581002,
0.150434798366333,0.153947211434901,0.15757053574031,0.178344893157862,
0.197306306129284,0.219592370862123,0.22453604752966,0.229375748144095,
0.250039112563139,0.270699953850697,0.285804554234559,0.292050517273299,
0.296686057701859,0.300587063445754,0.320363814274873,0.334366385364846,
0.338839373506665,0.357868118438046,0.375594823991995,0.378621596831454),
 .UNSPECIFIED.) ;
#1444=B_SPLINE_CURVE_WITH_KNOTS('',3,(#67447,#67448,#67449,#67450,#67451,
#67452,#67453,#67454,#67455,#67456,#67457,#67458,#67459,#67460,#67461,#67462,
#67463,#67464,#67465,#67466,#67467,#67468,#67469,#67470,#67471,#67472,#67473,
#67474,#67475,#67476,#67477,#67478,#67479,#67480,#67481,#67482,#67483,#67484,
#67485,#67486,#67487,#67488,#67489,#67490,#67491,#67492,#67493,#67494,#67495,
#67496,#67497,#67498,#67499,#67500,#67501,#67502,#67503,#67504,#67505,#67506,
#67507,#67508,#67509,#67510,#67511,#67512,#67513,#67514,#67515,#67516,#67517,
#67518,#67519,#67520,#67521,#67522,#67523,#67524,#67525,#67526,#67527,#67528,
#67529,#67530,#67531,#67532,#67533,#67534),.UNSPECIFIED.,.F.,.F.,(4,3,3,
3,3,3,3,3,3,3,3,3,3,3,3,3,3,3,3,3,3,3,3,3,3,3,3,3,3,4),(0.,0.0219453433760758,
0.0445198304945081,0.0636181399488659,0.0720883203064331,0.0767290754908875,
0.0810426558425648,0.102988645536193,0.124600257382722,0.142904031624236,
0.150434798509977,0.153947211955859,0.157570535874629,0.178344893214354,
0.19730630612937,0.219592370862188,0.224536047596205,0.229375748203205,
0.250039112667709,0.270699954016998,0.285804554457835,0.292050517506586,
0.296686057253529,0.300587063371026,0.320363814208887,0.33436638523497,
0.338839373502662,0.357868118393394,0.375594823991909,0.378621596831355),
 .UNSPECIFIED.) ;
#1445=B_SPLINE_CURVE_WITH_KNOTS('',3,(#67535,#67536,#67537,#67538,#67539,
#67540,#67541,#67542,#67543,#67544,#67545,#67546,#67547,#67548,#67549,#67550,
#67551,#67552,#67553,#67554,#67555,#67556,#67557,#67558,#67559,#67560,#67561,
#67562,#67563,#67564,#67565,#67566,#67567,#67568,#67569,#67570,#67571,#67572,
#67573,#67574,#67575,#67576,#67577,#67578,#67579,#67580,#67581,#67582,#67583,
#67584,#67585,#67586,#67587,#67588,#67589,#67590,#67591,#67592,#67593,#67594,
#67595,#67596,#67597,#67598,#67599,#67600,#67601,#67602,#67603,#67604,#67605,
#67606,#67607,#67608,#67609,#67610,#67611,#67612,#67613,#67614,#67615,#67616),
 .UNSPECIFIED.,.F.,.F.,(4,3,3,3,3,3,3,3,3,3,3,3,3,3,3,3,3,3,3,3,3,3,3,3,
3,3,3,4),(0.,0.0185729748977862,0.0384197360480747,0.0557856520545772,0.0645121329631303,
0.0684605101522518,0.0884970413840062,0.108898163423802,0.126010388592875,
0.133916009318279,0.137321793976508,0.158396640753416,0.177347064100094,
0.197886141621918,0.205726141448321,0.209179089633135,0.230196058731556,
0.251694583277031,0.267939623337495,0.278006322595857,0.281855411237803,
0.304704482145257,0.321841285325848,0.327920862075213,0.332525553640298,
0.355050945703461,0.37325169486762,0.376634694330848),.UNSPECIFIED.) ;
#1446=B_SPLINE_CURVE_WITH_KNOTS('',3,(#67617,#67618,#67619,#67620),
 .UNSPECIFIED.,.F.,.F.,(4,4),(-0.0138845519224747,0.),.UNSPECIFIED.) ;
#1447=B_SPLINE_CURVE_WITH_KNOTS('',3,(#67713,#67714,#67715,#67716,#67717,
#67718,#67719,#67720,#67721,#67722,#67723,#67724,#67725,#67726,#67727,#67728,
#67729,#67730,#67731,#67732,#67733,#67734,#67735,#67736,#67737,#67738,#67739,
#67740,#67741,#67742,#67743,#67744,#67745,#67746,#67747,#67748,#67749,#67750,
#67751,#67752,#67753,#67754,#67755,#67756,#67757,#67758,#67759,#67760,#67761,
#67762,#67763,#67764,#67765,#67766,#67767,#67768,#67769,#67770,#67771,#67772,
#67773,#67774,#67775,#67776,#67777,#67778,#67779,#67780,#67781,#67782,#67783,
#67784,#67785,#67786,#67787,#67788,#67789,#67790,#67791,#67792,#67793,#67794),
 .UNSPECIFIED.,.F.,.F.,(4,3,3,3,3,3,3,3,3,3,3,3,3,3,3,3,3,3,3,3,3,3,3,3,
3,3,3,4),(0.,0.0192105369393153,0.0384210738786305,0.0557868226563222,0.0645142011204561,
0.0684611170545584,0.0884988752384408,0.108900721836266,0.12601230740224,
0.133919117045334,0.137323885863973,0.158398930385445,0.177347064100164,
0.197885723726412,0.205726127529494,0.209179149862764,0.230195640933277,
0.251693894552056,0.267939944540674,0.2780072243568,0.281855977887993,0.304704907132977,
0.321841604066715,0.327924605076911,0.332531152092866,0.355056574852911,
0.373251694867928,0.376841042462691),.UNSPECIFIED.) ;
#1448=B_SPLINE_CURVE_WITH_KNOTS('',3,(#67796,#67797,#67798,#67799),
 .UNSPECIFIED.,.F.,.F.,(4,4),(-0.0135915899488536,0.),.UNSPECIFIED.) ;
#1449=B_SPLINE_CURVE_WITH_KNOTS('',3,(#67800,#67801,#67802,#67803,#67804,
#67805,#67806,#67807,#67808,#67809,#67810,#67811,#67812,#67813,#67814,#67815,
#67816,#67817,#67818,#67819,#67820,#67821,#67822,#67823,#67824,#67825,#67826,
#67827,#67828,#67829,#67830,#67831,#67832,#67833,#67834,#67835,#67836,#67837,
#67838,#67839,#67840,#67841,#67842,#67843,#67844,#67845,#67846,#67847,#67848,
#67849,#67850,#67851,#67852,#67853,#67854,#67855,#67856,#67857,#67858,#67859,
#67860,#67861,#67862,#67863,#67864,#67865,#67866,#67867,#67868,#67869,#67870,
#67871,#67872,#67873,#67874,#67875,#67876,#67877,#67878,#67879,#67880,#67881,
#67882,#67883,#67884,#67885,#67886,#67887),.UNSPECIFIED.,.F.,.F.,(4,3,3,
3,3,3,3,3,3,3,3,3,3,3,3,3,3,3,3,3,3,3,3,3,3,3,3,3,3,4),(0.,0.0219466832367342,
0.0445214891325778,0.0636195912571624,0.0720887573235693,0.0767300202064994,
0.0810429003250497,0.102989064460608,0.124770183534997,0.142904214183562,
0.150435214461133,0.153948842921585,0.157570925748775,0.17834508145342,
0.197306306129255,0.21959237086207,0.224536205782459,0.229375788908732,
0.250039268285765,0.270671218902195,0.285804804321276,0.292050816876209,
0.29668514998534,0.300586904076222,0.320363667238304,0.334366074527694,
0.338838978333996,0.357867609002265,0.375594823991774,0.378621596831228),
 .UNSPECIFIED.) ;
#1450=B_SPLINE_CURVE_WITH_KNOTS('',3,(#67981,#67982,#67983,#67984,#67985,
#67986,#67987,#67988,#67989,#67990,#67991,#67992,#67993,#67994,#67995,#67996,
#67997,#67998,#67999,#68000,#68001,#68002,#68003,#68004,#68005,#68006,#68007,
#68008,#68009,#68010,#68011,#68012,#68013,#68014,#68015,#68016,#68017,#68018,
#68019,#68020,#68021,#68022,#68023,#68024,#68025,#68026,#68027,#68028,#68029,
#68030,#68031,#68032,#68033,#68034,#68035,#68036,#68037,#68038,#68039,#68040,
#68041,#68042,#68043,#68044,#68045,#68046,#68047,#68048,#68049,#68050,#68051,
#68052,#68053,#68054,#68055,#68056,#68057,#68058,#68059,#68060,#68061,#68062,
#68063,#68064,#68065,#68066,#68067,#68068),.UNSPECIFIED.,.F.,.F.,(4,3,3,
3,3,3,3,3,3,3,3,3,3,3,3,3,3,3,3,3,3,3,3,3,3,3,3,3,3,4),(0.,0.02194668392425,
0.0445170790582017,0.0636195919983632,0.0720887575464768,0.076730020689144,
0.0810429004598939,0.102970387789171,0.124601244883116,0.142904214276635,
0.150435214673167,0.153948843786557,0.157570925953124,0.17834508154455,
0.197306306129309,0.219592370862138,0.224536205859184,0.229375788928963,
0.250039268366105,0.270700265757003,0.285804804442111,0.292050817016587,
0.296685149518139,0.300586903991452,0.320363667154172,0.334366074352361,
0.33883897815507,0.357867608757828,0.37559482399194,0.378621596831415),
 .UNSPECIFIED.) ;
#1451=B_SPLINE_CURVE_WITH_KNOTS('',3,(#68069,#68070,#68071,#68072,#68073,
#68074,#68075,#68076,#68077,#68078,#68079,#68080,#68081,#68082,#68083,#68084,
#68085,#68086,#68087,#68088,#68089,#68090,#68091,#68092,#68093,#68094,#68095,
#68096,#68097,#68098,#68099,#68100,#68101,#68102,#68103,#68104,#68105,#68106,
#68107,#68108,#68109,#68110,#68111,#68112,#68113,#68114,#68115,#68116,#68117,
#68118,#68119,#68120,#68121,#68122,#68123,#68124,#68125,#68126,#68127,#68128,
#68129,#68130,#68131,#68132,#68133,#68134,#68135,#68136,#68137,#68138,#68139,
#68140,#68141,#68142,#68143,#68144,#68145,#68146,#68147,#68148,#68149,#68150),
 .UNSPECIFIED.,.F.,.F.,(4,3,3,3,3,3,3,3,3,3,3,3,3,3,3,3,3,3,3,3,3,3,3,3,
3,3,3,4),(5.54425544496214E-15,0.0185745046356664,0.0384210745687243,0.05578682326015,
0.0645142021869443,0.0684611173773682,0.0886809202670926,0.108900723156817,
0.126012308392645,0.133919118648472,0.137323886999474,0.158398931615403,
0.17734706410013,0.197885723504055,0.20572612751327,0.209179149774556,0.230195640588201,
0.251693894061592,0.267939944783251,0.278007225045027,0.28185597836749,
0.304704907492569,0.321841604336379,0.327924608234368,0.332531156960973,
0.355056579722441,0.373251694867806,0.376640442450949),.UNSPECIFIED.) ;
#1452=B_SPLINE_CURVE_WITH_KNOTS('',3,(#68151,#68152,#68153,#68154),
 .UNSPECIFIED.,.F.,.F.,(4,4),(-0.0135914441700036,0.),.UNSPECIFIED.) ;
#1453=B_SPLINE_CURVE_WITH_KNOTS('',3,(#68247,#68248,#68249,#68250,#68251,
#68252,#68253,#68254,#68255,#68256,#68257,#68258,#68259,#68260,#68261,#68262,
#68263,#68264,#68265,#68266,#68267,#68268,#68269,#68270,#68271,#68272,#68273,
#68274,#68275,#68276,#68277,#68278,#68279,#68280,#68281,#68282,#68283,#68284,
#68285,#68286,#68287,#68288,#68289,#68290,#68291,#68292,#68293,#68294,#68295,
#68296,#68297,#68298,#68299,#68300,#68301,#68302,#68303,#68304,#68305,#68306,
#68307,#68308,#68309,#68310,#68311,#68312,#68313,#68314,#68315,#68316,#68317,
#68318,#68319,#68320,#68321,#68322,#68323,#68324,#68325,#68326,#68327,#68328),
 .UNSPECIFIED.,.F.,.F.,(4,3,3,3,3,3,3,3,3,3,3,3,3,3,3,3,3,3,3,3,3,3,3,3,
3,3,3,4),(0.,0.0186653277497641,0.0380199011942217,0.0557863969301571,0.0645134490238413,
0.0684608959992006,0.0886803456960418,0.108899795392883,0.126011612569693,
0.13391799191486,0.137323126160168,0.158398102128668,0.177347064100122,
0.197885878293307,0.205726136246136,0.209179131767074,0.230195799832242,
0.251694153565121,0.267939824662252,0.27800688974131,0.281855768049264,
0.304704749753896,0.32184148603237,0.327923223223719,0.332529082546112,
0.355054494362095,0.373251694867791,0.376840316779234),.UNSPECIFIED.) ;
#1454=B_SPLINE_CURVE_WITH_KNOTS('',3,(#68330,#68331,#68332,#68333),
 .UNSPECIFIED.,.F.,.F.,(4,4),(-0.0136957314155904,0.),.UNSPECIFIED.) ;
#1455=B_SPLINE_CURVE_WITH_KNOTS('',3,(#68334,#68335,#68336,#68337,#68338,
#68339,#68340,#68341,#68342,#68343,#68344,#68345,#68346,#68347,#68348,#68349,
#68350,#68351,#68352,#68353,#68354,#68355,#68356,#68357,#68358,#68359,#68360,
#68361,#68362,#68363,#68364,#68365,#68366,#68367,#68368,#68369,#68370,#68371,
#68372,#68373,#68374,#68375,#68376,#68377,#68378,#68379,#68380,#68381,#68382,
#68383,#68384,#68385,#68386,#68387,#68388,#68389,#68390,#68391,#68392,#68393,
#68394,#68395,#68396,#68397,#68398,#68399,#68400,#68401,#68402,#68403,#68404,
#68405,#68406,#68407,#68408,#68409,#68410,#68411,#68412,#68413,#68414,#68415,
#68416,#68417,#68418,#68419,#68420,#68421),.UNSPECIFIED.,.F.,.F.,(4,3,3,
3,3,3,3,3,3,3,3,3,3,3,3,3,3,3,3,3,3,3,3,3,3,3,3,3,3,4),(0.,0.0219461975997884,
0.0445208898907668,0.0636190669205846,0.0720885994199383,0.0767296783629433,
0.0810428117268152,0.102988914619533,0.12477009913424,0.142904150883007,
0.150435066187135,0.153948260028433,0.157570785971653,0.178345015861808,
0.197306306129309,0.219592370862132,0.22453615061269,0.229375774806808,
0.250063923624211,0.270700153327392,0.285804719459338,0.292050715582947,
0.296685462822605,0.300586960556721,0.320363721577313,0.334366190543196,
0.338839126472829,0.357867801974519,0.375594823991889,0.37862159683132),
 .UNSPECIFIED.) ;
#1456=B_SPLINE_CURVE_WITH_KNOTS('',3,(#68515,#68516,#68517,#68518,#68519,
#68520,#68521,#68522,#68523,#68524,#68525,#68526,#68527,#68528,#68529,#68530,
#68531,#68532,#68533,#68534,#68535,#68536,#68537,#68538,#68539,#68540,#68541,
#68542,#68543,#68544,#68545,#68546,#68547,#68548,#68549,#68550,#68551,#68552,
#68553,#68554,#68555,#68556,#68557,#68558,#68559,#68560,#68561,#68562,#68563,
#68564,#68565,#68566,#68567,#68568,#68569,#68570,#68571,#68572,#68573,#68574,
#68575,#68576,#68577,#68578,#68579,#68580,#68581,#68582,#68583,#68584,#68585,
#68586,#68587,#68588,#68589,#68590,#68591,#68592,#68593,#68594,#68595,#68596,
#68597,#68598,#68599,#68600,#68601,#68602),.UNSPECIFIED.,.F.,.F.,(4,3,3,
3,3,3,3,3,3,3,3,3,3,3,3,3,3,3,3,3,3,3,3,3,3,3,3,3,3,4),(0.,0.022060460365473,
0.0446310129567534,0.0636190676004925,0.0720885996247624,0.0767296788060056,
0.0810428118689025,0.102969752522996,0.124770099274268,0.142904150988042,
0.150435066396597,0.153948260818437,0.15757078615856,0.178345015953213,
0.197306306129363,0.219592370862223,0.224536150685866,0.229375774747225,
0.250039212190931,0.270700153395456,0.285804719367065,0.292050715531525,
0.296685462786989,0.300586960539555,0.32036372156161,0.334366190473772,
0.338839126428367,0.357867801873638,0.375594823992243,0.378621596831708),
 .UNSPECIFIED.) ;
#1457=B_SPLINE_CURVE_WITH_KNOTS('',3,(#68603,#68604,#68605,#68606,#68607,
#68608,#68609,#68610,#68611,#68612,#68613,#68614,#68615,#68616,#68617,#68618,
#68619,#68620,#68621,#68622,#68623,#68624,#68625,#68626,#68627,#68628,#68629,
#68630,#68631,#68632,#68633,#68634,#68635,#68636,#68637,#68638,#68639,#68640,
#68641,#68642,#68643,#68644,#68645,#68646,#68647,#68648,#68649,#68650,#68651,
#68652,#68653,#68654,#68655,#68656,#68657,#68658,#68659,#68660,#68661,#68662,
#68663,#68664,#68665,#68666,#68667,#68668,#68669,#68670,#68671,#68672,#68673,
#68674,#68675,#68676,#68677,#68678,#68679,#68680,#68681,#68682,#68683,#68684),
 .UNSPECIFIED.,.F.,.F.,(4,3,3,3,3,3,3,3,3,3,3,3,3,3,3,3,3,3,3,3,3,3,3,3,
3,3,3,4),(5.86898037579802E-15,0.0185739485137251,0.0384205879620368,0.0557863974793096,
0.0645134499942184,0.0684608962591978,0.0884982104060516,0.108959169029463,
0.126011613449541,0.133917993341252,0.13732312730515,0.15839810341835,0.177347064100219,
0.19788587809615,0.205726136237969,0.209179131790411,0.230436642512244,
0.251694153234078,0.267939824818217,0.278006890178637,0.281855768372809,
0.304704749996589,0.321841486214424,0.327923225385788,0.332529085719319,
0.355054497541321,0.373251694867928,0.376638087048362),.UNSPECIFIED.) ;
#1458=B_SPLINE_CURVE_WITH_KNOTS('',3,(#68685,#68686,#68687,#68688),
 .UNSPECIFIED.,.F.,.F.,(4,4),(-0.013695595170466,0.),.UNSPECIFIED.) ;
#1459=B_SPLINE_CURVE_WITH_KNOTS('',3,(#68726,#68727,#68728,#68729,#68730,
#68731,#68732,#68733,#68734,#68735,#68736,#68737,#68738,#68739,#68740,#68741,
#68742,#68743,#68744,#68745,#68746,#68747,#68748,#68749,#68750,#68751,#68752,
#68753,#68754,#68755,#68756,#68757,#68758,#68759,#68760,#68761,#68762,#68763,
#68764,#68765,#68766,#68767,#68768,#68769,#68770,#68771,#68772,#68773,#68774,
#68775,#68776,#68777,#68778,#68779,#68780,#68781,#68782,#68783,#68784,#68785,
#68786,#68787,#68788,#68789,#68790,#68791,#68792,#68793,#68794,#68795,#68796,
#68797,#68798,#68799,#68800,#68801,#68802,#68803,#68804,#68805,#68806,#68807),
 .UNSPECIFIED.,.F.,.F.,(4,3,3,3,3,3,3,3,3,3,3,3,3,3,3,3,3,3,3,3,3,3,3,3,
3,3,3,4),(0.,0.0185725451103903,0.0384193599840902,0.0557853229985777,0.064511551541945,
0.0684603399778252,0.0884965237471075,0.108897437788649,0.126009844366484,
0.1339151275527,0.137321204015421,0.158395989927514,0.17734706409999,0.197886255136487,
0.205726139728722,0.209179066900041,0.230196165563191,0.251694763856776,
0.267939537791735,0.278006079354413,0.281855257762263,0.304704367038516,
0.321841198995705,0.327919841261155,0.332524030692079,0.355049413867223,
0.373251694867274,0.376632749066777),.UNSPECIFIED.) ;
#1460=B_SPLINE_CURVE_WITH_KNOTS('',3,(#68809,#68810,#68811,#68812,#68813,
#68814,#68815,#68816,#68817,#68818,#68819,#68820,#68821,#68822,#68823,#68824,
#68825,#68826,#68827,#68828,#68829,#68830,#68831,#68832,#68833,#68834,#68835,
#68836,#68837,#68838,#68839,#68840,#68841,#68842,#68843,#68844,#68845,#68846,
#68847,#68848,#68849,#68850,#68851,#68852,#68853,#68854,#68855,#68856,#68857,
#68858,#68859,#68860,#68861,#68862,#68863,#68864,#68865,#68866,#68867,#68868,
#68869,#68870,#68871,#68872,#68873,#68874,#68875,#68876,#68877,#68878,#68879,
#68880,#68881,#68882,#68883,#68884,#68885,#68886,#68887,#68888,#68889,#68890,
#68891,#68892,#68893,#68894,#68895,#68896),.UNSPECIFIED.,.F.,.F.,(4,3,3,
3,3,3,3,3,3,3,3,3,3,3,3,3,3,3,3,3,3,3,3,3,3,3,3,3,3,4),(0.,0.0219449635441618,
0.0445193572281392,0.0636177258407953,0.0720881956305002,0.0767288068387337,
0.0810425866069912,0.102988523717188,0.12476986522952,0.142903975454487,
0.150434676809413,0.153946737384955,0.157570423094632,0.178344835953805,
0.197306306129388,0.219592370862226,0.224535999387828,0.229375735630069,
0.250039068149565,0.27069986487445,0.285804475479312,0.292050422080681,
0.296686337887541,0.300587110247004,0.320363854122266,0.334366467833364,
0.338839477495732,0.357868249573945,0.375594823992091,0.378621596831544),
 .UNSPECIFIED.) ;
#1461=B_SPLINE_CURVE_WITH_KNOTS('',3,(#68897,#68898,#68899,#68900),
 .UNSPECIFIED.,.F.,.F.,(4,4),(-0.0139707365649134,0.),.UNSPECIFIED.) ;
#1462=B_SPLINE_CURVE_WITH_KNOTS('',3,(#68993,#68994,#68995,#68996,#68997,
#68998,#68999,#69000,#69001,#69002,#69003,#69004,#69005,#69006,#69007,#69008,
#69009,#69010,#69011,#69012,#69013,#69014,#69015,#69016,#69017,#69018,#69019,
#69020,#69021,#69022,#69023,#69024,#69025,#69026,#69027,#69028,#69029,#69030,
#69031,#69032,#69033,#69034,#69035,#69036,#69037,#69038,#69039,#69040,#69041,
#69042,#69043,#69044,#69045,#69046,#69047,#69048,#69049,#69050,#69051,#69052,
#69053,#69054,#69055,#69056,#69057,#69058,#69059,#69060,#69061,#69062,#69063,
#69064,#69065,#69066,#69067,#69068,#69069,#69070,#69071,#69072,#69073,#69074),
 .UNSPECIFIED.,.F.,.F.,(4,3,3,3,3,3,3,3,3,3,3,3,3,3,3,3,3,3,3,3,3,3,3,3,
3,3,3,4),(0.,0.0185725445526958,0.0384193594961247,0.055785322571625,0.0645115507874783,
0.0684603398259577,0.088496523143581,0.108897436913417,0.126009843710094,
0.133915126485099,0.137321203268634,0.158395989100451,0.177347064100127,
0.197886255284734,0.205726139725896,0.209179066906955,0.230196165737754,
0.251694764126909,0.267939537662014,0.278006078980002,0.28185525752262,
0.304704366858893,0.321841198861098,0.327919839794464,0.332524028582538,
0.355049411823982,0.373251694867712,0.376838226244513),.UNSPECIFIED.) ;
#1463=B_SPLINE_CURVE_WITH_KNOTS('',3,(#69168,#69169,#69170,#69171,#69172,
#69173,#69174,#69175,#69176,#69177,#69178,#69179,#69180,#69181,#69182,#69183,
#69184,#69185,#69186,#69187,#69188,#69189,#69190,#69191,#69192,#69193,#69194,
#69195,#69196,#69197,#69198,#69199,#69200,#69201,#69202,#69203,#69204,#69205,
#69206,#69207,#69208,#69209,#69210,#69211,#69212,#69213,#69214,#69215,#69216,
#69217,#69218,#69219,#69220,#69221,#69222,#69223,#69224,#69225,#69226,#69227,
#69228,#69229,#69230,#69231,#69232,#69233,#69234,#69235,#69236,#69237,#69238,
#69239,#69240,#69241,#69242,#69243,#69244,#69245,#69246,#69247,#69248,#69249,
#69250,#69251,#69252,#69253,#69254,#69255),.UNSPECIFIED.,.F.,.F.,(4,3,3,
3,3,3,3,3,3,3,3,3,3,3,3,3,3,3,3,3,3,3,3,3,3,3,3,3,3,4),(0.,0.0219449640383438,
0.0445193578452532,0.0636177263807443,0.0720881957929118,0.0767288071884963,
0.081042586603963,0.102988523783161,0.124769865235439,0.142903975458875,
0.150434676914754,0.153946737722924,0.157570423195002,0.178344835982706,
0.197306306129181,0.219592370861987,0.224535999451756,0.229375735630213,
0.250039068191406,0.270699864974871,0.285804475544972,0.29205042217151,
0.296686337413507,0.300587110169541,0.320413064822319,0.334366467704069,
0.338839477396653,0.357868249441859,0.375594823991625,0.378621596831076),
 .UNSPECIFIED.) ;
#1464=B_SPLINE_CURVE_WITH_KNOTS('',3,(#69256,#69257,#69258,#69259),
 .UNSPECIFIED.,.F.,.F.,(4,4),(-0.013970623523499,0.),.UNSPECIFIED.) ;
#1779=PLANE('',#33320) ;
#1780=PLANE('',#33330) ;
#1781=PLANE('',#33340) ;
#1782=PLANE('',#33353) ;
#1783=PLANE('',#33360) ;
#1784=PLANE('',#33373) ;
#1785=PLANE('',#33375) ;
#1786=PLANE('',#33385) ;
#1787=PLANE('',#33386) ;
#1788=PLANE('',#33387) ;
#1789=PLANE('',#33388) ;
#1790=PLANE('',#33389) ;
#1791=PLANE('',#33390) ;
#1792=PLANE('',#33392) ;
#1793=PLANE('',#33393) ;
#1794=PLANE('',#33394) ;
#1795=PLANE('',#33395) ;
#1796=PLANE('',#33399) ;
#1797=PLANE('',#33413) ;
#1798=PLANE('',#33416) ;
#1799=PLANE('',#33419) ;
#1800=PLANE('',#33433) ;
#1801=PLANE('',#33436) ;
#1802=PLANE('',#33439) ;
#1803=PLANE('',#33440) ;
#1804=PLANE('',#33441) ;
#1805=PLANE('',#33442) ;
#1806=PLANE('',#33443) ;
#1807=PLANE('',#33444) ;
#1808=PLANE('',#33445) ;
#1809=PLANE('',#33446) ;
#1810=PLANE('',#33447) ;
#1811=PLANE('',#33448) ;
#1812=PLANE('',#33449) ;
#1813=PLANE('',#33450) ;
#1814=PLANE('',#33451) ;
#1815=PLANE('',#33452) ;
#1816=PLANE('',#33453) ;
#1817=PLANE('',#33468) ;
#1818=PLANE('',#33478) ;
#1819=PLANE('',#33480) ;
#1820=PLANE('',#33515) ;
#1821=PLANE('',#33517) ;
#1822=PLANE('',#33518) ;
#1823=PLANE('',#33519) ;
#1824=PLANE('',#33520) ;
#1825=PLANE('',#33521) ;
#1826=PLANE('',#33522) ;
#1827=PLANE('',#33523) ;
#1828=PLANE('',#33524) ;
#1829=PLANE('',#33525) ;
#1830=PLANE('',#33526) ;
#1831=PLANE('',#33527) ;
#1832=PLANE('',#33528) ;
#1833=PLANE('',#33529) ;
#1834=PLANE('',#33531) ;
#1835=PLANE('',#33532) ;
#1836=PLANE('',#33533) ;
#1837=PLANE('',#33534) ;
#1838=PLANE('',#33535) ;
#1839=PLANE('',#33537) ;
#1840=PLANE('',#33543) ;
#1841=PLANE('',#33553) ;
#1842=PLANE('',#33554) ;
#1843=PLANE('',#33555) ;
#1844=PLANE('',#33556) ;
#1845=PLANE('',#33557) ;
#1846=PLANE('',#33564) ;
#1847=PLANE('',#33587) ;
#1848=PLANE('',#33588) ;
#1849=PLANE('',#33590) ;
#1850=PLANE('',#33592) ;
#1851=PLANE('',#33594) ;
#1852=PLANE('',#33595) ;
#1853=PLANE('',#33596) ;
#1854=PLANE('',#33597) ;
#1855=PLANE('',#33598) ;
#1856=PLANE('',#33599) ;
#1857=PLANE('',#33602) ;
#1858=PLANE('',#33603) ;
#1859=PLANE('',#33606) ;
#1860=PLANE('',#33607) ;
#1861=PLANE('',#33608) ;
#1862=PLANE('',#33609) ;
#1863=PLANE('',#33610) ;
#1864=PLANE('',#33611) ;
#1865=PLANE('',#33612) ;
#1866=PLANE('',#33613) ;
#1867=PLANE('',#33623) ;
#1868=PLANE('',#33626) ;
#1869=PLANE('',#33631) ;
#1870=PLANE('',#33636) ;
#1871=PLANE('',#33637) ;
#1872=PLANE('',#33638) ;
#1873=PLANE('',#33639) ;
#1874=PLANE('',#33664) ;
#1875=PLANE('',#33667) ;
#1876=PLANE('',#33671) ;
#1877=PLANE('',#33678) ;
#1878=PLANE('',#33684) ;
#1879=PLANE('',#33692) ;
#1880=PLANE('',#33693) ;
#1881=PLANE('',#33694) ;
#1882=PLANE('',#33695) ;
#1883=PLANE('',#33696) ;
#1884=PLANE('',#33697) ;
#1885=PLANE('',#33698) ;
#1886=PLANE('',#33699) ;
#1887=PLANE('',#33700) ;
#1888=PLANE('',#33701) ;
#1889=PLANE('',#33702) ;
#1890=PLANE('',#33703) ;
#1891=PLANE('',#33704) ;
#1892=PLANE('',#33705) ;
#1893=PLANE('',#33706) ;
#1894=PLANE('',#33707) ;
#1895=PLANE('',#33708) ;
#1896=PLANE('',#33709) ;
#1897=PLANE('',#33710) ;
#1898=PLANE('',#33711) ;
#2479=FACE_OUTER_BOUND('',#4418,.T.) ;
#2480=FACE_OUTER_BOUND('',#4419,.T.) ;
#2481=FACE_OUTER_BOUND('',#4420,.T.) ;
#2482=FACE_OUTER_BOUND('',#4421,.T.) ;
#2483=FACE_OUTER_BOUND('',#4422,.T.) ;
#2484=FACE_OUTER_BOUND('',#4423,.T.) ;
#2485=FACE_OUTER_BOUND('',#4424,.T.) ;
#2486=FACE_OUTER_BOUND('',#4425,.T.) ;
#2487=FACE_OUTER_BOUND('',#4426,.T.) ;
#2488=FACE_OUTER_BOUND('',#4427,.T.) ;
#2489=FACE_OUTER_BOUND('',#4428,.T.) ;
#2490=FACE_OUTER_BOUND('',#4429,.T.) ;
#2491=FACE_OUTER_BOUND('',#4430,.T.) ;
#2492=FACE_OUTER_BOUND('',#4431,.T.) ;
#2493=FACE_OUTER_BOUND('',#4432,.T.) ;
#2494=FACE_OUTER_BOUND('',#4433,.T.) ;
#2495=FACE_OUTER_BOUND('',#4434,.T.) ;
#2496=FACE_OUTER_BOUND('',#4435,.T.) ;
#2497=FACE_OUTER_BOUND('',#4436,.T.) ;
#2498=FACE_OUTER_BOUND('',#4437,.T.) ;
#2499=FACE_OUTER_BOUND('',#4438,.T.) ;
#2500=FACE_OUTER_BOUND('',#4439,.T.) ;
#2501=FACE_OUTER_BOUND('',#4440,.T.) ;
#2502=FACE_OUTER_BOUND('',#4441,.T.) ;
#2503=FACE_OUTER_BOUND('',#4442,.T.) ;
#2504=FACE_OUTER_BOUND('',#4443,.T.) ;
#2505=FACE_OUTER_BOUND('',#4444,.T.) ;
#2506=FACE_OUTER_BOUND('',#4445,.T.) ;
#2507=FACE_OUTER_BOUND('',#4446,.T.) ;
#2508=FACE_OUTER_BOUND('',#4447,.T.) ;
#2509=FACE_OUTER_BOUND('',#4448,.T.) ;
#2510=FACE_OUTER_BOUND('',#4449,.T.) ;
#2511=FACE_OUTER_BOUND('',#4450,.T.) ;
#2512=FACE_OUTER_BOUND('',#4451,.T.) ;
#2513=FACE_OUTER_BOUND('',#4452,.T.) ;
#2514=FACE_OUTER_BOUND('',#4453,.T.) ;
#2515=FACE_OUTER_BOUND('',#4454,.T.) ;
#2516=FACE_OUTER_BOUND('',#4455,.T.) ;
#2517=FACE_OUTER_BOUND('',#4456,.T.) ;
#2518=FACE_OUTER_BOUND('',#4457,.T.) ;
#2519=FACE_OUTER_BOUND('',#4458,.T.) ;
#2520=FACE_OUTER_BOUND('',#4459,.T.) ;
#2521=FACE_OUTER_BOUND('',#4460,.T.) ;
#2522=FACE_OUTER_BOUND('',#4461,.T.) ;
#2523=FACE_OUTER_BOUND('',#4462,.T.) ;
#2524=FACE_OUTER_BOUND('',#4463,.T.) ;
#2525=FACE_OUTER_BOUND('',#4464,.T.) ;
#2526=FACE_OUTER_BOUND('',#4465,.T.) ;
#2527=FACE_OUTER_BOUND('',#4466,.T.) ;
#2528=FACE_OUTER_BOUND('',#4467,.T.) ;
#2529=FACE_OUTER_BOUND('',#4468,.T.) ;
#2530=FACE_OUTER_BOUND('',#4469,.T.) ;
#2531=FACE_OUTER_BOUND('',#4470,.T.) ;
#2532=FACE_OUTER_BOUND('',#4471,.T.) ;
#2533=FACE_OUTER_BOUND('',#4472,.T.) ;
#2534=FACE_OUTER_BOUND('',#4473,.T.) ;
#2535=FACE_OUTER_BOUND('',#4474,.T.) ;
#2536=FACE_OUTER_BOUND('',#4475,.T.) ;
#2537=FACE_OUTER_BOUND('',#4476,.T.) ;
#2538=FACE_OUTER_BOUND('',#4477,.T.) ;
#2539=FACE_OUTER_BOUND('',#4478,.T.) ;
#2540=FACE_OUTER_BOUND('',#4479,.T.) ;
#2541=FACE_OUTER_BOUND('',#4480,.T.) ;
#2542=FACE_OUTER_BOUND('',#4481,.T.) ;
#2543=FACE_OUTER_BOUND('',#4482,.T.) ;
#2544=FACE_OUTER_BOUND('',#4483,.T.) ;
#2545=FACE_OUTER_BOUND('',#4484,.T.) ;
#2546=FACE_OUTER_BOUND('',#4485,.T.) ;
#2547=FACE_OUTER_BOUND('',#4486,.T.) ;
#2548=FACE_OUTER_BOUND('',#4487,.T.) ;
#2549=FACE_OUTER_BOUND('',#4488,.T.) ;
#2550=FACE_OUTER_BOUND('',#4489,.T.) ;
#2551=FACE_OUTER_BOUND('',#4490,.T.) ;
#2552=FACE_OUTER_BOUND('',#4499,.T.) ;
#2553=FACE_OUTER_BOUND('',#4500,.T.) ;
#2554=FACE_OUTER_BOUND('',#4511,.T.) ;
#2555=FACE_OUTER_BOUND('',#4520,.T.) ;
#2556=FACE_OUTER_BOUND('',#4531,.T.) ;
#2557=FACE_OUTER_BOUND('',#4532,.T.) ;
#2558=FACE_OUTER_BOUND('',#4533,.T.) ;
#2559=FACE_OUTER_BOUND('',#4534,.T.) ;
#2560=FACE_OUTER_BOUND('',#4535,.T.) ;
#2561=FACE_OUTER_BOUND('',#4536,.T.) ;
#2562=FACE_OUTER_BOUND('',#4537,.T.) ;
#2563=FACE_OUTER_BOUND('',#4538,.T.) ;
#2564=FACE_OUTER_BOUND('',#4539,.T.) ;
#2565=FACE_OUTER_BOUND('',#4540,.T.) ;
#2566=FACE_OUTER_BOUND('',#4541,.T.) ;
#2567=FACE_OUTER_BOUND('',#4542,.T.) ;
#2568=FACE_OUTER_BOUND('',#4543,.T.) ;
#2569=FACE_OUTER_BOUND('',#4544,.T.) ;
#2570=FACE_OUTER_BOUND('',#4545,.T.) ;
#2571=FACE_OUTER_BOUND('',#4546,.T.) ;
#2572=FACE_OUTER_BOUND('',#4547,.T.) ;
#2573=FACE_OUTER_BOUND('',#4548,.T.) ;
#2574=FACE_OUTER_BOUND('',#4549,.T.) ;
#2575=FACE_OUTER_BOUND('',#4550,.T.) ;
#2576=FACE_OUTER_BOUND('',#4551,.T.) ;
#2577=FACE_OUTER_BOUND('',#4552,.T.) ;
#2578=FACE_OUTER_BOUND('',#4553,.T.) ;
#2579=FACE_OUTER_BOUND('',#4554,.T.) ;
#2580=FACE_OUTER_BOUND('',#4555,.T.) ;
#2581=FACE_OUTER_BOUND('',#4556,.T.) ;
#2582=FACE_OUTER_BOUND('',#4557,.T.) ;
#2583=FACE_OUTER_BOUND('',#4558,.T.) ;
#2584=FACE_OUTER_BOUND('',#4559,.T.) ;
#2585=FACE_OUTER_BOUND('',#4560,.T.) ;
#2586=FACE_OUTER_BOUND('',#4561,.T.) ;
#2587=FACE_OUTER_BOUND('',#4562,.T.) ;
#2588=FACE_OUTER_BOUND('',#4563,.T.) ;
#2589=FACE_OUTER_BOUND('',#4564,.T.) ;
#2590=FACE_OUTER_BOUND('',#4565,.T.) ;
#2591=FACE_OUTER_BOUND('',#4566,.T.) ;
#2592=FACE_OUTER_BOUND('',#4567,.T.) ;
#2593=FACE_OUTER_BOUND('',#4568,.T.) ;
#2594=FACE_OUTER_BOUND('',#4569,.T.) ;
#2595=FACE_OUTER_BOUND('',#4570,.T.) ;
#2596=FACE_OUTER_BOUND('',#4571,.T.) ;
#2597=FACE_OUTER_BOUND('',#4572,.T.) ;
#2598=FACE_OUTER_BOUND('',#4573,.T.) ;
#2599=FACE_OUTER_BOUND('',#4574,.T.) ;
#2600=FACE_OUTER_BOUND('',#4575,.T.) ;
#2601=FACE_OUTER_BOUND('',#4576,.T.) ;
#2602=FACE_OUTER_BOUND('',#4577,.T.) ;
#2603=FACE_OUTER_BOUND('',#4578,.T.) ;
#2604=FACE_OUTER_BOUND('',#4579,.T.) ;
#2605=FACE_OUTER_BOUND('',#4580,.T.) ;
#2606=FACE_OUTER_BOUND('',#4581,.T.) ;
#2607=FACE_OUTER_BOUND('',#4582,.T.) ;
#2608=FACE_OUTER_BOUND('',#4583,.T.) ;
#2609=FACE_OUTER_BOUND('',#4584,.T.) ;
#2610=FACE_OUTER_BOUND('',#4585,.T.) ;
#2611=FACE_OUTER_BOUND('',#4586,.T.) ;
#2612=FACE_OUTER_BOUND('',#4587,.T.) ;
#2613=FACE_OUTER_BOUND('',#4588,.T.) ;
#2614=FACE_OUTER_BOUND('',#4589,.T.) ;
#2615=FACE_OUTER_BOUND('',#4590,.T.) ;
#2616=FACE_OUTER_BOUND('',#4591,.T.) ;
#2617=FACE_OUTER_BOUND('',#4592,.T.) ;
#2618=FACE_OUTER_BOUND('',#4593,.T.) ;
#2619=FACE_OUTER_BOUND('',#4594,.T.) ;
#2620=FACE_OUTER_BOUND('',#4595,.T.) ;
#2621=FACE_OUTER_BOUND('',#4596,.T.) ;
#2622=FACE_OUTER_BOUND('',#4597,.T.) ;
#2623=FACE_OUTER_BOUND('',#4598,.T.) ;
#2624=FACE_OUTER_BOUND('',#4599,.T.) ;
#2625=FACE_OUTER_BOUND('',#4600,.T.) ;
#2626=FACE_OUTER_BOUND('',#4601,.T.) ;
#2627=FACE_OUTER_BOUND('',#4602,.T.) ;
#2628=FACE_OUTER_BOUND('',#4603,.T.) ;
#2629=FACE_OUTER_BOUND('',#4604,.T.) ;
#2630=FACE_OUTER_BOUND('',#4605,.T.) ;
#2631=FACE_OUTER_BOUND('',#4606,.T.) ;
#2632=FACE_OUTER_BOUND('',#4607,.T.) ;
#2633=FACE_OUTER_BOUND('',#4608,.T.) ;
#2634=FACE_OUTER_BOUND('',#4609,.T.) ;
#2635=FACE_OUTER_BOUND('',#4610,.T.) ;
#2636=FACE_OUTER_BOUND('',#4611,.T.) ;
#2637=FACE_OUTER_BOUND('',#4612,.T.) ;
#2638=FACE_OUTER_BOUND('',#4613,.T.) ;
#2639=FACE_OUTER_BOUND('',#4614,.T.) ;
#2640=FACE_OUTER_BOUND('',#4615,.T.) ;
#2641=FACE_OUTER_BOUND('',#4616,.T.) ;
#2642=FACE_OUTER_BOUND('',#4617,.T.) ;
#2643=FACE_OUTER_BOUND('',#4618,.T.) ;
#2644=FACE_OUTER_BOUND('',#4619,.T.) ;
#2645=FACE_OUTER_BOUND('',#4620,.T.) ;
#2646=FACE_OUTER_BOUND('',#4621,.T.) ;
#2647=FACE_OUTER_BOUND('',#4622,.T.) ;
#2648=FACE_OUTER_BOUND('',#4623,.T.) ;
#2649=FACE_OUTER_BOUND('',#4624,.T.) ;
#2650=FACE_OUTER_BOUND('',#4625,.T.) ;
#2651=FACE_OUTER_BOUND('',#4626,.T.) ;
#2652=FACE_OUTER_BOUND('',#4627,.T.) ;
#2653=FACE_OUTER_BOUND('',#4628,.T.) ;
#2654=FACE_OUTER_BOUND('',#4629,.T.) ;
#2655=FACE_OUTER_BOUND('',#4630,.T.) ;
#2656=FACE_OUTER_BOUND('',#4631,.T.) ;
#2657=FACE_OUTER_BOUND('',#4632,.T.) ;
#2658=FACE_OUTER_BOUND('',#4633,.T.) ;
#2659=FACE_OUTER_BOUND('',#4634,.T.) ;
#2660=FACE_OUTER_BOUND('',#4635,.T.) ;
#2661=FACE_OUTER_BOUND('',#4636,.T.) ;
#2662=FACE_OUTER_BOUND('',#4637,.T.) ;
#2663=FACE_OUTER_BOUND('',#4638,.T.) ;
#2664=FACE_OUTER_BOUND('',#4639,.T.) ;
#2665=FACE_OUTER_BOUND('',#4640,.T.) ;
#2666=FACE_OUTER_BOUND('',#4641,.T.) ;
#2667=FACE_OUTER_BOUND('',#4642,.T.) ;
#2668=FACE_OUTER_BOUND('',#4643,.T.) ;
#2669=FACE_OUTER_BOUND('',#4648,.T.) ;
#2670=FACE_OUTER_BOUND('',#4649,.T.) ;
#2671=FACE_OUTER_BOUND('',#4650,.T.) ;
#2672=FACE_OUTER_BOUND('',#4651,.T.) ;
#2673=FACE_OUTER_BOUND('',#4652,.T.) ;
#2674=FACE_OUTER_BOUND('',#4653,.T.) ;
#2675=FACE_OUTER_BOUND('',#4654,.T.) ;
#2676=FACE_OUTER_BOUND('',#4655,.T.) ;
#2677=FACE_OUTER_BOUND('',#4656,.T.) ;
#2678=FACE_OUTER_BOUND('',#4657,.T.) ;
#2679=FACE_OUTER_BOUND('',#4658,.T.) ;
#2680=FACE_OUTER_BOUND('',#4659,.T.) ;
#2681=FACE_OUTER_BOUND('',#4660,.T.) ;
#2682=FACE_OUTER_BOUND('',#4661,.T.) ;
#2683=FACE_OUTER_BOUND('',#4662,.T.) ;
#2684=FACE_OUTER_BOUND('',#4663,.T.) ;
#2685=FACE_OUTER_BOUND('',#4664,.T.) ;
#2686=FACE_OUTER_BOUND('',#4665,.T.) ;
#2687=FACE_OUTER_BOUND('',#4666,.T.) ;
#2688=FACE_OUTER_BOUND('',#4667,.T.) ;
#2689=FACE_OUTER_BOUND('',#4668,.T.) ;
#2690=FACE_OUTER_BOUND('',#4669,.T.) ;
#2691=FACE_OUTER_BOUND('',#4670,.T.) ;
#2692=FACE_OUTER_BOUND('',#4671,.T.) ;
#2693=FACE_OUTER_BOUND('',#4672,.T.) ;
#2694=FACE_OUTER_BOUND('',#4673,.T.) ;
#2695=FACE_OUTER_BOUND('',#4674,.T.) ;
#2696=FACE_OUTER_BOUND('',#4675,.T.) ;
#2697=FACE_OUTER_BOUND('',#4676,.T.) ;
#2698=FACE_OUTER_BOUND('',#4677,.T.) ;
#2699=FACE_OUTER_BOUND('',#4678,.T.) ;
#2700=FACE_OUTER_BOUND('',#4679,.T.) ;
#2701=FACE_OUTER_BOUND('',#4680,.T.) ;
#2702=FACE_OUTER_BOUND('',#4681,.T.) ;
#2703=FACE_OUTER_BOUND('',#4682,.T.) ;
#2704=FACE_OUTER_BOUND('',#4683,.T.) ;
#2705=FACE_OUTER_BOUND('',#4684,.T.) ;
#2706=FACE_OUTER_BOUND('',#4685,.T.) ;
#2707=FACE_OUTER_BOUND('',#4686,.T.) ;
#2708=FACE_OUTER_BOUND('',#4687,.T.) ;
#2709=FACE_OUTER_BOUND('',#4688,.T.) ;
#2710=FACE_OUTER_BOUND('',#4690,.T.) ;
#2711=FACE_OUTER_BOUND('',#4691,.T.) ;
#2712=FACE_OUTER_BOUND('',#4692,.T.) ;
#2713=FACE_OUTER_BOUND('',#4693,.T.) ;
#2714=FACE_OUTER_BOUND('',#4694,.T.) ;
#2715=FACE_OUTER_BOUND('',#4695,.T.) ;
#2716=FACE_OUTER_BOUND('',#4696,.T.) ;
#2717=FACE_OUTER_BOUND('',#4697,.T.) ;
#2718=FACE_OUTER_BOUND('',#4698,.T.) ;
#2719=FACE_OUTER_BOUND('',#4699,.T.) ;
#2720=FACE_OUTER_BOUND('',#4700,.T.) ;
#2721=FACE_OUTER_BOUND('',#4701,.T.) ;
#2722=FACE_OUTER_BOUND('',#4702,.T.) ;
#2723=FACE_OUTER_BOUND('',#4703,.T.) ;
#2724=FACE_OUTER_BOUND('',#4704,.T.) ;
#2725=FACE_OUTER_BOUND('',#4705,.T.) ;
#2726=FACE_OUTER_BOUND('',#4706,.T.) ;
#2727=FACE_OUTER_BOUND('',#4707,.T.) ;
#2728=FACE_OUTER_BOUND('',#4708,.T.) ;
#2729=FACE_OUTER_BOUND('',#4709,.T.) ;
#2730=FACE_OUTER_BOUND('',#4710,.T.) ;
#2731=FACE_OUTER_BOUND('',#4711,.T.) ;
#2732=FACE_OUTER_BOUND('',#4712,.T.) ;
#2733=FACE_OUTER_BOUND('',#4713,.T.) ;
#2734=FACE_OUTER_BOUND('',#4714,.T.) ;
#2735=FACE_OUTER_BOUND('',#4715,.T.) ;
#2736=FACE_OUTER_BOUND('',#4716,.T.) ;
#2737=FACE_OUTER_BOUND('',#4717,.T.) ;
#2738=FACE_OUTER_BOUND('',#4718,.T.) ;
#2739=FACE_OUTER_BOUND('',#4719,.T.) ;
#2740=FACE_OUTER_BOUND('',#4720,.T.) ;
#2741=FACE_OUTER_BOUND('',#4721,.T.) ;
#2742=FACE_OUTER_BOUND('',#4722,.T.) ;
#2743=FACE_OUTER_BOUND('',#4723,.T.) ;
#2744=FACE_OUTER_BOUND('',#4728,.T.) ;
#2745=FACE_OUTER_BOUND('',#4729,.T.) ;
#2746=FACE_OUTER_BOUND('',#4730,.T.) ;
#2747=FACE_OUTER_BOUND('',#4731,.T.) ;
#2748=FACE_OUTER_BOUND('',#4733,.T.) ;
#2749=FACE_OUTER_BOUND('',#4734,.T.) ;
#2750=FACE_OUTER_BOUND('',#4735,.T.) ;
#2751=FACE_OUTER_BOUND('',#4736,.T.) ;
#2752=FACE_OUTER_BOUND('',#4737,.T.) ;
#2753=FACE_OUTER_BOUND('',#4738,.T.) ;
#2754=FACE_OUTER_BOUND('',#4739,.T.) ;
#2755=FACE_OUTER_BOUND('',#4740,.T.) ;
#2756=FACE_OUTER_BOUND('',#4741,.T.) ;
#2757=FACE_OUTER_BOUND('',#4742,.T.) ;
#2758=FACE_OUTER_BOUND('',#4743,.T.) ;
#2759=FACE_OUTER_BOUND('',#4753,.T.) ;
#2760=FACE_OUTER_BOUND('',#4754,.T.) ;
#2761=FACE_OUTER_BOUND('',#4755,.T.) ;
#2762=FACE_OUTER_BOUND('',#4756,.T.) ;
#2763=FACE_OUTER_BOUND('',#4757,.T.) ;
#2764=FACE_OUTER_BOUND('',#4758,.T.) ;
#2765=FACE_OUTER_BOUND('',#4759,.T.) ;
#2766=FACE_OUTER_BOUND('',#4760,.T.) ;
#2767=FACE_OUTER_BOUND('',#4761,.T.) ;
#2768=FACE_OUTER_BOUND('',#4762,.T.) ;
#2769=FACE_OUTER_BOUND('',#4763,.T.) ;
#2770=FACE_OUTER_BOUND('',#4764,.T.) ;
#2771=FACE_OUTER_BOUND('',#4765,.T.) ;
#2772=FACE_OUTER_BOUND('',#4766,.T.) ;
#2773=FACE_OUTER_BOUND('',#4767,.T.) ;
#2774=FACE_OUTER_BOUND('',#4777,.T.) ;
#2775=FACE_OUTER_BOUND('',#4778,.T.) ;
#2776=FACE_OUTER_BOUND('',#4779,.T.) ;
#2777=FACE_OUTER_BOUND('',#4780,.T.) ;
#2778=FACE_OUTER_BOUND('',#4781,.T.) ;
#2779=FACE_OUTER_BOUND('',#4782,.T.) ;
#4418=EDGE_LOOP('',(#21550,#21551,#21552,#21553)) ;
#4419=EDGE_LOOP('',(#21554,#21555,#21556,#21557,#21558)) ;
#4420=EDGE_LOOP('',(#21559,#21560,#21561,#21562,#21563)) ;
#4421=EDGE_LOOP('',(#21564,#21565,#21566,#21567)) ;
#4422=EDGE_LOOP('',(#21568,#21569,#21570,#21571,#21572,#21573)) ;
#4423=EDGE_LOOP('',(#21574,#21575,#21576,#21577,#21578,#21579,#21580)) ;
#4424=EDGE_LOOP('',(#21581,#21582,#21583,#21584)) ;
#4425=EDGE_LOOP('',(#21585,#21586,#21587,#21588,#21589)) ;
#4426=EDGE_LOOP('',(#21590,#21591,#21592,#21593,#21594,#21595)) ;
#4427=EDGE_LOOP('',(#21596,#21597,#21598,#21599)) ;
#4428=EDGE_LOOP('',(#21600,#21601,#21602,#21603,#21604)) ;
#4429=EDGE_LOOP('',(#21605,#21606,#21607,#21608,#21609)) ;
#4430=EDGE_LOOP('',(#21610,#21611,#21612)) ;
#4431=EDGE_LOOP('',(#21613,#21614,#21615,#21616,#21617)) ;
#4432=EDGE_LOOP('',(#21618,#21619,#21620,#21621,#21622,#21623)) ;
#4433=EDGE_LOOP('',(#21624,#21625,#21626)) ;
#4434=EDGE_LOOP('',(#21627,#21628,#21629,#21630,#21631)) ;
#4435=EDGE_LOOP('',(#21632,#21633,#21634,#21635,#21636,#21637)) ;
#4436=EDGE_LOOP('',(#21638,#21639,#21640)) ;
#4437=EDGE_LOOP('',(#21641,#21642,#21643,#21644,#21645)) ;
#4438=EDGE_LOOP('',(#21646,#21647,#21648,#21649,#21650,#21651)) ;
#4439=EDGE_LOOP('',(#21652,#21653,#21654)) ;
#4440=EDGE_LOOP('',(#21655,#21656,#21657,#21658,#21659)) ;
#4441=EDGE_LOOP('',(#21660,#21661,#21662,#21663,#21664,#21665)) ;
#4442=EDGE_LOOP('',(#21666,#21667,#21668,#21669)) ;
#4443=EDGE_LOOP('',(#21670,#21671,#21672,#21673,#21674)) ;
#4444=EDGE_LOOP('',(#21675,#21676,#21677,#21678,#21679)) ;
#4445=EDGE_LOOP('',(#21680,#21681,#21682,#21683)) ;
#4446=EDGE_LOOP('',(#21684,#21685,#21686,#21687,#21688)) ;
#4447=EDGE_LOOP('',(#21689,#21690,#21691,#21692,#21693,#21694)) ;
#4448=EDGE_LOOP('',(#21695,#21696,#21697)) ;
#4449=EDGE_LOOP('',(#21698,#21699,#21700,#21701,#21702)) ;
#4450=EDGE_LOOP('',(#21703,#21704,#21705,#21706,#21707,#21708)) ;
#4451=EDGE_LOOP('',(#21709,#21710,#21711)) ;
#4452=EDGE_LOOP('',(#21712,#21713,#21714,#21715,#21716)) ;
#4453=EDGE_LOOP('',(#21717,#21718,#21719,#21720,#21721,#21722)) ;
#4454=EDGE_LOOP('',(#21723,#21724,#21725,#21726)) ;
#4455=EDGE_LOOP('',(#21727,#21728,#21729,#21730,#21731)) ;
#4456=EDGE_LOOP('',(#21732,#21733,#21734,#21735,#21736)) ;
#4457=EDGE_LOOP('',(#21737,#21738,#21739,#21740)) ;
#4458=EDGE_LOOP('',(#21741,#21742,#21743,#21744,#21745)) ;
#4459=EDGE_LOOP('',(#21746,#21747,#21748,#21749,#21750)) ;
#4460=EDGE_LOOP('',(#21751,#21752,#21753)) ;
#4461=EDGE_LOOP('',(#21754,#21755,#21756,#21757,#21758)) ;
#4462=EDGE_LOOP('',(#21759,#21760,#21761,#21762,#21763,#21764)) ;
#4463=EDGE_LOOP('',(#21765,#21766,#21767)) ;
#4464=EDGE_LOOP('',(#21768,#21769,#21770,#21771,#21772)) ;
#4465=EDGE_LOOP('',(#21773,#21774,#21775,#21776,#21777,#21778)) ;
#4466=EDGE_LOOP('',(#21779,#21780,#21781,#21782)) ;
#4467=EDGE_LOOP('',(#21783,#21784,#21785,#21786)) ;
#4468=EDGE_LOOP('',(#21787,#21788,#21789,#21790)) ;
#4469=EDGE_LOOP('',(#21791,#21792,#21793,#21794)) ;
#4470=EDGE_LOOP('',(#21795,#21796,#21797,#21798)) ;
#4471=EDGE_LOOP('',(#21799,#21800,#21801,#21802)) ;
#4472=EDGE_LOOP('',(#21803,#21804,#21805,#21806,#21807)) ;
#4473=EDGE_LOOP('',(#21808,#21809,#21810,#21811)) ;
#4474=EDGE_LOOP('',(#21812,#21813,#21814,#21815)) ;
#4475=EDGE_LOOP('',(#21816,#21817,#21818,#21819)) ;
#4476=EDGE_LOOP('',(#21820,#21821,#21822,#21823)) ;
#4477=EDGE_LOOP('',(#21824,#21825,#21826,#21827)) ;
#4478=EDGE_LOOP('',(#21828,#21829,#21830,#21831)) ;
#4479=EDGE_LOOP('',(#21832,#21833,#21834,#21835,#21836)) ;
#4480=EDGE_LOOP('',(#21837,#21838,#21839,#21840)) ;
#4481=EDGE_LOOP('',(#21841,#21842,#21843,#21844)) ;
#4482=EDGE_LOOP('',(#21845,#21846,#21847,#21848)) ;
#4483=EDGE_LOOP('',(#21849,#21850,#21851,#21852)) ;
#4484=EDGE_LOOP('',(#21853,#21854,#21855,#21856)) ;
#4485=EDGE_LOOP('',(#21857,#21858,#21859,#21860)) ;
#4486=EDGE_LOOP('',(#21861,#21862,#21863,#21864)) ;
#4487=EDGE_LOOP('',(#21865,#21866,#21867,#21868,#21869,#21870,#21871,#21872,
#21873,#21874,#21875,#21876)) ;
#4488=EDGE_LOOP('',(#21877,#21878,#21879,#21880)) ;
#4489=EDGE_LOOP('',(#21881,#21882,#21883,#21884)) ;
#4490=EDGE_LOOP('',(#21885,#21886,#21887,#21888,#21889,#21890,#21891,#21892,
#21893,#21894,#21895,#21896,#21897,#21898,#21899,#21900)) ;
#4491=EDGE_LOOP('',(#21901,#21902,#21903,#21904,#21905,#21906,#21907,#21908,
#21909,#21910,#21911,#21912,#21913,#21914)) ;
#4492=EDGE_LOOP('',(#21915,#21916,#21917,#21918,#21919,#21920)) ;
#4493=EDGE_LOOP('',(#21921,#21922,#21923,#21924,#21925,#21926)) ;
#4494=EDGE_LOOP('',(#21927)) ;
#4495=EDGE_LOOP('',(#21928,#21929,#21930,#21931)) ;
#4496=EDGE_LOOP('',(#21932,#21933,#21934,#21935)) ;
#4497=EDGE_LOOP('',(#21936,#21937,#21938,#21939)) ;
#4498=EDGE_LOOP('',(#21940)) ;
#4499=EDGE_LOOP('',(#21941,#21942,#21943,#21944)) ;
#4500=EDGE_LOOP('',(#21945,#21946,#21947,#21948,#21949,#21950,#21951,#21952,
#21953,#21954,#21955,#21956,#21957,#21958,#21959,#21960,#21961,#21962,#21963,
#21964,#21965,#21966,#21967,#21968)) ;
#4501=EDGE_LOOP('',(#21969)) ;
#4502=EDGE_LOOP('',(#21970,#21971,#21972,#21973)) ;
#4503=EDGE_LOOP('',(#21974,#21975,#21976,#21977)) ;
#4504=EDGE_LOOP('',(#21978,#21979,#21980,#21981)) ;
#4505=EDGE_LOOP('',(#21982,#21983,#21984,#21985)) ;
#4506=EDGE_LOOP('',(#21986)) ;
#4507=EDGE_LOOP('',(#21987,#21988,#21989,#21990,#21991,#21992)) ;
#4508=EDGE_LOOP('',(#21993,#21994,#21995,#21996,#21997,#21998)) ;
#4509=EDGE_LOOP('',(#21999,#22000,#22001,#22002,#22003,#22004,#22005,#22006)) ;
#4510=EDGE_LOOP('',(#22007,#22008,#22009,#22010,#22011,#22012,#22013,#22014,
#22015,#22016)) ;
#4511=EDGE_LOOP('',(#22017,#22018,#22019,#22020,#22021,#22022,#22023,#22024,
#22025,#22026,#22027,#22028,#22029,#22030,#22031,#22032)) ;
#4512=EDGE_LOOP('',(#22033)) ;
#4513=EDGE_LOOP('',(#22034,#22035,#22036,#22037)) ;
#4514=EDGE_LOOP('',(#22038,#22039,#22040,#22041)) ;
#4515=EDGE_LOOP('',(#22042,#22043,#22044,#22045)) ;
#4516=EDGE_LOOP('',(#22046,#22047,#22048,#22049,#22050,#22051)) ;
#4517=EDGE_LOOP('',(#22052)) ;
#4518=EDGE_LOOP('',(#22053,#22054,#22055,#22056,#22057)) ;
#4519=EDGE_LOOP('',(#22058,#22059,#22060,#22061,#22062)) ;
#4520=EDGE_LOOP('',(#22063,#22064,#22065,#22066,#22067,#22068,#22069,#22070,
#22071,#22072,#22073,#22074,#22075,#22076,#22077,#22078,#22079,#22080,#22081,
#22082,#22083,#22084,#22085,#22086)) ;
#4521=EDGE_LOOP('',(#22087,#22088,#22089,#22090,#22091,#22092,#22093,#22094)) ;
#4522=EDGE_LOOP('',(#22095,#22096,#22097,#22098,#22099)) ;
#4523=EDGE_LOOP('',(#22100,#22101,#22102,#22103,#22104)) ;
#4524=EDGE_LOOP('',(#22105,#22106,#22107,#22108,#22109,#22110)) ;
#4525=EDGE_LOOP('',(#22111,#22112,#22113,#22114)) ;
#4526=EDGE_LOOP('',(#22115,#22116,#22117,#22118)) ;
#4527=EDGE_LOOP('',(#22119,#22120,#22121,#22122)) ;
#4528=EDGE_LOOP('',(#22123,#22124,#22125,#22126)) ;
#4529=EDGE_LOOP('',(#22127)) ;
#4530=EDGE_LOOP('',(#22128)) ;
#4531=EDGE_LOOP('',(#22129,#22130,#22131,#22132,#22133,#22134,#22135,#22136)) ;
#4532=EDGE_LOOP('',(#22137,#22138,#22139,#22140,#22141,#22142,#22143,#22144)) ;
#4533=EDGE_LOOP('',(#22145,#22146,#22147,#22148)) ;
#4534=EDGE_LOOP('',(#22149,#22150,#22151,#22152)) ;
#4535=EDGE_LOOP('',(#22153,#22154,#22155,#22156)) ;
#4536=EDGE_LOOP('',(#22157,#22158,#22159,#22160)) ;
#4537=EDGE_LOOP('',(#22161,#22162,#22163,#22164)) ;
#4538=EDGE_LOOP('',(#22165,#22166,#22167,#22168)) ;
#4539=EDGE_LOOP('',(#22169,#22170,#22171,#22172)) ;
#4540=EDGE_LOOP('',(#22173,#22174,#22175,#22176)) ;
#4541=EDGE_LOOP('',(#22177,#22178,#22179,#22180)) ;
#4542=EDGE_LOOP('',(#22181,#22182,#22183,#22184,#22185,#22186,#22187)) ;
#4543=EDGE_LOOP('',(#22188,#22189,#22190,#22191,#22192,#22193,#22194,#22195)) ;
#4544=EDGE_LOOP('',(#22196,#22197,#22198,#22199)) ;
#4545=EDGE_LOOP('',(#22200,#22201,#22202,#22203)) ;
#4546=EDGE_LOOP('',(#22204,#22205,#22206,#22207,#22208,#22209,#22210)) ;
#4547=EDGE_LOOP('',(#22211,#22212,#22213,#22214)) ;
#4548=EDGE_LOOP('',(#22215,#22216,#22217,#22218)) ;
#4549=EDGE_LOOP('',(#22219,#22220,#22221,#22222)) ;
#4550=EDGE_LOOP('',(#22223,#22224,#22225,#22226)) ;
#4551=EDGE_LOOP('',(#22227,#22228,#22229,#22230)) ;
#4552=EDGE_LOOP('',(#22231,#22232,#22233,#22234)) ;
#4553=EDGE_LOOP('',(#22235,#22236,#22237,#22238)) ;
#4554=EDGE_LOOP('',(#22239,#22240,#22241,#22242)) ;
#4555=EDGE_LOOP('',(#22243,#22244,#22245,#22246)) ;
#4556=EDGE_LOOP('',(#22247,#22248,#22249,#22250)) ;
#4557=EDGE_LOOP('',(#22251,#22252,#22253,#22254)) ;
#4558=EDGE_LOOP('',(#22255,#22256,#22257,#22258)) ;
#4559=EDGE_LOOP('',(#22259,#22260,#22261,#22262)) ;
#4560=EDGE_LOOP('',(#22263,#22264,#22265,#22266)) ;
#4561=EDGE_LOOP('',(#22267,#22268,#22269,#22270)) ;
#4562=EDGE_LOOP('',(#22271,#22272,#22273,#22274)) ;
#4563=EDGE_LOOP('',(#22275,#22276,#22277,#22278)) ;
#4564=EDGE_LOOP('',(#22279,#22280,#22281,#22282)) ;
#4565=EDGE_LOOP('',(#22283,#22284,#22285,#22286)) ;
#4566=EDGE_LOOP('',(#22287,#22288,#22289,#22290)) ;
#4567=EDGE_LOOP('',(#22291,#22292,#22293,#22294)) ;
#4568=EDGE_LOOP('',(#22295,#22296,#22297,#22298)) ;
#4569=EDGE_LOOP('',(#22299,#22300,#22301,#22302)) ;
#4570=EDGE_LOOP('',(#22303,#22304,#22305,#22306)) ;
#4571=EDGE_LOOP('',(#22307,#22308,#22309,#22310)) ;
#4572=EDGE_LOOP('',(#22311,#22312,#22313,#22314)) ;
#4573=EDGE_LOOP('',(#22315,#22316,#22317,#22318)) ;
#4574=EDGE_LOOP('',(#22319,#22320,#22321,#22322)) ;
#4575=EDGE_LOOP('',(#22323,#22324,#22325,#22326)) ;
#4576=EDGE_LOOP('',(#22327,#22328,#22329,#22330)) ;
#4577=EDGE_LOOP('',(#22331,#22332,#22333,#22334)) ;
#4578=EDGE_LOOP('',(#22335,#22336,#22337,#22338)) ;
#4579=EDGE_LOOP('',(#22339,#22340,#22341,#22342)) ;
#4580=EDGE_LOOP('',(#22343,#22344,#22345,#22346)) ;
#4581=EDGE_LOOP('',(#22347,#22348,#22349,#22350)) ;
#4582=EDGE_LOOP('',(#22351,#22352,#22353,#22354)) ;
#4583=EDGE_LOOP('',(#22355,#22356,#22357,#22358,#22359,#22360,#22361,#22362)) ;
#4584=EDGE_LOOP('',(#22363,#22364,#22365,#22366)) ;
#4585=EDGE_LOOP('',(#22367,#22368,#22369,#22370)) ;
#4586=EDGE_LOOP('',(#22371,#22372,#22373,#22374)) ;
#4587=EDGE_LOOP('',(#22375,#22376,#22377,#22378)) ;
#4588=EDGE_LOOP('',(#22379,#22380,#22381,#22382)) ;
#4589=EDGE_LOOP('',(#22383,#22384,#22385,#22386,#22387,#22388,#22389,#22390)) ;
#4590=EDGE_LOOP('',(#22391,#22392,#22393,#22394)) ;
#4591=EDGE_LOOP('',(#22395,#22396,#22397,#22398)) ;
#4592=EDGE_LOOP('',(#22399,#22400,#22401,#22402)) ;
#4593=EDGE_LOOP('',(#22403,#22404,#22405,#22406)) ;
#4594=EDGE_LOOP('',(#22407,#22408,#22409,#22410)) ;
#4595=EDGE_LOOP('',(#22411,#22412,#22413,#22414)) ;
#4596=EDGE_LOOP('',(#22415,#22416,#22417,#22418,#22419)) ;
#4597=EDGE_LOOP('',(#22420,#22421,#22422,#22423,#22424)) ;
#4598=EDGE_LOOP('',(#22425,#22426,#22427,#22428,#22429)) ;
#4599=EDGE_LOOP('',(#22430,#22431,#22432,#22433,#22434)) ;
#4600=EDGE_LOOP('',(#22435,#22436,#22437,#22438)) ;
#4601=EDGE_LOOP('',(#22439,#22440,#22441,#22442)) ;
#4602=EDGE_LOOP('',(#22443,#22444,#22445,#22446)) ;
#4603=EDGE_LOOP('',(#22447,#22448,#22449,#22450)) ;
#4604=EDGE_LOOP('',(#22451,#22452,#22453,#22454)) ;
#4605=EDGE_LOOP('',(#22455,#22456,#22457,#22458)) ;
#4606=EDGE_LOOP('',(#22459,#22460,#22461,#22462)) ;
#4607=EDGE_LOOP('',(#22463,#22464,#22465,#22466,#22467,#22468)) ;
#4608=EDGE_LOOP('',(#22469,#22470,#22471,#22472)) ;
#4609=EDGE_LOOP('',(#22473,#22474,#22475,#22476)) ;
#4610=EDGE_LOOP('',(#22477,#22478,#22479,#22480)) ;
#4611=EDGE_LOOP('',(#22481,#22482,#22483,#22484)) ;
#4612=EDGE_LOOP('',(#22485,#22486,#22487,#22488)) ;
#4613=EDGE_LOOP('',(#22489,#22490,#22491,#22492)) ;
#4614=EDGE_LOOP('',(#22493,#22494,#22495,#22496)) ;
#4615=EDGE_LOOP('',(#22497,#22498,#22499,#22500)) ;
#4616=EDGE_LOOP('',(#22501,#22502,#22503,#22504)) ;
#4617=EDGE_LOOP('',(#22505,#22506,#22507,#22508)) ;
#4618=EDGE_LOOP('',(#22509,#22510,#22511,#22512)) ;
#4619=EDGE_LOOP('',(#22513,#22514,#22515,#22516)) ;
#4620=EDGE_LOOP('',(#22517,#22518,#22519,#22520)) ;
#4621=EDGE_LOOP('',(#22521,#22522,#22523,#22524)) ;
#4622=EDGE_LOOP('',(#22525,#22526,#22527,#22528)) ;
#4623=EDGE_LOOP('',(#22529,#22530,#22531,#22532)) ;
#4624=EDGE_LOOP('',(#22533,#22534,#22535,#22536)) ;
#4625=EDGE_LOOP('',(#22537,#22538,#22539,#22540)) ;
#4626=EDGE_LOOP('',(#22541,#22542,#22543,#22544)) ;
#4627=EDGE_LOOP('',(#22545,#22546,#22547,#22548)) ;
#4628=EDGE_LOOP('',(#22549,#22550,#22551,#22552)) ;
#4629=EDGE_LOOP('',(#22553,#22554,#22555,#22556)) ;
#4630=EDGE_LOOP('',(#22557,#22558,#22559,#22560,#22561,#22562,#22563,#22564)) ;
#4631=EDGE_LOOP('',(#22565,#22566,#22567,#22568,#22569,#22570,#22571,#22572)) ;
#4632=EDGE_LOOP('',(#22573,#22574,#22575,#22576)) ;
#4633=EDGE_LOOP('',(#22577,#22578,#22579,#22580)) ;
#4634=EDGE_LOOP('',(#22581,#22582,#22583,#22584,#22585,#22586,#22587,#22588)) ;
#4635=EDGE_LOOP('',(#22589,#22590,#22591,#22592)) ;
#4636=EDGE_LOOP('',(#22593,#22594,#22595,#22596)) ;
#4637=EDGE_LOOP('',(#22597,#22598,#22599,#22600)) ;
#4638=EDGE_LOOP('',(#22601,#22602,#22603,#22604,#22605,#22606)) ;
#4639=EDGE_LOOP('',(#22607,#22608,#22609,#22610,#22611,#22612,#22613,#22614)) ;
#4640=EDGE_LOOP('',(#22615,#22616,#22617,#22618,#22619,#22620,#22621,#22622)) ;
#4641=EDGE_LOOP('',(#22623,#22624,#22625,#22626,#22627,#22628,#22629,#22630)) ;
#4642=EDGE_LOOP('',(#22631,#22632,#22633,#22634,#22635,#22636,#22637,#22638)) ;
#4643=EDGE_LOOP('',(#22639,#22640,#22641,#22642,#22643,#22644,#22645,#22646,
#22647,#22648,#22649,#22650)) ;
#4644=EDGE_LOOP('',(#22651)) ;
#4645=EDGE_LOOP('',(#22652)) ;
#4646=EDGE_LOOP('',(#22653)) ;
#4647=EDGE_LOOP('',(#22654)) ;
#4648=EDGE_LOOP('',(#22655,#22656,#22657,#22658)) ;
#4649=EDGE_LOOP('',(#22659,#22660,#22661,#22662,#22663)) ;
#4650=EDGE_LOOP('',(#22664,#22665,#22666,#22667,#22668)) ;
#4651=EDGE_LOOP('',(#22669,#22670,#22671,#22672,#22673)) ;
#4652=EDGE_LOOP('',(#22674,#22675,#22676,#22677,#22678)) ;
#4653=EDGE_LOOP('',(#22679,#22680,#22681,#22682,#22683)) ;
#4654=EDGE_LOOP('',(#22684,#22685,#22686,#22687,#22688)) ;
#4655=EDGE_LOOP('',(#22689,#22690,#22691,#22692,#22693)) ;
#4656=EDGE_LOOP('',(#22694,#22695,#22696,#22697,#22698)) ;
#4657=EDGE_LOOP('',(#22699,#22700,#22701,#22702)) ;
#4658=EDGE_LOOP('',(#22703,#22704,#22705,#22706,#22707)) ;
#4659=EDGE_LOOP('',(#22708,#22709,#22710,#22711,#22712)) ;
#4660=EDGE_LOOP('',(#22713,#22714,#22715,#22716,#22717,#22718,#22719,#22720)) ;
#4661=EDGE_LOOP('',(#22721,#22722,#22723,#22724,#22725,#22726,#22727,#22728)) ;
#4662=EDGE_LOOP('',(#22729,#22730,#22731,#22732)) ;
#4663=EDGE_LOOP('',(#22733,#22734,#22735,#22736)) ;
#4664=EDGE_LOOP('',(#22737,#22738,#22739,#22740)) ;
#4665=EDGE_LOOP('',(#22741,#22742,#22743,#22744)) ;
#4666=EDGE_LOOP('',(#22745,#22746,#22747,#22748)) ;
#4667=EDGE_LOOP('',(#22749,#22750,#22751,#22752)) ;
#4668=EDGE_LOOP('',(#22753,#22754,#22755,#22756)) ;
#4669=EDGE_LOOP('',(#22757,#22758,#22759,#22760)) ;
#4670=EDGE_LOOP('',(#22761,#22762,#22763,#22764)) ;
#4671=EDGE_LOOP('',(#22765,#22766,#22767,#22768)) ;
#4672=EDGE_LOOP('',(#22769,#22770,#22771,#22772)) ;
#4673=EDGE_LOOP('',(#22773,#22774,#22775,#22776)) ;
#4674=EDGE_LOOP('',(#22777,#22778,#22779,#22780)) ;
#4675=EDGE_LOOP('',(#22781,#22782,#22783,#22784)) ;
#4676=EDGE_LOOP('',(#22785,#22786,#22787,#22788)) ;
#4677=EDGE_LOOP('',(#22789,#22790,#22791,#22792)) ;
#4678=EDGE_LOOP('',(#22793,#22794,#22795,#22796)) ;
#4679=EDGE_LOOP('',(#22797,#22798,#22799,#22800)) ;
#4680=EDGE_LOOP('',(#22801,#22802,#22803,#22804)) ;
#4681=EDGE_LOOP('',(#22805,#22806,#22807,#22808)) ;
#4682=EDGE_LOOP('',(#22809,#22810,#22811,#22812)) ;
#4683=EDGE_LOOP('',(#22813,#22814,#22815,#22816,#22817,#22818,#22819,#22820)) ;
#4684=EDGE_LOOP('',(#22821,#22822,#22823,#22824)) ;
#4685=EDGE_LOOP('',(#22825,#22826,#22827,#22828,#22829,#22830,#22831,#22832)) ;
#4686=EDGE_LOOP('',(#22833,#22834,#22835,#22836,#22837,#22838,#22839,#22840,
#22841,#22842)) ;
#4687=EDGE_LOOP('',(#22843,#22844,#22845,#22846,#22847,#22848)) ;
#4688=EDGE_LOOP('',(#22849,#22850,#22851,#22852,#22853,#22854,#22855,#22856,
#22857,#22858)) ;
#4689=EDGE_LOOP('',(#22859)) ;
#4690=EDGE_LOOP('',(#22860,#22861,#22862,#22863,#22864)) ;
#4691=EDGE_LOOP('',(#22865,#22866,#22867,#22868,#22869)) ;
#4692=EDGE_LOOP('',(#22870,#22871,#22872,#22873,#22874,#22875,#22876,#22877,
#22878,#22879,#22880,#22881)) ;
#4693=EDGE_LOOP('',(#22882,#22883,#22884,#22885,#22886,#22887,#22888,#22889,
#22890,#22891,#22892,#22893,#22894)) ;
#4694=EDGE_LOOP('',(#22895,#22896,#22897,#22898,#22899,#22900,#22901,#22902,
#22903,#22904,#22905,#22906)) ;
#4695=EDGE_LOOP('',(#22907,#22908,#22909,#22910,#22911,#22912,#22913,#22914,
#22915,#22916,#22917,#22918,#22919)) ;
#4696=EDGE_LOOP('',(#22920,#22921,#22922,#22923,#22924,#22925,#22926,#22927,
#22928,#22929,#22930,#22931)) ;
#4697=EDGE_LOOP('',(#22932,#22933,#22934,#22935,#22936,#22937,#22938,#22939,
#22940,#22941,#22942,#22943,#22944,#22945,#22946)) ;
#4698=EDGE_LOOP('',(#22947,#22948,#22949,#22950,#22951,#22952,#22953,#22954,
#22955,#22956,#22957,#22958)) ;
#4699=EDGE_LOOP('',(#22959,#22960,#22961,#22962,#22963,#22964,#22965,#22966,
#22967,#22968,#22969,#22970,#22971)) ;
#4700=EDGE_LOOP('',(#22972,#22973,#22974,#22975)) ;
#4701=EDGE_LOOP('',(#22976,#22977,#22978,#22979)) ;
#4702=EDGE_LOOP('',(#22980,#22981,#22982,#22983)) ;
#4703=EDGE_LOOP('',(#22984,#22985,#22986,#22987)) ;
#4704=EDGE_LOOP('',(#22988,#22989,#22990,#22991)) ;
#4705=EDGE_LOOP('',(#22992,#22993,#22994,#22995)) ;
#4706=EDGE_LOOP('',(#22996,#22997,#22998,#22999)) ;
#4707=EDGE_LOOP('',(#23000,#23001,#23002,#23003)) ;
#4708=EDGE_LOOP('',(#23004,#23005,#23006,#23007)) ;
#4709=EDGE_LOOP('',(#23008,#23009,#23010,#23011)) ;
#4710=EDGE_LOOP('',(#23012,#23013,#23014,#23015)) ;
#4711=EDGE_LOOP('',(#23016,#23017,#23018,#23019)) ;
#4712=EDGE_LOOP('',(#23020,#23021,#23022,#23023)) ;
#4713=EDGE_LOOP('',(#23024,#23025,#23026,#23027)) ;
#4714=EDGE_LOOP('',(#23028,#23029,#23030,#23031)) ;
#4715=EDGE_LOOP('',(#23032,#23033,#23034,#23035)) ;
#4716=EDGE_LOOP('',(#23036,#23037,#23038,#23039)) ;
#4717=EDGE_LOOP('',(#23040,#23041,#23042,#23043,#23044,#23045,#23046)) ;
#4718=EDGE_LOOP('',(#23047,#23048,#23049,#23050)) ;
#4719=EDGE_LOOP('',(#23051,#23052,#23053,#23054,#23055,#23056,#23057)) ;
#4720=EDGE_LOOP('',(#23058,#23059,#23060,#23061,#23062)) ;
#4721=EDGE_LOOP('',(#23063,#23064,#23065,#23066,#23067)) ;
#4722=EDGE_LOOP('',(#23068,#23069,#23070,#23071,#23072)) ;
#4723=EDGE_LOOP('',(#23073,#23074,#23075,#23076,#23077,#23078,#23079,#23080)) ;
#4724=EDGE_LOOP('',(#23081)) ;
#4725=EDGE_LOOP('',(#23082)) ;
#4726=EDGE_LOOP('',(#23083)) ;
#4727=EDGE_LOOP('',(#23084)) ;
#4728=EDGE_LOOP('',(#23085,#23086,#23087,#23088)) ;
#4729=EDGE_LOOP('',(#23089,#23090,#23091,#23092)) ;
#4730=EDGE_LOOP('',(#23093,#23094,#23095,#23096)) ;
#4731=EDGE_LOOP('',(#23097,#23098,#23099,#23100,#23101,#23102)) ;
#4732=EDGE_LOOP('',(#23103)) ;
#4733=EDGE_LOOP('',(#23104,#23105,#23106,#23107,#23108)) ;
#4734=EDGE_LOOP('',(#23109,#23110,#23111,#23112)) ;
#4735=EDGE_LOOP('',(#23113,#23114,#23115,#23116)) ;
#4736=EDGE_LOOP('',(#23117,#23118,#23119,#23120)) ;
#4737=EDGE_LOOP('',(#23121,#23122,#23123,#23124,#23125,#23126,#23127,#23128,
#23129,#23130,#23131,#23132)) ;
#4738=EDGE_LOOP('',(#23133,#23134,#23135,#23136,#23137,#23138,#23139,#23140,
#23141,#23142,#23143,#23144,#23145)) ;
#4739=EDGE_LOOP('',(#23146,#23147,#23148,#23149,#23150,#23151,#23152,#23153,
#23154,#23155,#23156,#23157)) ;
#4740=EDGE_LOOP('',(#23158,#23159,#23160,#23161,#23162,#23163,#23164,#23165,
#23166,#23167,#23168,#23169,#23170,#23171,#23172)) ;
#4741=EDGE_LOOP('',(#23173,#23174,#23175,#23176,#23177,#23178,#23179,#23180,
#23181,#23182,#23183,#23184,#23185,#23186)) ;
#4742=EDGE_LOOP('',(#23187,#23188,#23189,#23190,#23191,#23192,#23193,#23194,
#23195,#23196,#23197,#23198,#23199,#23200)) ;
#4743=EDGE_LOOP('',(#23201,#23202,#23203,#23204,#23205,#23206,#23207,#23208,
#23209,#23210,#23211,#23212,#23213,#23214,#23215,#23216,#23217,#23218,#23219,
#23220,#23221,#23222,#23223,#23224,#23225,#23226,#23227,#23228,#23229,#23230,
#23231,#23232)) ;
#4744=EDGE_LOOP('',(#23233,#23234,#23235,#23236,#23237,#23238)) ;
#4745=EDGE_LOOP('',(#23239,#23240,#23241,#23242,#23243,#23244)) ;
#4746=EDGE_LOOP('',(#23245,#23246,#23247,#23248,#23249,#23250)) ;
#4747=EDGE_LOOP('',(#23251,#23252,#23253,#23254,#23255,#23256)) ;
#4748=EDGE_LOOP('',(#23257,#23258,#23259,#23260,#23261,#23262)) ;
#4749=EDGE_LOOP('',(#23263,#23264,#23265,#23266,#23267)) ;
#4750=EDGE_LOOP('',(#23268,#23269,#23270,#23271,#23272)) ;
#4751=EDGE_LOOP('',(#23273,#23274,#23275,#23276,#23277)) ;
#4752=EDGE_LOOP('',(#23278,#23279,#23280,#23281,#23282)) ;
#4753=EDGE_LOOP('',(#23283,#23284,#23285,#23286,#23287,#23288,#23289,#23290,
#23291,#23292,#23293,#23294)) ;
#4754=EDGE_LOOP('',(#23295,#23296,#23297,#23298,#23299,#23300,#23301,#23302,
#23303,#23304,#23305,#23306,#23307)) ;
#4755=EDGE_LOOP('',(#23308,#23309,#23310,#23311)) ;
#4756=EDGE_LOOP('',(#23312,#23313,#23314,#23315)) ;
#4757=EDGE_LOOP('',(#23316,#23317,#23318,#23319)) ;
#4758=EDGE_LOOP('',(#23320,#23321,#23322,#23323)) ;
#4759=EDGE_LOOP('',(#23324,#23325,#23326,#23327)) ;
#4760=EDGE_LOOP('',(#23328,#23329,#23330,#23331)) ;
#4761=EDGE_LOOP('',(#23332,#23333,#23334,#23335)) ;
#4762=EDGE_LOOP('',(#23336,#23337,#23338,#23339)) ;
#4763=EDGE_LOOP('',(#23340,#23341,#23342,#23343)) ;
#4764=EDGE_LOOP('',(#23344,#23345,#23346,#23347)) ;
#4765=EDGE_LOOP('',(#23348,#23349,#23350,#23351)) ;
#4766=EDGE_LOOP('',(#23352,#23353,#23354,#23355)) ;
#4767=EDGE_LOOP('',(#23356,#23357,#23358,#23359,#23360,#23361,#23362,#23363,
#23364,#23365,#23366,#23367,#23368,#23369,#23370,#23371,#23372,#23373,#23374,
#23375,#23376,#23377,#23378,#23379,#23380,#23381,#23382,#23383,#23384,#23385)) ;
#4768=EDGE_LOOP('',(#23386,#23387,#23388,#23389,#23390,#23391)) ;
#4769=EDGE_LOOP('',(#23392,#23393,#23394,#23395,#23396,#23397)) ;
#4770=EDGE_LOOP('',(#23398,#23399,#23400,#23401,#23402,#23403)) ;
#4771=EDGE_LOOP('',(#23404,#23405,#23406,#23407,#23408,#23409)) ;
#4772=EDGE_LOOP('',(#23410,#23411,#23412,#23413,#23414,#23415)) ;
#4773=EDGE_LOOP('',(#23416,#23417,#23418,#23419,#23420,#23421)) ;
#4774=EDGE_LOOP('',(#23422,#23423,#23424,#23425,#23426,#23427)) ;
#4775=EDGE_LOOP('',(#23428,#23429,#23430,#23431,#23432,#23433)) ;
#4776=EDGE_LOOP('',(#23434,#23435,#23436,#23437,#23438,#23439)) ;
#4777=EDGE_LOOP('',(#23440,#23441,#23442,#23443)) ;
#4778=EDGE_LOOP('',(#23444,#23445,#23446,#23447)) ;
#4779=EDGE_LOOP('',(#23448,#23449,#23450,#23451)) ;
#4780=EDGE_LOOP('',(#23452,#23453,#23454,#23455)) ;
#4781=EDGE_LOOP('',(#23456,#23457,#23458,#23459)) ;
#4782=EDGE_LOOP('',(#23460,#23461,#23462,#23463)) ;
#6505=LINE('',#50228,#8824) ;
#6506=LINE('',#50299,#8825) ;
#6507=LINE('',#50538,#8826) ;
#6508=LINE('',#50751,#8827) ;
#6509=LINE('',#50782,#8828) ;
#6510=LINE('',#51024,#8829) ;
#6511=LINE('',#51289,#8830) ;
#6512=LINE('',#51360,#8831) ;
#6513=LINE('',#51601,#8832) ;
#6514=LINE('',#51825,#8833) ;
#6515=LINE('',#51894,#8834) ;
#6516=LINE('',#52133,#8835) ;
#6517=LINE('',#52348,#8836) ;
#6518=LINE('',#52397,#8837) ;
#6519=LINE('',#52706,#8838) ;
#6520=LINE('',#53062,#8839) ;
#6521=LINE('',#53111,#8840) ;
#6522=LINE('',#53420,#8841) ;
#6523=LINE('',#53776,#8842) ;
#6524=LINE('',#53825,#8843) ;
#6525=LINE('',#54134,#8844) ;
#6526=LINE('',#54490,#8845) ;
#6527=LINE('',#54539,#8846) ;
#6528=LINE('',#54848,#8847) ;
#6529=LINE('',#55204,#8848) ;
#6530=LINE('',#55275,#8849) ;
#6531=LINE('',#55510,#8850) ;
#6532=LINE('',#55723,#8851) ;
#6533=LINE('',#55794,#8852) ;
#6534=LINE('',#56035,#8853) ;
#6535=LINE('',#56259,#8854) ;
#6536=LINE('',#56308,#8855) ;
#6537=LINE('',#56617,#8856) ;
#6538=LINE('',#56973,#8857) ;
#6539=LINE('',#57022,#8858) ;
#6540=LINE('',#57329,#8859) ;
#6541=LINE('',#57685,#8860) ;
#6542=LINE('',#57754,#8861) ;
#6543=LINE('',#57997,#8862) ;
#6544=LINE('',#58214,#8863) ;
#6545=LINE('',#58283,#8864) ;
#6546=LINE('',#58524,#8865) ;
#6547=LINE('',#58737,#8866) ;
#6548=LINE('',#58786,#8867) ;
#6549=LINE('',#59095,#8868) ;
#6550=LINE('',#59451,#8869) ;
#6551=LINE('',#59500,#8870) ;
#6552=LINE('',#59809,#8871) ;
#6553=LINE('',#63661,#8872) ;
#6554=LINE('',#63664,#8873) ;
#6555=LINE('',#63670,#8874) ;
#6556=LINE('',#63673,#8875) ;
#6557=LINE('',#63679,#8876) ;
#6558=LINE('',#63682,#8877) ;
#6559=LINE('',#63688,#8878) ;
#6560=LINE('',#63691,#8879) ;
#6561=LINE('',#63697,#8880) ;
#6562=LINE('',#63700,#8881) ;
#6563=LINE('',#63703,#8882) ;
#6564=LINE('',#63706,#8883) ;
#6565=LINE('',#63708,#8884) ;
#6566=LINE('',#63712,#8885) ;
#6567=LINE('',#63715,#8886) ;
#6568=LINE('',#63716,#8887) ;
#6569=LINE('',#63722,#8888) ;
#6570=LINE('',#63725,#8889) ;
#6571=LINE('',#63731,#8890) ;
#6572=LINE('',#63734,#8891) ;
#6573=LINE('',#63736,#8892) ;
#6574=LINE('',#63738,#8893) ;
#6575=LINE('',#63740,#8894) ;
#6576=LINE('',#63744,#8895) ;
#6577=LINE('',#63746,#8896) ;
#6578=LINE('',#63748,#8897) ;
#6579=LINE('',#63752,#8898) ;
#6580=LINE('',#63754,#8899) ;
#6581=LINE('',#63756,#8900) ;
#6582=LINE('',#63758,#8901) ;
#6583=LINE('',#63759,#8902) ;
#6584=LINE('',#63762,#8903) ;
#6585=LINE('',#63764,#8904) ;
#6586=LINE('',#63766,#8905) ;
#6587=LINE('',#63768,#8906) ;
#6588=LINE('',#63770,#8907) ;
#6589=LINE('',#63772,#8908) ;
#6590=LINE('',#63776,#8909) ;
#6591=LINE('',#63780,#8910) ;
#6592=LINE('',#63782,#8911) ;
#6593=LINE('',#63784,#8912) ;
#6594=LINE('',#63786,#8913) ;
#6595=LINE('',#63787,#8914) ;
#6596=LINE('',#64142,#8915) ;
#6597=LINE('',#64144,#8916) ;
#6598=LINE('',#64146,#8917) ;
#6599=LINE('',#64147,#8918) ;
#6600=LINE('',#64150,#8919) ;
#6601=LINE('',#64152,#8920) ;
#6602=LINE('',#64154,#8921) ;
#6603=LINE('',#64155,#8922) ;
#6604=LINE('',#64158,#8923) ;
#6605=LINE('',#64160,#8924) ;
#6606=LINE('',#64162,#8925) ;
#6607=LINE('',#64163,#8926) ;
#6608=LINE('',#64171,#8927) ;
#6609=LINE('',#64174,#8928) ;
#6610=LINE('',#64176,#8929) ;
#6611=LINE('',#64178,#8930) ;
#6612=LINE('',#64180,#8931) ;
#6613=LINE('',#64181,#8932) ;
#6614=LINE('',#64183,#8933) ;
#6615=LINE('',#64187,#8934) ;
#6616=LINE('',#64189,#8935) ;
#6617=LINE('',#64191,#8936) ;
#6618=LINE('',#64195,#8937) ;
#6619=LINE('',#64197,#8938) ;
#6620=LINE('',#64199,#8939) ;
#6621=LINE('',#64203,#8940) ;
#6622=LINE('',#64205,#8941) ;
#6623=LINE('',#64207,#8942) ;
#6624=LINE('',#64210,#8943) ;
#6625=LINE('',#64215,#8944) ;
#6626=LINE('',#64217,#8945) ;
#6627=LINE('',#64219,#8946) ;
#6628=LINE('',#64220,#8947) ;
#6629=LINE('',#64223,#8948) ;
#6630=LINE('',#64225,#8949) ;
#6631=LINE('',#64227,#8950) ;
#6632=LINE('',#64228,#8951) ;
#6633=LINE('',#64231,#8952) ;
#6634=LINE('',#64233,#8953) ;
#6635=LINE('',#64235,#8954) ;
#6636=LINE('',#64236,#8955) ;
#6637=LINE('',#64239,#8956) ;
#6638=LINE('',#64241,#8957) ;
#6639=LINE('',#64243,#8958) ;
#6640=LINE('',#64244,#8959) ;
#6641=LINE('',#64599,#8960) ;
#6642=LINE('',#64603,#8961) ;
#6643=LINE('',#64607,#8962) ;
#6644=LINE('',#64611,#8963) ;
#6645=LINE('',#64615,#8964) ;
#6646=LINE('',#64617,#8965) ;
#6647=LINE('',#64619,#8966) ;
#6648=LINE('',#64621,#8967) ;
#6649=LINE('',#64623,#8968) ;
#6650=LINE('',#64625,#8969) ;
#6651=LINE('',#64629,#8970) ;
#6652=LINE('',#64632,#8971) ;
#6653=LINE('',#64635,#8972) ;
#6654=LINE('',#64637,#8973) ;
#6655=LINE('',#64639,#8974) ;
#6656=LINE('',#64641,#8975) ;
#6657=LINE('',#64643,#8976) ;
#6658=LINE('',#64647,#8977) ;
#6659=LINE('',#64649,#8978) ;
#6660=LINE('',#64651,#8979) ;
#6661=LINE('',#64655,#8980) ;
#6662=LINE('',#64656,#8981) ;
#6663=LINE('',#64657,#8982) ;
#6664=LINE('',#64662,#8983) ;
#6665=LINE('',#64664,#8984) ;
#6666=LINE('',#64666,#8985) ;
#6667=LINE('',#64667,#8986) ;
#6668=LINE('',#64670,#8987) ;
#6669=LINE('',#64672,#8988) ;
#6670=LINE('',#64674,#8989) ;
#6671=LINE('',#64675,#8990) ;
#6672=LINE('',#64678,#8991) ;
#6673=LINE('',#64680,#8992) ;
#6674=LINE('',#64682,#8993) ;
#6675=LINE('',#64683,#8994) ;
#6676=LINE('',#64688,#8995) ;
#6677=LINE('',#64692,#8996) ;
#6678=LINE('',#64694,#8997) ;
#6679=LINE('',#64695,#8998) ;
#6680=LINE('',#65050,#8999) ;
#6681=LINE('',#65052,#9000) ;
#6682=LINE('',#65056,#9001) ;
#6683=LINE('',#65058,#9002) ;
#6684=LINE('',#65060,#9003) ;
#6685=LINE('',#65064,#9004) ;
#6686=LINE('',#65066,#9005) ;
#6687=LINE('',#65068,#9006) ;
#6688=LINE('',#65072,#9007) ;
#6689=LINE('',#65074,#9008) ;
#6690=LINE('',#65076,#9009) ;
#6691=LINE('',#65080,#9010) ;
#6692=LINE('',#65082,#9011) ;
#6693=LINE('',#65084,#9012) ;
#6694=LINE('',#65086,#9013) ;
#6695=LINE('',#65087,#9014) ;
#6696=LINE('',#65088,#9015) ;
#6697=LINE('',#65093,#9016) ;
#6698=LINE('',#65097,#9017) ;
#6699=LINE('',#65101,#9018) ;
#6700=LINE('',#65104,#9019) ;
#6701=LINE('',#65459,#9020) ;
#6702=LINE('',#65463,#9021) ;
#6703=LINE('',#65465,#9022) ;
#6704=LINE('',#65466,#9023) ;
#6705=LINE('',#65469,#9024) ;
#6706=LINE('',#65471,#9025) ;
#6707=LINE('',#65473,#9026) ;
#6708=LINE('',#65474,#9027) ;
#6709=LINE('',#65477,#9028) ;
#6710=LINE('',#65479,#9029) ;
#6711=LINE('',#65481,#9030) ;
#6712=LINE('',#65482,#9031) ;
#6713=LINE('',#65485,#9032) ;
#6714=LINE('',#65487,#9033) ;
#6715=LINE('',#65489,#9034) ;
#6716=LINE('',#65490,#9035) ;
#6717=LINE('',#65493,#9036) ;
#6718=LINE('',#65495,#9037) ;
#6719=LINE('',#65497,#9038) ;
#6720=LINE('',#65498,#9039) ;
#6721=LINE('',#65507,#9040) ;
#6722=LINE('',#65508,#9041) ;
#6723=LINE('',#65509,#9042) ;
#6724=LINE('',#65510,#9043) ;
#6725=LINE('',#65513,#9044) ;
#6726=LINE('',#65515,#9045) ;
#6727=LINE('',#65517,#9046) ;
#6728=LINE('',#65530,#9047) ;
#6729=LINE('',#65532,#9048) ;
#6730=LINE('',#65533,#9049) ;
#6731=LINE('',#65537,#9050) ;
#6732=LINE('',#65540,#9051) ;
#6733=LINE('',#65545,#9052) ;
#6734=LINE('',#65550,#9053) ;
#6735=LINE('',#65553,#9054) ;
#6736=LINE('',#65556,#9055) ;
#6737=LINE('',#65558,#9056) ;
#6738=LINE('',#65559,#9057) ;
#6739=LINE('',#65562,#9058) ;
#6740=LINE('',#65563,#9059) ;
#6741=LINE('',#65609,#9060) ;
#6742=LINE('',#65622,#9061) ;
#6743=LINE('',#65623,#9062) ;
#6744=LINE('',#65626,#9063) ;
#6745=LINE('',#65627,#9064) ;
#6746=LINE('',#65628,#9065) ;
#6747=LINE('',#65630,#9066) ;
#6748=LINE('',#65632,#9067) ;
#6749=LINE('',#65634,#9068) ;
#6750=LINE('',#65637,#9069) ;
#6751=LINE('',#65639,#9070) ;
#6752=LINE('',#65641,#9071) ;
#6753=LINE('',#65642,#9072) ;
#6754=LINE('',#65644,#9073) ;
#6755=LINE('',#65649,#9074) ;
#6756=LINE('',#65653,#9075) ;
#6757=LINE('',#65655,#9076) ;
#6758=LINE('',#65656,#9077) ;
#6759=LINE('',#65662,#9078) ;
#6760=LINE('',#65670,#9079) ;
#6761=LINE('',#65678,#9080) ;
#6762=LINE('',#65681,#9081) ;
#6763=LINE('',#65683,#9082) ;
#6764=LINE('',#65684,#9083) ;
#6765=LINE('',#65687,#9084) ;
#6766=LINE('',#65691,#9085) ;
#6767=LINE('',#65692,#9086) ;
#6768=LINE('',#65695,#9087) ;
#6769=LINE('',#65699,#9088) ;
#6770=LINE('',#65700,#9089) ;
#6771=LINE('',#65706,#9090) ;
#6772=LINE('',#65714,#9091) ;
#6773=LINE('',#65722,#9092) ;
#6774=LINE('',#65725,#9093) ;
#6775=LINE('',#65727,#9094) ;
#6776=LINE('',#65728,#9095) ;
#6777=LINE('',#65731,#9096) ;
#6778=LINE('',#65735,#9097) ;
#6779=LINE('',#65736,#9098) ;
#6780=LINE('',#65739,#9099) ;
#6781=LINE('',#65743,#9100) ;
#6782=LINE('',#65744,#9101) ;
#6783=LINE('',#65748,#9102) ;
#6784=LINE('',#65750,#9103) ;
#6785=LINE('',#65752,#9104) ;
#6786=LINE('',#65753,#9105) ;
#6787=LINE('',#65756,#9106) ;
#6788=LINE('',#65758,#9107) ;
#6789=LINE('',#65759,#9108) ;
#6790=LINE('',#65762,#9109) ;
#6791=LINE('',#65764,#9110) ;
#6792=LINE('',#65765,#9111) ;
#6793=LINE('',#65768,#9112) ;
#6794=LINE('',#65770,#9113) ;
#6795=LINE('',#65771,#9114) ;
#6796=LINE('',#65774,#9115) ;
#6797=LINE('',#65776,#9116) ;
#6798=LINE('',#65777,#9117) ;
#6799=LINE('',#65779,#9118) ;
#6800=LINE('',#65780,#9119) ;
#6801=LINE('',#65784,#9120) ;
#6802=LINE('',#65786,#9121) ;
#6803=LINE('',#65788,#9122) ;
#6804=LINE('',#65789,#9123) ;
#6805=LINE('',#65792,#9124) ;
#6806=LINE('',#65794,#9125) ;
#6807=LINE('',#65795,#9126) ;
#6808=LINE('',#65798,#9127) ;
#6809=LINE('',#65800,#9128) ;
#6810=LINE('',#65801,#9129) ;
#6811=LINE('',#65804,#9130) ;
#6812=LINE('',#65806,#9131) ;
#6813=LINE('',#65807,#9132) ;
#6814=LINE('',#65810,#9133) ;
#6815=LINE('',#65812,#9134) ;
#6816=LINE('',#65813,#9135) ;
#6817=LINE('',#65815,#9136) ;
#6818=LINE('',#65816,#9137) ;
#6819=LINE('',#65824,#9138) ;
#6820=LINE('',#65830,#9139) ;
#6821=LINE('',#65833,#9140) ;
#6822=LINE('',#65840,#9141) ;
#6823=LINE('',#65845,#9142) ;
#6824=LINE('',#65849,#9143) ;
#6825=LINE('',#65851,#9144) ;
#6826=LINE('',#65852,#9145) ;
#6827=LINE('',#65853,#9146) ;
#6828=LINE('',#65857,#9147) ;
#6829=LINE('',#65859,#9148) ;
#6830=LINE('',#65863,#9149) ;
#6831=LINE('',#65865,#9150) ;
#6832=LINE('',#65869,#9151) ;
#6833=LINE('',#65871,#9152) ;
#6834=LINE('',#65874,#9153) ;
#6835=LINE('',#65878,#9154) ;
#6836=LINE('',#65884,#9155) ;
#6837=LINE('',#65890,#9156) ;
#6838=LINE('',#65897,#9157) ;
#6839=LINE('',#65900,#9158) ;
#6840=LINE('',#65906,#9159) ;
#6841=LINE('',#65909,#9160) ;
#6842=LINE('',#65915,#9161) ;
#6843=LINE('',#65918,#9162) ;
#6844=LINE('',#65924,#9163) ;
#6845=LINE('',#65927,#9164) ;
#6846=LINE('',#65933,#9165) ;
#6847=LINE('',#65939,#9166) ;
#6848=LINE('',#65942,#9167) ;
#6849=LINE('',#65951,#9168) ;
#6850=LINE('',#65953,#9169) ;
#6851=LINE('',#65954,#9170) ;
#6852=LINE('',#65956,#9171) ;
#6853=LINE('',#65957,#9172) ;
#6854=LINE('',#65959,#9173) ;
#6855=LINE('',#65960,#9174) ;
#6856=LINE('',#65963,#9175) ;
#6857=LINE('',#65965,#9176) ;
#6858=LINE('',#65966,#9177) ;
#6859=LINE('',#65968,#9178) ;
#6860=LINE('',#65970,#9179) ;
#6861=LINE('',#65973,#9180) ;
#6862=LINE('',#65974,#9181) ;
#6863=LINE('',#65976,#9182) ;
#6864=LINE('',#65978,#9183) ;
#6865=LINE('',#65981,#9184) ;
#6866=LINE('',#65982,#9185) ;
#6867=LINE('',#65984,#9186) ;
#6868=LINE('',#65986,#9187) ;
#6869=LINE('',#65991,#9188) ;
#6870=LINE('',#65992,#9189) ;
#6871=LINE('',#65994,#9190) ;
#6872=LINE('',#65996,#9191) ;
#6873=LINE('',#65999,#9192) ;
#6874=LINE('',#66001,#9193) ;
#6875=LINE('',#66004,#9194) ;
#6876=LINE('',#66006,#9195) ;
#6877=LINE('',#66011,#9196) ;
#6878=LINE('',#66014,#9197) ;
#6879=LINE('',#66017,#9198) ;
#6880=LINE('',#66019,#9199) ;
#6881=LINE('',#66023,#9200) ;
#6882=LINE('',#66028,#9201) ;
#6883=LINE('',#66034,#9202) ;
#6884=LINE('',#66036,#9203) ;
#6885=LINE('',#66037,#9204) ;
#6886=LINE('',#66039,#9205) ;
#6887=LINE('',#66040,#9206) ;
#6888=LINE('',#66042,#9207) ;
#6889=LINE('',#66043,#9208) ;
#6890=LINE('',#66045,#9209) ;
#6891=LINE('',#66046,#9210) ;
#6892=LINE('',#66050,#9211) ;
#6893=LINE('',#66051,#9212) ;
#6894=LINE('',#66053,#9213) ;
#6895=LINE('',#66055,#9214) ;
#6896=LINE('',#66056,#9215) ;
#6897=LINE('',#66058,#9216) ;
#6898=LINE('',#66060,#9217) ;
#6899=LINE('',#66064,#9218) ;
#6900=LINE('',#66068,#9219) ;
#6901=LINE('',#66069,#9220) ;
#6902=LINE('',#66082,#9221) ;
#6903=LINE('',#66088,#9222) ;
#6904=LINE('',#66093,#9223) ;
#6905=LINE('',#66098,#9224) ;
#6906=LINE('',#66103,#9225) ;
#6907=LINE('',#66108,#9226) ;
#6908=LINE('',#66113,#9227) ;
#6909=LINE('',#66118,#9228) ;
#6910=LINE('',#66123,#9229) ;
#6911=LINE('',#66127,#9230) ;
#6912=LINE('',#66128,#9231) ;
#6913=LINE('',#66129,#9232) ;
#6914=LINE('',#66135,#9233) ;
#6915=LINE('',#66138,#9234) ;
#6916=LINE('',#66139,#9235) ;
#6917=LINE('',#66141,#9236) ;
#6918=LINE('',#66142,#9237) ;
#6919=LINE('',#66143,#9238) ;
#6920=LINE('',#66145,#9239) ;
#6921=LINE('',#66146,#9240) ;
#6922=LINE('',#66148,#9241) ;
#6923=LINE('',#66150,#9242) ;
#6924=LINE('',#66154,#9243) ;
#6925=LINE('',#66156,#9244) ;
#6926=LINE('',#66157,#9245) ;
#6927=LINE('',#66159,#9246) ;
#6928=LINE('',#66160,#9247) ;
#6929=LINE('',#66167,#9248) ;
#6930=LINE('',#66168,#9249) ;
#6931=LINE('',#66170,#9250) ;
#6932=LINE('',#66172,#9251) ;
#6933=LINE('',#66175,#9252) ;
#6934=LINE('',#66176,#9253) ;
#6935=LINE('',#66178,#9254) ;
#6936=LINE('',#66180,#9255) ;
#6937=LINE('',#66191,#9256) ;
#6938=LINE('',#66194,#9257) ;
#6939=LINE('',#66195,#9258) ;
#6940=LINE('',#66199,#9259) ;
#6941=LINE('',#66201,#9260) ;
#6942=LINE('',#66202,#9261) ;
#6943=LINE('',#66210,#9262) ;
#6944=LINE('',#66211,#9263) ;
#6945=LINE('',#66212,#9264) ;
#6946=LINE('',#66217,#9265) ;
#6947=LINE('',#66220,#9266) ;
#6948=LINE('',#66959,#9267) ;
#6949=LINE('',#66961,#9268) ;
#6950=LINE('',#66962,#9269) ;
#6951=LINE('',#66965,#9270) ;
#6952=LINE('',#66967,#9271) ;
#6953=LINE('',#66968,#9272) ;
#6954=LINE('',#66971,#9273) ;
#6955=LINE('',#66973,#9274) ;
#6956=LINE('',#66974,#9275) ;
#6957=LINE('',#66977,#9276) ;
#6958=LINE('',#66979,#9277) ;
#6959=LINE('',#66980,#9278) ;
#6960=LINE('',#67009,#9279) ;
#6961=LINE('',#67016,#9280) ;
#6962=LINE('',#67020,#9281) ;
#6963=LINE('',#67024,#9282) ;
#6964=LINE('',#67028,#9283) ;
#6965=LINE('',#67033,#9284) ;
#6966=LINE('',#67060,#9285) ;
#6967=LINE('',#67063,#9286) ;
#6968=LINE('',#68692,#9287) ;
#6969=LINE('',#68694,#9288) ;
#6970=LINE('',#68696,#9289) ;
#6971=LINE('',#68698,#9290) ;
#6972=LINE('',#68700,#9291) ;
#6973=LINE('',#68701,#9292) ;
#6974=LINE('',#68704,#9293) ;
#6975=LINE('',#68706,#9294) ;
#6976=LINE('',#68708,#9295) ;
#6977=LINE('',#68710,#9296) ;
#6978=LINE('',#68712,#9297) ;
#6979=LINE('',#68713,#9298) ;
#6980=LINE('',#68716,#9299) ;
#6981=LINE('',#68718,#9300) ;
#6982=LINE('',#68720,#9301) ;
#6983=LINE('',#68722,#9302) ;
#6984=LINE('',#68724,#9303) ;
#6985=LINE('',#68725,#9304) ;
#6986=LINE('',#69263,#9305) ;
#6987=LINE('',#69264,#9306) ;
#6988=LINE('',#69265,#9307) ;
#6989=LINE('',#69268,#9308) ;
#6990=LINE('',#69269,#9309) ;
#6991=LINE('',#69272,#9310) ;
#6992=LINE('',#69273,#9311) ;
#6993=LINE('',#69276,#9312) ;
#6994=LINE('',#69277,#9313) ;
#6995=LINE('',#69280,#9314) ;
#6996=LINE('',#69281,#9315) ;
#6997=LINE('',#69283,#9316) ;
#6998=LINE('',#69287,#9317) ;
#6999=LINE('',#69288,#9318) ;
#7000=LINE('',#69289,#9319) ;
#7001=LINE('',#69292,#9320) ;
#7002=LINE('',#69293,#9321) ;
#7003=LINE('',#69296,#9322) ;
#7004=LINE('',#69297,#9323) ;
#7005=LINE('',#69300,#9324) ;
#7006=LINE('',#69301,#9325) ;
#7007=LINE('',#69304,#9326) ;
#7008=LINE('',#69305,#9327) ;
#7009=LINE('',#69307,#9328) ;
#7010=LINE('',#69311,#9329) ;
#7011=LINE('',#69313,#9330) ;
#7012=LINE('',#69315,#9331) ;
#7013=LINE('',#69317,#9332) ;
#7014=LINE('',#69319,#9333) ;
#7015=LINE('',#69320,#9334) ;
#7016=LINE('',#69322,#9335) ;
#7017=LINE('',#69323,#9336) ;
#7018=LINE('',#69325,#9337) ;
#7019=LINE('',#69327,#9338) ;
#7020=LINE('',#69329,#9339) ;
#7021=LINE('',#69331,#9340) ;
#8824=VECTOR('',#37655,2.05475) ;
#8825=VECTOR('',#37660,2.05475) ;
#8826=VECTOR('',#37663,2.05475) ;
#8827=VECTOR('',#37668,2.05475000000001) ;
#8828=VECTOR('',#37673,2.05475000000001) ;
#8829=VECTOR('',#37676,2.05475000000001) ;
#8830=VECTOR('',#37681,2.05475000000001) ;
#8831=VECTOR('',#37686,2.05475000000001) ;
#8832=VECTOR('',#37689,2.05475000000001) ;
#8833=VECTOR('',#37694,2.05474999999993) ;
#8834=VECTOR('',#37699,2.05474999999993) ;
#8835=VECTOR('',#37702,2.05474999999993) ;
#8836=VECTOR('',#37707,1.66599999999999) ;
#8837=VECTOR('',#37712,1.66599999999999) ;
#8838=VECTOR('',#37717,1.66599999999999) ;
#8839=VECTOR('',#37722,1.66599999999999) ;
#8840=VECTOR('',#37727,1.66599999999999) ;
#8841=VECTOR('',#37732,1.66599999999999) ;
#8842=VECTOR('',#37737,1.66599999999999) ;
#8843=VECTOR('',#37742,1.66599999999999) ;
#8844=VECTOR('',#37747,1.66599999999999) ;
#8845=VECTOR('',#37752,1.66599999999998) ;
#8846=VECTOR('',#37757,1.66599999999998) ;
#8847=VECTOR('',#37762,1.66599999999998) ;
#8848=VECTOR('',#37767,2.05475) ;
#8849=VECTOR('',#37772,2.05475) ;
#8850=VECTOR('',#37775,2.05475) ;
#8851=VECTOR('',#37780,2.05475) ;
#8852=VECTOR('',#37785,2.05475) ;
#8853=VECTOR('',#37788,2.05475) ;
#8854=VECTOR('',#37793,1.666) ;
#8855=VECTOR('',#37798,1.666) ;
#8856=VECTOR('',#37803,1.666) ;
#8857=VECTOR('',#37808,1.666) ;
#8858=VECTOR('',#37813,1.666) ;
#8859=VECTOR('',#37818,1.666) ;
#8860=VECTOR('',#37823,2.05475) ;
#8861=VECTOR('',#37828,2.05475) ;
#8862=VECTOR('',#37831,2.05475) ;
#8863=VECTOR('',#37836,2.05475) ;
#8864=VECTOR('',#37841,2.05475) ;
#8865=VECTOR('',#37844,2.05475) ;
#8866=VECTOR('',#37849,1.66600000000001) ;
#8867=VECTOR('',#37854,1.66600000000001) ;
#8868=VECTOR('',#37859,1.66600000000001) ;
#8869=VECTOR('',#37864,1.66600000000001) ;
#8870=VECTOR('',#37869,1.66600000000001) ;
#8871=VECTOR('',#37874,1.66600000000001) ;
#8872=VECTOR('',#37913,10.) ;
#8873=VECTOR('',#37916,10.) ;
#8874=VECTOR('',#37921,2.5) ;
#8875=VECTOR('',#37924,10.) ;
#8876=VECTOR('',#37929,2.5) ;
#8877=VECTOR('',#37932,2.5) ;
#8878=VECTOR('',#37937,2.5) ;
#8879=VECTOR('',#37940,2.5) ;
#8880=VECTOR('',#37945,10.) ;
#8881=VECTOR('',#37948,2.5) ;
#8882=VECTOR('',#37951,10.) ;
#8883=VECTOR('',#37954,10.) ;
#8884=VECTOR('',#37955,10.) ;
#8885=VECTOR('',#37958,10.) ;
#8886=VECTOR('',#37961,10.) ;
#8887=VECTOR('',#37962,10.) ;
#8888=VECTOR('',#37967,115.) ;
#8889=VECTOR('',#37970,111.) ;
#8890=VECTOR('',#37975,10.) ;
#8891=VECTOR('',#37978,10.) ;
#8892=VECTOR('',#37981,10.) ;
#8893=VECTOR('',#37982,10.) ;
#8894=VECTOR('',#37983,10.) ;
#8895=VECTOR('',#37986,10.) ;
#8896=VECTOR('',#37987,10.) ;
#8897=VECTOR('',#37988,10.) ;
#8898=VECTOR('',#37991,10.) ;
#8899=VECTOR('',#37992,10.) ;
#8900=VECTOR('',#37993,10.) ;
#8901=VECTOR('',#37994,10.) ;
#8902=VECTOR('',#37995,10.) ;
#8903=VECTOR('',#37996,10.) ;
#8904=VECTOR('',#37997,1.65) ;
#8905=VECTOR('',#37998,83.9) ;
#8906=VECTOR('',#37999,1.65) ;
#8907=VECTOR('',#38000,10.) ;
#8908=VECTOR('',#38001,10.) ;
#8909=VECTOR('',#38004,10.) ;
#8910=VECTOR('',#38007,10.) ;
#8911=VECTOR('',#38008,10.) ;
#8912=VECTOR('',#38009,10.) ;
#8913=VECTOR('',#38010,10.) ;
#8914=VECTOR('',#38011,10.) ;
#8915=VECTOR('',#38014,10.) ;
#8916=VECTOR('',#38015,10.) ;
#8917=VECTOR('',#38016,10.) ;
#8918=VECTOR('',#38017,10.) ;
#8919=VECTOR('',#38018,10.) ;
#8920=VECTOR('',#38019,10.) ;
#8921=VECTOR('',#38020,10.) ;
#8922=VECTOR('',#38021,10.) ;
#8923=VECTOR('',#38022,10.) ;
#8924=VECTOR('',#38023,10.) ;
#8925=VECTOR('',#38024,10.) ;
#8926=VECTOR('',#38025,10.) ;
#8927=VECTOR('',#38032,10.) ;
#8928=VECTOR('',#38035,10.) ;
#8929=VECTOR('',#38038,10.) ;
#8930=VECTOR('',#38039,10.) ;
#8931=VECTOR('',#38040,10.) ;
#8932=VECTOR('',#38041,10.) ;
#8933=VECTOR('',#38042,10.) ;
#8934=VECTOR('',#38045,10.) ;
#8935=VECTOR('',#38046,10.) ;
#8936=VECTOR('',#38047,10.) ;
#8937=VECTOR('',#38050,10.) ;
#8938=VECTOR('',#38051,10.) ;
#8939=VECTOR('',#38052,10.) ;
#8940=VECTOR('',#38055,10.) ;
#8941=VECTOR('',#38056,10.) ;
#8942=VECTOR('',#38057,10.) ;
#8943=VECTOR('',#38060,10.) ;
#8944=VECTOR('',#38063,10.) ;
#8945=VECTOR('',#38064,10.) ;
#8946=VECTOR('',#38065,10.) ;
#8947=VECTOR('',#38066,10.) ;
#8948=VECTOR('',#38067,10.) ;
#8949=VECTOR('',#38068,10.) ;
#8950=VECTOR('',#38069,10.) ;
#8951=VECTOR('',#38070,10.) ;
#8952=VECTOR('',#38071,10.) ;
#8953=VECTOR('',#38072,10.) ;
#8954=VECTOR('',#38073,10.) ;
#8955=VECTOR('',#38074,10.) ;
#8956=VECTOR('',#38075,10.) ;
#8957=VECTOR('',#38076,10.) ;
#8958=VECTOR('',#38077,10.) ;
#8959=VECTOR('',#38078,10.) ;
#8960=VECTOR('',#38081,10.) ;
#8961=VECTOR('',#38084,10.) ;
#8962=VECTOR('',#38087,10.) ;
#8963=VECTOR('',#38090,10.) ;
#8964=VECTOR('',#38093,10.) ;
#8965=VECTOR('',#38094,10.) ;
#8966=VECTOR('',#38095,27.5) ;
#8967=VECTOR('',#38096,10.) ;
#8968=VECTOR('',#38097,10.) ;
#8969=VECTOR('',#38098,10.) ;
#8970=VECTOR('',#38101,10.) ;
#8971=VECTOR('',#38104,10.) ;
#8972=VECTOR('',#38107,10.) ;
#8973=VECTOR('',#38108,10.) ;
#8974=VECTOR('',#38109,10.) ;
#8975=VECTOR('',#38110,196.3) ;
#8976=VECTOR('',#38111,19.) ;
#8977=VECTOR('',#38114,19.) ;
#8978=VECTOR('',#38115,3.98) ;
#8979=VECTOR('',#38116,19.) ;
#8980=VECTOR('',#38119,19.) ;
#8981=VECTOR('',#38120,196.3) ;
#8982=VECTOR('',#38121,10.) ;
#8983=VECTOR('',#38124,2.) ;
#8984=VECTOR('',#38125,7.) ;
#8985=VECTOR('',#38126,2.) ;
#8986=VECTOR('',#38127,7.) ;
#8987=VECTOR('',#38128,2.) ;
#8988=VECTOR('',#38129,7.) ;
#8989=VECTOR('',#38130,2.) ;
#8990=VECTOR('',#38131,7.) ;
#8991=VECTOR('',#38132,2.) ;
#8992=VECTOR('',#38133,7.) ;
#8993=VECTOR('',#38134,2.) ;
#8994=VECTOR('',#38135,7.) ;
#8995=VECTOR('',#38138,79.4000000028) ;
#8996=VECTOR('',#38141,14.0000000028) ;
#8997=VECTOR('',#38142,89.9) ;
#8998=VECTOR('',#38143,14.) ;
#8999=VECTOR('',#38148,143.) ;
#9000=VECTOR('',#38149,19.) ;
#9001=VECTOR('',#38152,19.) ;
#9002=VECTOR('',#38153,3.98) ;
#9003=VECTOR('',#38154,19.) ;
#9004=VECTOR('',#38157,19.) ;
#9005=VECTOR('',#38158,41.3) ;
#9006=VECTOR('',#38159,19.) ;
#9007=VECTOR('',#38162,19.) ;
#9008=VECTOR('',#38163,4.) ;
#9009=VECTOR('',#38164,19.) ;
#9010=VECTOR('',#38167,19.) ;
#9011=VECTOR('',#38168,143.) ;
#9012=VECTOR('',#38169,10.) ;
#9013=VECTOR('',#38170,10.) ;
#9014=VECTOR('',#38171,10.) ;
#9015=VECTOR('',#38172,10.) ;
#9016=VECTOR('',#38175,10.) ;
#9017=VECTOR('',#38178,10.) ;
#9018=VECTOR('',#38181,10.) ;
#9019=VECTOR('',#38184,10.) ;
#9020=VECTOR('',#38187,23.0000000028) ;
#9021=VECTOR('',#38190,14.0000000028) ;
#9022=VECTOR('',#38191,33.5) ;
#9023=VECTOR('',#38192,14.) ;
#9024=VECTOR('',#38193,2.) ;
#9025=VECTOR('',#38194,7.) ;
#9026=VECTOR('',#38195,2.) ;
#9027=VECTOR('',#38196,7.) ;
#9028=VECTOR('',#38197,2.) ;
#9029=VECTOR('',#38198,7.) ;
#9030=VECTOR('',#38199,2.) ;
#9031=VECTOR('',#38200,7.) ;
#9032=VECTOR('',#38201,2.) ;
#9033=VECTOR('',#38202,7.) ;
#9034=VECTOR('',#38203,2.) ;
#9035=VECTOR('',#38204,7.) ;
#9036=VECTOR('',#38205,2.) ;
#9037=VECTOR('',#38206,7.) ;
#9038=VECTOR('',#38207,2.) ;
#9039=VECTOR('',#38208,7.) ;
#9040=VECTOR('',#38217,10.) ;
#9041=VECTOR('',#38218,10.) ;
#9042=VECTOR('',#38219,10.) ;
#9043=VECTOR('',#38220,10.) ;
#9044=VECTOR('',#38223,10.) ;
#9045=VECTOR('',#38224,10.) ;
#9046=VECTOR('',#38225,10.) ;
#9047=VECTOR('',#38226,10.) ;
#9048=VECTOR('',#38227,10.) ;
#9049=VECTOR('',#38228,10.) ;
#9050=VECTOR('',#38233,141.) ;
#9051=VECTOR('',#38236,141.) ;
#9052=VECTOR('',#38243,194.3) ;
#9053=VECTOR('',#38248,0.5) ;
#9054=VECTOR('',#38253,10.) ;
#9055=VECTOR('',#38256,10.) ;
#9056=VECTOR('',#38257,10.) ;
#9057=VECTOR('',#38258,10.) ;
#9058=VECTOR('',#38261,10.) ;
#9059=VECTOR('',#38262,10.) ;
#9060=VECTOR('',#38263,10.) ;
#9061=VECTOR('',#38266,10.) ;
#9062=VECTOR('',#38267,10.) ;
#9063=VECTOR('',#38270,10.) ;
#9064=VECTOR('',#38271,10.) ;
#9065=VECTOR('',#38272,10.) ;
#9066=VECTOR('',#38275,10.) ;
#9067=VECTOR('',#38276,10.) ;
#9068=VECTOR('',#38279,10.) ;
#9069=VECTOR('',#38284,10.) ;
#9070=VECTOR('',#38287,10.) ;
#9071=VECTOR('',#38288,10.) ;
#9072=VECTOR('',#38289,10.) ;
#9073=VECTOR('',#38292,10.) ;
#9074=VECTOR('',#38297,10.) ;
#9075=VECTOR('',#38302,1.25) ;
#9076=VECTOR('',#38303,10.) ;
#9077=VECTOR('',#38304,0.75) ;
#9078=VECTOR('',#38311,10.) ;
#9079=VECTOR('',#38322,10.) ;
#9080=VECTOR('',#38333,10.) ;
#9081=VECTOR('',#38336,1.25) ;
#9082=VECTOR('',#38337,10.) ;
#9083=VECTOR('',#38338,1.25) ;
#9084=VECTOR('',#38341,0.5) ;
#9085=VECTOR('',#38346,10.) ;
#9086=VECTOR('',#38347,10.) ;
#9087=VECTOR('',#38350,1.25) ;
#9088=VECTOR('',#38355,0.75) ;
#9089=VECTOR('',#38356,10.) ;
#9090=VECTOR('',#38363,10.) ;
#9091=VECTOR('',#38374,10.) ;
#9092=VECTOR('',#38385,10.) ;
#9093=VECTOR('',#38388,1.25) ;
#9094=VECTOR('',#38389,10.) ;
#9095=VECTOR('',#38390,10.) ;
#9096=VECTOR('',#38393,0.5) ;
#9097=VECTOR('',#38398,10.) ;
#9098=VECTOR('',#38399,10.) ;
#9099=VECTOR('',#38402,1.25) ;
#9100=VECTOR('',#38407,10.) ;
#9101=VECTOR('',#38408,10.) ;
#9102=VECTOR('',#38411,9.99999999999998) ;
#9103=VECTOR('',#38412,1000.) ;
#9104=VECTOR('',#38413,9.99999999999998) ;
#9105=VECTOR('',#38414,1000.) ;
#9106=VECTOR('',#38417,9.99999999999998) ;
#9107=VECTOR('',#38418,9.99999999999998) ;
#9108=VECTOR('',#38419,1000.) ;
#9109=VECTOR('',#38422,10.) ;
#9110=VECTOR('',#38423,10.) ;
#9111=VECTOR('',#38424,1000.) ;
#9112=VECTOR('',#38427,10.) ;
#9113=VECTOR('',#38428,10.) ;
#9114=VECTOR('',#38429,1000.) ;
#9115=VECTOR('',#38432,10.) ;
#9116=VECTOR('',#38433,1000.) ;
#9117=VECTOR('',#38434,10.) ;
#9118=VECTOR('',#38437,10.) ;
#9119=VECTOR('',#38438,10.) ;
#9120=VECTOR('',#38441,9.99999999999998) ;
#9121=VECTOR('',#38442,1000.) ;
#9122=VECTOR('',#38443,9.99999999999998) ;
#9123=VECTOR('',#38444,1000.) ;
#9124=VECTOR('',#38447,9.99999999999998) ;
#9125=VECTOR('',#38448,9.99999999999998) ;
#9126=VECTOR('',#38449,1000.) ;
#9127=VECTOR('',#38452,10.) ;
#9128=VECTOR('',#38453,10.) ;
#9129=VECTOR('',#38454,1000.) ;
#9130=VECTOR('',#38457,10.) ;
#9131=VECTOR('',#38458,10.) ;
#9132=VECTOR('',#38459,1000.) ;
#9133=VECTOR('',#38462,10.) ;
#9134=VECTOR('',#38463,1000.) ;
#9135=VECTOR('',#38464,10.) ;
#9136=VECTOR('',#38467,10.) ;
#9137=VECTOR('',#38468,10.) ;
#9138=VECTOR('',#38479,10.) ;
#9139=VECTOR('',#38486,10.) ;
#9140=VECTOR('',#38489,10.) ;
#9141=VECTOR('',#38498,10.) ;
#9142=VECTOR('',#38503,10.) ;
#9143=VECTOR('',#38508,2.5) ;
#9144=VECTOR('',#38509,2.) ;
#9145=VECTOR('',#38510,4.) ;
#9146=VECTOR('',#38511,2.5) ;
#9147=VECTOR('',#38516,2.20000000000002) ;
#9148=VECTOR('',#38519,1.65) ;
#9149=VECTOR('',#38524,2.2) ;
#9150=VECTOR('',#38527,1.65) ;
#9151=VECTOR('',#38532,2.2) ;
#9152=VECTOR('',#38535,1.65) ;
#9153=VECTOR('',#38538,10.) ;
#9154=VECTOR('',#38543,10.) ;
#9155=VECTOR('',#38550,1.75) ;
#9156=VECTOR('',#38557,2.25) ;
#9157=VECTOR('',#38564,2.) ;
#9158=VECTOR('',#38567,2.) ;
#9159=VECTOR('',#38572,2.) ;
#9160=VECTOR('',#38575,2.) ;
#9161=VECTOR('',#38580,2.) ;
#9162=VECTOR('',#38583,2.) ;
#9163=VECTOR('',#38588,2.) ;
#9164=VECTOR('',#38591,2.) ;
#9165=VECTOR('',#38598,2.) ;
#9166=VECTOR('',#38603,2.) ;
#9167=VECTOR('',#38606,2.) ;
#9168=VECTOR('',#38619,12.35000000085) ;
#9169=VECTOR('',#38622,2.5) ;
#9170=VECTOR('',#38623,2.5) ;
#9171=VECTOR('',#38626,2.5) ;
#9172=VECTOR('',#38627,2.5) ;
#9173=VECTOR('',#38630,2.5) ;
#9174=VECTOR('',#38631,2.5) ;
#9175=VECTOR('',#38636,2.5) ;
#9176=VECTOR('',#38639,2.5) ;
#9177=VECTOR('',#38640,2.5) ;
#9178=VECTOR('',#38643,2.5) ;
#9179=VECTOR('',#38646,2.5) ;
#9180=VECTOR('',#38651,2.5) ;
#9181=VECTOR('',#38652,2.5) ;
#9182=VECTOR('',#38655,2.5) ;
#9183=VECTOR('',#38658,2.5) ;
#9184=VECTOR('',#38663,2.5) ;
#9185=VECTOR('',#38664,2.5) ;
#9186=VECTOR('',#38667,2.5) ;
#9187=VECTOR('',#38670,2.5) ;
#9188=VECTOR('',#38679,2.5) ;
#9189=VECTOR('',#38680,2.5) ;
#9190=VECTOR('',#38683,2.5) ;
#9191=VECTOR('',#38686,2.5) ;
#9192=VECTOR('',#38691,2.5) ;
#9193=VECTOR('',#38692,4.) ;
#9194=VECTOR('',#38697,2.33) ;
#9195=VECTOR('',#38698,3.83) ;
#9196=VECTOR('',#38705,3.98) ;
#9197=VECTOR('',#38708,4.) ;
#9198=VECTOR('',#38713,2.33) ;
#9199=VECTOR('',#38714,3.83) ;
#9200=VECTOR('',#38719,41.3) ;
#9201=VECTOR('',#38726,23.00000000085) ;
#9202=VECTOR('',#38735,12.35) ;
#9203=VECTOR('',#38738,2.33) ;
#9204=VECTOR('',#38739,3.83) ;
#9205=VECTOR('',#38742,2.33) ;
#9206=VECTOR('',#38743,3.83) ;
#9207=VECTOR('',#38746,4.) ;
#9208=VECTOR('',#38747,2.5) ;
#9209=VECTOR('',#38750,4.) ;
#9210=VECTOR('',#38751,2.5) ;
#9211=VECTOR('',#38754,4.45) ;
#9212=VECTOR('',#38755,10.) ;
#9213=VECTOR('',#38756,10.) ;
#9214=VECTOR('',#38757,87.4) ;
#9215=VECTOR('',#38758,10.) ;
#9216=VECTOR('',#38759,10.) ;
#9217=VECTOR('',#38760,12.35000000085) ;
#9218=VECTOR('',#38763,79.40000000085) ;
#9219=VECTOR('',#38766,0.9) ;
#9220=VECTOR('',#38767,7.) ;
#9221=VECTOR('',#38780,10.) ;
#9222=VECTOR('',#38787,1.75) ;
#9223=VECTOR('',#38794,2.25) ;
#9224=VECTOR('',#38799,1.75) ;
#9225=VECTOR('',#38806,2.25) ;
#9226=VECTOR('',#38811,1.75) ;
#9227=VECTOR('',#38818,2.25) ;
#9228=VECTOR('',#38823,1.75) ;
#9229=VECTOR('',#38830,2.25) ;
#9230=VECTOR('',#38833,10.) ;
#9231=VECTOR('',#38834,2.5) ;
#9232=VECTOR('',#38835,2.5) ;
#9233=VECTOR('',#38846,2.5) ;
#9234=VECTOR('',#38849,3.83) ;
#9235=VECTOR('',#38850,2.33) ;
#9236=VECTOR('',#38853,2.33) ;
#9237=VECTOR('',#38854,3.83) ;
#9238=VECTOR('',#38855,2.5) ;
#9239=VECTOR('',#38858,2.5) ;
#9240=VECTOR('',#38859,2.5) ;
#9241=VECTOR('',#38862,2.5) ;
#9242=VECTOR('',#38865,2.5) ;
#9243=VECTOR('',#38870,2.25) ;
#9244=VECTOR('',#38871,7.) ;
#9245=VECTOR('',#38872,2.25) ;
#9246=VECTOR('',#38875,2.5) ;
#9247=VECTOR('',#38876,2.5) ;
#9248=VECTOR('',#38889,2.5) ;
#9249=VECTOR('',#38890,2.5) ;
#9250=VECTOR('',#38893,2.5) ;
#9251=VECTOR('',#38896,2.5) ;
#9252=VECTOR('',#38901,2.5) ;
#9253=VECTOR('',#38902,2.5) ;
#9254=VECTOR('',#38905,2.5) ;
#9255=VECTOR('',#38908,2.5) ;
#9256=VECTOR('',#38927,194.3) ;
#9257=VECTOR('',#38932,3.83) ;
#9258=VECTOR('',#38933,2.33) ;
#9259=VECTOR('',#38938,3.98) ;
#9260=VECTOR('',#38941,2.33) ;
#9261=VECTOR('',#38942,3.83) ;
#9262=VECTOR('',#38953,31.) ;
#9263=VECTOR('',#38954,1.65) ;
#9264=VECTOR('',#38955,1.65) ;
#9265=VECTOR('',#38960,1.65) ;
#9266=VECTOR('',#38965,2.2) ;
#9267=VECTOR('',#38968,10.) ;
#9268=VECTOR('',#38969,10.) ;
#9269=VECTOR('',#38970,10.) ;
#9270=VECTOR('',#38973,10.) ;
#9271=VECTOR('',#38974,10.) ;
#9272=VECTOR('',#38975,10.) ;
#9273=VECTOR('',#38978,10.) ;
#9274=VECTOR('',#38979,10.) ;
#9275=VECTOR('',#38980,10.) ;
#9276=VECTOR('',#38983,10.) ;
#9277=VECTOR('',#38984,10.) ;
#9278=VECTOR('',#38985,10.) ;
#9279=VECTOR('',#39038,10.) ;
#9280=VECTOR('',#39049,10.) ;
#9281=VECTOR('',#39056,10.) ;
#9282=VECTOR('',#39061,10.) ;
#9283=VECTOR('',#39066,10.) ;
#9284=VECTOR('',#39071,10.) ;
#9285=VECTOR('',#39084,10.) ;
#9286=VECTOR('',#39087,10.) ;
#9287=VECTOR('',#39100,10.) ;
#9288=VECTOR('',#39101,10.) ;
#9289=VECTOR('',#39102,9.99999999999998) ;
#9290=VECTOR('',#39103,9.99999999999998) ;
#9291=VECTOR('',#39104,10.) ;
#9292=VECTOR('',#39105,10.) ;
#9293=VECTOR('',#39106,10.) ;
#9294=VECTOR('',#39107,10.) ;
#9295=VECTOR('',#39108,9.99999999999998) ;
#9296=VECTOR('',#39109,9.99999999999998) ;
#9297=VECTOR('',#39110,10.) ;
#9298=VECTOR('',#39111,10.) ;
#9299=VECTOR('',#39112,10.) ;
#9300=VECTOR('',#39113,10.) ;
#9301=VECTOR('',#39114,9.99999999999998) ;
#9302=VECTOR('',#39115,9.99999999999998) ;
#9303=VECTOR('',#39116,10.) ;
#9304=VECTOR('',#39117,10.) ;
#9305=VECTOR('',#39120,10.) ;
#9306=VECTOR('',#39121,1000.) ;
#9307=VECTOR('',#39122,1000.) ;
#9308=VECTOR('',#39125,10.) ;
#9309=VECTOR('',#39126,1000.) ;
#9310=VECTOR('',#39129,10.) ;
#9311=VECTOR('',#39130,1000.) ;
#9312=VECTOR('',#39133,10.) ;
#9313=VECTOR('',#39134,1000.) ;
#9314=VECTOR('',#39137,9.99999999999998) ;
#9315=VECTOR('',#39138,1000.) ;
#9316=VECTOR('',#39141,9.99999999999998) ;
#9317=VECTOR('',#39144,10.) ;
#9318=VECTOR('',#39145,1000.) ;
#9319=VECTOR('',#39146,1000.) ;
#9320=VECTOR('',#39149,10.) ;
#9321=VECTOR('',#39150,1000.) ;
#9322=VECTOR('',#39153,10.) ;
#9323=VECTOR('',#39154,1000.) ;
#9324=VECTOR('',#39157,10.) ;
#9325=VECTOR('',#39158,1000.) ;
#9326=VECTOR('',#39161,9.99999999999998) ;
#9327=VECTOR('',#39162,1000.) ;
#9328=VECTOR('',#39165,9.99999999999998) ;
#9329=VECTOR('',#39168,10.) ;
#9330=VECTOR('',#39169,10.) ;
#9331=VECTOR('',#39170,10.) ;
#9332=VECTOR('',#39171,9.99999999999998) ;
#9333=VECTOR('',#39172,9.99999999999998) ;
#9334=VECTOR('',#39173,10.) ;
#9335=VECTOR('',#39176,1000.) ;
#9336=VECTOR('',#39177,1000.) ;
#9337=VECTOR('',#39180,1000.) ;
#9338=VECTOR('',#39183,1000.) ;
#9339=VECTOR('',#39186,1000.) ;
#9340=VECTOR('',#39189,1000.) ;
#11073=CIRCLE('',#33202,2.05475000000016) ;
#11074=CIRCLE('',#33205,2.05475000000007) ;
#11075=CIRCLE('',#33207,2.05475000000044) ;
#11076=CIRCLE('',#33210,2.0547500000002) ;
#11077=CIRCLE('',#33212,2.05475000000044) ;
#11078=CIRCLE('',#33215,2.0547500000002) ;
#11079=CIRCLE('',#33217,2.05475000000009) ;
#11080=CIRCLE('',#33220,2.05475) ;
#11081=CIRCLE('',#33222,1.66599999999999) ;
#11082=CIRCLE('',#33224,1.66599999999999) ;
#11083=CIRCLE('',#33226,1.66599999999999) ;
#11084=CIRCLE('',#33228,1.66599999999999) ;
#11085=CIRCLE('',#33230,1.66599999999999) ;
#11086=CIRCLE('',#33232,1.66599999999999) ;
#11087=CIRCLE('',#33234,1.66599999999999) ;
#11088=CIRCLE('',#33236,1.66599999999999) ;
#11089=CIRCLE('',#33238,1.66599999999999) ;
#11090=CIRCLE('',#33240,1.66599999999999) ;
#11091=CIRCLE('',#33242,1.66599999999999) ;
#11092=CIRCLE('',#33244,1.66599999999999) ;
#11093=CIRCLE('',#33246,2.05475) ;
#11094=CIRCLE('',#33249,2.05475) ;
#11095=CIRCLE('',#33251,2.05475) ;
#11096=CIRCLE('',#33254,2.05475) ;
#11097=CIRCLE('',#33256,1.666) ;
#11098=CIRCLE('',#33258,1.666) ;
#11099=CIRCLE('',#33260,1.666) ;
#11100=CIRCLE('',#33262,1.666) ;
#11101=CIRCLE('',#33264,1.666) ;
#11102=CIRCLE('',#33266,1.666) ;
#11103=CIRCLE('',#33268,2.05475) ;
#11104=CIRCLE('',#33271,2.05475) ;
#11105=CIRCLE('',#33273,2.05475) ;
#11106=CIRCLE('',#33276,2.05475) ;
#11107=CIRCLE('',#33278,1.66600000000001) ;
#11108=CIRCLE('',#33280,1.66600000000001) ;
#11109=CIRCLE('',#33282,1.66600000000001) ;
#11110=CIRCLE('',#33284,1.66600000000001) ;
#11111=CIRCLE('',#33286,1.66600000000001) ;
#11112=CIRCLE('',#33288,1.66600000000001) ;
#11113=CIRCLE('',#33306,0.5) ;
#11114=CIRCLE('',#33307,0.5) ;
#11115=CIRCLE('',#33309,2.) ;
#11116=CIRCLE('',#33310,2.) ;
#11117=CIRCLE('',#33312,2.) ;
#11118=CIRCLE('',#33313,2.) ;
#11119=CIRCLE('',#33315,2.) ;
#11120=CIRCLE('',#33316,2.) ;
#11121=CIRCLE('',#33318,2.) ;
#11122=CIRCLE('',#33319,2.) ;
#11123=CIRCLE('',#33321,0.5) ;
#11124=CIRCLE('',#33322,2.) ;
#11125=CIRCLE('',#33323,2.) ;
#11126=CIRCLE('',#33325,2.) ;
#11127=CIRCLE('',#33326,2.) ;
#11128=CIRCLE('',#33328,1.) ;
#11129=CIRCLE('',#33329,1.) ;
#11130=CIRCLE('',#33331,2.) ;
#11131=CIRCLE('',#33332,2.) ;
#11132=CIRCLE('',#33333,5.) ;
#11133=CIRCLE('',#33334,5.) ;
#11134=CIRCLE('',#33335,1.65) ;
#11135=CIRCLE('',#33336,1.65) ;
#11136=CIRCLE('',#33338,0.5) ;
#11137=CIRCLE('',#33339,0.5) ;
#11138=CIRCLE('',#33341,2.) ;
#11139=CIRCLE('',#33342,2.) ;
#11140=CIRCLE('',#33343,2.) ;
#11141=CIRCLE('',#33344,2.) ;
#11142=CIRCLE('',#33345,1.65) ;
#11143=CIRCLE('',#33346,1.65) ;
#11144=CIRCLE('',#33347,0.125) ;
#11145=CIRCLE('',#33348,0.125) ;
#11146=CIRCLE('',#33349,0.125) ;
#11147=CIRCLE('',#33350,0.125) ;
#11148=CIRCLE('',#33351,5.) ;
#11149=CIRCLE('',#33352,5.) ;
#11150=CIRCLE('',#33354,2.) ;
#11151=CIRCLE('',#33355,2.) ;
#11152=CIRCLE('',#33356,2.75) ;
#11153=CIRCLE('',#33357,5.25) ;
#11154=CIRCLE('',#33358,5.25) ;
#11155=CIRCLE('',#33359,2.75000000000003) ;
#11156=CIRCLE('',#33361,2.) ;
#11157=CIRCLE('',#33362,2.) ;
#11158=CIRCLE('',#33363,2.) ;
#11159=CIRCLE('',#33364,2.) ;
#11160=CIRCLE('',#33365,0.250000000000004) ;
#11161=CIRCLE('',#33366,0.250000000000012) ;
#11162=CIRCLE('',#33367,0.250000000000003) ;
#11163=CIRCLE('',#33368,0.249999999999986) ;
#11164=CIRCLE('',#33369,5.25) ;
#11165=CIRCLE('',#33370,5.25) ;
#11166=CIRCLE('',#33371,2.75) ;
#11167=CIRCLE('',#33372,2.7499999999968) ;
#11168=CIRCLE('',#33374,2.) ;
#11169=CIRCLE('',#33377,2.) ;
#11170=CIRCLE('',#33379,2.) ;
#11171=CIRCLE('',#33381,2.) ;
#11172=CIRCLE('',#33383,0.5) ;
#11173=CIRCLE('',#33384,0.5) ;
#11174=CIRCLE('',#33391,2.) ;
#11175=CIRCLE('',#33397,1.) ;
#11176=CIRCLE('',#33398,1.) ;
#11177=CIRCLE('',#33401,0.999999999999996) ;
#11178=CIRCLE('',#33402,1.) ;
#11179=CIRCLE('',#33404,0.999999404657181) ;
#11180=CIRCLE('',#33405,4.) ;
#11181=CIRCLE('',#33407,1.0000005953428) ;
#11182=CIRCLE('',#33409,1.00000000000001) ;
#11183=CIRCLE('',#33410,4.) ;
#11184=CIRCLE('',#33412,1.) ;
#11185=CIRCLE('',#33415,4.) ;
#11186=CIRCLE('',#33418,4.) ;
#11187=CIRCLE('',#33421,1.00000000000001) ;
#11188=CIRCLE('',#33422,1.) ;
#11189=CIRCLE('',#33424,0.999999404660006) ;
#11190=CIRCLE('',#33425,4.) ;
#11191=CIRCLE('',#33427,1.00000059533998) ;
#11192=CIRCLE('',#33429,0.999999999999979) ;
#11193=CIRCLE('',#33430,4.) ;
#11194=CIRCLE('',#33432,1.) ;
#11195=CIRCLE('',#33435,4.) ;
#11196=CIRCLE('',#33438,4.) ;
#11197=CIRCLE('',#33455,0.5) ;
#11198=CIRCLE('',#33456,0.5) ;
#11199=CIRCLE('',#33458,0.5) ;
#11200=CIRCLE('',#33459,0.5) ;
#11201=CIRCLE('',#33461,0.5) ;
#11202=CIRCLE('',#33463,0.5) ;
#11203=CIRCLE('',#33464,0.5) ;
#11204=CIRCLE('',#33466,0.5) ;
#11205=CIRCLE('',#33467,0.5) ;
#11206=CIRCLE('',#33470,1.65) ;
#11207=CIRCLE('',#33473,1.65) ;
#11208=CIRCLE('',#33476,1.65) ;
#11209=CIRCLE('',#33479,3.25) ;
#11210=CIRCLE('',#33481,3.25) ;
#11211=CIRCLE('',#33483,1.75) ;
#11212=CIRCLE('',#33484,1.75) ;
#11213=CIRCLE('',#33485,1.75) ;
#11214=CIRCLE('',#33487,2.75) ;
#11215=CIRCLE('',#33489,2.) ;
#11216=CIRCLE('',#33490,2.) ;
#11217=CIRCLE('',#33492,2.) ;
#11218=CIRCLE('',#33493,2.) ;
#11219=CIRCLE('',#33495,2.) ;
#11220=CIRCLE('',#33496,2.) ;
#11221=CIRCLE('',#33498,2.) ;
#11222=CIRCLE('',#33499,2.) ;
#11223=CIRCLE('',#33501,2.) ;
#11224=CIRCLE('',#33502,2.) ;
#11225=CIRCLE('',#33504,2.) ;
#11226=CIRCLE('',#33505,2.) ;
#11227=CIRCLE('',#33507,3.25) ;
#11228=CIRCLE('',#33508,3.25) ;
#11229=CIRCLE('',#33509,2.) ;
#11230=CIRCLE('',#33511,3.25) ;
#11231=CIRCLE('',#33530,3.25) ;
#11232=CIRCLE('',#33536,2.) ;
#11233=CIRCLE('',#33538,2.) ;
#11234=CIRCLE('',#33540,2.) ;
#11235=CIRCLE('',#33542,2.) ;
#11236=CIRCLE('',#33544,2.) ;
#11237=CIRCLE('',#33546,2.) ;
#11238=CIRCLE('',#33548,3.25) ;
#11239=CIRCLE('',#33550,3.25) ;
#11240=CIRCLE('',#33551,2.) ;
#11241=CIRCLE('',#33558,2.) ;
#11242=CIRCLE('',#33559,2.) ;
#11243=CIRCLE('',#33560,2.75) ;
#11244=CIRCLE('',#33561,2.75) ;
#11245=CIRCLE('',#33562,2.75) ;
#11246=CIRCLE('',#33563,2.75) ;
#11247=CIRCLE('',#33565,2.) ;
#11248=CIRCLE('',#33566,2.) ;
#11249=CIRCLE('',#33568,1.75) ;
#11250=CIRCLE('',#33569,1.75) ;
#11251=CIRCLE('',#33570,1.75) ;
#11252=CIRCLE('',#33573,1.75) ;
#11253=CIRCLE('',#33574,1.75) ;
#11254=CIRCLE('',#33575,1.75) ;
#11255=CIRCLE('',#33578,1.75) ;
#11256=CIRCLE('',#33579,1.75) ;
#11257=CIRCLE('',#33580,1.75) ;
#11258=CIRCLE('',#33583,1.75) ;
#11259=CIRCLE('',#33584,1.75) ;
#11260=CIRCLE('',#33585,1.75) ;
#11261=CIRCLE('',#33589,3.25) ;
#11262=CIRCLE('',#33591,3.25) ;
#11263=CIRCLE('',#33593,2.) ;
#11264=CIRCLE('',#33604,3.25) ;
#11265=CIRCLE('',#33605,3.25) ;
#11266=CIRCLE('',#33615,3.25) ;
#11267=CIRCLE('',#33616,3.25) ;
#11268=CIRCLE('',#33618,3.25) ;
#11269=CIRCLE('',#33620,3.25) ;
#11270=CIRCLE('',#33622,2.) ;
#11271=CIRCLE('',#33625,2.) ;
#11272=CIRCLE('',#33628,3.25) ;
#11273=CIRCLE('',#33629,3.25) ;
#11274=CIRCLE('',#33633,1.65000070880266) ;
#11275=CIRCLE('',#33634,1.65000070880266) ;
#11276=CIRCLE('',#33641,0.125000000000002) ;
#11277=CIRCLE('',#33643,0.124999999999993) ;
#11278=CIRCLE('',#33645,0.125000000000002) ;
#11279=CIRCLE('',#33646,0.125000000000028) ;
#11280=CIRCLE('',#33648,0.125000000000011) ;
#11281=CIRCLE('',#33650,0.125000000000002) ;
#11282=CIRCLE('',#33651,0.124999999999957) ;
#11283=CIRCLE('',#33653,0.125000000000002) ;
#11284=CIRCLE('',#33655,0.124999999999975) ;
#11285=CIRCLE('',#33656,0.125000000000028) ;
#11286=CIRCLE('',#33659,0.125000000000011) ;
#11287=CIRCLE('',#33660,0.125000000000028) ;
#11288=CIRCLE('',#33665,2.) ;
#11289=CIRCLE('',#33666,2.) ;
#11290=CIRCLE('',#33668,2.) ;
#11291=CIRCLE('',#33670,2.00000000000003) ;
#11292=CIRCLE('',#33672,2.) ;
#11293=CIRCLE('',#33675,1.99999999999999) ;
#11294=CIRCLE('',#33677,1.99999999999998) ;
#11295=CIRCLE('',#33679,2.) ;
#11296=CIRCLE('',#33680,2.) ;
#11297=CIRCLE('',#33681,2.) ;
#11298=CIRCLE('',#33683,1.99999999999996) ;
#11299=CIRCLE('',#33685,2.) ;
#11300=CIRCLE('',#33686,2.) ;
#11301=CIRCLE('',#33688,2.00000000000003) ;
#11302=CIRCLE('',#33689,1.99999999999999) ;
#11303=CIRCLE('',#33691,2.00000000000003) ;
#13050=VERTEX_POINT('',#50226) ;
#13051=VERTEX_POINT('',#50227) ;
#13052=VERTEX_POINT('',#50229) ;
#13053=VERTEX_POINT('',#50258) ;
#13054=VERTEX_POINT('',#50297) ;
#13055=VERTEX_POINT('',#50298) ;
#13056=VERTEX_POINT('',#50300) ;
#13057=VERTEX_POINT('',#50536) ;
#13058=VERTEX_POINT('',#50537) ;
#13059=VERTEX_POINT('',#50539) ;
#13060=VERTEX_POINT('',#50631) ;
#13061=VERTEX_POINT('',#50672) ;
#13062=VERTEX_POINT('',#50749) ;
#13063=VERTEX_POINT('',#50750) ;
#13064=VERTEX_POINT('',#50752) ;
#13065=VERTEX_POINT('',#50759) ;
#13066=VERTEX_POINT('',#50780) ;
#13067=VERTEX_POINT('',#50781) ;
#13068=VERTEX_POINT('',#50783) ;
#13069=VERTEX_POINT('',#50902) ;
#13070=VERTEX_POINT('',#51022) ;
#13071=VERTEX_POINT('',#51023) ;
#13072=VERTEX_POINT('',#51025) ;
#13073=VERTEX_POINT('',#51050) ;
#13074=VERTEX_POINT('',#51142) ;
#13075=VERTEX_POINT('',#51183) ;
#13076=VERTEX_POINT('',#51185) ;
#13077=VERTEX_POINT('',#51287) ;
#13078=VERTEX_POINT('',#51288) ;
#13079=VERTEX_POINT('',#51290) ;
#13080=VERTEX_POINT('',#51319) ;
#13081=VERTEX_POINT('',#51358) ;
#13082=VERTEX_POINT('',#51359) ;
#13083=VERTEX_POINT('',#51361) ;
#13084=VERTEX_POINT('',#51599) ;
#13085=VERTEX_POINT('',#51600) ;
#13086=VERTEX_POINT('',#51602) ;
#13087=VERTEX_POINT('',#51694) ;
#13088=VERTEX_POINT('',#51735) ;
#13089=VERTEX_POINT('',#51737) ;
#13090=VERTEX_POINT('',#51823) ;
#13091=VERTEX_POINT('',#51824) ;
#13092=VERTEX_POINT('',#51826) ;
#13093=VERTEX_POINT('',#51853) ;
#13094=VERTEX_POINT('',#51892) ;
#13095=VERTEX_POINT('',#51893) ;
#13096=VERTEX_POINT('',#51895) ;
#13097=VERTEX_POINT('',#52131) ;
#13098=VERTEX_POINT('',#52132) ;
#13099=VERTEX_POINT('',#52134) ;
#13100=VERTEX_POINT('',#52226) ;
#13101=VERTEX_POINT('',#52267) ;
#13102=VERTEX_POINT('',#52346) ;
#13103=VERTEX_POINT('',#52347) ;
#13104=VERTEX_POINT('',#52349) ;
#13105=VERTEX_POINT('',#52395) ;
#13106=VERTEX_POINT('',#52396) ;
#13107=VERTEX_POINT('',#52398) ;
#13108=VERTEX_POINT('',#52704) ;
#13109=VERTEX_POINT('',#52705) ;
#13110=VERTEX_POINT('',#52707) ;
#13111=VERTEX_POINT('',#52718) ;
#13112=VERTEX_POINT('',#52849) ;
#13113=VERTEX_POINT('',#52851) ;
#13114=VERTEX_POINT('',#53060) ;
#13115=VERTEX_POINT('',#53061) ;
#13116=VERTEX_POINT('',#53063) ;
#13117=VERTEX_POINT('',#53109) ;
#13118=VERTEX_POINT('',#53110) ;
#13119=VERTEX_POINT('',#53112) ;
#13120=VERTEX_POINT('',#53418) ;
#13121=VERTEX_POINT('',#53419) ;
#13122=VERTEX_POINT('',#53421) ;
#13123=VERTEX_POINT('',#53432) ;
#13124=VERTEX_POINT('',#53563) ;
#13125=VERTEX_POINT('',#53565) ;
#13126=VERTEX_POINT('',#53774) ;
#13127=VERTEX_POINT('',#53775) ;
#13128=VERTEX_POINT('',#53777) ;
#13129=VERTEX_POINT('',#53823) ;
#13130=VERTEX_POINT('',#53824) ;
#13131=VERTEX_POINT('',#53826) ;
#13132=VERTEX_POINT('',#54132) ;
#13133=VERTEX_POINT('',#54133) ;
#13134=VERTEX_POINT('',#54135) ;
#13135=VERTEX_POINT('',#54146) ;
#13136=VERTEX_POINT('',#54277) ;
#13137=VERTEX_POINT('',#54279) ;
#13138=VERTEX_POINT('',#54488) ;
#13139=VERTEX_POINT('',#54489) ;
#13140=VERTEX_POINT('',#54491) ;
#13141=VERTEX_POINT('',#54537) ;
#13142=VERTEX_POINT('',#54538) ;
#13143=VERTEX_POINT('',#54540) ;
#13144=VERTEX_POINT('',#54846) ;
#13145=VERTEX_POINT('',#54847) ;
#13146=VERTEX_POINT('',#54849) ;
#13147=VERTEX_POINT('',#54860) ;
#13148=VERTEX_POINT('',#54991) ;
#13149=VERTEX_POINT('',#54993) ;
#13150=VERTEX_POINT('',#55202) ;
#13151=VERTEX_POINT('',#55203) ;
#13152=VERTEX_POINT('',#55205) ;
#13153=VERTEX_POINT('',#55234) ;
#13154=VERTEX_POINT('',#55273) ;
#13155=VERTEX_POINT('',#55274) ;
#13156=VERTEX_POINT('',#55276) ;
#13157=VERTEX_POINT('',#55508) ;
#13158=VERTEX_POINT('',#55509) ;
#13159=VERTEX_POINT('',#55511) ;
#13160=VERTEX_POINT('',#55603) ;
#13161=VERTEX_POINT('',#55644) ;
#13162=VERTEX_POINT('',#55721) ;
#13163=VERTEX_POINT('',#55722) ;
#13164=VERTEX_POINT('',#55724) ;
#13165=VERTEX_POINT('',#55753) ;
#13166=VERTEX_POINT('',#55792) ;
#13167=VERTEX_POINT('',#55793) ;
#13168=VERTEX_POINT('',#55795) ;
#13169=VERTEX_POINT('',#56033) ;
#13170=VERTEX_POINT('',#56034) ;
#13171=VERTEX_POINT('',#56036) ;
#13172=VERTEX_POINT('',#56128) ;
#13173=VERTEX_POINT('',#56169) ;
#13174=VERTEX_POINT('',#56171) ;
#13175=VERTEX_POINT('',#56257) ;
#13176=VERTEX_POINT('',#56258) ;
#13177=VERTEX_POINT('',#56260) ;
#13178=VERTEX_POINT('',#56306) ;
#13179=VERTEX_POINT('',#56307) ;
#13180=VERTEX_POINT('',#56309) ;
#13181=VERTEX_POINT('',#56615) ;
#13182=VERTEX_POINT('',#56616) ;
#13183=VERTEX_POINT('',#56618) ;
#13184=VERTEX_POINT('',#56629) ;
#13185=VERTEX_POINT('',#56760) ;
#13186=VERTEX_POINT('',#56762) ;
#13187=VERTEX_POINT('',#56971) ;
#13188=VERTEX_POINT('',#56972) ;
#13189=VERTEX_POINT('',#56974) ;
#13190=VERTEX_POINT('',#57020) ;
#13191=VERTEX_POINT('',#57021) ;
#13192=VERTEX_POINT('',#57023) ;
#13193=VERTEX_POINT('',#57327) ;
#13194=VERTEX_POINT('',#57328) ;
#13195=VERTEX_POINT('',#57330) ;
#13196=VERTEX_POINT('',#57341) ;
#13197=VERTEX_POINT('',#57472) ;
#13198=VERTEX_POINT('',#57474) ;
#13199=VERTEX_POINT('',#57683) ;
#13200=VERTEX_POINT('',#57684) ;
#13201=VERTEX_POINT('',#57686) ;
#13202=VERTEX_POINT('',#57713) ;
#13203=VERTEX_POINT('',#57752) ;
#13204=VERTEX_POINT('',#57753) ;
#13205=VERTEX_POINT('',#57755) ;
#13206=VERTEX_POINT('',#57995) ;
#13207=VERTEX_POINT('',#57996) ;
#13208=VERTEX_POINT('',#57998) ;
#13209=VERTEX_POINT('',#58090) ;
#13210=VERTEX_POINT('',#58131) ;
#13211=VERTEX_POINT('',#58212) ;
#13212=VERTEX_POINT('',#58213) ;
#13213=VERTEX_POINT('',#58215) ;
#13214=VERTEX_POINT('',#58242) ;
#13215=VERTEX_POINT('',#58281) ;
#13216=VERTEX_POINT('',#58282) ;
#13217=VERTEX_POINT('',#58284) ;
#13218=VERTEX_POINT('',#58522) ;
#13219=VERTEX_POINT('',#58523) ;
#13220=VERTEX_POINT('',#58525) ;
#13221=VERTEX_POINT('',#58617) ;
#13222=VERTEX_POINT('',#58658) ;
#13223=VERTEX_POINT('',#58735) ;
#13224=VERTEX_POINT('',#58736) ;
#13225=VERTEX_POINT('',#58738) ;
#13226=VERTEX_POINT('',#58784) ;
#13227=VERTEX_POINT('',#58785) ;
#13228=VERTEX_POINT('',#58787) ;
#13229=VERTEX_POINT('',#59093) ;
#13230=VERTEX_POINT('',#59094) ;
#13231=VERTEX_POINT('',#59096) ;
#13232=VERTEX_POINT('',#59107) ;
#13233=VERTEX_POINT('',#59238) ;
#13234=VERTEX_POINT('',#59240) ;
#13235=VERTEX_POINT('',#59449) ;
#13236=VERTEX_POINT('',#59450) ;
#13237=VERTEX_POINT('',#59452) ;
#13238=VERTEX_POINT('',#59498) ;
#13239=VERTEX_POINT('',#59499) ;
#13240=VERTEX_POINT('',#59501) ;
#13241=VERTEX_POINT('',#59807) ;
#13242=VERTEX_POINT('',#59808) ;
#13243=VERTEX_POINT('',#59810) ;
#13244=VERTEX_POINT('',#59821) ;
#13245=VERTEX_POINT('',#59952) ;
#13246=VERTEX_POINT('',#59954) ;
#13247=VERTEX_POINT('',#61455) ;
#13248=VERTEX_POINT('',#62981) ;
#13249=VERTEX_POINT('',#63657) ;
#13250=VERTEX_POINT('',#63658) ;
#13251=VERTEX_POINT('',#63660) ;
#13252=VERTEX_POINT('',#63662) ;
#13253=VERTEX_POINT('',#63666) ;
#13254=VERTEX_POINT('',#63667) ;
#13255=VERTEX_POINT('',#63669) ;
#13256=VERTEX_POINT('',#63671) ;
#13257=VERTEX_POINT('',#63675) ;
#13258=VERTEX_POINT('',#63676) ;
#13259=VERTEX_POINT('',#63678) ;
#13260=VERTEX_POINT('',#63680) ;
#13261=VERTEX_POINT('',#63684) ;
#13262=VERTEX_POINT('',#63685) ;
#13263=VERTEX_POINT('',#63687) ;
#13264=VERTEX_POINT('',#63689) ;
#13265=VERTEX_POINT('',#63693) ;
#13266=VERTEX_POINT('',#63694) ;
#13267=VERTEX_POINT('',#63696) ;
#13268=VERTEX_POINT('',#63698) ;
#13269=VERTEX_POINT('',#63702) ;
#13270=VERTEX_POINT('',#63704) ;
#13271=VERTEX_POINT('',#63707) ;
#13272=VERTEX_POINT('',#63709) ;
#13273=VERTEX_POINT('',#63711) ;
#13274=VERTEX_POINT('',#63713) ;
#13275=VERTEX_POINT('',#63718) ;
#13276=VERTEX_POINT('',#63719) ;
#13277=VERTEX_POINT('',#63721) ;
#13278=VERTEX_POINT('',#63723) ;
#13279=VERTEX_POINT('',#63727) ;
#13280=VERTEX_POINT('',#63728) ;
#13281=VERTEX_POINT('',#63730) ;
#13282=VERTEX_POINT('',#63732) ;
#13283=VERTEX_POINT('',#63737) ;
#13284=VERTEX_POINT('',#63739) ;
#13285=VERTEX_POINT('',#63741) ;
#13286=VERTEX_POINT('',#63743) ;
#13287=VERTEX_POINT('',#63745) ;
#13288=VERTEX_POINT('',#63747) ;
#13289=VERTEX_POINT('',#63749) ;
#13290=VERTEX_POINT('',#63751) ;
#13291=VERTEX_POINT('',#63753) ;
#13292=VERTEX_POINT('',#63755) ;
#13293=VERTEX_POINT('',#63757) ;
#13294=VERTEX_POINT('',#63760) ;
#13295=VERTEX_POINT('',#63761) ;
#13296=VERTEX_POINT('',#63763) ;
#13297=VERTEX_POINT('',#63765) ;
#13298=VERTEX_POINT('',#63767) ;
#13299=VERTEX_POINT('',#63769) ;
#13300=VERTEX_POINT('',#63771) ;
#13301=VERTEX_POINT('',#63773) ;
#13302=VERTEX_POINT('',#63775) ;
#13303=VERTEX_POINT('',#63777) ;
#13304=VERTEX_POINT('',#63779) ;
#13305=VERTEX_POINT('',#63781) ;
#13306=VERTEX_POINT('',#63783) ;
#13307=VERTEX_POINT('',#63785) ;
#13308=VERTEX_POINT('',#63788) ;
#13309=VERTEX_POINT('',#63963) ;
#13310=VERTEX_POINT('',#64138) ;
#13311=VERTEX_POINT('',#64140) ;
#13312=VERTEX_POINT('',#64141) ;
#13313=VERTEX_POINT('',#64143) ;
#13314=VERTEX_POINT('',#64145) ;
#13315=VERTEX_POINT('',#64148) ;
#13316=VERTEX_POINT('',#64149) ;
#13317=VERTEX_POINT('',#64151) ;
#13318=VERTEX_POINT('',#64153) ;
#13319=VERTEX_POINT('',#64156) ;
#13320=VERTEX_POINT('',#64157) ;
#13321=VERTEX_POINT('',#64159) ;
#13322=VERTEX_POINT('',#64161) ;
#13323=VERTEX_POINT('',#64164) ;
#13324=VERTEX_POINT('',#64167) ;
#13325=VERTEX_POINT('',#64168) ;
#13326=VERTEX_POINT('',#64170) ;
#13327=VERTEX_POINT('',#64172) ;
#13328=VERTEX_POINT('',#64177) ;
#13329=VERTEX_POINT('',#64179) ;
#13330=VERTEX_POINT('',#64182) ;
#13331=VERTEX_POINT('',#64184) ;
#13332=VERTEX_POINT('',#64186) ;
#13333=VERTEX_POINT('',#64188) ;
#13334=VERTEX_POINT('',#64190) ;
#13335=VERTEX_POINT('',#64192) ;
#13336=VERTEX_POINT('',#64194) ;
#13337=VERTEX_POINT('',#64196) ;
#13338=VERTEX_POINT('',#64198) ;
#13339=VERTEX_POINT('',#64200) ;
#13340=VERTEX_POINT('',#64202) ;
#13341=VERTEX_POINT('',#64204) ;
#13342=VERTEX_POINT('',#64206) ;
#13343=VERTEX_POINT('',#64208) ;
#13344=VERTEX_POINT('',#64211) ;
#13345=VERTEX_POINT('',#64213) ;
#13346=VERTEX_POINT('',#64214) ;
#13347=VERTEX_POINT('',#64216) ;
#13348=VERTEX_POINT('',#64218) ;
#13349=VERTEX_POINT('',#64221) ;
#13350=VERTEX_POINT('',#64222) ;
#13351=VERTEX_POINT('',#64224) ;
#13352=VERTEX_POINT('',#64226) ;
#13353=VERTEX_POINT('',#64229) ;
#13354=VERTEX_POINT('',#64230) ;
#13355=VERTEX_POINT('',#64232) ;
#13356=VERTEX_POINT('',#64234) ;
#13357=VERTEX_POINT('',#64237) ;
#13358=VERTEX_POINT('',#64238) ;
#13359=VERTEX_POINT('',#64240) ;
#13360=VERTEX_POINT('',#64242) ;
#13361=VERTEX_POINT('',#64245) ;
#13362=VERTEX_POINT('',#64247) ;
#13363=VERTEX_POINT('',#64422) ;
#13364=VERTEX_POINT('',#64597) ;
#13365=VERTEX_POINT('',#64598) ;
#13366=VERTEX_POINT('',#64600) ;
#13367=VERTEX_POINT('',#64602) ;
#13368=VERTEX_POINT('',#64604) ;
#13369=VERTEX_POINT('',#64606) ;
#13370=VERTEX_POINT('',#64608) ;
#13371=VERTEX_POINT('',#64610) ;
#13372=VERTEX_POINT('',#64613) ;
#13373=VERTEX_POINT('',#64614) ;
#13374=VERTEX_POINT('',#64616) ;
#13375=VERTEX_POINT('',#64618) ;
#13376=VERTEX_POINT('',#64620) ;
#13377=VERTEX_POINT('',#64622) ;
#13378=VERTEX_POINT('',#64624) ;
#13379=VERTEX_POINT('',#64626) ;
#13380=VERTEX_POINT('',#64628) ;
#13381=VERTEX_POINT('',#64630) ;
#13382=VERTEX_POINT('',#64634) ;
#13383=VERTEX_POINT('',#64636) ;
#13384=VERTEX_POINT('',#64638) ;
#13385=VERTEX_POINT('',#64640) ;
#13386=VERTEX_POINT('',#64642) ;
#13387=VERTEX_POINT('',#64644) ;
#13388=VERTEX_POINT('',#64646) ;
#13389=VERTEX_POINT('',#64648) ;
#13390=VERTEX_POINT('',#64650) ;
#13391=VERTEX_POINT('',#64652) ;
#13392=VERTEX_POINT('',#64654) ;
#13393=VERTEX_POINT('',#64658) ;
#13394=VERTEX_POINT('',#64660) ;
#13395=VERTEX_POINT('',#64661) ;
#13396=VERTEX_POINT('',#64663) ;
#13397=VERTEX_POINT('',#64665) ;
#13398=VERTEX_POINT('',#64668) ;
#13399=VERTEX_POINT('',#64669) ;
#13400=VERTEX_POINT('',#64671) ;
#13401=VERTEX_POINT('',#64673) ;
#13402=VERTEX_POINT('',#64676) ;
#13403=VERTEX_POINT('',#64677) ;
#13404=VERTEX_POINT('',#64679) ;
#13405=VERTEX_POINT('',#64681) ;
#13406=VERTEX_POINT('',#64684) ;
#13407=VERTEX_POINT('',#64685) ;
#13408=VERTEX_POINT('',#64687) ;
#13409=VERTEX_POINT('',#64689) ;
#13410=VERTEX_POINT('',#64691) ;
#13411=VERTEX_POINT('',#64693) ;
#13412=VERTEX_POINT('',#64696) ;
#13413=VERTEX_POINT('',#64780) ;
#13414=VERTEX_POINT('',#64955) ;
#13415=VERTEX_POINT('',#65049) ;
#13416=VERTEX_POINT('',#65051) ;
#13417=VERTEX_POINT('',#65053) ;
#13418=VERTEX_POINT('',#65055) ;
#13419=VERTEX_POINT('',#65057) ;
#13420=VERTEX_POINT('',#65059) ;
#13421=VERTEX_POINT('',#65061) ;
#13422=VERTEX_POINT('',#65063) ;
#13423=VERTEX_POINT('',#65065) ;
#13424=VERTEX_POINT('',#65067) ;
#13425=VERTEX_POINT('',#65069) ;
#13426=VERTEX_POINT('',#65071) ;
#13427=VERTEX_POINT('',#65073) ;
#13428=VERTEX_POINT('',#65075) ;
#13429=VERTEX_POINT('',#65077) ;
#13430=VERTEX_POINT('',#65079) ;
#13431=VERTEX_POINT('',#65081) ;
#13432=VERTEX_POINT('',#65083) ;
#13433=VERTEX_POINT('',#65085) ;
#13434=VERTEX_POINT('',#65089) ;
#13435=VERTEX_POINT('',#65090) ;
#13436=VERTEX_POINT('',#65092) ;
#13437=VERTEX_POINT('',#65094) ;
#13438=VERTEX_POINT('',#65096) ;
#13439=VERTEX_POINT('',#65098) ;
#13440=VERTEX_POINT('',#65100) ;
#13441=VERTEX_POINT('',#65102) ;
#13442=VERTEX_POINT('',#65187) ;
#13443=VERTEX_POINT('',#65362) ;
#13444=VERTEX_POINT('',#65455) ;
#13445=VERTEX_POINT('',#65456) ;
#13446=VERTEX_POINT('',#65458) ;
#13447=VERTEX_POINT('',#65460) ;
#13448=VERTEX_POINT('',#65462) ;
#13449=VERTEX_POINT('',#65464) ;
#13450=VERTEX_POINT('',#65467) ;
#13451=VERTEX_POINT('',#65468) ;
#13452=VERTEX_POINT('',#65470) ;
#13453=VERTEX_POINT('',#65472) ;
#13454=VERTEX_POINT('',#65475) ;
#13455=VERTEX_POINT('',#65476) ;
#13456=VERTEX_POINT('',#65478) ;
#13457=VERTEX_POINT('',#65480) ;
#13458=VERTEX_POINT('',#65483) ;
#13459=VERTEX_POINT('',#65484) ;
#13460=VERTEX_POINT('',#65486) ;
#13461=VERTEX_POINT('',#65488) ;
#13462=VERTEX_POINT('',#65491) ;
#13463=VERTEX_POINT('',#65492) ;
#13464=VERTEX_POINT('',#65494) ;
#13465=VERTEX_POINT('',#65496) ;
#13466=VERTEX_POINT('',#65499) ;
#13467=VERTEX_POINT('',#65501) ;
#13468=VERTEX_POINT('',#65504) ;
#13469=VERTEX_POINT('',#65506) ;
#13470=VERTEX_POINT('',#65512) ;
#13471=VERTEX_POINT('',#65514) ;
#13472=VERTEX_POINT('',#65516) ;
#13473=VERTEX_POINT('',#65518) ;
#13474=VERTEX_POINT('',#65529) ;
#13475=VERTEX_POINT('',#65531) ;
#13476=VERTEX_POINT('',#65535) ;
#13477=VERTEX_POINT('',#65539) ;
#13478=VERTEX_POINT('',#65543) ;
#13479=VERTEX_POINT('',#65547) ;
#13480=VERTEX_POINT('',#65549) ;
#13481=VERTEX_POINT('',#65555) ;
#13482=VERTEX_POINT('',#65557) ;
#13483=VERTEX_POINT('',#65561) ;
#13484=VERTEX_POINT('',#65608) ;
#13485=VERTEX_POINT('',#65621) ;
#13486=VERTEX_POINT('',#65625) ;
#13487=VERTEX_POINT('',#65631) ;
#13488=VERTEX_POINT('',#65640) ;
#13489=VERTEX_POINT('',#65646) ;
#13490=VERTEX_POINT('',#65648) ;
#13491=VERTEX_POINT('',#65652) ;
#13492=VERTEX_POINT('',#65654) ;
#13493=VERTEX_POINT('',#65658) ;
#13494=VERTEX_POINT('',#65660) ;
#13495=VERTEX_POINT('',#65664) ;
#13496=VERTEX_POINT('',#65668) ;
#13497=VERTEX_POINT('',#65672) ;
#13498=VERTEX_POINT('',#65676) ;
#13499=VERTEX_POINT('',#65680) ;
#13500=VERTEX_POINT('',#65682) ;
#13501=VERTEX_POINT('',#65686) ;
#13502=VERTEX_POINT('',#65690) ;
#13503=VERTEX_POINT('',#65694) ;
#13504=VERTEX_POINT('',#65698) ;
#13505=VERTEX_POINT('',#65702) ;
#13506=VERTEX_POINT('',#65704) ;
#13507=VERTEX_POINT('',#65708) ;
#13508=VERTEX_POINT('',#65712) ;
#13509=VERTEX_POINT('',#65716) ;
#13510=VERTEX_POINT('',#65720) ;
#13511=VERTEX_POINT('',#65724) ;
#13512=VERTEX_POINT('',#65726) ;
#13513=VERTEX_POINT('',#65730) ;
#13514=VERTEX_POINT('',#65734) ;
#13515=VERTEX_POINT('',#65738) ;
#13516=VERTEX_POINT('',#65742) ;
#13517=VERTEX_POINT('',#65746) ;
#13518=VERTEX_POINT('',#65747) ;
#13519=VERTEX_POINT('',#65749) ;
#13520=VERTEX_POINT('',#65751) ;
#13521=VERTEX_POINT('',#65755) ;
#13522=VERTEX_POINT('',#65757) ;
#13523=VERTEX_POINT('',#65761) ;
#13524=VERTEX_POINT('',#65763) ;
#13525=VERTEX_POINT('',#65767) ;
#13526=VERTEX_POINT('',#65769) ;
#13527=VERTEX_POINT('',#65773) ;
#13528=VERTEX_POINT('',#65775) ;
#13529=VERTEX_POINT('',#65782) ;
#13530=VERTEX_POINT('',#65783) ;
#13531=VERTEX_POINT('',#65785) ;
#13532=VERTEX_POINT('',#65787) ;
#13533=VERTEX_POINT('',#65791) ;
#13534=VERTEX_POINT('',#65793) ;
#13535=VERTEX_POINT('',#65797) ;
#13536=VERTEX_POINT('',#65799) ;
#13537=VERTEX_POINT('',#65803) ;
#13538=VERTEX_POINT('',#65805) ;
#13539=VERTEX_POINT('',#65809) ;
#13540=VERTEX_POINT('',#65811) ;
#13541=VERTEX_POINT('',#65820) ;
#13542=VERTEX_POINT('',#65822) ;
#13543=VERTEX_POINT('',#65826) ;
#13544=VERTEX_POINT('',#65828) ;
#13545=VERTEX_POINT('',#65832) ;
#13546=VERTEX_POINT('',#65836) ;
#13547=VERTEX_POINT('',#65838) ;
#13548=VERTEX_POINT('',#65842) ;
#13549=VERTEX_POINT('',#65844) ;
#13550=VERTEX_POINT('',#65848) ;
#13551=VERTEX_POINT('',#65850) ;
#13552=VERTEX_POINT('',#65855) ;
#13553=VERTEX_POINT('',#65861) ;
#13554=VERTEX_POINT('',#65867) ;
#13555=VERTEX_POINT('',#65873) ;
#13556=VERTEX_POINT('',#65877) ;
#13557=VERTEX_POINT('',#65881) ;
#13558=VERTEX_POINT('',#65883) ;
#13559=VERTEX_POINT('',#65885) ;
#13560=VERTEX_POINT('',#65889) ;
#13561=VERTEX_POINT('',#65893) ;
#13562=VERTEX_POINT('',#65894) ;
#13563=VERTEX_POINT('',#65896) ;
#13564=VERTEX_POINT('',#65898) ;
#13565=VERTEX_POINT('',#65902) ;
#13566=VERTEX_POINT('',#65903) ;
#13567=VERTEX_POINT('',#65905) ;
#13568=VERTEX_POINT('',#65907) ;
#13569=VERTEX_POINT('',#65911) ;
#13570=VERTEX_POINT('',#65912) ;
#13571=VERTEX_POINT('',#65914) ;
#13572=VERTEX_POINT('',#65916) ;
#13573=VERTEX_POINT('',#65920) ;
#13574=VERTEX_POINT('',#65921) ;
#13575=VERTEX_POINT('',#65923) ;
#13576=VERTEX_POINT('',#65925) ;
#13577=VERTEX_POINT('',#65929) ;
#13578=VERTEX_POINT('',#65931) ;
#13579=VERTEX_POINT('',#65935) ;
#13580=VERTEX_POINT('',#65936) ;
#13581=VERTEX_POINT('',#65938) ;
#13582=VERTEX_POINT('',#65940) ;
#13583=VERTEX_POINT('',#65944) ;
#13584=VERTEX_POINT('',#65946) ;
#13585=VERTEX_POINT('',#66000) ;
#13586=VERTEX_POINT('',#66005) ;
#13587=VERTEX_POINT('',#66009) ;
#13588=VERTEX_POINT('',#66013) ;
#13589=VERTEX_POINT('',#66018) ;
#13590=VERTEX_POINT('',#66022) ;
#13591=VERTEX_POINT('',#66026) ;
#13592=VERTEX_POINT('',#66030) ;
#13593=VERTEX_POINT('',#66048) ;
#13594=VERTEX_POINT('',#66049) ;
#13595=VERTEX_POINT('',#66052) ;
#13596=VERTEX_POINT('',#66054) ;
#13597=VERTEX_POINT('',#66057) ;
#13598=VERTEX_POINT('',#66059) ;
#13599=VERTEX_POINT('',#66061) ;
#13600=VERTEX_POINT('',#66063) ;
#13601=VERTEX_POINT('',#66065) ;
#13602=VERTEX_POINT('',#66067) ;
#13603=VERTEX_POINT('',#66070) ;
#13604=VERTEX_POINT('',#66072) ;
#13605=VERTEX_POINT('',#66074) ;
#13606=VERTEX_POINT('',#66076) ;
#13607=VERTEX_POINT('',#66079) ;
#13608=VERTEX_POINT('',#66081) ;
#13609=VERTEX_POINT('',#66085) ;
#13610=VERTEX_POINT('',#66087) ;
#13611=VERTEX_POINT('',#66089) ;
#13612=VERTEX_POINT('',#66095) ;
#13613=VERTEX_POINT('',#66097) ;
#13614=VERTEX_POINT('',#66099) ;
#13615=VERTEX_POINT('',#66105) ;
#13616=VERTEX_POINT('',#66107) ;
#13617=VERTEX_POINT('',#66109) ;
#13618=VERTEX_POINT('',#66115) ;
#13619=VERTEX_POINT('',#66117) ;
#13620=VERTEX_POINT('',#66119) ;
#13621=VERTEX_POINT('',#66125) ;
#13622=VERTEX_POINT('',#66126) ;
#13623=VERTEX_POINT('',#66136) ;
#13624=VERTEX_POINT('',#66153) ;
#13625=VERTEX_POINT('',#66155) ;
#13626=VERTEX_POINT('',#66190) ;
#13627=VERTEX_POINT('',#66197) ;
#13628=VERTEX_POINT('',#66208) ;
#13629=VERTEX_POINT('',#66209) ;
#13630=VERTEX_POINT('',#66214) ;
#13631=VERTEX_POINT('',#66215) ;
#13632=VERTEX_POINT('',#66958) ;
#13633=VERTEX_POINT('',#66960) ;
#13634=VERTEX_POINT('',#66964) ;
#13635=VERTEX_POINT('',#66966) ;
#13636=VERTEX_POINT('',#66970) ;
#13637=VERTEX_POINT('',#66972) ;
#13638=VERTEX_POINT('',#66976) ;
#13639=VERTEX_POINT('',#66978) ;
#13640=VERTEX_POINT('',#67006) ;
#13641=VERTEX_POINT('',#67008) ;
#13642=VERTEX_POINT('',#67014) ;
#13643=VERTEX_POINT('',#67022) ;
#13644=VERTEX_POINT('',#67026) ;
#13645=VERTEX_POINT('',#67030) ;
#13646=VERTEX_POINT('',#67032) ;
#13647=VERTEX_POINT('',#67057) ;
#13648=VERTEX_POINT('',#67059) ;
#13649=VERTEX_POINT('',#67061) ;
#13650=VERTEX_POINT('',#67261) ;
#13651=VERTEX_POINT('',#67446) ;
#13652=VERTEX_POINT('',#67795) ;
#13653=VERTEX_POINT('',#67980) ;
#13654=VERTEX_POINT('',#68329) ;
#13655=VERTEX_POINT('',#68514) ;
#13656=VERTEX_POINT('',#68690) ;
#13657=VERTEX_POINT('',#68691) ;
#13658=VERTEX_POINT('',#68693) ;
#13659=VERTEX_POINT('',#68695) ;
#13660=VERTEX_POINT('',#68697) ;
#13661=VERTEX_POINT('',#68699) ;
#13662=VERTEX_POINT('',#68702) ;
#13663=VERTEX_POINT('',#68703) ;
#13664=VERTEX_POINT('',#68705) ;
#13665=VERTEX_POINT('',#68707) ;
#13666=VERTEX_POINT('',#68709) ;
#13667=VERTEX_POINT('',#68711) ;
#13668=VERTEX_POINT('',#68714) ;
#13669=VERTEX_POINT('',#68715) ;
#13670=VERTEX_POINT('',#68717) ;
#13671=VERTEX_POINT('',#68719) ;
#13672=VERTEX_POINT('',#68721) ;
#13673=VERTEX_POINT('',#68723) ;
#13674=VERTEX_POINT('',#68808) ;
#13675=VERTEX_POINT('',#69167) ;
#13676=VERTEX_POINT('',#69261) ;
#13677=VERTEX_POINT('',#69262) ;
#13678=VERTEX_POINT('',#69267) ;
#13679=VERTEX_POINT('',#69271) ;
#13680=VERTEX_POINT('',#69275) ;
#13681=VERTEX_POINT('',#69279) ;
#13682=VERTEX_POINT('',#69285) ;
#13683=VERTEX_POINT('',#69286) ;
#13684=VERTEX_POINT('',#69291) ;
#13685=VERTEX_POINT('',#69295) ;
#13686=VERTEX_POINT('',#69299) ;
#13687=VERTEX_POINT('',#69303) ;
#13688=VERTEX_POINT('',#69309) ;
#13689=VERTEX_POINT('',#69310) ;
#13690=VERTEX_POINT('',#69312) ;
#13691=VERTEX_POINT('',#69314) ;
#13692=VERTEX_POINT('',#69316) ;
#13693=VERTEX_POINT('',#69318) ;
#16181=EDGE_CURVE('',#13050,#13051,#6505,.T.) ;
#16182=EDGE_CURVE('',#13051,#13052,#1256,.T.) ;
#16183=EDGE_CURVE('',#13053,#13052,#11073,.T.) ;
#16184=EDGE_CURVE('',#13050,#13053,#1257,.F.) ;
#16185=EDGE_CURVE('',#13054,#13055,#6506,.T.) ;
#16186=EDGE_CURVE('',#13055,#13056,#1258,.T.) ;
#16187=EDGE_CURVE('',#13056,#13051,#1259,.T.) ;
#16188=EDGE_CURVE('',#13054,#13050,#1260,.F.) ;
#16189=EDGE_CURVE('',#13057,#13058,#6507,.T.) ;
#16190=EDGE_CURVE('',#13059,#13057,#1261,.T.) ;
#16191=EDGE_CURVE('',#13060,#13059,#1262,.T.) ;
#16192=EDGE_CURVE('',#13061,#13060,#11074,.T.) ;
#16193=EDGE_CURVE('',#13061,#13058,#1263,.T.) ;
#16194=EDGE_CURVE('',#13062,#13063,#6508,.T.) ;
#16195=EDGE_CURVE('',#13063,#13064,#1264,.T.) ;
#16196=EDGE_CURVE('',#13065,#13064,#11075,.T.) ;
#16197=EDGE_CURVE('',#13062,#13065,#1265,.F.) ;
#16198=EDGE_CURVE('',#13066,#13067,#6509,.T.) ;
#16199=EDGE_CURVE('',#13067,#13068,#1266,.T.) ;
#16200=EDGE_CURVE('',#13068,#13063,#1267,.T.) ;
#16201=EDGE_CURVE('',#13069,#13062,#1268,.F.) ;
#16202=EDGE_CURVE('',#13066,#13069,#1269,.F.) ;
#16203=EDGE_CURVE('',#13070,#13071,#6510,.T.) ;
#16204=EDGE_CURVE('',#13072,#13070,#1270,.F.) ;
#16205=EDGE_CURVE('',#13073,#13072,#1271,.T.) ;
#16206=EDGE_CURVE('',#13074,#13073,#1272,.T.) ;
#16207=EDGE_CURVE('',#13075,#13074,#11076,.T.) ;
#16208=EDGE_CURVE('',#13075,#13076,#1273,.T.) ;
#16209=EDGE_CURVE('',#13076,#13071,#1274,.T.) ;
#16210=EDGE_CURVE('',#13077,#13078,#6511,.T.) ;
#16211=EDGE_CURVE('',#13078,#13079,#1275,.T.) ;
#16212=EDGE_CURVE('',#13080,#13079,#11077,.T.) ;
#16213=EDGE_CURVE('',#13077,#13080,#1276,.F.) ;
#16214=EDGE_CURVE('',#13081,#13082,#6512,.T.) ;
#16215=EDGE_CURVE('',#13082,#13083,#1277,.T.) ;
#16216=EDGE_CURVE('',#13083,#13078,#1278,.T.) ;
#16217=EDGE_CURVE('',#13081,#13077,#1279,.F.) ;
#16218=EDGE_CURVE('',#13084,#13085,#6513,.T.) ;
#16219=EDGE_CURVE('',#13086,#13084,#1280,.T.) ;
#16220=EDGE_CURVE('',#13087,#13086,#1281,.T.) ;
#16221=EDGE_CURVE('',#13088,#13087,#11078,.T.) ;
#16222=EDGE_CURVE('',#13088,#13089,#1282,.T.) ;
#16223=EDGE_CURVE('',#13089,#13085,#1283,.T.) ;
#16224=EDGE_CURVE('',#13090,#13091,#6514,.T.) ;
#16225=EDGE_CURVE('',#13091,#13092,#1284,.T.) ;
#16226=EDGE_CURVE('',#13093,#13092,#11079,.T.) ;
#16227=EDGE_CURVE('',#13090,#13093,#1285,.F.) ;
#16228=EDGE_CURVE('',#13094,#13095,#6515,.T.) ;
#16229=EDGE_CURVE('',#13095,#13096,#1286,.T.) ;
#16230=EDGE_CURVE('',#13096,#13091,#1287,.T.) ;
#16231=EDGE_CURVE('',#13094,#13090,#1288,.F.) ;
#16232=EDGE_CURVE('',#13097,#13098,#6516,.T.) ;
#16233=EDGE_CURVE('',#13099,#13097,#1289,.T.) ;
#16234=EDGE_CURVE('',#13100,#13099,#1290,.T.) ;
#16235=EDGE_CURVE('',#13101,#13100,#11080,.T.) ;
#16236=EDGE_CURVE('',#13101,#13098,#1291,.T.) ;
#16237=EDGE_CURVE('',#13102,#13103,#6517,.T.) ;
#16238=EDGE_CURVE('',#13104,#13103,#11081,.T.) ;
#16239=EDGE_CURVE('',#13104,#13102,#1292,.T.) ;
#16240=EDGE_CURVE('',#13105,#13106,#6518,.T.) ;
#16241=EDGE_CURVE('',#13106,#13107,#1293,.T.) ;
#16242=EDGE_CURVE('',#13103,#13107,#11082,.T.) ;
#16243=EDGE_CURVE('',#13102,#13105,#1294,.F.) ;
#16244=EDGE_CURVE('',#13108,#13109,#6519,.T.) ;
#16245=EDGE_CURVE('',#13108,#13110,#1295,.F.) ;
#16246=EDGE_CURVE('',#13110,#13111,#1296,.T.) ;
#16247=EDGE_CURVE('',#13112,#13111,#11083,.T.) ;
#16248=EDGE_CURVE('',#13112,#13113,#1297,.T.) ;
#16249=EDGE_CURVE('',#13113,#13109,#1298,.T.) ;
#16250=EDGE_CURVE('',#13114,#13115,#6520,.T.) ;
#16251=EDGE_CURVE('',#13116,#13115,#11084,.T.) ;
#16252=EDGE_CURVE('',#13116,#13114,#1299,.T.) ;
#16253=EDGE_CURVE('',#13117,#13118,#6521,.T.) ;
#16254=EDGE_CURVE('',#13118,#13119,#1300,.T.) ;
#16255=EDGE_CURVE('',#13115,#13119,#11085,.T.) ;
#16256=EDGE_CURVE('',#13114,#13117,#1301,.F.) ;
#16257=EDGE_CURVE('',#13120,#13121,#6522,.T.) ;
#16258=EDGE_CURVE('',#13120,#13122,#1302,.F.) ;
#16259=EDGE_CURVE('',#13122,#13123,#1303,.T.) ;
#16260=EDGE_CURVE('',#13124,#13123,#11086,.T.) ;
#16261=EDGE_CURVE('',#13124,#13125,#1304,.T.) ;
#16262=EDGE_CURVE('',#13125,#13121,#1305,.T.) ;
#16263=EDGE_CURVE('',#13126,#13127,#6523,.T.) ;
#16264=EDGE_CURVE('',#13128,#13127,#11087,.T.) ;
#16265=EDGE_CURVE('',#13128,#13126,#1306,.T.) ;
#16266=EDGE_CURVE('',#13129,#13130,#6524,.T.) ;
#16267=EDGE_CURVE('',#13130,#13131,#1307,.T.) ;
#16268=EDGE_CURVE('',#13127,#13131,#11088,.T.) ;
#16269=EDGE_CURVE('',#13126,#13129,#1308,.F.) ;
#16270=EDGE_CURVE('',#13132,#13133,#6525,.T.) ;
#16271=EDGE_CURVE('',#13132,#13134,#1309,.F.) ;
#16272=EDGE_CURVE('',#13134,#13135,#1310,.T.) ;
#16273=EDGE_CURVE('',#13136,#13135,#11089,.T.) ;
#16274=EDGE_CURVE('',#13136,#13137,#1311,.T.) ;
#16275=EDGE_CURVE('',#13137,#13133,#1312,.T.) ;
#16276=EDGE_CURVE('',#13138,#13139,#6526,.T.) ;
#16277=EDGE_CURVE('',#13140,#13139,#11090,.T.) ;
#16278=EDGE_CURVE('',#13140,#13138,#1313,.T.) ;
#16279=EDGE_CURVE('',#13141,#13142,#6527,.T.) ;
#16280=EDGE_CURVE('',#13142,#13143,#1314,.T.) ;
#16281=EDGE_CURVE('',#13139,#13143,#11091,.T.) ;
#16282=EDGE_CURVE('',#13138,#13141,#1315,.F.) ;
#16283=EDGE_CURVE('',#13144,#13145,#6528,.T.) ;
#16284=EDGE_CURVE('',#13144,#13146,#1316,.F.) ;
#16285=EDGE_CURVE('',#13146,#13147,#1317,.T.) ;
#16286=EDGE_CURVE('',#13148,#13147,#11092,.T.) ;
#16287=EDGE_CURVE('',#13148,#13149,#1318,.T.) ;
#16288=EDGE_CURVE('',#13149,#13145,#1319,.T.) ;
#16289=EDGE_CURVE('',#13150,#13151,#6529,.T.) ;
#16290=EDGE_CURVE('',#13151,#13152,#1320,.T.) ;
#16291=EDGE_CURVE('',#13153,#13152,#11093,.T.) ;
#16292=EDGE_CURVE('',#13150,#13153,#1321,.F.) ;
#16293=EDGE_CURVE('',#13154,#13155,#6530,.T.) ;
#16294=EDGE_CURVE('',#13155,#13156,#1322,.T.) ;
#16295=EDGE_CURVE('',#13156,#13151,#1323,.T.) ;
#16296=EDGE_CURVE('',#13154,#13150,#1324,.F.) ;
#16297=EDGE_CURVE('',#13157,#13158,#6531,.T.) ;
#16298=EDGE_CURVE('',#13159,#13157,#1325,.T.) ;
#16299=EDGE_CURVE('',#13160,#13159,#1326,.T.) ;
#16300=EDGE_CURVE('',#13161,#13160,#11094,.T.) ;
#16301=EDGE_CURVE('',#13161,#13158,#1327,.T.) ;
#16302=EDGE_CURVE('',#13162,#13163,#6532,.T.) ;
#16303=EDGE_CURVE('',#13163,#13164,#1328,.T.) ;
#16304=EDGE_CURVE('',#13165,#13164,#11095,.T.) ;
#16305=EDGE_CURVE('',#13162,#13165,#1329,.F.) ;
#16306=EDGE_CURVE('',#13166,#13167,#6533,.T.) ;
#16307=EDGE_CURVE('',#13167,#13168,#1330,.T.) ;
#16308=EDGE_CURVE('',#13168,#13163,#1331,.T.) ;
#16309=EDGE_CURVE('',#13166,#13162,#1332,.F.) ;
#16310=EDGE_CURVE('',#13169,#13170,#6534,.T.) ;
#16311=EDGE_CURVE('',#13171,#13169,#1333,.T.) ;
#16312=EDGE_CURVE('',#13172,#13171,#1334,.T.) ;
#16313=EDGE_CURVE('',#13173,#13172,#11096,.T.) ;
#16314=EDGE_CURVE('',#13173,#13174,#1335,.T.) ;
#16315=EDGE_CURVE('',#13174,#13170,#1336,.T.) ;
#16316=EDGE_CURVE('',#13175,#13176,#6535,.T.) ;
#16317=EDGE_CURVE('',#13177,#13176,#11097,.T.) ;
#16318=EDGE_CURVE('',#13177,#13175,#1337,.T.) ;
#16319=EDGE_CURVE('',#13178,#13179,#6536,.T.) ;
#16320=EDGE_CURVE('',#13179,#13180,#1338,.T.) ;
#16321=EDGE_CURVE('',#13176,#13180,#11098,.T.) ;
#16322=EDGE_CURVE('',#13175,#13178,#1339,.F.) ;
#16323=EDGE_CURVE('',#13181,#13182,#6537,.T.) ;
#16324=EDGE_CURVE('',#13181,#13183,#1340,.F.) ;
#16325=EDGE_CURVE('',#13183,#13184,#1341,.T.) ;
#16326=EDGE_CURVE('',#13185,#13184,#11099,.T.) ;
#16327=EDGE_CURVE('',#13185,#13186,#1342,.T.) ;
#16328=EDGE_CURVE('',#13186,#13182,#1343,.T.) ;
#16329=EDGE_CURVE('',#13187,#13188,#6538,.T.) ;
#16330=EDGE_CURVE('',#13189,#13188,#11100,.T.) ;
#16331=EDGE_CURVE('',#13189,#13187,#1344,.T.) ;
#16332=EDGE_CURVE('',#13190,#13191,#6539,.T.) ;
#16333=EDGE_CURVE('',#13191,#13192,#1345,.T.) ;
#16334=EDGE_CURVE('',#13188,#13192,#11101,.T.) ;
#16335=EDGE_CURVE('',#13187,#13190,#1346,.F.) ;
#16336=EDGE_CURVE('',#13193,#13194,#6540,.T.) ;
#16337=EDGE_CURVE('',#13193,#13195,#1347,.F.) ;
#16338=EDGE_CURVE('',#13195,#13196,#1348,.T.) ;
#16339=EDGE_CURVE('',#13197,#13196,#11102,.T.) ;
#16340=EDGE_CURVE('',#13197,#13198,#1349,.T.) ;
#16341=EDGE_CURVE('',#13198,#13194,#1350,.T.) ;
#16342=EDGE_CURVE('',#13199,#13200,#6541,.T.) ;
#16343=EDGE_CURVE('',#13200,#13201,#1351,.T.) ;
#16344=EDGE_CURVE('',#13202,#13201,#11103,.T.) ;
#16345=EDGE_CURVE('',#13199,#13202,#1352,.F.) ;
#16346=EDGE_CURVE('',#13203,#13204,#6542,.T.) ;
#16347=EDGE_CURVE('',#13204,#13205,#1353,.T.) ;
#16348=EDGE_CURVE('',#13205,#13200,#1354,.T.) ;
#16349=EDGE_CURVE('',#13203,#13199,#1355,.F.) ;
#16350=EDGE_CURVE('',#13206,#13207,#6543,.T.) ;
#16351=EDGE_CURVE('',#13208,#13206,#1356,.T.) ;
#16352=EDGE_CURVE('',#13209,#13208,#1357,.T.) ;
#16353=EDGE_CURVE('',#13210,#13209,#11104,.T.) ;
#16354=EDGE_CURVE('',#13210,#13207,#1358,.T.) ;
#16355=EDGE_CURVE('',#13211,#13212,#6544,.T.) ;
#16356=EDGE_CURVE('',#13212,#13213,#1359,.T.) ;
#16357=EDGE_CURVE('',#13214,#13213,#11105,.T.) ;
#16358=EDGE_CURVE('',#13211,#13214,#1360,.F.) ;
#16359=EDGE_CURVE('',#13215,#13216,#6545,.T.) ;
#16360=EDGE_CURVE('',#13216,#13217,#1361,.T.) ;
#16361=EDGE_CURVE('',#13217,#13212,#1362,.T.) ;
#16362=EDGE_CURVE('',#13215,#13211,#1363,.F.) ;
#16363=EDGE_CURVE('',#13218,#13219,#6546,.T.) ;
#16364=EDGE_CURVE('',#13220,#13218,#1364,.T.) ;
#16365=EDGE_CURVE('',#13221,#13220,#1365,.T.) ;
#16366=EDGE_CURVE('',#13222,#13221,#11106,.T.) ;
#16367=EDGE_CURVE('',#13222,#13219,#1366,.T.) ;
#16368=EDGE_CURVE('',#13223,#13224,#6547,.T.) ;
#16369=EDGE_CURVE('',#13225,#13224,#11107,.T.) ;
#16370=EDGE_CURVE('',#13225,#13223,#1367,.T.) ;
#16371=EDGE_CURVE('',#13226,#13227,#6548,.T.) ;
#16372=EDGE_CURVE('',#13227,#13228,#1368,.T.) ;
#16373=EDGE_CURVE('',#13224,#13228,#11108,.T.) ;
#16374=EDGE_CURVE('',#13223,#13226,#1369,.F.) ;
#16375=EDGE_CURVE('',#13229,#13230,#6549,.T.) ;
#16376=EDGE_CURVE('',#13229,#13231,#1370,.F.) ;
#16377=EDGE_CURVE('',#13231,#13232,#1371,.T.) ;
#16378=EDGE_CURVE('',#13233,#13232,#11109,.T.) ;
#16379=EDGE_CURVE('',#13233,#13234,#1372,.T.) ;
#16380=EDGE_CURVE('',#13234,#13230,#1373,.T.) ;
#16381=EDGE_CURVE('',#13235,#13236,#6550,.T.) ;
#16382=EDGE_CURVE('',#13237,#13236,#11110,.T.) ;
#16383=EDGE_CURVE('',#13237,#13235,#1374,.T.) ;
#16384=EDGE_CURVE('',#13238,#13239,#6551,.T.) ;
#16385=EDGE_CURVE('',#13239,#13240,#1375,.T.) ;
#16386=EDGE_CURVE('',#13236,#13240,#11111,.T.) ;
#16387=EDGE_CURVE('',#13235,#13238,#1376,.F.) ;
#16388=EDGE_CURVE('',#13241,#13242,#6552,.T.) ;
#16389=EDGE_CURVE('',#13241,#13243,#1377,.F.) ;
#16390=EDGE_CURVE('',#13243,#13244,#1378,.T.) ;
#16391=EDGE_CURVE('',#13245,#13244,#11112,.T.) ;
#16392=EDGE_CURVE('',#13245,#13246,#1379,.T.) ;
#16393=EDGE_CURVE('',#13246,#13242,#1380,.T.) ;
#16394=EDGE_CURVE('',#13242,#13239,#1381,.T.) ;
#16395=EDGE_CURVE('',#13238,#13241,#1382,.F.) ;
#16396=EDGE_CURVE('',#13230,#13227,#1383,.T.) ;
#16397=EDGE_CURVE('',#13226,#13229,#1384,.F.) ;
#16398=EDGE_CURVE('',#13219,#13216,#1385,.T.) ;
#16399=EDGE_CURVE('',#13218,#13215,#1386,.F.) ;
#16400=EDGE_CURVE('',#13207,#13204,#1387,.T.) ;
#16401=EDGE_CURVE('',#13206,#13203,#1388,.F.) ;
#16402=EDGE_CURVE('',#13194,#13191,#1389,.T.) ;
#16403=EDGE_CURVE('',#13190,#13193,#1390,.F.) ;
#16404=EDGE_CURVE('',#13182,#13179,#1391,.T.) ;
#16405=EDGE_CURVE('',#13178,#13181,#1392,.F.) ;
#16406=EDGE_CURVE('',#13170,#13247,#1393,.T.) ;
#16407=EDGE_CURVE('',#13247,#13167,#1394,.T.) ;
#16408=EDGE_CURVE('',#13169,#13166,#1395,.F.) ;
#16409=EDGE_CURVE('',#13158,#13155,#1396,.T.) ;
#16410=EDGE_CURVE('',#13157,#13154,#1397,.F.) ;
#16411=EDGE_CURVE('',#13145,#13142,#1398,.T.) ;
#16412=EDGE_CURVE('',#13141,#13144,#1399,.F.) ;
#16413=EDGE_CURVE('',#13133,#13130,#1400,.T.) ;
#16414=EDGE_CURVE('',#13129,#13132,#1401,.F.) ;
#16415=EDGE_CURVE('',#13121,#13118,#1402,.T.) ;
#16416=EDGE_CURVE('',#13117,#13120,#1403,.F.) ;
#16417=EDGE_CURVE('',#13109,#13106,#1404,.T.) ;
#16418=EDGE_CURVE('',#13105,#13108,#1405,.F.) ;
#16419=EDGE_CURVE('',#13098,#13095,#1406,.T.) ;
#16420=EDGE_CURVE('',#13097,#13094,#1407,.F.) ;
#16421=EDGE_CURVE('',#13085,#13248,#1408,.T.) ;
#16422=EDGE_CURVE('',#13248,#13082,#1409,.T.) ;
#16423=EDGE_CURVE('',#13084,#13081,#1410,.F.) ;
#16424=EDGE_CURVE('',#13071,#13067,#1411,.T.) ;
#16425=EDGE_CURVE('',#13070,#13066,#1412,.F.) ;
#16426=EDGE_CURVE('',#13058,#13055,#1413,.T.) ;
#16427=EDGE_CURVE('',#13057,#13054,#1414,.F.) ;
#16428=EDGE_CURVE('',#13249,#13250,#11113,.T.) ;
#16429=EDGE_CURVE('',#13249,#13251,#6553,.T.) ;
#16430=EDGE_CURVE('',#13251,#13252,#11114,.T.) ;
#16431=EDGE_CURVE('',#13252,#13250,#6554,.T.) ;
#16432=EDGE_CURVE('',#13253,#13254,#11115,.T.) ;
#16433=EDGE_CURVE('',#13253,#13255,#6555,.T.) ;
#16434=EDGE_CURVE('',#13256,#13255,#11116,.T.) ;
#16435=EDGE_CURVE('',#13256,#13254,#6556,.T.) ;
#16436=EDGE_CURVE('',#13257,#13258,#11117,.T.) ;
#16437=EDGE_CURVE('',#13257,#13259,#6557,.T.) ;
#16438=EDGE_CURVE('',#13260,#13259,#11118,.T.) ;
#16439=EDGE_CURVE('',#13260,#13258,#6558,.T.) ;
#16440=EDGE_CURVE('',#13261,#13262,#11119,.T.) ;
#16441=EDGE_CURVE('',#13261,#13263,#6559,.T.) ;
#16442=EDGE_CURVE('',#13264,#13263,#11120,.T.) ;
#16443=EDGE_CURVE('',#13264,#13262,#6560,.T.) ;
#16444=EDGE_CURVE('',#13265,#13266,#11121,.T.) ;
#16445=EDGE_CURVE('',#13265,#13267,#6561,.T.) ;
#16446=EDGE_CURVE('',#13268,#13267,#11122,.T.) ;
#16447=EDGE_CURVE('',#13268,#13266,#6562,.T.) ;
#16448=EDGE_CURVE('',#13269,#13250,#6563,.T.) ;
#16449=EDGE_CURVE('',#13270,#13269,#11123,.T.) ;
#16450=EDGE_CURVE('',#13258,#13270,#6564,.T.) ;
#16451=EDGE_CURVE('',#13271,#13260,#6565,.T.) ;
#16452=EDGE_CURVE('',#13272,#13271,#11124,.T.) ;
#16453=EDGE_CURVE('',#13273,#13272,#6566,.T.) ;
#16454=EDGE_CURVE('',#13274,#13273,#11125,.T.) ;
#16455=EDGE_CURVE('',#13263,#13274,#6567,.T.) ;
#16456=EDGE_CURVE('',#13249,#13261,#6568,.T.) ;
#16457=EDGE_CURVE('',#13275,#13276,#11126,.T.) ;
#16458=EDGE_CURVE('',#13275,#13277,#6569,.T.) ;
#16459=EDGE_CURVE('',#13278,#13277,#11127,.T.) ;
#16460=EDGE_CURVE('',#13276,#13278,#6570,.T.) ;
#16461=EDGE_CURVE('',#13279,#13280,#11128,.T.) ;
#16462=EDGE_CURVE('',#13280,#13281,#6571,.T.) ;
#16463=EDGE_CURVE('',#13282,#13281,#11129,.T.) ;
#16464=EDGE_CURVE('',#13282,#13279,#6572,.T.) ;
#16465=EDGE_CURVE('',#13257,#13254,#6573,.T.) ;
#16466=EDGE_CURVE('',#13283,#13270,#6574,.T.) ;
#16467=EDGE_CURVE('',#13283,#13284,#6575,.F.) ;
#16468=EDGE_CURVE('',#13284,#13285,#11130,.F.) ;
#16469=EDGE_CURVE('',#13285,#13286,#6576,.T.) ;
#16470=EDGE_CURVE('',#13287,#13286,#6577,.T.) ;
#16471=EDGE_CURVE('',#13287,#13288,#6578,.F.) ;
#16472=EDGE_CURVE('',#13288,#13289,#11131,.F.) ;
#16473=EDGE_CURVE('',#13289,#13290,#6579,.T.) ;
#16474=EDGE_CURVE('',#13291,#13290,#6580,.T.) ;
#16475=EDGE_CURVE('',#13292,#13291,#6581,.T.) ;
#16476=EDGE_CURVE('',#13293,#13292,#6582,.T.) ;
#16477=EDGE_CURVE('',#13253,#13293,#6583,.T.) ;
#16478=EDGE_CURVE('',#13294,#13295,#6584,.T.) ;
#16479=EDGE_CURVE('',#13296,#13295,#6585,.T.) ;
#16480=EDGE_CURVE('',#13296,#13297,#6586,.T.) ;
#16481=EDGE_CURVE('',#13298,#13297,#6587,.T.) ;
#16482=EDGE_CURVE('',#13298,#13299,#6588,.T.) ;
#16483=EDGE_CURVE('',#13300,#13299,#6589,.T.) ;
#16484=EDGE_CURVE('',#13301,#13300,#11132,.T.) ;
#16485=EDGE_CURVE('',#13302,#13301,#6590,.T.) ;
#16486=EDGE_CURVE('',#13303,#13302,#11133,.T.) ;
#16487=EDGE_CURVE('',#13304,#13303,#6591,.T.) ;
#16488=EDGE_CURVE('',#13304,#13305,#6592,.T.) ;
#16489=EDGE_CURVE('',#13306,#13305,#6593,.T.) ;
#16490=EDGE_CURVE('',#13306,#13307,#6594,.T.) ;
#16491=EDGE_CURVE('',#13294,#13307,#6595,.T.) ;
#16492=EDGE_CURVE('',#13152,#13308,#1415,.T.) ;
#16493=EDGE_CURVE('',#13308,#13189,#1416,.T.) ;
#16494=EDGE_CURVE('',#13192,#13153,#1417,.T.) ;
#16495=EDGE_CURVE('',#13164,#13309,#1418,.T.) ;
#16496=EDGE_CURVE('',#13309,#13177,#1419,.T.) ;
#16497=EDGE_CURVE('',#13180,#13165,#1420,.T.) ;
#16498=EDGE_CURVE('',#13310,#13310,#11134,.T.) ;
#16499=EDGE_CURVE('',#13311,#13312,#6596,.T.) ;
#16500=EDGE_CURVE('',#13313,#13311,#6597,.T.) ;
#16501=EDGE_CURVE('',#13314,#13313,#6598,.T.) ;
#16502=EDGE_CURVE('',#13312,#13314,#6599,.T.) ;
#16503=EDGE_CURVE('',#13315,#13316,#6600,.T.) ;
#16504=EDGE_CURVE('',#13317,#13315,#6601,.T.) ;
#16505=EDGE_CURVE('',#13318,#13317,#6602,.T.) ;
#16506=EDGE_CURVE('',#13316,#13318,#6603,.T.) ;
#16507=EDGE_CURVE('',#13319,#13320,#6604,.T.) ;
#16508=EDGE_CURVE('',#13321,#13319,#6605,.T.) ;
#16509=EDGE_CURVE('',#13322,#13321,#6606,.T.) ;
#16510=EDGE_CURVE('',#13320,#13322,#6607,.T.) ;
#16511=EDGE_CURVE('',#13323,#13323,#11135,.T.) ;
#16512=EDGE_CURVE('',#13324,#13325,#11136,.T.) ;
#16513=EDGE_CURVE('',#13324,#13326,#6608,.T.) ;
#16514=EDGE_CURVE('',#13326,#13327,#11137,.T.) ;
#16515=EDGE_CURVE('',#13327,#13325,#6609,.T.) ;
#16516=EDGE_CURVE('',#13265,#13262,#6610,.T.) ;
#16517=EDGE_CURVE('',#13328,#13266,#6611,.T.) ;
#16518=EDGE_CURVE('',#13329,#13328,#6612,.T.) ;
#16519=EDGE_CURVE('',#13325,#13329,#6613,.T.) ;
#16520=EDGE_CURVE('',#13327,#13330,#6614,.F.) ;
#16521=EDGE_CURVE('',#13330,#13331,#11138,.F.) ;
#16522=EDGE_CURVE('',#13331,#13332,#6615,.F.) ;
#16523=EDGE_CURVE('',#13333,#13332,#6616,.T.) ;
#16524=EDGE_CURVE('',#13333,#13334,#6617,.F.) ;
#16525=EDGE_CURVE('',#13334,#13335,#11139,.F.) ;
#16526=EDGE_CURVE('',#13335,#13336,#6618,.F.) ;
#16527=EDGE_CURVE('',#13337,#13336,#6619,.T.) ;
#16528=EDGE_CURVE('',#13337,#13338,#6620,.T.) ;
#16529=EDGE_CURVE('',#13338,#13339,#11140,.F.) ;
#16530=EDGE_CURVE('',#13339,#13340,#6621,.F.) ;
#16531=EDGE_CURVE('',#13341,#13340,#6622,.T.) ;
#16532=EDGE_CURVE('',#13341,#13342,#6623,.T.) ;
#16533=EDGE_CURVE('',#13342,#13343,#11141,.F.) ;
#16534=EDGE_CURVE('',#13343,#13251,#6624,.F.) ;
#16535=EDGE_CURVE('',#13344,#13344,#11142,.T.) ;
#16536=EDGE_CURVE('',#13345,#13346,#6625,.T.) ;
#16537=EDGE_CURVE('',#13347,#13345,#6626,.T.) ;
#16538=EDGE_CURVE('',#13348,#13347,#6627,.T.) ;
#16539=EDGE_CURVE('',#13346,#13348,#6628,.T.) ;
#16540=EDGE_CURVE('',#13349,#13350,#6629,.T.) ;
#16541=EDGE_CURVE('',#13351,#13349,#6630,.T.) ;
#16542=EDGE_CURVE('',#13352,#13351,#6631,.T.) ;
#16543=EDGE_CURVE('',#13350,#13352,#6632,.T.) ;
#16544=EDGE_CURVE('',#13353,#13354,#6633,.T.) ;
#16545=EDGE_CURVE('',#13355,#13353,#6634,.T.) ;
#16546=EDGE_CURVE('',#13356,#13355,#6635,.T.) ;
#16547=EDGE_CURVE('',#13354,#13356,#6636,.T.) ;
#16548=EDGE_CURVE('',#13357,#13358,#6637,.T.) ;
#16549=EDGE_CURVE('',#13359,#13357,#6638,.T.) ;
#16550=EDGE_CURVE('',#13360,#13359,#6639,.T.) ;
#16551=EDGE_CURVE('',#13358,#13360,#6640,.T.) ;
#16552=EDGE_CURVE('',#13361,#13361,#11143,.T.) ;
#16553=EDGE_CURVE('',#13213,#13362,#1421,.T.) ;
#16554=EDGE_CURVE('',#13362,#13225,#1422,.T.) ;
#16555=EDGE_CURVE('',#13228,#13214,#1423,.T.) ;
#16556=EDGE_CURVE('',#13201,#13363,#1424,.T.) ;
#16557=EDGE_CURVE('',#13363,#13237,#1425,.T.) ;
#16558=EDGE_CURVE('',#13240,#13202,#1426,.T.) ;
#16559=EDGE_CURVE('',#13364,#13365,#6641,.T.) ;
#16560=EDGE_CURVE('',#13366,#13365,#11144,.T.) ;
#16561=EDGE_CURVE('',#13366,#13367,#6642,.T.) ;
#16562=EDGE_CURVE('',#13368,#13367,#11145,.T.) ;
#16563=EDGE_CURVE('',#13368,#13369,#6643,.T.) ;
#16564=EDGE_CURVE('',#13370,#13369,#11146,.T.) ;
#16565=EDGE_CURVE('',#13370,#13371,#6644,.T.) ;
#16566=EDGE_CURVE('',#13364,#13371,#11147,.T.) ;
#16567=EDGE_CURVE('',#13372,#13373,#6645,.T.) ;
#16568=EDGE_CURVE('',#13374,#13373,#6646,.T.) ;
#16569=EDGE_CURVE('',#13374,#13375,#6647,.T.) ;
#16570=EDGE_CURVE('',#13376,#13375,#6648,.T.) ;
#16571=EDGE_CURVE('',#13376,#13377,#6649,.T.) ;
#16572=EDGE_CURVE('',#13378,#13377,#6650,.T.) ;
#16573=EDGE_CURVE('',#13379,#13378,#11148,.T.) ;
#16574=EDGE_CURVE('',#13380,#13379,#6651,.T.) ;
#16575=EDGE_CURVE('',#13381,#13380,#11149,.T.) ;
#16576=EDGE_CURVE('',#13372,#13381,#6652,.T.) ;
#16577=EDGE_CURVE('',#13382,#13255,#6653,.T.) ;
#16578=EDGE_CURVE('',#13383,#13382,#6654,.T.) ;
#16579=EDGE_CURVE('',#13384,#13383,#6655,.T.) ;
#16580=EDGE_CURVE('',#13384,#13385,#6656,.T.) ;
#16581=EDGE_CURVE('',#13385,#13386,#6657,.T.) ;
#16582=EDGE_CURVE('',#13386,#13387,#11150,.T.) ;
#16583=EDGE_CURVE('',#13388,#13387,#6658,.T.) ;
#16584=EDGE_CURVE('',#13389,#13388,#6659,.T.) ;
#16585=EDGE_CURVE('',#13389,#13390,#6660,.T.) ;
#16586=EDGE_CURVE('',#13390,#13391,#11151,.T.) ;
#16587=EDGE_CURVE('',#13391,#13392,#6661,.T.) ;
#16588=EDGE_CURVE('',#13392,#13271,#6662,.T.) ;
#16589=EDGE_CURVE('',#13256,#13259,#6663,.T.) ;
#16590=EDGE_CURVE('',#13393,#13393,#11152,.T.) ;
#16591=EDGE_CURVE('',#13394,#13395,#6664,.T.) ;
#16592=EDGE_CURVE('',#13396,#13394,#6665,.T.) ;
#16593=EDGE_CURVE('',#13397,#13396,#6666,.T.) ;
#16594=EDGE_CURVE('',#13395,#13397,#6667,.T.) ;
#16595=EDGE_CURVE('',#13398,#13399,#6668,.T.) ;
#16596=EDGE_CURVE('',#13400,#13398,#6669,.T.) ;
#16597=EDGE_CURVE('',#13401,#13400,#6670,.T.) ;
#16598=EDGE_CURVE('',#13399,#13401,#6671,.T.) ;
#16599=EDGE_CURVE('',#13402,#13403,#6672,.T.) ;
#16600=EDGE_CURVE('',#13404,#13402,#6673,.T.) ;
#16601=EDGE_CURVE('',#13405,#13404,#6674,.T.) ;
#16602=EDGE_CURVE('',#13403,#13405,#6675,.T.) ;
#16603=EDGE_CURVE('',#13406,#13407,#11153,.T.) ;
#16604=EDGE_CURVE('',#13408,#13407,#6676,.T.) ;
#16605=EDGE_CURVE('',#13408,#13409,#11154,.T.) ;
#16606=EDGE_CURVE('',#13410,#13409,#6677,.T.) ;
#16607=EDGE_CURVE('',#13411,#13410,#6678,.T.) ;
#16608=EDGE_CURVE('',#13406,#13411,#6679,.T.) ;
#16609=EDGE_CURVE('',#13412,#13412,#11155,.T.) ;
#16610=EDGE_CURVE('',#13196,#13161,#1427,.T.) ;
#16611=EDGE_CURVE('',#13160,#13413,#1428,.T.) ;
#16612=EDGE_CURVE('',#13413,#13197,#1429,.T.) ;
#16613=EDGE_CURVE('',#13184,#13173,#1430,.T.) ;
#16614=EDGE_CURVE('',#13172,#13414,#1431,.T.) ;
#16615=EDGE_CURVE('',#13414,#13185,#1432,.T.) ;
#16616=EDGE_CURVE('',#13415,#13274,#6680,.T.) ;
#16617=EDGE_CURVE('',#13415,#13416,#6681,.T.) ;
#16618=EDGE_CURVE('',#13416,#13417,#11156,.T.) ;
#16619=EDGE_CURVE('',#13417,#13418,#6682,.T.) ;
#16620=EDGE_CURVE('',#13418,#13419,#6683,.T.) ;
#16621=EDGE_CURVE('',#13419,#13420,#6684,.T.) ;
#16622=EDGE_CURVE('',#13420,#13421,#11157,.T.) ;
#16623=EDGE_CURVE('',#13422,#13421,#6685,.T.) ;
#16624=EDGE_CURVE('',#13423,#13422,#6686,.T.) ;
#16625=EDGE_CURVE('',#13423,#13424,#6687,.T.) ;
#16626=EDGE_CURVE('',#13424,#13425,#11158,.T.) ;
#16627=EDGE_CURVE('',#13425,#13426,#6688,.T.) ;
#16628=EDGE_CURVE('',#13427,#13426,#6689,.T.) ;
#16629=EDGE_CURVE('',#13427,#13428,#6690,.T.) ;
#16630=EDGE_CURVE('',#13428,#13429,#11159,.T.) ;
#16631=EDGE_CURVE('',#13429,#13430,#6691,.T.) ;
#16632=EDGE_CURVE('',#13431,#13430,#6692,.T.) ;
#16633=EDGE_CURVE('',#13432,#13431,#6693,.T.) ;
#16634=EDGE_CURVE('',#13433,#13432,#6694,.T.) ;
#16635=EDGE_CURVE('',#13268,#13433,#6695,.T.) ;
#16636=EDGE_CURVE('',#13264,#13267,#6696,.T.) ;
#16637=EDGE_CURVE('',#13434,#13435,#11160,.T.) ;
#16638=EDGE_CURVE('',#13436,#13434,#6697,.T.) ;
#16639=EDGE_CURVE('',#13437,#13436,#11161,.T.) ;
#16640=EDGE_CURVE('',#13438,#13437,#6698,.T.) ;
#16641=EDGE_CURVE('',#13439,#13438,#11162,.T.) ;
#16642=EDGE_CURVE('',#13440,#13439,#6699,.T.) ;
#16643=EDGE_CURVE('',#13441,#13440,#11163,.T.) ;
#16644=EDGE_CURVE('',#13435,#13441,#6700,.T.) ;
#16645=EDGE_CURVE('',#13232,#13222,#1433,.T.) ;
#16646=EDGE_CURVE('',#13221,#13442,#1434,.T.) ;
#16647=EDGE_CURVE('',#13442,#13233,#1435,.T.) ;
#16648=EDGE_CURVE('',#13244,#13210,#1436,.T.) ;
#16649=EDGE_CURVE('',#13209,#13443,#1437,.T.) ;
#16650=EDGE_CURVE('',#13443,#13245,#1438,.T.) ;
#16651=EDGE_CURVE('',#13444,#13445,#11164,.T.) ;
#16652=EDGE_CURVE('',#13446,#13445,#6701,.T.) ;
#16653=EDGE_CURVE('',#13446,#13447,#11165,.T.) ;
#16654=EDGE_CURVE('',#13448,#13447,#6702,.T.) ;
#16655=EDGE_CURVE('',#13449,#13448,#6703,.T.) ;
#16656=EDGE_CURVE('',#13444,#13449,#6704,.T.) ;
#16657=EDGE_CURVE('',#13450,#13451,#6705,.T.) ;
#16658=EDGE_CURVE('',#13452,#13450,#6706,.T.) ;
#16659=EDGE_CURVE('',#13453,#13452,#6707,.T.) ;
#16660=EDGE_CURVE('',#13451,#13453,#6708,.T.) ;
#16661=EDGE_CURVE('',#13454,#13455,#6709,.T.) ;
#16662=EDGE_CURVE('',#13456,#13454,#6710,.T.) ;
#16663=EDGE_CURVE('',#13457,#13456,#6711,.T.) ;
#16664=EDGE_CURVE('',#13455,#13457,#6712,.T.) ;
#16665=EDGE_CURVE('',#13458,#13459,#6713,.T.) ;
#16666=EDGE_CURVE('',#13460,#13458,#6714,.T.) ;
#16667=EDGE_CURVE('',#13461,#13460,#6715,.T.) ;
#16668=EDGE_CURVE('',#13459,#13461,#6716,.T.) ;
#16669=EDGE_CURVE('',#13462,#13463,#6717,.T.) ;
#16670=EDGE_CURVE('',#13464,#13462,#6718,.T.) ;
#16671=EDGE_CURVE('',#13465,#13464,#6719,.T.) ;
#16672=EDGE_CURVE('',#13463,#13465,#6720,.T.) ;
#16673=EDGE_CURVE('',#13466,#13466,#11166,.T.) ;
#16674=EDGE_CURVE('',#13467,#13467,#11167,.T.) ;
#16675=EDGE_CURVE('',#13431,#13468,#11168,.T.) ;
#16676=EDGE_CURVE('',#13469,#13468,#6721,.T.) ;
#16677=EDGE_CURVE('',#13281,#13469,#6722,.T.) ;
#16678=EDGE_CURVE('',#13281,#13324,#6723,.T.) ;
#16679=EDGE_CURVE('',#13329,#13432,#6724,.T.) ;
#16680=EDGE_CURVE('',#13470,#13279,#6725,.T.) ;
#16681=EDGE_CURVE('',#13282,#13471,#6726,.T.) ;
#16682=EDGE_CURVE('',#13471,#13472,#6727,.T.) ;
#16683=EDGE_CURVE('',#13472,#13473,#1439,.T.) ;
#16684=EDGE_CURVE('',#13474,#13473,#6728,.T.) ;
#16685=EDGE_CURVE('',#13474,#13475,#6729,.T.) ;
#16686=EDGE_CURVE('',#13475,#13470,#6730,.T.) ;
#16687=EDGE_CURVE('',#13476,#13430,#11169,.T.) ;
#16688=EDGE_CURVE('',#13468,#13476,#6731,.T.) ;
#16689=EDGE_CURVE('',#13477,#13273,#6732,.T.) ;
#16690=EDGE_CURVE('',#13415,#13477,#11170,.T.) ;
#16691=EDGE_CURVE('',#13478,#13392,#11171,.T.) ;
#16692=EDGE_CURVE('',#13478,#13272,#6733,.T.) ;
#16693=EDGE_CURVE('',#13290,#13479,#11172,.T.) ;
#16694=EDGE_CURVE('',#13480,#13479,#6734,.T.) ;
#16695=EDGE_CURVE('',#13291,#13480,#11173,.T.) ;
#16696=EDGE_CURVE('',#13433,#13328,#6735,.T.) ;
#16697=EDGE_CURVE('',#13473,#13481,#6736,.T.) ;
#16698=EDGE_CURVE('',#13481,#13482,#6737,.T.) ;
#16699=EDGE_CURVE('',#13482,#13474,#6738,.T.) ;
#16700=EDGE_CURVE('',#13483,#13475,#6739,.T.) ;
#16701=EDGE_CURVE('',#13483,#13482,#6740,.T.) ;
#16702=EDGE_CURVE('',#13472,#13484,#6741,.T.) ;
#16703=EDGE_CURVE('',#13481,#13484,#1440,.T.) ;
#16704=EDGE_CURVE('',#13470,#13485,#6742,.T.) ;
#16705=EDGE_CURVE('',#13485,#13483,#6743,.T.) ;
#16706=EDGE_CURVE('',#13486,#13276,#6744,.T.) ;
#16707=EDGE_CURVE('',#13486,#13280,#6745,.T.) ;
#16708=EDGE_CURVE('',#13275,#13485,#6746,.T.) ;
#16709=EDGE_CURVE('',#13480,#13280,#6747,.T.) ;
#16710=EDGE_CURVE('',#13487,#13486,#6748,.T.) ;
#16711=EDGE_CURVE('',#13487,#13384,#11174,.T.) ;
#16712=EDGE_CURVE('',#13383,#13292,#6749,.T.) ;
#16713=EDGE_CURVE('',#13293,#13382,#6750,.T.) ;
#16714=EDGE_CURVE('',#13278,#13469,#6751,.T.) ;
#16715=EDGE_CURVE('',#13488,#13277,#6752,.T.) ;
#16716=EDGE_CURVE('',#13488,#13471,#6753,.T.) ;
#16717=EDGE_CURVE('',#13484,#13488,#6754,.T.) ;
#16718=EDGE_CURVE('',#13307,#13489,#11175,.T.) ;
#16719=EDGE_CURVE('',#13489,#13490,#6755,.T.) ;
#16720=EDGE_CURVE('',#13490,#13294,#11176,.T.) ;
#16721=EDGE_CURVE('',#13489,#13491,#6756,.T.) ;
#16722=EDGE_CURVE('',#13492,#13491,#6757,.T.) ;
#16723=EDGE_CURVE('',#13490,#13492,#6758,.T.) ;
#16724=EDGE_CURVE('',#13493,#13300,#11177,.T.) ;
#16725=EDGE_CURVE('',#13299,#13494,#11178,.T.) ;
#16726=EDGE_CURVE('',#13494,#13493,#6759,.T.) ;
#16727=EDGE_CURVE('',#13495,#13301,#11179,.T.) ;
#16728=EDGE_CURVE('',#13493,#13495,#11180,.T.) ;
#16729=EDGE_CURVE('',#13496,#13302,#11181,.T.) ;
#16730=EDGE_CURVE('',#13495,#13496,#6760,.T.) ;
#16731=EDGE_CURVE('',#13497,#13303,#11182,.T.) ;
#16732=EDGE_CURVE('',#13496,#13497,#11183,.T.) ;
#16733=EDGE_CURVE('',#13304,#13498,#11184,.F.) ;
#16734=EDGE_CURVE('',#13497,#13498,#6761,.T.) ;
#16735=EDGE_CURVE('',#13499,#13497,#6762,.T.) ;
#16736=EDGE_CURVE('',#13500,#13499,#6763,.T.) ;
#16737=EDGE_CURVE('',#13500,#13498,#6764,.T.) ;
#16738=EDGE_CURVE('',#13496,#13501,#6765,.T.) ;
#16739=EDGE_CURVE('',#13499,#13501,#11185,.T.) ;
#16740=EDGE_CURVE('',#13502,#13495,#6766,.T.) ;
#16741=EDGE_CURVE('',#13501,#13502,#6767,.T.) ;
#16742=EDGE_CURVE('',#13493,#13503,#6768,.T.) ;
#16743=EDGE_CURVE('',#13502,#13503,#11186,.T.) ;
#16744=EDGE_CURVE('',#13494,#13504,#6769,.T.) ;
#16745=EDGE_CURVE('',#13503,#13504,#6770,.T.) ;
#16746=EDGE_CURVE('',#13505,#13378,#11187,.T.) ;
#16747=EDGE_CURVE('',#13377,#13506,#11188,.T.) ;
#16748=EDGE_CURVE('',#13506,#13505,#6771,.T.) ;
#16749=EDGE_CURVE('',#13507,#13379,#11189,.T.) ;
#16750=EDGE_CURVE('',#13505,#13507,#11190,.T.) ;
#16751=EDGE_CURVE('',#13508,#13380,#11191,.T.) ;
#16752=EDGE_CURVE('',#13507,#13508,#6772,.T.) ;
#16753=EDGE_CURVE('',#13509,#13381,#11192,.T.) ;
#16754=EDGE_CURVE('',#13508,#13509,#11193,.T.) ;
#16755=EDGE_CURVE('',#13510,#13372,#11194,.T.) ;
#16756=EDGE_CURVE('',#13509,#13510,#6773,.T.) ;
#16757=EDGE_CURVE('',#13511,#13509,#6774,.T.) ;
#16758=EDGE_CURVE('',#13512,#13511,#6775,.T.) ;
#16759=EDGE_CURVE('',#13512,#13510,#6776,.T.) ;
#16760=EDGE_CURVE('',#13508,#13513,#6777,.T.) ;
#16761=EDGE_CURVE('',#13511,#13513,#11195,.T.) ;
#16762=EDGE_CURVE('',#13514,#13507,#6778,.T.) ;
#16763=EDGE_CURVE('',#13513,#13514,#6779,.T.) ;
#16764=EDGE_CURVE('',#13505,#13515,#6780,.T.) ;
#16765=EDGE_CURVE('',#13514,#13515,#11196,.T.) ;
#16766=EDGE_CURVE('',#13506,#13516,#6781,.T.) ;
#16767=EDGE_CURVE('',#13515,#13516,#6782,.T.) ;
#16768=EDGE_CURVE('',#13517,#13518,#6783,.T.) ;
#16769=EDGE_CURVE('',#13517,#13519,#6784,.T.) ;
#16770=EDGE_CURVE('',#13520,#13519,#6785,.T.) ;
#16771=EDGE_CURVE('',#13518,#13520,#6786,.T.) ;
#16772=EDGE_CURVE('',#13518,#13521,#6787,.T.) ;
#16773=EDGE_CURVE('',#13522,#13520,#6788,.T.) ;
#16774=EDGE_CURVE('',#13521,#13522,#6789,.T.) ;
#16775=EDGE_CURVE('',#13521,#13523,#6790,.T.) ;
#16776=EDGE_CURVE('',#13524,#13522,#6791,.T.) ;
#16777=EDGE_CURVE('',#13523,#13524,#6792,.T.) ;
#16778=EDGE_CURVE('',#13523,#13525,#6793,.T.) ;
#16779=EDGE_CURVE('',#13526,#13524,#6794,.T.) ;
#16780=EDGE_CURVE('',#13525,#13526,#6795,.T.) ;
#16781=EDGE_CURVE('',#13527,#13517,#6796,.T.) ;
#16782=EDGE_CURVE('',#13527,#13528,#6797,.T.) ;
#16783=EDGE_CURVE('',#13519,#13528,#6798,.T.) ;
#16784=EDGE_CURVE('',#13525,#13527,#6799,.T.) ;
#16785=EDGE_CURVE('',#13528,#13526,#6800,.T.) ;
#16786=EDGE_CURVE('',#13529,#13530,#6801,.T.) ;
#16787=EDGE_CURVE('',#13529,#13531,#6802,.T.) ;
#16788=EDGE_CURVE('',#13532,#13531,#6803,.T.) ;
#16789=EDGE_CURVE('',#13530,#13532,#6804,.T.) ;
#16790=EDGE_CURVE('',#13530,#13533,#6805,.T.) ;
#16791=EDGE_CURVE('',#13534,#13532,#6806,.T.) ;
#16792=EDGE_CURVE('',#13533,#13534,#6807,.T.) ;
#16793=EDGE_CURVE('',#13533,#13535,#6808,.T.) ;
#16794=EDGE_CURVE('',#13536,#13534,#6809,.T.) ;
#16795=EDGE_CURVE('',#13535,#13536,#6810,.T.) ;
#16796=EDGE_CURVE('',#13535,#13537,#6811,.T.) ;
#16797=EDGE_CURVE('',#13538,#13536,#6812,.T.) ;
#16798=EDGE_CURVE('',#13537,#13538,#6813,.T.) ;
#16799=EDGE_CURVE('',#13539,#13529,#6814,.T.) ;
#16800=EDGE_CURVE('',#13539,#13540,#6815,.T.) ;
#16801=EDGE_CURVE('',#13531,#13540,#6816,.T.) ;
#16802=EDGE_CURVE('',#13537,#13539,#6817,.T.) ;
#16803=EDGE_CURVE('',#13540,#13538,#6818,.T.) ;
#16804=EDGE_CURVE('',#13541,#13333,#11197,.T.) ;
#16805=EDGE_CURVE('',#13332,#13542,#11198,.T.) ;
#16806=EDGE_CURVE('',#13542,#13541,#6819,.T.) ;
#16807=EDGE_CURVE('',#13543,#13287,#11199,.T.) ;
#16808=EDGE_CURVE('',#13286,#13544,#11200,.T.) ;
#16809=EDGE_CURVE('',#13544,#13543,#6820,.T.) ;
#16810=EDGE_CURVE('',#13269,#13545,#6821,.T.) ;
#16811=EDGE_CURVE('',#13545,#13283,#11201,.T.) ;
#16812=EDGE_CURVE('',#13546,#13341,#11202,.T.) ;
#16813=EDGE_CURVE('',#13340,#13547,#11203,.T.) ;
#16814=EDGE_CURVE('',#13547,#13546,#6822,.T.) ;
#16815=EDGE_CURVE('',#13336,#13548,#11204,.T.) ;
#16816=EDGE_CURVE('',#13548,#13549,#6823,.T.) ;
#16817=EDGE_CURVE('',#13549,#13337,#11205,.T.) ;
#16818=EDGE_CURVE('',#13550,#13326,#6824,.T.) ;
#16819=EDGE_CURVE('',#13551,#13550,#6825,.T.) ;
#16820=EDGE_CURVE('',#13476,#13551,#6826,.T.) ;
#16821=EDGE_CURVE('',#13330,#13429,#6827,.T.) ;
#16822=EDGE_CURVE('',#13552,#13552,#11206,.T.) ;
#16823=EDGE_CURVE('',#13552,#13412,#6828,.T.) ;
#16824=EDGE_CURVE('',#13323,#13552,#6829,.T.) ;
#16825=EDGE_CURVE('',#13553,#13553,#11207,.T.) ;
#16826=EDGE_CURVE('',#13553,#13466,#6830,.T.) ;
#16827=EDGE_CURVE('',#13553,#13361,#6831,.T.) ;
#16828=EDGE_CURVE('',#13554,#13554,#11208,.T.) ;
#16829=EDGE_CURVE('',#13554,#13393,#6832,.T.) ;
#16830=EDGE_CURVE('',#13310,#13554,#6833,.T.) ;
#16831=EDGE_CURVE('',#13512,#13555,#6834,.T.) ;
#16832=EDGE_CURVE('',#13373,#13555,#11209,.T.) ;
#16833=EDGE_CURVE('',#13556,#13516,#6835,.T.) ;
#16834=EDGE_CURVE('',#13376,#13556,#11210,.T.) ;
#16835=EDGE_CURVE('',#13557,#13557,#11211,.F.) ;
#16836=EDGE_CURVE('',#13557,#13558,#6836,.T.) ;
#16837=EDGE_CURVE('',#13558,#13559,#11212,.T.) ;
#16838=EDGE_CURVE('',#13559,#13558,#11213,.T.) ;
#16839=EDGE_CURVE('',#13559,#13560,#6837,.T.) ;
#16840=EDGE_CURVE('',#13560,#13560,#11214,.T.) ;
#16841=EDGE_CURVE('',#13561,#13562,#11215,.T.) ;
#16842=EDGE_CURVE('',#13561,#13563,#6838,.T.) ;
#16843=EDGE_CURVE('',#13564,#13563,#11216,.T.) ;
#16844=EDGE_CURVE('',#13564,#13562,#6839,.T.) ;
#16845=EDGE_CURVE('',#13565,#13566,#11217,.T.) ;
#16846=EDGE_CURVE('',#13565,#13567,#6840,.T.) ;
#16847=EDGE_CURVE('',#13568,#13567,#11218,.T.) ;
#16848=EDGE_CURVE('',#13568,#13566,#6841,.T.) ;
#16849=EDGE_CURVE('',#13569,#13570,#11219,.T.) ;
#16850=EDGE_CURVE('',#13569,#13571,#6842,.T.) ;
#16851=EDGE_CURVE('',#13572,#13571,#11220,.T.) ;
#16852=EDGE_CURVE('',#13572,#13570,#6843,.T.) ;
#16853=EDGE_CURVE('',#13573,#13574,#11221,.T.) ;
#16854=EDGE_CURVE('',#13573,#13575,#6844,.T.) ;
#16855=EDGE_CURVE('',#13576,#13575,#11222,.T.) ;
#16856=EDGE_CURVE('',#13576,#13574,#6845,.T.) ;
#16857=EDGE_CURVE('',#13577,#13551,#11223,.T.) ;
#16858=EDGE_CURVE('',#13578,#13550,#11224,.T.) ;
#16859=EDGE_CURVE('',#13578,#13577,#6846,.T.) ;
#16860=EDGE_CURVE('',#13579,#13580,#11225,.T.) ;
#16861=EDGE_CURVE('',#13580,#13581,#6847,.T.) ;
#16862=EDGE_CURVE('',#13582,#13581,#11226,.T.) ;
#16863=EDGE_CURVE('',#13582,#13579,#6848,.T.) ;
#16864=EDGE_CURVE('',#13583,#13447,#11227,.T.) ;
#16865=EDGE_CURVE('',#13446,#13584,#11228,.T.) ;
#16866=EDGE_CURVE('',#13583,#13584,#11229,.T.) ;
#16867=EDGE_CURVE('',#13448,#13375,#11230,.T.) ;
#16868=EDGE_CURVE('',#13583,#13556,#6849,.T.) ;
#16869=EDGE_CURVE('',#13334,#13425,#6850,.T.) ;
#16870=EDGE_CURVE('',#13424,#13335,#6851,.T.) ;
#16871=EDGE_CURVE('',#13420,#13339,#6852,.T.) ;
#16872=EDGE_CURVE('',#13338,#13421,#6853,.T.) ;
#16873=EDGE_CURVE('',#13416,#13343,#6854,.T.) ;
#16874=EDGE_CURVE('',#13342,#13417,#6855,.T.) ;
#16875=EDGE_CURVE('',#13428,#13331,#6856,.T.) ;
#16876=EDGE_CURVE('',#13463,#13352,#6857,.T.) ;
#16877=EDGE_CURVE('',#13350,#13465,#6858,.T.) ;
#16878=EDGE_CURVE('',#13349,#13464,#6859,.T.) ;
#16879=EDGE_CURVE('',#13351,#13462,#6860,.T.) ;
#16880=EDGE_CURVE('',#13459,#13356,#6861,.T.) ;
#16881=EDGE_CURVE('',#13354,#13461,#6862,.T.) ;
#16882=EDGE_CURVE('',#13353,#13460,#6863,.T.) ;
#16883=EDGE_CURVE('',#13355,#13458,#6864,.T.) ;
#16884=EDGE_CURVE('',#13455,#13360,#6865,.T.) ;
#16885=EDGE_CURVE('',#13358,#13457,#6866,.T.) ;
#16886=EDGE_CURVE('',#13357,#13456,#6867,.T.) ;
#16887=EDGE_CURVE('',#13359,#13454,#6868,.T.) ;
#16888=EDGE_CURVE('',#13374,#13449,#11231,.T.) ;
#16889=EDGE_CURVE('',#13345,#13452,#6869,.T.) ;
#16890=EDGE_CURVE('',#13347,#13450,#6870,.T.) ;
#16891=EDGE_CURVE('',#13451,#13348,#6871,.T.) ;
#16892=EDGE_CURVE('',#13346,#13453,#6872,.T.) ;
#16893=EDGE_CURVE('',#13581,#13541,#6873,.T.) ;
#16894=EDGE_CURVE('',#13585,#13580,#6874,.T.) ;
#16895=EDGE_CURVE('',#13585,#13426,#11232,.T.) ;
#16896=EDGE_CURVE('',#13546,#13566,#6875,.T.) ;
#16897=EDGE_CURVE('',#13586,#13568,#6876,.T.) ;
#16898=EDGE_CURVE('',#13586,#13418,#11233,.T.) ;
#16899=EDGE_CURVE('',#13419,#13587,#11234,.T.) ;
#16900=EDGE_CURVE('',#13586,#13587,#6877,.T.) ;
#16901=EDGE_CURVE('',#13588,#13585,#6878,.T.) ;
#16902=EDGE_CURVE('',#13427,#13588,#11235,.T.) ;
#16903=EDGE_CURVE('',#13562,#13549,#6879,.T.) ;
#16904=EDGE_CURVE('',#13589,#13564,#6880,.T.) ;
#16905=EDGE_CURVE('',#13589,#13422,#11236,.T.) ;
#16906=EDGE_CURVE('',#13590,#13589,#6881,.T.) ;
#16907=EDGE_CURVE('',#13423,#13590,#11237,.T.) ;
#16908=EDGE_CURVE('',#13591,#13445,#11238,.T.) ;
#16909=EDGE_CURVE('',#13591,#13584,#6882,.T.) ;
#16910=EDGE_CURVE('',#13444,#13592,#11239,.T.) ;
#16911=EDGE_CURVE('',#13591,#13592,#11240,.T.) ;
#16912=EDGE_CURVE('',#13555,#13592,#6883,.T.) ;
#16913=EDGE_CURVE('',#13561,#13547,#6884,.T.) ;
#16914=EDGE_CURVE('',#13563,#13587,#6885,.T.) ;
#16915=EDGE_CURVE('',#13565,#13252,#6886,.T.) ;
#16916=EDGE_CURVE('',#13567,#13477,#6887,.T.) ;
#16917=EDGE_CURVE('',#13579,#13590,#6888,.T.) ;
#16918=EDGE_CURVE('',#13548,#13582,#6889,.T.) ;
#16919=EDGE_CURVE('',#13577,#13588,#6890,.T.) ;
#16920=EDGE_CURVE('',#13542,#13578,#6891,.T.) ;
#16921=EDGE_CURVE('',#13593,#13594,#6892,.T.) ;
#16922=EDGE_CURVE('',#13593,#13492,#6893,.T.) ;
#16923=EDGE_CURVE('',#13595,#13492,#6894,.T.) ;
#16924=EDGE_CURVE('',#13595,#13596,#6895,.T.) ;
#16925=EDGE_CURVE('',#13504,#13596,#6896,.T.) ;
#16926=EDGE_CURVE('',#13504,#13597,#6897,.T.) ;
#16927=EDGE_CURVE('',#13598,#13597,#6898,.T.) ;
#16928=EDGE_CURVE('',#13598,#13599,#11241,.T.) ;
#16929=EDGE_CURVE('',#13600,#13599,#6899,.T.) ;
#16930=EDGE_CURVE('',#13600,#13601,#11242,.T.) ;
#16931=EDGE_CURVE('',#13602,#13601,#6900,.T.) ;
#16932=EDGE_CURVE('',#13602,#13594,#6901,.T.) ;
#16933=EDGE_CURVE('',#13603,#13603,#11243,.T.) ;
#16934=EDGE_CURVE('',#13604,#13604,#11244,.T.) ;
#16935=EDGE_CURVE('',#13605,#13605,#11245,.T.) ;
#16936=EDGE_CURVE('',#13606,#13606,#11246,.T.) ;
#16937=EDGE_CURVE('',#13607,#13595,#11247,.T.) ;
#16938=EDGE_CURVE('',#13608,#13607,#6902,.T.) ;
#16939=EDGE_CURVE('',#13596,#13608,#11248,.T.) ;
#16940=EDGE_CURVE('',#13609,#13609,#11249,.F.) ;
#16941=EDGE_CURVE('',#13609,#13610,#6903,.T.) ;
#16942=EDGE_CURVE('',#13611,#13610,#11250,.T.) ;
#16943=EDGE_CURVE('',#13610,#13611,#11251,.T.) ;
#16944=EDGE_CURVE('',#13611,#13606,#6904,.T.) ;
#16945=EDGE_CURVE('',#13612,#13612,#11252,.F.) ;
#16946=EDGE_CURVE('',#13612,#13613,#6905,.T.) ;
#16947=EDGE_CURVE('',#13614,#13613,#11253,.T.) ;
#16948=EDGE_CURVE('',#13613,#13614,#11254,.T.) ;
#16949=EDGE_CURVE('',#13614,#13605,#6906,.T.) ;
#16950=EDGE_CURVE('',#13615,#13615,#11255,.F.) ;
#16951=EDGE_CURVE('',#13615,#13616,#6907,.T.) ;
#16952=EDGE_CURVE('',#13617,#13616,#11256,.T.) ;
#16953=EDGE_CURVE('',#13616,#13617,#11257,.T.) ;
#16954=EDGE_CURVE('',#13617,#13604,#6908,.T.) ;
#16955=EDGE_CURVE('',#13618,#13618,#11258,.F.) ;
#16956=EDGE_CURVE('',#13618,#13619,#6909,.T.) ;
#16957=EDGE_CURVE('',#13620,#13619,#11259,.T.) ;
#16958=EDGE_CURVE('',#13619,#13620,#11260,.T.) ;
#16959=EDGE_CURVE('',#13620,#13603,#6910,.T.) ;
#16960=EDGE_CURVE('',#13621,#13622,#6911,.T.) ;
#16961=EDGE_CURVE('',#13594,#13622,#6912,.T.) ;
#16962=EDGE_CURVE('',#13621,#13602,#6913,.T.) ;
#16963=EDGE_CURVE('',#13295,#13593,#11261,.T.) ;
#16964=EDGE_CURVE('',#13298,#13597,#11262,.T.) ;
#16965=EDGE_CURVE('',#13390,#13285,#6914,.T.) ;
#16966=EDGE_CURVE('',#13389,#13623,#11263,.T.) ;
#16967=EDGE_CURVE('',#13570,#13623,#6915,.T.) ;
#16968=EDGE_CURVE('',#13544,#13572,#6916,.T.) ;
#16969=EDGE_CURVE('',#13571,#13545,#6917,.T.) ;
#16970=EDGE_CURVE('',#13478,#13569,#6918,.T.) ;
#16971=EDGE_CURVE('',#13284,#13391,#6919,.T.) ;
#16972=EDGE_CURVE('',#13320,#13397,#6920,.T.) ;
#16973=EDGE_CURVE('',#13319,#13396,#6921,.T.) ;
#16974=EDGE_CURVE('',#13395,#13322,#6922,.T.) ;
#16975=EDGE_CURVE('',#13321,#13394,#6923,.T.) ;
#16976=EDGE_CURVE('',#13305,#13624,#6924,.T.) ;
#16977=EDGE_CURVE('',#13625,#13624,#6925,.T.) ;
#16978=EDGE_CURVE('',#13306,#13625,#6926,.T.) ;
#16979=EDGE_CURVE('',#13288,#13387,#6927,.T.) ;
#16980=EDGE_CURVE('',#13386,#13289,#6928,.T.) ;
#16981=EDGE_CURVE('',#13296,#13411,#11264,.T.) ;
#16982=EDGE_CURVE('',#13410,#13297,#11265,.T.) ;
#16983=EDGE_CURVE('',#13313,#13398,#6929,.T.) ;
#16984=EDGE_CURVE('',#13399,#13314,#6930,.T.) ;
#16985=EDGE_CURVE('',#13311,#13400,#6931,.T.) ;
#16986=EDGE_CURVE('',#13312,#13401,#6932,.T.) ;
#16987=EDGE_CURVE('',#13317,#13402,#6933,.T.) ;
#16988=EDGE_CURVE('',#13403,#13318,#6934,.T.) ;
#16989=EDGE_CURVE('',#13315,#13404,#6935,.T.) ;
#16990=EDGE_CURVE('',#13316,#13405,#6936,.T.) ;
#16991=EDGE_CURVE('',#13600,#13407,#11266,.T.) ;
#16992=EDGE_CURVE('',#13406,#13601,#11267,.T.) ;
#16993=EDGE_CURVE('',#13408,#13599,#11268,.T.) ;
#16994=EDGE_CURVE('',#13598,#13409,#11269,.T.) ;
#16995=EDGE_CURVE('',#13487,#13626,#6937,.T.) ;
#16996=EDGE_CURVE('',#13385,#13626,#11270,.T.) ;
#16997=EDGE_CURVE('',#13574,#13626,#6938,.T.) ;
#16998=EDGE_CURVE('',#13479,#13576,#6939,.T.) ;
#16999=EDGE_CURVE('',#13627,#13388,#11271,.T.) ;
#17000=EDGE_CURVE('',#13623,#13627,#6940,.T.) ;
#17001=EDGE_CURVE('',#13575,#13543,#6941,.T.) ;
#17002=EDGE_CURVE('',#13627,#13573,#6942,.T.) ;
#17003=EDGE_CURVE('',#13625,#13594,#11272,.T.) ;
#17004=EDGE_CURVE('',#13602,#13624,#11273,.T.) ;
#17005=EDGE_CURVE('',#13628,#13629,#6943,.T.) ;
#17006=EDGE_CURVE('',#13629,#13516,#6944,.T.) ;
#17007=EDGE_CURVE('',#13628,#13512,#6945,.T.) ;
#17008=EDGE_CURVE('',#13630,#13631,#11274,.T.) ;
#17009=EDGE_CURVE('',#13630,#13344,#6946,.T.) ;
#17010=EDGE_CURVE('',#13631,#13630,#11275,.T.) ;
#17011=EDGE_CURVE('',#13631,#13467,#6947,.T.) ;
#17012=EDGE_CURVE('',#13371,#13632,#6948,.T.) ;
#17013=EDGE_CURVE('',#13633,#13370,#6949,.T.) ;
#17014=EDGE_CURVE('',#13632,#13633,#6950,.T.) ;
#17015=EDGE_CURVE('',#13369,#13634,#6951,.T.) ;
#17016=EDGE_CURVE('',#13635,#13368,#6952,.T.) ;
#17017=EDGE_CURVE('',#13634,#13635,#6953,.T.) ;
#17018=EDGE_CURVE('',#13636,#13366,#6954,.T.) ;
#17019=EDGE_CURVE('',#13637,#13636,#6955,.T.) ;
#17020=EDGE_CURVE('',#13367,#13637,#6956,.T.) ;
#17021=EDGE_CURVE('',#13638,#13364,#6957,.T.) ;
#17022=EDGE_CURVE('',#13639,#13638,#6958,.T.) ;
#17023=EDGE_CURVE('',#13365,#13639,#6959,.T.) ;
#17024=EDGE_CURVE('',#13637,#13635,#11276,.F.) ;
#17025=EDGE_CURVE('',#13639,#13636,#11277,.F.) ;
#17026=EDGE_CURVE('',#13636,#13440,#11278,.T.) ;
#17027=EDGE_CURVE('',#13439,#13637,#11279,.T.) ;
#17028=EDGE_CURVE('',#13634,#13633,#11280,.F.) ;
#17029=EDGE_CURVE('',#13633,#13436,#11281,.T.) ;
#17030=EDGE_CURVE('',#13434,#13632,#11282,.T.) ;
#17031=EDGE_CURVE('',#13632,#13638,#11283,.F.) ;
#17032=EDGE_CURVE('',#13638,#13435,#11284,.T.) ;
#17033=EDGE_CURVE('',#13441,#13639,#11285,.T.) ;
#17034=EDGE_CURVE('',#13635,#13438,#11286,.T.) ;
#17035=EDGE_CURVE('',#13437,#13634,#11287,.T.) ;
#17036=EDGE_CURVE('',#13640,#13628,#11288,.T.) ;
#17037=EDGE_CURVE('',#13641,#13640,#6960,.T.) ;
#17038=EDGE_CURVE('',#13629,#13641,#11289,.T.) ;
#17039=EDGE_CURVE('',#13621,#13500,#11290,.T.) ;
#17040=EDGE_CURVE('',#13642,#13499,#11291,.T.) ;
#17041=EDGE_CURVE('',#13642,#13621,#6961,.T.) ;
#17042=EDGE_CURVE('',#13491,#13622,#11292,.T.) ;
#17043=EDGE_CURVE('',#13622,#13607,#6962,.T.) ;
#17044=EDGE_CURVE('',#13515,#13643,#11293,.T.) ;
#17045=EDGE_CURVE('',#13641,#13643,#6963,.T.) ;
#17046=EDGE_CURVE('',#13503,#13644,#11294,.T.) ;
#17047=EDGE_CURVE('',#13608,#13644,#6964,.T.) ;
#17048=EDGE_CURVE('',#13645,#13642,#11295,.T.) ;
#17049=EDGE_CURVE('',#13646,#13645,#6965,.T.) ;
#17050=EDGE_CURVE('',#13644,#13646,#11296,.T.) ;
#17051=EDGE_CURVE('',#13502,#13646,#11297,.T.) ;
#17052=EDGE_CURVE('',#13501,#13645,#11298,.T.) ;
#17053=EDGE_CURVE('',#13643,#13647,#11299,.T.) ;
#17054=EDGE_CURVE('',#13648,#13640,#6966,.T.) ;
#17055=EDGE_CURVE('',#13649,#13648,#11300,.T.) ;
#17056=EDGE_CURVE('',#13647,#13649,#6967,.T.) ;
#17057=EDGE_CURVE('',#13648,#13511,#11301,.T.) ;
#17058=EDGE_CURVE('',#13514,#13647,#11302,.T.) ;
#17059=EDGE_CURVE('',#13513,#13649,#11303,.T.) ;
#17060=EDGE_CURVE('',#13143,#13093,#1441,.T.) ;
#17061=EDGE_CURVE('',#13650,#13148,#1442,.T.) ;
#17062=EDGE_CURVE('',#13100,#13650,#1443,.T.) ;
#17063=EDGE_CURVE('',#13092,#13651,#1444,.T.) ;
#17064=EDGE_CURVE('',#13147,#13101,#1445,.T.) ;
#17065=EDGE_CURVE('',#13651,#13140,#1446,.T.) ;
#17066=EDGE_CURVE('',#13119,#13080,#1447,.T.) ;
#17067=EDGE_CURVE('',#13652,#13124,#1448,.T.) ;
#17068=EDGE_CURVE('',#13087,#13652,#1449,.T.) ;
#17069=EDGE_CURVE('',#13079,#13653,#1450,.T.) ;
#17070=EDGE_CURVE('',#13123,#13088,#1451,.T.) ;
#17071=EDGE_CURVE('',#13653,#13116,#1452,.T.) ;
#17072=EDGE_CURVE('',#13107,#13065,#1453,.T.) ;
#17073=EDGE_CURVE('',#13654,#13112,#1454,.T.) ;
#17074=EDGE_CURVE('',#13074,#13654,#1455,.T.) ;
#17075=EDGE_CURVE('',#13064,#13655,#1456,.T.) ;
#17076=EDGE_CURVE('',#13111,#13075,#1457,.T.) ;
#17077=EDGE_CURVE('',#13655,#13104,#1458,.T.) ;
#17078=EDGE_CURVE('',#13656,#13657,#6968,.T.) ;
#17079=EDGE_CURVE('',#13657,#13658,#6969,.T.) ;
#17080=EDGE_CURVE('',#13658,#13659,#6970,.T.) ;
#17081=EDGE_CURVE('',#13659,#13660,#6971,.T.) ;
#17082=EDGE_CURVE('',#13660,#13661,#6972,.T.) ;
#17083=EDGE_CURVE('',#13661,#13656,#6973,.T.) ;
#17084=EDGE_CURVE('',#13662,#13663,#6974,.T.) ;
#17085=EDGE_CURVE('',#13663,#13664,#6975,.T.) ;
#17086=EDGE_CURVE('',#13664,#13665,#6976,.T.) ;
#17087=EDGE_CURVE('',#13665,#13666,#6977,.T.) ;
#17088=EDGE_CURVE('',#13666,#13667,#6978,.T.) ;
#17089=EDGE_CURVE('',#13667,#13662,#6979,.T.) ;
#17090=EDGE_CURVE('',#13668,#13669,#6980,.T.) ;
#17091=EDGE_CURVE('',#13669,#13670,#6981,.T.) ;
#17092=EDGE_CURVE('',#13670,#13671,#6982,.T.) ;
#17093=EDGE_CURVE('',#13671,#13672,#6983,.T.) ;
#17094=EDGE_CURVE('',#13672,#13673,#6984,.T.) ;
#17095=EDGE_CURVE('',#13673,#13668,#6985,.T.) ;
#17096=EDGE_CURVE('',#13135,#13061,#1459,.T.) ;
#17097=EDGE_CURVE('',#13060,#13674,#1460,.T.) ;
#17098=EDGE_CURVE('',#13674,#13136,#1461,.T.) ;
#17099=EDGE_CURVE('',#13131,#13053,#1462,.T.) ;
#17100=EDGE_CURVE('',#13052,#13675,#1463,.T.) ;
#17101=EDGE_CURVE('',#13675,#13128,#1464,.T.) ;
#17102=EDGE_CURVE('',#13676,#13677,#6986,.T.) ;
#17103=EDGE_CURVE('',#13676,#13668,#6987,.T.) ;
#17104=EDGE_CURVE('',#13677,#13673,#6988,.T.) ;
#17105=EDGE_CURVE('',#13677,#13678,#6989,.T.) ;
#17106=EDGE_CURVE('',#13678,#13672,#6990,.T.) ;
#17107=EDGE_CURVE('',#13679,#13676,#6991,.T.) ;
#17108=EDGE_CURVE('',#13679,#13669,#6992,.T.) ;
#17109=EDGE_CURVE('',#13680,#13679,#6993,.T.) ;
#17110=EDGE_CURVE('',#13680,#13670,#6994,.T.) ;
#17111=EDGE_CURVE('',#13681,#13680,#6995,.T.) ;
#17112=EDGE_CURVE('',#13681,#13671,#6996,.T.) ;
#17113=EDGE_CURVE('',#13678,#13681,#6997,.T.) ;
#17114=EDGE_CURVE('',#13682,#13683,#6998,.T.) ;
#17115=EDGE_CURVE('',#13682,#13656,#6999,.T.) ;
#17116=EDGE_CURVE('',#13683,#13661,#7000,.T.) ;
#17117=EDGE_CURVE('',#13683,#13684,#7001,.T.) ;
#17118=EDGE_CURVE('',#13684,#13660,#7002,.T.) ;
#17119=EDGE_CURVE('',#13685,#13682,#7003,.T.) ;
#17120=EDGE_CURVE('',#13685,#13657,#7004,.T.) ;
#17121=EDGE_CURVE('',#13686,#13685,#7005,.T.) ;
#17122=EDGE_CURVE('',#13686,#13658,#7006,.T.) ;
#17123=EDGE_CURVE('',#13687,#13686,#7007,.T.) ;
#17124=EDGE_CURVE('',#13687,#13659,#7008,.T.) ;
#17125=EDGE_CURVE('',#13684,#13687,#7009,.T.) ;
#17126=EDGE_CURVE('',#13688,#13689,#7010,.T.) ;
#17127=EDGE_CURVE('',#13689,#13690,#7011,.T.) ;
#17128=EDGE_CURVE('',#13690,#13691,#7012,.T.) ;
#17129=EDGE_CURVE('',#13691,#13692,#7013,.T.) ;
#17130=EDGE_CURVE('',#13692,#13693,#7014,.T.) ;
#17131=EDGE_CURVE('',#13693,#13688,#7015,.T.) ;
#17132=EDGE_CURVE('',#13689,#13662,#7016,.T.) ;
#17133=EDGE_CURVE('',#13690,#13667,#7017,.T.) ;
#17134=EDGE_CURVE('',#13691,#13666,#7018,.T.) ;
#17135=EDGE_CURVE('',#13688,#13663,#7019,.T.) ;
#17136=EDGE_CURVE('',#13693,#13664,#7020,.T.) ;
#17137=EDGE_CURVE('',#13692,#13665,#7021,.T.) ;
#21550=ORIENTED_EDGE('',*,*,#16181,.T.) ;
#21551=ORIENTED_EDGE('',*,*,#16182,.T.) ;
#21552=ORIENTED_EDGE('',*,*,#16183,.F.) ;
#21553=ORIENTED_EDGE('',*,*,#16184,.F.) ;
#21554=ORIENTED_EDGE('',*,*,#16185,.T.) ;
#21555=ORIENTED_EDGE('',*,*,#16186,.T.) ;
#21556=ORIENTED_EDGE('',*,*,#16187,.T.) ;
#21557=ORIENTED_EDGE('',*,*,#16181,.F.) ;
#21558=ORIENTED_EDGE('',*,*,#16188,.F.) ;
#21559=ORIENTED_EDGE('',*,*,#16189,.F.) ;
#21560=ORIENTED_EDGE('',*,*,#16190,.F.) ;
#21561=ORIENTED_EDGE('',*,*,#16191,.F.) ;
#21562=ORIENTED_EDGE('',*,*,#16192,.F.) ;
#21563=ORIENTED_EDGE('',*,*,#16193,.T.) ;
#21564=ORIENTED_EDGE('',*,*,#16194,.T.) ;
#21565=ORIENTED_EDGE('',*,*,#16195,.T.) ;
#21566=ORIENTED_EDGE('',*,*,#16196,.F.) ;
#21567=ORIENTED_EDGE('',*,*,#16197,.F.) ;
#21568=ORIENTED_EDGE('',*,*,#16198,.T.) ;
#21569=ORIENTED_EDGE('',*,*,#16199,.T.) ;
#21570=ORIENTED_EDGE('',*,*,#16200,.T.) ;
#21571=ORIENTED_EDGE('',*,*,#16194,.F.) ;
#21572=ORIENTED_EDGE('',*,*,#16201,.F.) ;
#21573=ORIENTED_EDGE('',*,*,#16202,.F.) ;
#21574=ORIENTED_EDGE('',*,*,#16203,.F.) ;
#21575=ORIENTED_EDGE('',*,*,#16204,.F.) ;
#21576=ORIENTED_EDGE('',*,*,#16205,.F.) ;
#21577=ORIENTED_EDGE('',*,*,#16206,.F.) ;
#21578=ORIENTED_EDGE('',*,*,#16207,.F.) ;
#21579=ORIENTED_EDGE('',*,*,#16208,.T.) ;
#21580=ORIENTED_EDGE('',*,*,#16209,.T.) ;
#21581=ORIENTED_EDGE('',*,*,#16210,.T.) ;
#21582=ORIENTED_EDGE('',*,*,#16211,.T.) ;
#21583=ORIENTED_EDGE('',*,*,#16212,.F.) ;
#21584=ORIENTED_EDGE('',*,*,#16213,.F.) ;
#21585=ORIENTED_EDGE('',*,*,#16214,.T.) ;
#21586=ORIENTED_EDGE('',*,*,#16215,.T.) ;
#21587=ORIENTED_EDGE('',*,*,#16216,.T.) ;
#21588=ORIENTED_EDGE('',*,*,#16210,.F.) ;
#21589=ORIENTED_EDGE('',*,*,#16217,.F.) ;
#21590=ORIENTED_EDGE('',*,*,#16218,.F.) ;
#21591=ORIENTED_EDGE('',*,*,#16219,.F.) ;
#21592=ORIENTED_EDGE('',*,*,#16220,.F.) ;
#21593=ORIENTED_EDGE('',*,*,#16221,.F.) ;
#21594=ORIENTED_EDGE('',*,*,#16222,.T.) ;
#21595=ORIENTED_EDGE('',*,*,#16223,.T.) ;
#21596=ORIENTED_EDGE('',*,*,#16224,.T.) ;
#21597=ORIENTED_EDGE('',*,*,#16225,.T.) ;
#21598=ORIENTED_EDGE('',*,*,#16226,.F.) ;
#21599=ORIENTED_EDGE('',*,*,#16227,.F.) ;
#21600=ORIENTED_EDGE('',*,*,#16228,.T.) ;
#21601=ORIENTED_EDGE('',*,*,#16229,.T.) ;
#21602=ORIENTED_EDGE('',*,*,#16230,.T.) ;
#21603=ORIENTED_EDGE('',*,*,#16224,.F.) ;
#21604=ORIENTED_EDGE('',*,*,#16231,.F.) ;
#21605=ORIENTED_EDGE('',*,*,#16232,.F.) ;
#21606=ORIENTED_EDGE('',*,*,#16233,.F.) ;
#21607=ORIENTED_EDGE('',*,*,#16234,.F.) ;
#21608=ORIENTED_EDGE('',*,*,#16235,.F.) ;
#21609=ORIENTED_EDGE('',*,*,#16236,.T.) ;
#21610=ORIENTED_EDGE('',*,*,#16237,.T.) ;
#21611=ORIENTED_EDGE('',*,*,#16238,.F.) ;
#21612=ORIENTED_EDGE('',*,*,#16239,.T.) ;
#21613=ORIENTED_EDGE('',*,*,#16240,.T.) ;
#21614=ORIENTED_EDGE('',*,*,#16241,.T.) ;
#21615=ORIENTED_EDGE('',*,*,#16242,.F.) ;
#21616=ORIENTED_EDGE('',*,*,#16237,.F.) ;
#21617=ORIENTED_EDGE('',*,*,#16243,.T.) ;
#21618=ORIENTED_EDGE('',*,*,#16244,.F.) ;
#21619=ORIENTED_EDGE('',*,*,#16245,.T.) ;
#21620=ORIENTED_EDGE('',*,*,#16246,.T.) ;
#21621=ORIENTED_EDGE('',*,*,#16247,.F.) ;
#21622=ORIENTED_EDGE('',*,*,#16248,.T.) ;
#21623=ORIENTED_EDGE('',*,*,#16249,.T.) ;
#21624=ORIENTED_EDGE('',*,*,#16250,.T.) ;
#21625=ORIENTED_EDGE('',*,*,#16251,.F.) ;
#21626=ORIENTED_EDGE('',*,*,#16252,.T.) ;
#21627=ORIENTED_EDGE('',*,*,#16253,.T.) ;
#21628=ORIENTED_EDGE('',*,*,#16254,.T.) ;
#21629=ORIENTED_EDGE('',*,*,#16255,.F.) ;
#21630=ORIENTED_EDGE('',*,*,#16250,.F.) ;
#21631=ORIENTED_EDGE('',*,*,#16256,.T.) ;
#21632=ORIENTED_EDGE('',*,*,#16257,.F.) ;
#21633=ORIENTED_EDGE('',*,*,#16258,.T.) ;
#21634=ORIENTED_EDGE('',*,*,#16259,.T.) ;
#21635=ORIENTED_EDGE('',*,*,#16260,.F.) ;
#21636=ORIENTED_EDGE('',*,*,#16261,.T.) ;
#21637=ORIENTED_EDGE('',*,*,#16262,.T.) ;
#21638=ORIENTED_EDGE('',*,*,#16263,.T.) ;
#21639=ORIENTED_EDGE('',*,*,#16264,.F.) ;
#21640=ORIENTED_EDGE('',*,*,#16265,.T.) ;
#21641=ORIENTED_EDGE('',*,*,#16266,.T.) ;
#21642=ORIENTED_EDGE('',*,*,#16267,.T.) ;
#21643=ORIENTED_EDGE('',*,*,#16268,.F.) ;
#21644=ORIENTED_EDGE('',*,*,#16263,.F.) ;
#21645=ORIENTED_EDGE('',*,*,#16269,.T.) ;
#21646=ORIENTED_EDGE('',*,*,#16270,.F.) ;
#21647=ORIENTED_EDGE('',*,*,#16271,.T.) ;
#21648=ORIENTED_EDGE('',*,*,#16272,.T.) ;
#21649=ORIENTED_EDGE('',*,*,#16273,.F.) ;
#21650=ORIENTED_EDGE('',*,*,#16274,.T.) ;
#21651=ORIENTED_EDGE('',*,*,#16275,.T.) ;
#21652=ORIENTED_EDGE('',*,*,#16276,.T.) ;
#21653=ORIENTED_EDGE('',*,*,#16277,.F.) ;
#21654=ORIENTED_EDGE('',*,*,#16278,.T.) ;
#21655=ORIENTED_EDGE('',*,*,#16279,.T.) ;
#21656=ORIENTED_EDGE('',*,*,#16280,.T.) ;
#21657=ORIENTED_EDGE('',*,*,#16281,.F.) ;
#21658=ORIENTED_EDGE('',*,*,#16276,.F.) ;
#21659=ORIENTED_EDGE('',*,*,#16282,.T.) ;
#21660=ORIENTED_EDGE('',*,*,#16283,.F.) ;
#21661=ORIENTED_EDGE('',*,*,#16284,.T.) ;
#21662=ORIENTED_EDGE('',*,*,#16285,.T.) ;
#21663=ORIENTED_EDGE('',*,*,#16286,.F.) ;
#21664=ORIENTED_EDGE('',*,*,#16287,.T.) ;
#21665=ORIENTED_EDGE('',*,*,#16288,.T.) ;
#21666=ORIENTED_EDGE('',*,*,#16289,.T.) ;
#21667=ORIENTED_EDGE('',*,*,#16290,.T.) ;
#21668=ORIENTED_EDGE('',*,*,#16291,.F.) ;
#21669=ORIENTED_EDGE('',*,*,#16292,.F.) ;
#21670=ORIENTED_EDGE('',*,*,#16293,.T.) ;
#21671=ORIENTED_EDGE('',*,*,#16294,.T.) ;
#21672=ORIENTED_EDGE('',*,*,#16295,.T.) ;
#21673=ORIENTED_EDGE('',*,*,#16289,.F.) ;
#21674=ORIENTED_EDGE('',*,*,#16296,.F.) ;
#21675=ORIENTED_EDGE('',*,*,#16297,.F.) ;
#21676=ORIENTED_EDGE('',*,*,#16298,.F.) ;
#21677=ORIENTED_EDGE('',*,*,#16299,.F.) ;
#21678=ORIENTED_EDGE('',*,*,#16300,.F.) ;
#21679=ORIENTED_EDGE('',*,*,#16301,.T.) ;
#21680=ORIENTED_EDGE('',*,*,#16302,.T.) ;
#21681=ORIENTED_EDGE('',*,*,#16303,.T.) ;
#21682=ORIENTED_EDGE('',*,*,#16304,.F.) ;
#21683=ORIENTED_EDGE('',*,*,#16305,.F.) ;
#21684=ORIENTED_EDGE('',*,*,#16306,.T.) ;
#21685=ORIENTED_EDGE('',*,*,#16307,.T.) ;
#21686=ORIENTED_EDGE('',*,*,#16308,.T.) ;
#21687=ORIENTED_EDGE('',*,*,#16302,.F.) ;
#21688=ORIENTED_EDGE('',*,*,#16309,.F.) ;
#21689=ORIENTED_EDGE('',*,*,#16310,.F.) ;
#21690=ORIENTED_EDGE('',*,*,#16311,.F.) ;
#21691=ORIENTED_EDGE('',*,*,#16312,.F.) ;
#21692=ORIENTED_EDGE('',*,*,#16313,.F.) ;
#21693=ORIENTED_EDGE('',*,*,#16314,.T.) ;
#21694=ORIENTED_EDGE('',*,*,#16315,.T.) ;
#21695=ORIENTED_EDGE('',*,*,#16316,.T.) ;
#21696=ORIENTED_EDGE('',*,*,#16317,.F.) ;
#21697=ORIENTED_EDGE('',*,*,#16318,.T.) ;
#21698=ORIENTED_EDGE('',*,*,#16319,.T.) ;
#21699=ORIENTED_EDGE('',*,*,#16320,.T.) ;
#21700=ORIENTED_EDGE('',*,*,#16321,.F.) ;
#21701=ORIENTED_EDGE('',*,*,#16316,.F.) ;
#21702=ORIENTED_EDGE('',*,*,#16322,.T.) ;
#21703=ORIENTED_EDGE('',*,*,#16323,.F.) ;
#21704=ORIENTED_EDGE('',*,*,#16324,.T.) ;
#21705=ORIENTED_EDGE('',*,*,#16325,.T.) ;
#21706=ORIENTED_EDGE('',*,*,#16326,.F.) ;
#21707=ORIENTED_EDGE('',*,*,#16327,.T.) ;
#21708=ORIENTED_EDGE('',*,*,#16328,.T.) ;
#21709=ORIENTED_EDGE('',*,*,#16329,.T.) ;
#21710=ORIENTED_EDGE('',*,*,#16330,.F.) ;
#21711=ORIENTED_EDGE('',*,*,#16331,.T.) ;
#21712=ORIENTED_EDGE('',*,*,#16332,.T.) ;
#21713=ORIENTED_EDGE('',*,*,#16333,.T.) ;
#21714=ORIENTED_EDGE('',*,*,#16334,.F.) ;
#21715=ORIENTED_EDGE('',*,*,#16329,.F.) ;
#21716=ORIENTED_EDGE('',*,*,#16335,.T.) ;
#21717=ORIENTED_EDGE('',*,*,#16336,.F.) ;
#21718=ORIENTED_EDGE('',*,*,#16337,.T.) ;
#21719=ORIENTED_EDGE('',*,*,#16338,.T.) ;
#21720=ORIENTED_EDGE('',*,*,#16339,.F.) ;
#21721=ORIENTED_EDGE('',*,*,#16340,.T.) ;
#21722=ORIENTED_EDGE('',*,*,#16341,.T.) ;
#21723=ORIENTED_EDGE('',*,*,#16342,.T.) ;
#21724=ORIENTED_EDGE('',*,*,#16343,.T.) ;
#21725=ORIENTED_EDGE('',*,*,#16344,.F.) ;
#21726=ORIENTED_EDGE('',*,*,#16345,.F.) ;
#21727=ORIENTED_EDGE('',*,*,#16346,.T.) ;
#21728=ORIENTED_EDGE('',*,*,#16347,.T.) ;
#21729=ORIENTED_EDGE('',*,*,#16348,.T.) ;
#21730=ORIENTED_EDGE('',*,*,#16342,.F.) ;
#21731=ORIENTED_EDGE('',*,*,#16349,.F.) ;
#21732=ORIENTED_EDGE('',*,*,#16350,.F.) ;
#21733=ORIENTED_EDGE('',*,*,#16351,.F.) ;
#21734=ORIENTED_EDGE('',*,*,#16352,.F.) ;
#21735=ORIENTED_EDGE('',*,*,#16353,.F.) ;
#21736=ORIENTED_EDGE('',*,*,#16354,.T.) ;
#21737=ORIENTED_EDGE('',*,*,#16355,.T.) ;
#21738=ORIENTED_EDGE('',*,*,#16356,.T.) ;
#21739=ORIENTED_EDGE('',*,*,#16357,.F.) ;
#21740=ORIENTED_EDGE('',*,*,#16358,.F.) ;
#21741=ORIENTED_EDGE('',*,*,#16359,.T.) ;
#21742=ORIENTED_EDGE('',*,*,#16360,.T.) ;
#21743=ORIENTED_EDGE('',*,*,#16361,.T.) ;
#21744=ORIENTED_EDGE('',*,*,#16355,.F.) ;
#21745=ORIENTED_EDGE('',*,*,#16362,.F.) ;
#21746=ORIENTED_EDGE('',*,*,#16363,.F.) ;
#21747=ORIENTED_EDGE('',*,*,#16364,.F.) ;
#21748=ORIENTED_EDGE('',*,*,#16365,.F.) ;
#21749=ORIENTED_EDGE('',*,*,#16366,.F.) ;
#21750=ORIENTED_EDGE('',*,*,#16367,.T.) ;
#21751=ORIENTED_EDGE('',*,*,#16368,.T.) ;
#21752=ORIENTED_EDGE('',*,*,#16369,.F.) ;
#21753=ORIENTED_EDGE('',*,*,#16370,.T.) ;
#21754=ORIENTED_EDGE('',*,*,#16371,.T.) ;
#21755=ORIENTED_EDGE('',*,*,#16372,.T.) ;
#21756=ORIENTED_EDGE('',*,*,#16373,.F.) ;
#21757=ORIENTED_EDGE('',*,*,#16368,.F.) ;
#21758=ORIENTED_EDGE('',*,*,#16374,.T.) ;
#21759=ORIENTED_EDGE('',*,*,#16375,.F.) ;
#21760=ORIENTED_EDGE('',*,*,#16376,.T.) ;
#21761=ORIENTED_EDGE('',*,*,#16377,.T.) ;
#21762=ORIENTED_EDGE('',*,*,#16378,.F.) ;
#21763=ORIENTED_EDGE('',*,*,#16379,.T.) ;
#21764=ORIENTED_EDGE('',*,*,#16380,.T.) ;
#21765=ORIENTED_EDGE('',*,*,#16381,.T.) ;
#21766=ORIENTED_EDGE('',*,*,#16382,.F.) ;
#21767=ORIENTED_EDGE('',*,*,#16383,.T.) ;
#21768=ORIENTED_EDGE('',*,*,#16384,.T.) ;
#21769=ORIENTED_EDGE('',*,*,#16385,.T.) ;
#21770=ORIENTED_EDGE('',*,*,#16386,.F.) ;
#21771=ORIENTED_EDGE('',*,*,#16381,.F.) ;
#21772=ORIENTED_EDGE('',*,*,#16387,.T.) ;
#21773=ORIENTED_EDGE('',*,*,#16388,.F.) ;
#21774=ORIENTED_EDGE('',*,*,#16389,.T.) ;
#21775=ORIENTED_EDGE('',*,*,#16390,.T.) ;
#21776=ORIENTED_EDGE('',*,*,#16391,.F.) ;
#21777=ORIENTED_EDGE('',*,*,#16392,.T.) ;
#21778=ORIENTED_EDGE('',*,*,#16393,.T.) ;
#21779=ORIENTED_EDGE('',*,*,#16388,.T.) ;
#21780=ORIENTED_EDGE('',*,*,#16394,.T.) ;
#21781=ORIENTED_EDGE('',*,*,#16384,.F.) ;
#21782=ORIENTED_EDGE('',*,*,#16395,.T.) ;
#21783=ORIENTED_EDGE('',*,*,#16375,.T.) ;
#21784=ORIENTED_EDGE('',*,*,#16396,.T.) ;
#21785=ORIENTED_EDGE('',*,*,#16371,.F.) ;
#21786=ORIENTED_EDGE('',*,*,#16397,.T.) ;
#21787=ORIENTED_EDGE('',*,*,#16363,.T.) ;
#21788=ORIENTED_EDGE('',*,*,#16398,.T.) ;
#21789=ORIENTED_EDGE('',*,*,#16359,.F.) ;
#21790=ORIENTED_EDGE('',*,*,#16399,.F.) ;
#21791=ORIENTED_EDGE('',*,*,#16350,.T.) ;
#21792=ORIENTED_EDGE('',*,*,#16400,.T.) ;
#21793=ORIENTED_EDGE('',*,*,#16346,.F.) ;
#21794=ORIENTED_EDGE('',*,*,#16401,.F.) ;
#21795=ORIENTED_EDGE('',*,*,#16336,.T.) ;
#21796=ORIENTED_EDGE('',*,*,#16402,.T.) ;
#21797=ORIENTED_EDGE('',*,*,#16332,.F.) ;
#21798=ORIENTED_EDGE('',*,*,#16403,.T.) ;
#21799=ORIENTED_EDGE('',*,*,#16323,.T.) ;
#21800=ORIENTED_EDGE('',*,*,#16404,.T.) ;
#21801=ORIENTED_EDGE('',*,*,#16319,.F.) ;
#21802=ORIENTED_EDGE('',*,*,#16405,.T.) ;
#21803=ORIENTED_EDGE('',*,*,#16310,.T.) ;
#21804=ORIENTED_EDGE('',*,*,#16406,.T.) ;
#21805=ORIENTED_EDGE('',*,*,#16407,.T.) ;
#21806=ORIENTED_EDGE('',*,*,#16306,.F.) ;
#21807=ORIENTED_EDGE('',*,*,#16408,.F.) ;
#21808=ORIENTED_EDGE('',*,*,#16297,.T.) ;
#21809=ORIENTED_EDGE('',*,*,#16409,.T.) ;
#21810=ORIENTED_EDGE('',*,*,#16293,.F.) ;
#21811=ORIENTED_EDGE('',*,*,#16410,.F.) ;
#21812=ORIENTED_EDGE('',*,*,#16283,.T.) ;
#21813=ORIENTED_EDGE('',*,*,#16411,.T.) ;
#21814=ORIENTED_EDGE('',*,*,#16279,.F.) ;
#21815=ORIENTED_EDGE('',*,*,#16412,.T.) ;
#21816=ORIENTED_EDGE('',*,*,#16270,.T.) ;
#21817=ORIENTED_EDGE('',*,*,#16413,.T.) ;
#21818=ORIENTED_EDGE('',*,*,#16266,.F.) ;
#21819=ORIENTED_EDGE('',*,*,#16414,.T.) ;
#21820=ORIENTED_EDGE('',*,*,#16257,.T.) ;
#21821=ORIENTED_EDGE('',*,*,#16415,.T.) ;
#21822=ORIENTED_EDGE('',*,*,#16253,.F.) ;
#21823=ORIENTED_EDGE('',*,*,#16416,.T.) ;
#21824=ORIENTED_EDGE('',*,*,#16244,.T.) ;
#21825=ORIENTED_EDGE('',*,*,#16417,.T.) ;
#21826=ORIENTED_EDGE('',*,*,#16240,.F.) ;
#21827=ORIENTED_EDGE('',*,*,#16418,.T.) ;
#21828=ORIENTED_EDGE('',*,*,#16232,.T.) ;
#21829=ORIENTED_EDGE('',*,*,#16419,.T.) ;
#21830=ORIENTED_EDGE('',*,*,#16228,.F.) ;
#21831=ORIENTED_EDGE('',*,*,#16420,.F.) ;
#21832=ORIENTED_EDGE('',*,*,#16218,.T.) ;
#21833=ORIENTED_EDGE('',*,*,#16421,.T.) ;
#21834=ORIENTED_EDGE('',*,*,#16422,.T.) ;
#21835=ORIENTED_EDGE('',*,*,#16214,.F.) ;
#21836=ORIENTED_EDGE('',*,*,#16423,.F.) ;
#21837=ORIENTED_EDGE('',*,*,#16203,.T.) ;
#21838=ORIENTED_EDGE('',*,*,#16424,.T.) ;
#21839=ORIENTED_EDGE('',*,*,#16198,.F.) ;
#21840=ORIENTED_EDGE('',*,*,#16425,.F.) ;
#21841=ORIENTED_EDGE('',*,*,#16189,.T.) ;
#21842=ORIENTED_EDGE('',*,*,#16426,.T.) ;
#21843=ORIENTED_EDGE('',*,*,#16185,.F.) ;
#21844=ORIENTED_EDGE('',*,*,#16427,.F.) ;
#21845=ORIENTED_EDGE('',*,*,#16428,.F.) ;
#21846=ORIENTED_EDGE('',*,*,#16429,.T.) ;
#21847=ORIENTED_EDGE('',*,*,#16430,.T.) ;
#21848=ORIENTED_EDGE('',*,*,#16431,.T.) ;
#21849=ORIENTED_EDGE('',*,*,#16432,.F.) ;
#21850=ORIENTED_EDGE('',*,*,#16433,.T.) ;
#21851=ORIENTED_EDGE('',*,*,#16434,.F.) ;
#21852=ORIENTED_EDGE('',*,*,#16435,.T.) ;
#21853=ORIENTED_EDGE('',*,*,#16436,.F.) ;
#21854=ORIENTED_EDGE('',*,*,#16437,.T.) ;
#21855=ORIENTED_EDGE('',*,*,#16438,.F.) ;
#21856=ORIENTED_EDGE('',*,*,#16439,.T.) ;
#21857=ORIENTED_EDGE('',*,*,#16440,.F.) ;
#21858=ORIENTED_EDGE('',*,*,#16441,.T.) ;
#21859=ORIENTED_EDGE('',*,*,#16442,.F.) ;
#21860=ORIENTED_EDGE('',*,*,#16443,.T.) ;
#21861=ORIENTED_EDGE('',*,*,#16444,.F.) ;
#21862=ORIENTED_EDGE('',*,*,#16445,.T.) ;
#21863=ORIENTED_EDGE('',*,*,#16446,.F.) ;
#21864=ORIENTED_EDGE('',*,*,#16447,.T.) ;
#21865=ORIENTED_EDGE('',*,*,#16428,.T.) ;
#21866=ORIENTED_EDGE('',*,*,#16448,.F.) ;
#21867=ORIENTED_EDGE('',*,*,#16449,.F.) ;
#21868=ORIENTED_EDGE('',*,*,#16450,.F.) ;
#21869=ORIENTED_EDGE('',*,*,#16439,.F.) ;
#21870=ORIENTED_EDGE('',*,*,#16451,.F.) ;
#21871=ORIENTED_EDGE('',*,*,#16452,.F.) ;
#21872=ORIENTED_EDGE('',*,*,#16453,.F.) ;
#21873=ORIENTED_EDGE('',*,*,#16454,.F.) ;
#21874=ORIENTED_EDGE('',*,*,#16455,.F.) ;
#21875=ORIENTED_EDGE('',*,*,#16441,.F.) ;
#21876=ORIENTED_EDGE('',*,*,#16456,.F.) ;
#21877=ORIENTED_EDGE('',*,*,#16457,.F.) ;
#21878=ORIENTED_EDGE('',*,*,#16458,.T.) ;
#21879=ORIENTED_EDGE('',*,*,#16459,.F.) ;
#21880=ORIENTED_EDGE('',*,*,#16460,.F.) ;
#21881=ORIENTED_EDGE('',*,*,#16461,.T.) ;
#21882=ORIENTED_EDGE('',*,*,#16462,.T.) ;
#21883=ORIENTED_EDGE('',*,*,#16463,.F.) ;
#21884=ORIENTED_EDGE('',*,*,#16464,.T.) ;
#21885=ORIENTED_EDGE('',*,*,#16432,.T.) ;
#21886=ORIENTED_EDGE('',*,*,#16465,.F.) ;
#21887=ORIENTED_EDGE('',*,*,#16436,.T.) ;
#21888=ORIENTED_EDGE('',*,*,#16450,.T.) ;
#21889=ORIENTED_EDGE('',*,*,#16466,.F.) ;
#21890=ORIENTED_EDGE('',*,*,#16467,.T.) ;
#21891=ORIENTED_EDGE('',*,*,#16468,.T.) ;
#21892=ORIENTED_EDGE('',*,*,#16469,.T.) ;
#21893=ORIENTED_EDGE('',*,*,#16470,.F.) ;
#21894=ORIENTED_EDGE('',*,*,#16471,.T.) ;
#21895=ORIENTED_EDGE('',*,*,#16472,.T.) ;
#21896=ORIENTED_EDGE('',*,*,#16473,.T.) ;
#21897=ORIENTED_EDGE('',*,*,#16474,.F.) ;
#21898=ORIENTED_EDGE('',*,*,#16475,.F.) ;
#21899=ORIENTED_EDGE('',*,*,#16476,.F.) ;
#21900=ORIENTED_EDGE('',*,*,#16477,.F.) ;
#21901=ORIENTED_EDGE('',*,*,#16478,.T.) ;
#21902=ORIENTED_EDGE('',*,*,#16479,.F.) ;
#21903=ORIENTED_EDGE('',*,*,#16480,.T.) ;
#21904=ORIENTED_EDGE('',*,*,#16481,.F.) ;
#21905=ORIENTED_EDGE('',*,*,#16482,.T.) ;
#21906=ORIENTED_EDGE('',*,*,#16483,.F.) ;
#21907=ORIENTED_EDGE('',*,*,#16484,.F.) ;
#21908=ORIENTED_EDGE('',*,*,#16485,.F.) ;
#21909=ORIENTED_EDGE('',*,*,#16486,.F.) ;
#21910=ORIENTED_EDGE('',*,*,#16487,.F.) ;
#21911=ORIENTED_EDGE('',*,*,#16488,.T.) ;
#21912=ORIENTED_EDGE('',*,*,#16489,.F.) ;
#21913=ORIENTED_EDGE('',*,*,#16490,.T.) ;
#21914=ORIENTED_EDGE('',*,*,#16491,.F.) ;
#21915=ORIENTED_EDGE('',*,*,#16492,.T.) ;
#21916=ORIENTED_EDGE('',*,*,#16493,.T.) ;
#21917=ORIENTED_EDGE('',*,*,#16330,.T.) ;
#21918=ORIENTED_EDGE('',*,*,#16334,.T.) ;
#21919=ORIENTED_EDGE('',*,*,#16494,.T.) ;
#21920=ORIENTED_EDGE('',*,*,#16291,.T.) ;
#21921=ORIENTED_EDGE('',*,*,#16495,.T.) ;
#21922=ORIENTED_EDGE('',*,*,#16496,.T.) ;
#21923=ORIENTED_EDGE('',*,*,#16317,.T.) ;
#21924=ORIENTED_EDGE('',*,*,#16321,.T.) ;
#21925=ORIENTED_EDGE('',*,*,#16497,.T.) ;
#21926=ORIENTED_EDGE('',*,*,#16304,.T.) ;
#21927=ORIENTED_EDGE('',*,*,#16498,.F.) ;
#21928=ORIENTED_EDGE('',*,*,#16499,.F.) ;
#21929=ORIENTED_EDGE('',*,*,#16500,.F.) ;
#21930=ORIENTED_EDGE('',*,*,#16501,.F.) ;
#21931=ORIENTED_EDGE('',*,*,#16502,.F.) ;
#21932=ORIENTED_EDGE('',*,*,#16503,.F.) ;
#21933=ORIENTED_EDGE('',*,*,#16504,.F.) ;
#21934=ORIENTED_EDGE('',*,*,#16505,.F.) ;
#21935=ORIENTED_EDGE('',*,*,#16506,.F.) ;
#21936=ORIENTED_EDGE('',*,*,#16507,.F.) ;
#21937=ORIENTED_EDGE('',*,*,#16508,.F.) ;
#21938=ORIENTED_EDGE('',*,*,#16509,.F.) ;
#21939=ORIENTED_EDGE('',*,*,#16510,.F.) ;
#21940=ORIENTED_EDGE('',*,*,#16511,.F.) ;
#21941=ORIENTED_EDGE('',*,*,#16512,.F.) ;
#21942=ORIENTED_EDGE('',*,*,#16513,.T.) ;
#21943=ORIENTED_EDGE('',*,*,#16514,.T.) ;
#21944=ORIENTED_EDGE('',*,*,#16515,.T.) ;
#21945=ORIENTED_EDGE('',*,*,#16456,.T.) ;
#21946=ORIENTED_EDGE('',*,*,#16440,.T.) ;
#21947=ORIENTED_EDGE('',*,*,#16516,.F.) ;
#21948=ORIENTED_EDGE('',*,*,#16444,.T.) ;
#21949=ORIENTED_EDGE('',*,*,#16517,.F.) ;
#21950=ORIENTED_EDGE('',*,*,#16518,.F.) ;
#21951=ORIENTED_EDGE('',*,*,#16519,.F.) ;
#21952=ORIENTED_EDGE('',*,*,#16515,.F.) ;
#21953=ORIENTED_EDGE('',*,*,#16520,.T.) ;
#21954=ORIENTED_EDGE('',*,*,#16521,.T.) ;
#21955=ORIENTED_EDGE('',*,*,#16522,.T.) ;
#21956=ORIENTED_EDGE('',*,*,#16523,.F.) ;
#21957=ORIENTED_EDGE('',*,*,#16524,.T.) ;
#21958=ORIENTED_EDGE('',*,*,#16525,.T.) ;
#21959=ORIENTED_EDGE('',*,*,#16526,.T.) ;
#21960=ORIENTED_EDGE('',*,*,#16527,.F.) ;
#21961=ORIENTED_EDGE('',*,*,#16528,.T.) ;
#21962=ORIENTED_EDGE('',*,*,#16529,.T.) ;
#21963=ORIENTED_EDGE('',*,*,#16530,.T.) ;
#21964=ORIENTED_EDGE('',*,*,#16531,.F.) ;
#21965=ORIENTED_EDGE('',*,*,#16532,.T.) ;
#21966=ORIENTED_EDGE('',*,*,#16533,.T.) ;
#21967=ORIENTED_EDGE('',*,*,#16534,.T.) ;
#21968=ORIENTED_EDGE('',*,*,#16429,.F.) ;
#21969=ORIENTED_EDGE('',*,*,#16535,.F.) ;
#21970=ORIENTED_EDGE('',*,*,#16536,.F.) ;
#21971=ORIENTED_EDGE('',*,*,#16537,.F.) ;
#21972=ORIENTED_EDGE('',*,*,#16538,.F.) ;
#21973=ORIENTED_EDGE('',*,*,#16539,.F.) ;
#21974=ORIENTED_EDGE('',*,*,#16540,.F.) ;
#21975=ORIENTED_EDGE('',*,*,#16541,.F.) ;
#21976=ORIENTED_EDGE('',*,*,#16542,.F.) ;
#21977=ORIENTED_EDGE('',*,*,#16543,.F.) ;
#21978=ORIENTED_EDGE('',*,*,#16544,.F.) ;
#21979=ORIENTED_EDGE('',*,*,#16545,.F.) ;
#21980=ORIENTED_EDGE('',*,*,#16546,.F.) ;
#21981=ORIENTED_EDGE('',*,*,#16547,.F.) ;
#21982=ORIENTED_EDGE('',*,*,#16548,.F.) ;
#21983=ORIENTED_EDGE('',*,*,#16549,.F.) ;
#21984=ORIENTED_EDGE('',*,*,#16550,.F.) ;
#21985=ORIENTED_EDGE('',*,*,#16551,.F.) ;
#21986=ORIENTED_EDGE('',*,*,#16552,.F.) ;
#21987=ORIENTED_EDGE('',*,*,#16553,.T.) ;
#21988=ORIENTED_EDGE('',*,*,#16554,.T.) ;
#21989=ORIENTED_EDGE('',*,*,#16369,.T.) ;
#21990=ORIENTED_EDGE('',*,*,#16373,.T.) ;
#21991=ORIENTED_EDGE('',*,*,#16555,.T.) ;
#21992=ORIENTED_EDGE('',*,*,#16357,.T.) ;
#21993=ORIENTED_EDGE('',*,*,#16556,.T.) ;
#21994=ORIENTED_EDGE('',*,*,#16557,.T.) ;
#21995=ORIENTED_EDGE('',*,*,#16382,.T.) ;
#21996=ORIENTED_EDGE('',*,*,#16386,.T.) ;
#21997=ORIENTED_EDGE('',*,*,#16558,.T.) ;
#21998=ORIENTED_EDGE('',*,*,#16344,.T.) ;
#21999=ORIENTED_EDGE('',*,*,#16559,.T.) ;
#22000=ORIENTED_EDGE('',*,*,#16560,.F.) ;
#22001=ORIENTED_EDGE('',*,*,#16561,.T.) ;
#22002=ORIENTED_EDGE('',*,*,#16562,.F.) ;
#22003=ORIENTED_EDGE('',*,*,#16563,.T.) ;
#22004=ORIENTED_EDGE('',*,*,#16564,.F.) ;
#22005=ORIENTED_EDGE('',*,*,#16565,.T.) ;
#22006=ORIENTED_EDGE('',*,*,#16566,.F.) ;
#22007=ORIENTED_EDGE('',*,*,#16567,.T.) ;
#22008=ORIENTED_EDGE('',*,*,#16568,.F.) ;
#22009=ORIENTED_EDGE('',*,*,#16569,.T.) ;
#22010=ORIENTED_EDGE('',*,*,#16570,.F.) ;
#22011=ORIENTED_EDGE('',*,*,#16571,.T.) ;
#22012=ORIENTED_EDGE('',*,*,#16572,.F.) ;
#22013=ORIENTED_EDGE('',*,*,#16573,.F.) ;
#22014=ORIENTED_EDGE('',*,*,#16574,.F.) ;
#22015=ORIENTED_EDGE('',*,*,#16575,.F.) ;
#22016=ORIENTED_EDGE('',*,*,#16576,.F.) ;
#22017=ORIENTED_EDGE('',*,*,#16434,.T.) ;
#22018=ORIENTED_EDGE('',*,*,#16577,.F.) ;
#22019=ORIENTED_EDGE('',*,*,#16578,.F.) ;
#22020=ORIENTED_EDGE('',*,*,#16579,.F.) ;
#22021=ORIENTED_EDGE('',*,*,#16580,.T.) ;
#22022=ORIENTED_EDGE('',*,*,#16581,.T.) ;
#22023=ORIENTED_EDGE('',*,*,#16582,.T.) ;
#22024=ORIENTED_EDGE('',*,*,#16583,.F.) ;
#22025=ORIENTED_EDGE('',*,*,#16584,.F.) ;
#22026=ORIENTED_EDGE('',*,*,#16585,.T.) ;
#22027=ORIENTED_EDGE('',*,*,#16586,.T.) ;
#22028=ORIENTED_EDGE('',*,*,#16587,.T.) ;
#22029=ORIENTED_EDGE('',*,*,#16588,.T.) ;
#22030=ORIENTED_EDGE('',*,*,#16451,.T.) ;
#22031=ORIENTED_EDGE('',*,*,#16438,.T.) ;
#22032=ORIENTED_EDGE('',*,*,#16589,.F.) ;
#22033=ORIENTED_EDGE('',*,*,#16590,.F.) ;
#22034=ORIENTED_EDGE('',*,*,#16591,.F.) ;
#22035=ORIENTED_EDGE('',*,*,#16592,.F.) ;
#22036=ORIENTED_EDGE('',*,*,#16593,.F.) ;
#22037=ORIENTED_EDGE('',*,*,#16594,.F.) ;
#22038=ORIENTED_EDGE('',*,*,#16595,.F.) ;
#22039=ORIENTED_EDGE('',*,*,#16596,.F.) ;
#22040=ORIENTED_EDGE('',*,*,#16597,.F.) ;
#22041=ORIENTED_EDGE('',*,*,#16598,.F.) ;
#22042=ORIENTED_EDGE('',*,*,#16599,.F.) ;
#22043=ORIENTED_EDGE('',*,*,#16600,.F.) ;
#22044=ORIENTED_EDGE('',*,*,#16601,.F.) ;
#22045=ORIENTED_EDGE('',*,*,#16602,.F.) ;
#22046=ORIENTED_EDGE('',*,*,#16603,.T.) ;
#22047=ORIENTED_EDGE('',*,*,#16604,.F.) ;
#22048=ORIENTED_EDGE('',*,*,#16605,.T.) ;
#22049=ORIENTED_EDGE('',*,*,#16606,.F.) ;
#22050=ORIENTED_EDGE('',*,*,#16607,.F.) ;
#22051=ORIENTED_EDGE('',*,*,#16608,.F.) ;
#22052=ORIENTED_EDGE('',*,*,#16609,.F.) ;
#22053=ORIENTED_EDGE('',*,*,#16610,.T.) ;
#22054=ORIENTED_EDGE('',*,*,#16300,.T.) ;
#22055=ORIENTED_EDGE('',*,*,#16611,.T.) ;
#22056=ORIENTED_EDGE('',*,*,#16612,.T.) ;
#22057=ORIENTED_EDGE('',*,*,#16339,.T.) ;
#22058=ORIENTED_EDGE('',*,*,#16613,.T.) ;
#22059=ORIENTED_EDGE('',*,*,#16313,.T.) ;
#22060=ORIENTED_EDGE('',*,*,#16614,.T.) ;
#22061=ORIENTED_EDGE('',*,*,#16615,.T.) ;
#22062=ORIENTED_EDGE('',*,*,#16326,.T.) ;
#22063=ORIENTED_EDGE('',*,*,#16455,.T.) ;
#22064=ORIENTED_EDGE('',*,*,#16616,.F.) ;
#22065=ORIENTED_EDGE('',*,*,#16617,.T.) ;
#22066=ORIENTED_EDGE('',*,*,#16618,.T.) ;
#22067=ORIENTED_EDGE('',*,*,#16619,.T.) ;
#22068=ORIENTED_EDGE('',*,*,#16620,.T.) ;
#22069=ORIENTED_EDGE('',*,*,#16621,.T.) ;
#22070=ORIENTED_EDGE('',*,*,#16622,.T.) ;
#22071=ORIENTED_EDGE('',*,*,#16623,.F.) ;
#22072=ORIENTED_EDGE('',*,*,#16624,.F.) ;
#22073=ORIENTED_EDGE('',*,*,#16625,.T.) ;
#22074=ORIENTED_EDGE('',*,*,#16626,.T.) ;
#22075=ORIENTED_EDGE('',*,*,#16627,.T.) ;
#22076=ORIENTED_EDGE('',*,*,#16628,.F.) ;
#22077=ORIENTED_EDGE('',*,*,#16629,.T.) ;
#22078=ORIENTED_EDGE('',*,*,#16630,.T.) ;
#22079=ORIENTED_EDGE('',*,*,#16631,.T.) ;
#22080=ORIENTED_EDGE('',*,*,#16632,.F.) ;
#22081=ORIENTED_EDGE('',*,*,#16633,.F.) ;
#22082=ORIENTED_EDGE('',*,*,#16634,.F.) ;
#22083=ORIENTED_EDGE('',*,*,#16635,.F.) ;
#22084=ORIENTED_EDGE('',*,*,#16446,.T.) ;
#22085=ORIENTED_EDGE('',*,*,#16636,.F.) ;
#22086=ORIENTED_EDGE('',*,*,#16442,.T.) ;
#22087=ORIENTED_EDGE('',*,*,#16637,.F.) ;
#22088=ORIENTED_EDGE('',*,*,#16638,.F.) ;
#22089=ORIENTED_EDGE('',*,*,#16639,.F.) ;
#22090=ORIENTED_EDGE('',*,*,#16640,.F.) ;
#22091=ORIENTED_EDGE('',*,*,#16641,.F.) ;
#22092=ORIENTED_EDGE('',*,*,#16642,.F.) ;
#22093=ORIENTED_EDGE('',*,*,#16643,.F.) ;
#22094=ORIENTED_EDGE('',*,*,#16644,.F.) ;
#22095=ORIENTED_EDGE('',*,*,#16645,.T.) ;
#22096=ORIENTED_EDGE('',*,*,#16366,.T.) ;
#22097=ORIENTED_EDGE('',*,*,#16646,.T.) ;
#22098=ORIENTED_EDGE('',*,*,#16647,.T.) ;
#22099=ORIENTED_EDGE('',*,*,#16378,.T.) ;
#22100=ORIENTED_EDGE('',*,*,#16648,.T.) ;
#22101=ORIENTED_EDGE('',*,*,#16353,.T.) ;
#22102=ORIENTED_EDGE('',*,*,#16649,.T.) ;
#22103=ORIENTED_EDGE('',*,*,#16650,.T.) ;
#22104=ORIENTED_EDGE('',*,*,#16391,.T.) ;
#22105=ORIENTED_EDGE('',*,*,#16651,.T.) ;
#22106=ORIENTED_EDGE('',*,*,#16652,.F.) ;
#22107=ORIENTED_EDGE('',*,*,#16653,.T.) ;
#22108=ORIENTED_EDGE('',*,*,#16654,.F.) ;
#22109=ORIENTED_EDGE('',*,*,#16655,.F.) ;
#22110=ORIENTED_EDGE('',*,*,#16656,.F.) ;
#22111=ORIENTED_EDGE('',*,*,#16657,.F.) ;
#22112=ORIENTED_EDGE('',*,*,#16658,.F.) ;
#22113=ORIENTED_EDGE('',*,*,#16659,.F.) ;
#22114=ORIENTED_EDGE('',*,*,#16660,.F.) ;
#22115=ORIENTED_EDGE('',*,*,#16661,.F.) ;
#22116=ORIENTED_EDGE('',*,*,#16662,.F.) ;
#22117=ORIENTED_EDGE('',*,*,#16663,.F.) ;
#22118=ORIENTED_EDGE('',*,*,#16664,.F.) ;
#22119=ORIENTED_EDGE('',*,*,#16665,.F.) ;
#22120=ORIENTED_EDGE('',*,*,#16666,.F.) ;
#22121=ORIENTED_EDGE('',*,*,#16667,.F.) ;
#22122=ORIENTED_EDGE('',*,*,#16668,.F.) ;
#22123=ORIENTED_EDGE('',*,*,#16669,.F.) ;
#22124=ORIENTED_EDGE('',*,*,#16670,.F.) ;
#22125=ORIENTED_EDGE('',*,*,#16671,.F.) ;
#22126=ORIENTED_EDGE('',*,*,#16672,.F.) ;
#22127=ORIENTED_EDGE('',*,*,#16673,.F.) ;
#22128=ORIENTED_EDGE('',*,*,#16674,.F.) ;
#22129=ORIENTED_EDGE('',*,*,#16675,.T.) ;
#22130=ORIENTED_EDGE('',*,*,#16676,.F.) ;
#22131=ORIENTED_EDGE('',*,*,#16677,.F.) ;
#22132=ORIENTED_EDGE('',*,*,#16678,.T.) ;
#22133=ORIENTED_EDGE('',*,*,#16512,.T.) ;
#22134=ORIENTED_EDGE('',*,*,#16519,.T.) ;
#22135=ORIENTED_EDGE('',*,*,#16679,.T.) ;
#22136=ORIENTED_EDGE('',*,*,#16633,.T.) ;
#22137=ORIENTED_EDGE('',*,*,#16680,.T.) ;
#22138=ORIENTED_EDGE('',*,*,#16464,.F.) ;
#22139=ORIENTED_EDGE('',*,*,#16681,.T.) ;
#22140=ORIENTED_EDGE('',*,*,#16682,.T.) ;
#22141=ORIENTED_EDGE('',*,*,#16683,.T.) ;
#22142=ORIENTED_EDGE('',*,*,#16684,.F.) ;
#22143=ORIENTED_EDGE('',*,*,#16685,.T.) ;
#22144=ORIENTED_EDGE('',*,*,#16686,.T.) ;
#22145=ORIENTED_EDGE('',*,*,#16632,.T.) ;
#22146=ORIENTED_EDGE('',*,*,#16687,.F.) ;
#22147=ORIENTED_EDGE('',*,*,#16688,.F.) ;
#22148=ORIENTED_EDGE('',*,*,#16675,.F.) ;
#22149=ORIENTED_EDGE('',*,*,#16689,.F.) ;
#22150=ORIENTED_EDGE('',*,*,#16690,.F.) ;
#22151=ORIENTED_EDGE('',*,*,#16616,.T.) ;
#22152=ORIENTED_EDGE('',*,*,#16454,.T.) ;
#22153=ORIENTED_EDGE('',*,*,#16588,.F.) ;
#22154=ORIENTED_EDGE('',*,*,#16691,.F.) ;
#22155=ORIENTED_EDGE('',*,*,#16692,.T.) ;
#22156=ORIENTED_EDGE('',*,*,#16452,.T.) ;
#22157=ORIENTED_EDGE('',*,*,#16474,.T.) ;
#22158=ORIENTED_EDGE('',*,*,#16693,.T.) ;
#22159=ORIENTED_EDGE('',*,*,#16694,.F.) ;
#22160=ORIENTED_EDGE('',*,*,#16695,.F.) ;
#22161=ORIENTED_EDGE('',*,*,#16447,.F.) ;
#22162=ORIENTED_EDGE('',*,*,#16635,.T.) ;
#22163=ORIENTED_EDGE('',*,*,#16696,.T.) ;
#22164=ORIENTED_EDGE('',*,*,#16517,.T.) ;
#22165=ORIENTED_EDGE('',*,*,#16697,.T.) ;
#22166=ORIENTED_EDGE('',*,*,#16698,.T.) ;
#22167=ORIENTED_EDGE('',*,*,#16699,.T.) ;
#22168=ORIENTED_EDGE('',*,*,#16684,.T.) ;
#22169=ORIENTED_EDGE('',*,*,#16700,.T.) ;
#22170=ORIENTED_EDGE('',*,*,#16685,.F.) ;
#22171=ORIENTED_EDGE('',*,*,#16699,.F.) ;
#22172=ORIENTED_EDGE('',*,*,#16701,.F.) ;
#22173=ORIENTED_EDGE('',*,*,#16702,.T.) ;
#22174=ORIENTED_EDGE('',*,*,#16703,.F.) ;
#22175=ORIENTED_EDGE('',*,*,#16697,.F.) ;
#22176=ORIENTED_EDGE('',*,*,#16683,.F.) ;
#22177=ORIENTED_EDGE('',*,*,#16704,.F.) ;
#22178=ORIENTED_EDGE('',*,*,#16686,.F.) ;
#22179=ORIENTED_EDGE('',*,*,#16700,.F.) ;
#22180=ORIENTED_EDGE('',*,*,#16705,.F.) ;
#22181=ORIENTED_EDGE('',*,*,#16457,.T.) ;
#22182=ORIENTED_EDGE('',*,*,#16706,.F.) ;
#22183=ORIENTED_EDGE('',*,*,#16707,.T.) ;
#22184=ORIENTED_EDGE('',*,*,#16461,.F.) ;
#22185=ORIENTED_EDGE('',*,*,#16680,.F.) ;
#22186=ORIENTED_EDGE('',*,*,#16704,.T.) ;
#22187=ORIENTED_EDGE('',*,*,#16708,.F.) ;
#22188=ORIENTED_EDGE('',*,*,#16709,.T.) ;
#22189=ORIENTED_EDGE('',*,*,#16707,.F.) ;
#22190=ORIENTED_EDGE('',*,*,#16710,.F.) ;
#22191=ORIENTED_EDGE('',*,*,#16711,.T.) ;
#22192=ORIENTED_EDGE('',*,*,#16579,.T.) ;
#22193=ORIENTED_EDGE('',*,*,#16712,.T.) ;
#22194=ORIENTED_EDGE('',*,*,#16475,.T.) ;
#22195=ORIENTED_EDGE('',*,*,#16695,.T.) ;
#22196=ORIENTED_EDGE('',*,*,#16634,.T.) ;
#22197=ORIENTED_EDGE('',*,*,#16679,.F.) ;
#22198=ORIENTED_EDGE('',*,*,#16518,.T.) ;
#22199=ORIENTED_EDGE('',*,*,#16696,.F.) ;
#22200=ORIENTED_EDGE('',*,*,#16476,.T.) ;
#22201=ORIENTED_EDGE('',*,*,#16712,.F.) ;
#22202=ORIENTED_EDGE('',*,*,#16578,.T.) ;
#22203=ORIENTED_EDGE('',*,*,#16713,.F.) ;
#22204=ORIENTED_EDGE('',*,*,#16677,.T.) ;
#22205=ORIENTED_EDGE('',*,*,#16714,.F.) ;
#22206=ORIENTED_EDGE('',*,*,#16459,.T.) ;
#22207=ORIENTED_EDGE('',*,*,#16715,.F.) ;
#22208=ORIENTED_EDGE('',*,*,#16716,.T.) ;
#22209=ORIENTED_EDGE('',*,*,#16681,.F.) ;
#22210=ORIENTED_EDGE('',*,*,#16463,.T.) ;
#22211=ORIENTED_EDGE('',*,*,#16716,.F.) ;
#22212=ORIENTED_EDGE('',*,*,#16717,.F.) ;
#22213=ORIENTED_EDGE('',*,*,#16702,.F.) ;
#22214=ORIENTED_EDGE('',*,*,#16682,.F.) ;
#22215=ORIENTED_EDGE('',*,*,#16718,.T.) ;
#22216=ORIENTED_EDGE('',*,*,#16719,.T.) ;
#22217=ORIENTED_EDGE('',*,*,#16720,.T.) ;
#22218=ORIENTED_EDGE('',*,*,#16491,.T.) ;
#22219=ORIENTED_EDGE('',*,*,#16719,.F.) ;
#22220=ORIENTED_EDGE('',*,*,#16721,.T.) ;
#22221=ORIENTED_EDGE('',*,*,#16722,.F.) ;
#22222=ORIENTED_EDGE('',*,*,#16723,.F.) ;
#22223=ORIENTED_EDGE('',*,*,#16724,.T.) ;
#22224=ORIENTED_EDGE('',*,*,#16483,.T.) ;
#22225=ORIENTED_EDGE('',*,*,#16725,.T.) ;
#22226=ORIENTED_EDGE('',*,*,#16726,.T.) ;
#22227=ORIENTED_EDGE('',*,*,#16727,.T.) ;
#22228=ORIENTED_EDGE('',*,*,#16484,.T.) ;
#22229=ORIENTED_EDGE('',*,*,#16724,.F.) ;
#22230=ORIENTED_EDGE('',*,*,#16728,.T.) ;
#22231=ORIENTED_EDGE('',*,*,#16729,.T.) ;
#22232=ORIENTED_EDGE('',*,*,#16485,.T.) ;
#22233=ORIENTED_EDGE('',*,*,#16727,.F.) ;
#22234=ORIENTED_EDGE('',*,*,#16730,.T.) ;
#22235=ORIENTED_EDGE('',*,*,#16731,.T.) ;
#22236=ORIENTED_EDGE('',*,*,#16486,.T.) ;
#22237=ORIENTED_EDGE('',*,*,#16729,.F.) ;
#22238=ORIENTED_EDGE('',*,*,#16732,.T.) ;
#22239=ORIENTED_EDGE('',*,*,#16733,.F.) ;
#22240=ORIENTED_EDGE('',*,*,#16487,.T.) ;
#22241=ORIENTED_EDGE('',*,*,#16731,.F.) ;
#22242=ORIENTED_EDGE('',*,*,#16734,.T.) ;
#22243=ORIENTED_EDGE('',*,*,#16734,.F.) ;
#22244=ORIENTED_EDGE('',*,*,#16735,.F.) ;
#22245=ORIENTED_EDGE('',*,*,#16736,.F.) ;
#22246=ORIENTED_EDGE('',*,*,#16737,.T.) ;
#22247=ORIENTED_EDGE('',*,*,#16732,.F.) ;
#22248=ORIENTED_EDGE('',*,*,#16738,.T.) ;
#22249=ORIENTED_EDGE('',*,*,#16739,.F.) ;
#22250=ORIENTED_EDGE('',*,*,#16735,.T.) ;
#22251=ORIENTED_EDGE('',*,*,#16730,.F.) ;
#22252=ORIENTED_EDGE('',*,*,#16740,.F.) ;
#22253=ORIENTED_EDGE('',*,*,#16741,.F.) ;
#22254=ORIENTED_EDGE('',*,*,#16738,.F.) ;
#22255=ORIENTED_EDGE('',*,*,#16728,.F.) ;
#22256=ORIENTED_EDGE('',*,*,#16742,.T.) ;
#22257=ORIENTED_EDGE('',*,*,#16743,.F.) ;
#22258=ORIENTED_EDGE('',*,*,#16740,.T.) ;
#22259=ORIENTED_EDGE('',*,*,#16726,.F.) ;
#22260=ORIENTED_EDGE('',*,*,#16744,.T.) ;
#22261=ORIENTED_EDGE('',*,*,#16745,.F.) ;
#22262=ORIENTED_EDGE('',*,*,#16742,.F.) ;
#22263=ORIENTED_EDGE('',*,*,#16746,.T.) ;
#22264=ORIENTED_EDGE('',*,*,#16572,.T.) ;
#22265=ORIENTED_EDGE('',*,*,#16747,.T.) ;
#22266=ORIENTED_EDGE('',*,*,#16748,.T.) ;
#22267=ORIENTED_EDGE('',*,*,#16749,.T.) ;
#22268=ORIENTED_EDGE('',*,*,#16573,.T.) ;
#22269=ORIENTED_EDGE('',*,*,#16746,.F.) ;
#22270=ORIENTED_EDGE('',*,*,#16750,.T.) ;
#22271=ORIENTED_EDGE('',*,*,#16751,.T.) ;
#22272=ORIENTED_EDGE('',*,*,#16574,.T.) ;
#22273=ORIENTED_EDGE('',*,*,#16749,.F.) ;
#22274=ORIENTED_EDGE('',*,*,#16752,.T.) ;
#22275=ORIENTED_EDGE('',*,*,#16753,.T.) ;
#22276=ORIENTED_EDGE('',*,*,#16575,.T.) ;
#22277=ORIENTED_EDGE('',*,*,#16751,.F.) ;
#22278=ORIENTED_EDGE('',*,*,#16754,.T.) ;
#22279=ORIENTED_EDGE('',*,*,#16755,.T.) ;
#22280=ORIENTED_EDGE('',*,*,#16576,.T.) ;
#22281=ORIENTED_EDGE('',*,*,#16753,.F.) ;
#22282=ORIENTED_EDGE('',*,*,#16756,.T.) ;
#22283=ORIENTED_EDGE('',*,*,#16756,.F.) ;
#22284=ORIENTED_EDGE('',*,*,#16757,.F.) ;
#22285=ORIENTED_EDGE('',*,*,#16758,.F.) ;
#22286=ORIENTED_EDGE('',*,*,#16759,.T.) ;
#22287=ORIENTED_EDGE('',*,*,#16754,.F.) ;
#22288=ORIENTED_EDGE('',*,*,#16760,.T.) ;
#22289=ORIENTED_EDGE('',*,*,#16761,.F.) ;
#22290=ORIENTED_EDGE('',*,*,#16757,.T.) ;
#22291=ORIENTED_EDGE('',*,*,#16752,.F.) ;
#22292=ORIENTED_EDGE('',*,*,#16762,.F.) ;
#22293=ORIENTED_EDGE('',*,*,#16763,.F.) ;
#22294=ORIENTED_EDGE('',*,*,#16760,.F.) ;
#22295=ORIENTED_EDGE('',*,*,#16750,.F.) ;
#22296=ORIENTED_EDGE('',*,*,#16764,.T.) ;
#22297=ORIENTED_EDGE('',*,*,#16765,.F.) ;
#22298=ORIENTED_EDGE('',*,*,#16762,.T.) ;
#22299=ORIENTED_EDGE('',*,*,#16748,.F.) ;
#22300=ORIENTED_EDGE('',*,*,#16766,.T.) ;
#22301=ORIENTED_EDGE('',*,*,#16767,.F.) ;
#22302=ORIENTED_EDGE('',*,*,#16764,.F.) ;
#22303=ORIENTED_EDGE('',*,*,#16768,.F.) ;
#22304=ORIENTED_EDGE('',*,*,#16769,.T.) ;
#22305=ORIENTED_EDGE('',*,*,#16770,.F.) ;
#22306=ORIENTED_EDGE('',*,*,#16771,.F.) ;
#22307=ORIENTED_EDGE('',*,*,#16772,.F.) ;
#22308=ORIENTED_EDGE('',*,*,#16771,.T.) ;
#22309=ORIENTED_EDGE('',*,*,#16773,.F.) ;
#22310=ORIENTED_EDGE('',*,*,#16774,.F.) ;
#22311=ORIENTED_EDGE('',*,*,#16775,.F.) ;
#22312=ORIENTED_EDGE('',*,*,#16774,.T.) ;
#22313=ORIENTED_EDGE('',*,*,#16776,.F.) ;
#22314=ORIENTED_EDGE('',*,*,#16777,.F.) ;
#22315=ORIENTED_EDGE('',*,*,#16778,.F.) ;
#22316=ORIENTED_EDGE('',*,*,#16777,.T.) ;
#22317=ORIENTED_EDGE('',*,*,#16779,.F.) ;
#22318=ORIENTED_EDGE('',*,*,#16780,.F.) ;
#22319=ORIENTED_EDGE('',*,*,#16781,.F.) ;
#22320=ORIENTED_EDGE('',*,*,#16782,.T.) ;
#22321=ORIENTED_EDGE('',*,*,#16783,.F.) ;
#22322=ORIENTED_EDGE('',*,*,#16769,.F.) ;
#22323=ORIENTED_EDGE('',*,*,#16784,.F.) ;
#22324=ORIENTED_EDGE('',*,*,#16780,.T.) ;
#22325=ORIENTED_EDGE('',*,*,#16785,.F.) ;
#22326=ORIENTED_EDGE('',*,*,#16782,.F.) ;
#22327=ORIENTED_EDGE('',*,*,#16786,.F.) ;
#22328=ORIENTED_EDGE('',*,*,#16787,.T.) ;
#22329=ORIENTED_EDGE('',*,*,#16788,.F.) ;
#22330=ORIENTED_EDGE('',*,*,#16789,.F.) ;
#22331=ORIENTED_EDGE('',*,*,#16790,.F.) ;
#22332=ORIENTED_EDGE('',*,*,#16789,.T.) ;
#22333=ORIENTED_EDGE('',*,*,#16791,.F.) ;
#22334=ORIENTED_EDGE('',*,*,#16792,.F.) ;
#22335=ORIENTED_EDGE('',*,*,#16793,.F.) ;
#22336=ORIENTED_EDGE('',*,*,#16792,.T.) ;
#22337=ORIENTED_EDGE('',*,*,#16794,.F.) ;
#22338=ORIENTED_EDGE('',*,*,#16795,.F.) ;
#22339=ORIENTED_EDGE('',*,*,#16796,.F.) ;
#22340=ORIENTED_EDGE('',*,*,#16795,.T.) ;
#22341=ORIENTED_EDGE('',*,*,#16797,.F.) ;
#22342=ORIENTED_EDGE('',*,*,#16798,.F.) ;
#22343=ORIENTED_EDGE('',*,*,#16799,.F.) ;
#22344=ORIENTED_EDGE('',*,*,#16800,.T.) ;
#22345=ORIENTED_EDGE('',*,*,#16801,.F.) ;
#22346=ORIENTED_EDGE('',*,*,#16787,.F.) ;
#22347=ORIENTED_EDGE('',*,*,#16802,.F.) ;
#22348=ORIENTED_EDGE('',*,*,#16798,.T.) ;
#22349=ORIENTED_EDGE('',*,*,#16803,.F.) ;
#22350=ORIENTED_EDGE('',*,*,#16800,.F.) ;
#22351=ORIENTED_EDGE('',*,*,#16433,.F.) ;
#22352=ORIENTED_EDGE('',*,*,#16477,.T.) ;
#22353=ORIENTED_EDGE('',*,*,#16713,.T.) ;
#22354=ORIENTED_EDGE('',*,*,#16577,.T.) ;
#22355=ORIENTED_EDGE('',*,*,#16458,.F.) ;
#22356=ORIENTED_EDGE('',*,*,#16708,.T.) ;
#22357=ORIENTED_EDGE('',*,*,#16705,.T.) ;
#22358=ORIENTED_EDGE('',*,*,#16701,.T.) ;
#22359=ORIENTED_EDGE('',*,*,#16698,.F.) ;
#22360=ORIENTED_EDGE('',*,*,#16703,.T.) ;
#22361=ORIENTED_EDGE('',*,*,#16717,.T.) ;
#22362=ORIENTED_EDGE('',*,*,#16715,.T.) ;
#22363=ORIENTED_EDGE('',*,*,#16804,.T.) ;
#22364=ORIENTED_EDGE('',*,*,#16523,.T.) ;
#22365=ORIENTED_EDGE('',*,*,#16805,.T.) ;
#22366=ORIENTED_EDGE('',*,*,#16806,.T.) ;
#22367=ORIENTED_EDGE('',*,*,#16807,.T.) ;
#22368=ORIENTED_EDGE('',*,*,#16470,.T.) ;
#22369=ORIENTED_EDGE('',*,*,#16808,.T.) ;
#22370=ORIENTED_EDGE('',*,*,#16809,.T.) ;
#22371=ORIENTED_EDGE('',*,*,#16810,.T.) ;
#22372=ORIENTED_EDGE('',*,*,#16811,.T.) ;
#22373=ORIENTED_EDGE('',*,*,#16466,.T.) ;
#22374=ORIENTED_EDGE('',*,*,#16449,.T.) ;
#22375=ORIENTED_EDGE('',*,*,#16812,.T.) ;
#22376=ORIENTED_EDGE('',*,*,#16531,.T.) ;
#22377=ORIENTED_EDGE('',*,*,#16813,.T.) ;
#22378=ORIENTED_EDGE('',*,*,#16814,.T.) ;
#22379=ORIENTED_EDGE('',*,*,#16815,.T.) ;
#22380=ORIENTED_EDGE('',*,*,#16816,.T.) ;
#22381=ORIENTED_EDGE('',*,*,#16817,.T.) ;
#22382=ORIENTED_EDGE('',*,*,#16527,.T.) ;
#22383=ORIENTED_EDGE('',*,*,#16818,.F.) ;
#22384=ORIENTED_EDGE('',*,*,#16819,.F.) ;
#22385=ORIENTED_EDGE('',*,*,#16820,.F.) ;
#22386=ORIENTED_EDGE('',*,*,#16687,.T.) ;
#22387=ORIENTED_EDGE('',*,*,#16631,.F.) ;
#22388=ORIENTED_EDGE('',*,*,#16821,.F.) ;
#22389=ORIENTED_EDGE('',*,*,#16520,.F.) ;
#22390=ORIENTED_EDGE('',*,*,#16514,.F.) ;
#22391=ORIENTED_EDGE('',*,*,#16822,.T.) ;
#22392=ORIENTED_EDGE('',*,*,#16823,.T.) ;
#22393=ORIENTED_EDGE('',*,*,#16609,.T.) ;
#22394=ORIENTED_EDGE('',*,*,#16823,.F.) ;
#22395=ORIENTED_EDGE('',*,*,#16511,.T.) ;
#22396=ORIENTED_EDGE('',*,*,#16824,.T.) ;
#22397=ORIENTED_EDGE('',*,*,#16822,.F.) ;
#22398=ORIENTED_EDGE('',*,*,#16824,.F.) ;
#22399=ORIENTED_EDGE('',*,*,#16825,.T.) ;
#22400=ORIENTED_EDGE('',*,*,#16826,.T.) ;
#22401=ORIENTED_EDGE('',*,*,#16673,.T.) ;
#22402=ORIENTED_EDGE('',*,*,#16826,.F.) ;
#22403=ORIENTED_EDGE('',*,*,#16825,.F.) ;
#22404=ORIENTED_EDGE('',*,*,#16827,.T.) ;
#22405=ORIENTED_EDGE('',*,*,#16552,.T.) ;
#22406=ORIENTED_EDGE('',*,*,#16827,.F.) ;
#22407=ORIENTED_EDGE('',*,*,#16828,.T.) ;
#22408=ORIENTED_EDGE('',*,*,#16829,.T.) ;
#22409=ORIENTED_EDGE('',*,*,#16590,.T.) ;
#22410=ORIENTED_EDGE('',*,*,#16829,.F.) ;
#22411=ORIENTED_EDGE('',*,*,#16498,.T.) ;
#22412=ORIENTED_EDGE('',*,*,#16830,.T.) ;
#22413=ORIENTED_EDGE('',*,*,#16828,.F.) ;
#22414=ORIENTED_EDGE('',*,*,#16830,.F.) ;
#22415=ORIENTED_EDGE('',*,*,#16831,.T.) ;
#22416=ORIENTED_EDGE('',*,*,#16832,.F.) ;
#22417=ORIENTED_EDGE('',*,*,#16567,.F.) ;
#22418=ORIENTED_EDGE('',*,*,#16755,.F.) ;
#22419=ORIENTED_EDGE('',*,*,#16759,.F.) ;
#22420=ORIENTED_EDGE('',*,*,#16833,.T.) ;
#22421=ORIENTED_EDGE('',*,*,#16766,.F.) ;
#22422=ORIENTED_EDGE('',*,*,#16747,.F.) ;
#22423=ORIENTED_EDGE('',*,*,#16571,.F.) ;
#22424=ORIENTED_EDGE('',*,*,#16834,.T.) ;
#22425=ORIENTED_EDGE('',*,*,#16835,.F.) ;
#22426=ORIENTED_EDGE('',*,*,#16836,.T.) ;
#22427=ORIENTED_EDGE('',*,*,#16837,.T.) ;
#22428=ORIENTED_EDGE('',*,*,#16838,.T.) ;
#22429=ORIENTED_EDGE('',*,*,#16836,.F.) ;
#22430=ORIENTED_EDGE('',*,*,#16838,.F.) ;
#22431=ORIENTED_EDGE('',*,*,#16839,.T.) ;
#22432=ORIENTED_EDGE('',*,*,#16840,.T.) ;
#22433=ORIENTED_EDGE('',*,*,#16839,.F.) ;
#22434=ORIENTED_EDGE('',*,*,#16837,.F.) ;
#22435=ORIENTED_EDGE('',*,*,#16841,.F.) ;
#22436=ORIENTED_EDGE('',*,*,#16842,.T.) ;
#22437=ORIENTED_EDGE('',*,*,#16843,.F.) ;
#22438=ORIENTED_EDGE('',*,*,#16844,.T.) ;
#22439=ORIENTED_EDGE('',*,*,#16845,.F.) ;
#22440=ORIENTED_EDGE('',*,*,#16846,.T.) ;
#22441=ORIENTED_EDGE('',*,*,#16847,.F.) ;
#22442=ORIENTED_EDGE('',*,*,#16848,.T.) ;
#22443=ORIENTED_EDGE('',*,*,#16849,.F.) ;
#22444=ORIENTED_EDGE('',*,*,#16850,.T.) ;
#22445=ORIENTED_EDGE('',*,*,#16851,.F.) ;
#22446=ORIENTED_EDGE('',*,*,#16852,.T.) ;
#22447=ORIENTED_EDGE('',*,*,#16853,.F.) ;
#22448=ORIENTED_EDGE('',*,*,#16854,.T.) ;
#22449=ORIENTED_EDGE('',*,*,#16855,.F.) ;
#22450=ORIENTED_EDGE('',*,*,#16856,.T.) ;
#22451=ORIENTED_EDGE('',*,*,#16857,.T.) ;
#22452=ORIENTED_EDGE('',*,*,#16819,.T.) ;
#22453=ORIENTED_EDGE('',*,*,#16858,.F.) ;
#22454=ORIENTED_EDGE('',*,*,#16859,.T.) ;
#22455=ORIENTED_EDGE('',*,*,#16860,.T.) ;
#22456=ORIENTED_EDGE('',*,*,#16861,.T.) ;
#22457=ORIENTED_EDGE('',*,*,#16862,.F.) ;
#22458=ORIENTED_EDGE('',*,*,#16863,.T.) ;
#22459=ORIENTED_EDGE('',*,*,#16864,.T.) ;
#22460=ORIENTED_EDGE('',*,*,#16653,.F.) ;
#22461=ORIENTED_EDGE('',*,*,#16865,.T.) ;
#22462=ORIENTED_EDGE('',*,*,#16866,.F.) ;
#22463=ORIENTED_EDGE('',*,*,#16570,.T.) ;
#22464=ORIENTED_EDGE('',*,*,#16867,.F.) ;
#22465=ORIENTED_EDGE('',*,*,#16654,.T.) ;
#22466=ORIENTED_EDGE('',*,*,#16864,.F.) ;
#22467=ORIENTED_EDGE('',*,*,#16868,.T.) ;
#22468=ORIENTED_EDGE('',*,*,#16834,.F.) ;
#22469=ORIENTED_EDGE('',*,*,#16525,.F.) ;
#22470=ORIENTED_EDGE('',*,*,#16869,.T.) ;
#22471=ORIENTED_EDGE('',*,*,#16626,.F.) ;
#22472=ORIENTED_EDGE('',*,*,#16870,.T.) ;
#22473=ORIENTED_EDGE('',*,*,#16622,.F.) ;
#22474=ORIENTED_EDGE('',*,*,#16871,.T.) ;
#22475=ORIENTED_EDGE('',*,*,#16529,.F.) ;
#22476=ORIENTED_EDGE('',*,*,#16872,.T.) ;
#22477=ORIENTED_EDGE('',*,*,#16618,.F.) ;
#22478=ORIENTED_EDGE('',*,*,#16873,.T.) ;
#22479=ORIENTED_EDGE('',*,*,#16533,.F.) ;
#22480=ORIENTED_EDGE('',*,*,#16874,.T.) ;
#22481=ORIENTED_EDGE('',*,*,#16445,.F.) ;
#22482=ORIENTED_EDGE('',*,*,#16516,.T.) ;
#22483=ORIENTED_EDGE('',*,*,#16443,.F.) ;
#22484=ORIENTED_EDGE('',*,*,#16636,.T.) ;
#22485=ORIENTED_EDGE('',*,*,#16521,.F.) ;
#22486=ORIENTED_EDGE('',*,*,#16821,.T.) ;
#22487=ORIENTED_EDGE('',*,*,#16630,.F.) ;
#22488=ORIENTED_EDGE('',*,*,#16875,.T.) ;
#22489=ORIENTED_EDGE('',*,*,#16876,.F.) ;
#22490=ORIENTED_EDGE('',*,*,#16672,.T.) ;
#22491=ORIENTED_EDGE('',*,*,#16877,.F.) ;
#22492=ORIENTED_EDGE('',*,*,#16543,.T.) ;
#22493=ORIENTED_EDGE('',*,*,#16877,.T.) ;
#22494=ORIENTED_EDGE('',*,*,#16671,.T.) ;
#22495=ORIENTED_EDGE('',*,*,#16878,.F.) ;
#22496=ORIENTED_EDGE('',*,*,#16540,.T.) ;
#22497=ORIENTED_EDGE('',*,*,#16878,.T.) ;
#22498=ORIENTED_EDGE('',*,*,#16670,.T.) ;
#22499=ORIENTED_EDGE('',*,*,#16879,.F.) ;
#22500=ORIENTED_EDGE('',*,*,#16541,.T.) ;
#22501=ORIENTED_EDGE('',*,*,#16879,.T.) ;
#22502=ORIENTED_EDGE('',*,*,#16669,.T.) ;
#22503=ORIENTED_EDGE('',*,*,#16876,.T.) ;
#22504=ORIENTED_EDGE('',*,*,#16542,.T.) ;
#22505=ORIENTED_EDGE('',*,*,#16880,.F.) ;
#22506=ORIENTED_EDGE('',*,*,#16668,.T.) ;
#22507=ORIENTED_EDGE('',*,*,#16881,.F.) ;
#22508=ORIENTED_EDGE('',*,*,#16547,.T.) ;
#22509=ORIENTED_EDGE('',*,*,#16881,.T.) ;
#22510=ORIENTED_EDGE('',*,*,#16667,.T.) ;
#22511=ORIENTED_EDGE('',*,*,#16882,.F.) ;
#22512=ORIENTED_EDGE('',*,*,#16544,.T.) ;
#22513=ORIENTED_EDGE('',*,*,#16882,.T.) ;
#22514=ORIENTED_EDGE('',*,*,#16666,.T.) ;
#22515=ORIENTED_EDGE('',*,*,#16883,.F.) ;
#22516=ORIENTED_EDGE('',*,*,#16545,.T.) ;
#22517=ORIENTED_EDGE('',*,*,#16883,.T.) ;
#22518=ORIENTED_EDGE('',*,*,#16665,.T.) ;
#22519=ORIENTED_EDGE('',*,*,#16880,.T.) ;
#22520=ORIENTED_EDGE('',*,*,#16546,.T.) ;
#22521=ORIENTED_EDGE('',*,*,#16884,.F.) ;
#22522=ORIENTED_EDGE('',*,*,#16664,.T.) ;
#22523=ORIENTED_EDGE('',*,*,#16885,.F.) ;
#22524=ORIENTED_EDGE('',*,*,#16551,.T.) ;
#22525=ORIENTED_EDGE('',*,*,#16885,.T.) ;
#22526=ORIENTED_EDGE('',*,*,#16663,.T.) ;
#22527=ORIENTED_EDGE('',*,*,#16886,.F.) ;
#22528=ORIENTED_EDGE('',*,*,#16548,.T.) ;
#22529=ORIENTED_EDGE('',*,*,#16886,.T.) ;
#22530=ORIENTED_EDGE('',*,*,#16662,.T.) ;
#22531=ORIENTED_EDGE('',*,*,#16887,.F.) ;
#22532=ORIENTED_EDGE('',*,*,#16549,.T.) ;
#22533=ORIENTED_EDGE('',*,*,#16887,.T.) ;
#22534=ORIENTED_EDGE('',*,*,#16661,.T.) ;
#22535=ORIENTED_EDGE('',*,*,#16884,.T.) ;
#22536=ORIENTED_EDGE('',*,*,#16550,.T.) ;
#22537=ORIENTED_EDGE('',*,*,#16569,.F.) ;
#22538=ORIENTED_EDGE('',*,*,#16888,.T.) ;
#22539=ORIENTED_EDGE('',*,*,#16655,.T.) ;
#22540=ORIENTED_EDGE('',*,*,#16867,.T.) ;
#22541=ORIENTED_EDGE('',*,*,#16889,.T.) ;
#22542=ORIENTED_EDGE('',*,*,#16658,.T.) ;
#22543=ORIENTED_EDGE('',*,*,#16890,.F.) ;
#22544=ORIENTED_EDGE('',*,*,#16537,.T.) ;
#22545=ORIENTED_EDGE('',*,*,#16890,.T.) ;
#22546=ORIENTED_EDGE('',*,*,#16657,.T.) ;
#22547=ORIENTED_EDGE('',*,*,#16891,.T.) ;
#22548=ORIENTED_EDGE('',*,*,#16538,.T.) ;
#22549=ORIENTED_EDGE('',*,*,#16891,.F.) ;
#22550=ORIENTED_EDGE('',*,*,#16660,.T.) ;
#22551=ORIENTED_EDGE('',*,*,#16892,.F.) ;
#22552=ORIENTED_EDGE('',*,*,#16539,.T.) ;
#22553=ORIENTED_EDGE('',*,*,#16892,.T.) ;
#22554=ORIENTED_EDGE('',*,*,#16659,.T.) ;
#22555=ORIENTED_EDGE('',*,*,#16889,.F.) ;
#22556=ORIENTED_EDGE('',*,*,#16536,.T.) ;
#22557=ORIENTED_EDGE('',*,*,#16893,.F.) ;
#22558=ORIENTED_EDGE('',*,*,#16861,.F.) ;
#22559=ORIENTED_EDGE('',*,*,#16894,.F.) ;
#22560=ORIENTED_EDGE('',*,*,#16895,.T.) ;
#22561=ORIENTED_EDGE('',*,*,#16627,.F.) ;
#22562=ORIENTED_EDGE('',*,*,#16869,.F.) ;
#22563=ORIENTED_EDGE('',*,*,#16524,.F.) ;
#22564=ORIENTED_EDGE('',*,*,#16804,.F.) ;
#22565=ORIENTED_EDGE('',*,*,#16896,.T.) ;
#22566=ORIENTED_EDGE('',*,*,#16848,.F.) ;
#22567=ORIENTED_EDGE('',*,*,#16897,.F.) ;
#22568=ORIENTED_EDGE('',*,*,#16898,.T.) ;
#22569=ORIENTED_EDGE('',*,*,#16619,.F.) ;
#22570=ORIENTED_EDGE('',*,*,#16874,.F.) ;
#22571=ORIENTED_EDGE('',*,*,#16532,.F.) ;
#22572=ORIENTED_EDGE('',*,*,#16812,.F.) ;
#22573=ORIENTED_EDGE('',*,*,#16899,.F.) ;
#22574=ORIENTED_EDGE('',*,*,#16620,.F.) ;
#22575=ORIENTED_EDGE('',*,*,#16898,.F.) ;
#22576=ORIENTED_EDGE('',*,*,#16900,.T.) ;
#22577=ORIENTED_EDGE('',*,*,#16895,.F.) ;
#22578=ORIENTED_EDGE('',*,*,#16901,.F.) ;
#22579=ORIENTED_EDGE('',*,*,#16902,.F.) ;
#22580=ORIENTED_EDGE('',*,*,#16628,.T.) ;
#22581=ORIENTED_EDGE('',*,*,#16903,.F.) ;
#22582=ORIENTED_EDGE('',*,*,#16844,.F.) ;
#22583=ORIENTED_EDGE('',*,*,#16904,.F.) ;
#22584=ORIENTED_EDGE('',*,*,#16905,.T.) ;
#22585=ORIENTED_EDGE('',*,*,#16623,.T.) ;
#22586=ORIENTED_EDGE('',*,*,#16872,.F.) ;
#22587=ORIENTED_EDGE('',*,*,#16528,.F.) ;
#22588=ORIENTED_EDGE('',*,*,#16817,.F.) ;
#22589=ORIENTED_EDGE('',*,*,#16905,.F.) ;
#22590=ORIENTED_EDGE('',*,*,#16906,.F.) ;
#22591=ORIENTED_EDGE('',*,*,#16907,.F.) ;
#22592=ORIENTED_EDGE('',*,*,#16624,.T.) ;
#22593=ORIENTED_EDGE('',*,*,#16865,.F.) ;
#22594=ORIENTED_EDGE('',*,*,#16652,.T.) ;
#22595=ORIENTED_EDGE('',*,*,#16908,.F.) ;
#22596=ORIENTED_EDGE('',*,*,#16909,.T.) ;
#22597=ORIENTED_EDGE('',*,*,#16908,.T.) ;
#22598=ORIENTED_EDGE('',*,*,#16651,.F.) ;
#22599=ORIENTED_EDGE('',*,*,#16910,.T.) ;
#22600=ORIENTED_EDGE('',*,*,#16911,.F.) ;
#22601=ORIENTED_EDGE('',*,*,#16832,.T.) ;
#22602=ORIENTED_EDGE('',*,*,#16912,.T.) ;
#22603=ORIENTED_EDGE('',*,*,#16910,.F.) ;
#22604=ORIENTED_EDGE('',*,*,#16656,.T.) ;
#22605=ORIENTED_EDGE('',*,*,#16888,.F.) ;
#22606=ORIENTED_EDGE('',*,*,#16568,.T.) ;
#22607=ORIENTED_EDGE('',*,*,#16913,.T.) ;
#22608=ORIENTED_EDGE('',*,*,#16813,.F.) ;
#22609=ORIENTED_EDGE('',*,*,#16530,.F.) ;
#22610=ORIENTED_EDGE('',*,*,#16871,.F.) ;
#22611=ORIENTED_EDGE('',*,*,#16621,.F.) ;
#22612=ORIENTED_EDGE('',*,*,#16899,.T.) ;
#22613=ORIENTED_EDGE('',*,*,#16914,.F.) ;
#22614=ORIENTED_EDGE('',*,*,#16842,.F.) ;
#22615=ORIENTED_EDGE('',*,*,#16915,.T.) ;
#22616=ORIENTED_EDGE('',*,*,#16430,.F.) ;
#22617=ORIENTED_EDGE('',*,*,#16534,.F.) ;
#22618=ORIENTED_EDGE('',*,*,#16873,.F.) ;
#22619=ORIENTED_EDGE('',*,*,#16617,.F.) ;
#22620=ORIENTED_EDGE('',*,*,#16690,.T.) ;
#22621=ORIENTED_EDGE('',*,*,#16916,.F.) ;
#22622=ORIENTED_EDGE('',*,*,#16846,.F.) ;
#22623=ORIENTED_EDGE('',*,*,#16526,.F.) ;
#22624=ORIENTED_EDGE('',*,*,#16870,.F.) ;
#22625=ORIENTED_EDGE('',*,*,#16625,.F.) ;
#22626=ORIENTED_EDGE('',*,*,#16907,.T.) ;
#22627=ORIENTED_EDGE('',*,*,#16917,.F.) ;
#22628=ORIENTED_EDGE('',*,*,#16863,.F.) ;
#22629=ORIENTED_EDGE('',*,*,#16918,.F.) ;
#22630=ORIENTED_EDGE('',*,*,#16815,.F.) ;
#22631=ORIENTED_EDGE('',*,*,#16522,.F.) ;
#22632=ORIENTED_EDGE('',*,*,#16875,.F.) ;
#22633=ORIENTED_EDGE('',*,*,#16629,.F.) ;
#22634=ORIENTED_EDGE('',*,*,#16902,.T.) ;
#22635=ORIENTED_EDGE('',*,*,#16919,.F.) ;
#22636=ORIENTED_EDGE('',*,*,#16859,.F.) ;
#22637=ORIENTED_EDGE('',*,*,#16920,.F.) ;
#22638=ORIENTED_EDGE('',*,*,#16805,.F.) ;
#22639=ORIENTED_EDGE('',*,*,#16921,.F.) ;
#22640=ORIENTED_EDGE('',*,*,#16922,.T.) ;
#22641=ORIENTED_EDGE('',*,*,#16923,.F.) ;
#22642=ORIENTED_EDGE('',*,*,#16924,.T.) ;
#22643=ORIENTED_EDGE('',*,*,#16925,.F.) ;
#22644=ORIENTED_EDGE('',*,*,#16926,.T.) ;
#22645=ORIENTED_EDGE('',*,*,#16927,.F.) ;
#22646=ORIENTED_EDGE('',*,*,#16928,.T.) ;
#22647=ORIENTED_EDGE('',*,*,#16929,.F.) ;
#22648=ORIENTED_EDGE('',*,*,#16930,.T.) ;
#22649=ORIENTED_EDGE('',*,*,#16931,.F.) ;
#22650=ORIENTED_EDGE('',*,*,#16932,.T.) ;
#22651=ORIENTED_EDGE('',*,*,#16933,.F.) ;
#22652=ORIENTED_EDGE('',*,*,#16934,.F.) ;
#22653=ORIENTED_EDGE('',*,*,#16935,.F.) ;
#22654=ORIENTED_EDGE('',*,*,#16936,.F.) ;
#22655=ORIENTED_EDGE('',*,*,#16937,.F.) ;
#22656=ORIENTED_EDGE('',*,*,#16938,.F.) ;
#22657=ORIENTED_EDGE('',*,*,#16939,.F.) ;
#22658=ORIENTED_EDGE('',*,*,#16924,.F.) ;
#22659=ORIENTED_EDGE('',*,*,#16940,.F.) ;
#22660=ORIENTED_EDGE('',*,*,#16941,.T.) ;
#22661=ORIENTED_EDGE('',*,*,#16942,.F.) ;
#22662=ORIENTED_EDGE('',*,*,#16943,.F.) ;
#22663=ORIENTED_EDGE('',*,*,#16941,.F.) ;
#22664=ORIENTED_EDGE('',*,*,#16942,.T.) ;
#22665=ORIENTED_EDGE('',*,*,#16943,.T.) ;
#22666=ORIENTED_EDGE('',*,*,#16944,.T.) ;
#22667=ORIENTED_EDGE('',*,*,#16936,.T.) ;
#22668=ORIENTED_EDGE('',*,*,#16944,.F.) ;
#22669=ORIENTED_EDGE('',*,*,#16945,.F.) ;
#22670=ORIENTED_EDGE('',*,*,#16946,.T.) ;
#22671=ORIENTED_EDGE('',*,*,#16947,.F.) ;
#22672=ORIENTED_EDGE('',*,*,#16948,.F.) ;
#22673=ORIENTED_EDGE('',*,*,#16946,.F.) ;
#22674=ORIENTED_EDGE('',*,*,#16947,.T.) ;
#22675=ORIENTED_EDGE('',*,*,#16948,.T.) ;
#22676=ORIENTED_EDGE('',*,*,#16949,.T.) ;
#22677=ORIENTED_EDGE('',*,*,#16935,.T.) ;
#22678=ORIENTED_EDGE('',*,*,#16949,.F.) ;
#22679=ORIENTED_EDGE('',*,*,#16950,.F.) ;
#22680=ORIENTED_EDGE('',*,*,#16951,.T.) ;
#22681=ORIENTED_EDGE('',*,*,#16952,.F.) ;
#22682=ORIENTED_EDGE('',*,*,#16953,.F.) ;
#22683=ORIENTED_EDGE('',*,*,#16951,.F.) ;
#22684=ORIENTED_EDGE('',*,*,#16952,.T.) ;
#22685=ORIENTED_EDGE('',*,*,#16953,.T.) ;
#22686=ORIENTED_EDGE('',*,*,#16954,.T.) ;
#22687=ORIENTED_EDGE('',*,*,#16934,.T.) ;
#22688=ORIENTED_EDGE('',*,*,#16954,.F.) ;
#22689=ORIENTED_EDGE('',*,*,#16955,.F.) ;
#22690=ORIENTED_EDGE('',*,*,#16956,.T.) ;
#22691=ORIENTED_EDGE('',*,*,#16957,.F.) ;
#22692=ORIENTED_EDGE('',*,*,#16958,.F.) ;
#22693=ORIENTED_EDGE('',*,*,#16956,.F.) ;
#22694=ORIENTED_EDGE('',*,*,#16957,.T.) ;
#22695=ORIENTED_EDGE('',*,*,#16958,.T.) ;
#22696=ORIENTED_EDGE('',*,*,#16959,.T.) ;
#22697=ORIENTED_EDGE('',*,*,#16933,.T.) ;
#22698=ORIENTED_EDGE('',*,*,#16959,.F.) ;
#22699=ORIENTED_EDGE('',*,*,#16960,.T.) ;
#22700=ORIENTED_EDGE('',*,*,#16961,.F.) ;
#22701=ORIENTED_EDGE('',*,*,#16932,.F.) ;
#22702=ORIENTED_EDGE('',*,*,#16962,.F.) ;
#22703=ORIENTED_EDGE('',*,*,#16723,.T.) ;
#22704=ORIENTED_EDGE('',*,*,#16922,.F.) ;
#22705=ORIENTED_EDGE('',*,*,#16963,.F.) ;
#22706=ORIENTED_EDGE('',*,*,#16478,.F.) ;
#22707=ORIENTED_EDGE('',*,*,#16720,.F.) ;
#22708=ORIENTED_EDGE('',*,*,#16926,.F.) ;
#22709=ORIENTED_EDGE('',*,*,#16744,.F.) ;
#22710=ORIENTED_EDGE('',*,*,#16725,.F.) ;
#22711=ORIENTED_EDGE('',*,*,#16482,.F.) ;
#22712=ORIENTED_EDGE('',*,*,#16964,.T.) ;
#22713=ORIENTED_EDGE('',*,*,#16808,.F.) ;
#22714=ORIENTED_EDGE('',*,*,#16469,.F.) ;
#22715=ORIENTED_EDGE('',*,*,#16965,.F.) ;
#22716=ORIENTED_EDGE('',*,*,#16585,.F.) ;
#22717=ORIENTED_EDGE('',*,*,#16966,.T.) ;
#22718=ORIENTED_EDGE('',*,*,#16967,.F.) ;
#22719=ORIENTED_EDGE('',*,*,#16852,.F.) ;
#22720=ORIENTED_EDGE('',*,*,#16968,.F.) ;
#22721=ORIENTED_EDGE('',*,*,#16969,.F.) ;
#22722=ORIENTED_EDGE('',*,*,#16850,.F.) ;
#22723=ORIENTED_EDGE('',*,*,#16970,.F.) ;
#22724=ORIENTED_EDGE('',*,*,#16691,.T.) ;
#22725=ORIENTED_EDGE('',*,*,#16587,.F.) ;
#22726=ORIENTED_EDGE('',*,*,#16971,.F.) ;
#22727=ORIENTED_EDGE('',*,*,#16467,.F.) ;
#22728=ORIENTED_EDGE('',*,*,#16811,.F.) ;
#22729=ORIENTED_EDGE('',*,*,#16972,.T.) ;
#22730=ORIENTED_EDGE('',*,*,#16593,.T.) ;
#22731=ORIENTED_EDGE('',*,*,#16973,.F.) ;
#22732=ORIENTED_EDGE('',*,*,#16507,.T.) ;
#22733=ORIENTED_EDGE('',*,*,#16974,.F.) ;
#22734=ORIENTED_EDGE('',*,*,#16594,.T.) ;
#22735=ORIENTED_EDGE('',*,*,#16972,.F.) ;
#22736=ORIENTED_EDGE('',*,*,#16510,.T.) ;
#22737=ORIENTED_EDGE('',*,*,#16975,.T.) ;
#22738=ORIENTED_EDGE('',*,*,#16591,.T.) ;
#22739=ORIENTED_EDGE('',*,*,#16974,.T.) ;
#22740=ORIENTED_EDGE('',*,*,#16509,.T.) ;
#22741=ORIENTED_EDGE('',*,*,#16973,.T.) ;
#22742=ORIENTED_EDGE('',*,*,#16592,.T.) ;
#22743=ORIENTED_EDGE('',*,*,#16975,.F.) ;
#22744=ORIENTED_EDGE('',*,*,#16508,.T.) ;
#22745=ORIENTED_EDGE('',*,*,#16489,.T.) ;
#22746=ORIENTED_EDGE('',*,*,#16976,.T.) ;
#22747=ORIENTED_EDGE('',*,*,#16977,.F.) ;
#22748=ORIENTED_EDGE('',*,*,#16978,.F.) ;
#22749=ORIENTED_EDGE('',*,*,#16472,.F.) ;
#22750=ORIENTED_EDGE('',*,*,#16979,.T.) ;
#22751=ORIENTED_EDGE('',*,*,#16582,.F.) ;
#22752=ORIENTED_EDGE('',*,*,#16980,.T.) ;
#22753=ORIENTED_EDGE('',*,*,#16468,.F.) ;
#22754=ORIENTED_EDGE('',*,*,#16971,.T.) ;
#22755=ORIENTED_EDGE('',*,*,#16586,.F.) ;
#22756=ORIENTED_EDGE('',*,*,#16965,.T.) ;
#22757=ORIENTED_EDGE('',*,*,#16437,.F.) ;
#22758=ORIENTED_EDGE('',*,*,#16465,.T.) ;
#22759=ORIENTED_EDGE('',*,*,#16435,.F.) ;
#22760=ORIENTED_EDGE('',*,*,#16589,.T.) ;
#22761=ORIENTED_EDGE('',*,*,#16480,.F.) ;
#22762=ORIENTED_EDGE('',*,*,#16981,.T.) ;
#22763=ORIENTED_EDGE('',*,*,#16607,.T.) ;
#22764=ORIENTED_EDGE('',*,*,#16982,.T.) ;
#22765=ORIENTED_EDGE('',*,*,#16983,.T.) ;
#22766=ORIENTED_EDGE('',*,*,#16595,.T.) ;
#22767=ORIENTED_EDGE('',*,*,#16984,.T.) ;
#22768=ORIENTED_EDGE('',*,*,#16501,.T.) ;
#22769=ORIENTED_EDGE('',*,*,#16985,.T.) ;
#22770=ORIENTED_EDGE('',*,*,#16596,.T.) ;
#22771=ORIENTED_EDGE('',*,*,#16983,.F.) ;
#22772=ORIENTED_EDGE('',*,*,#16500,.T.) ;
#22773=ORIENTED_EDGE('',*,*,#16986,.T.) ;
#22774=ORIENTED_EDGE('',*,*,#16597,.T.) ;
#22775=ORIENTED_EDGE('',*,*,#16985,.F.) ;
#22776=ORIENTED_EDGE('',*,*,#16499,.T.) ;
#22777=ORIENTED_EDGE('',*,*,#16984,.F.) ;
#22778=ORIENTED_EDGE('',*,*,#16598,.T.) ;
#22779=ORIENTED_EDGE('',*,*,#16986,.F.) ;
#22780=ORIENTED_EDGE('',*,*,#16502,.T.) ;
#22781=ORIENTED_EDGE('',*,*,#16987,.T.) ;
#22782=ORIENTED_EDGE('',*,*,#16599,.T.) ;
#22783=ORIENTED_EDGE('',*,*,#16988,.T.) ;
#22784=ORIENTED_EDGE('',*,*,#16505,.T.) ;
#22785=ORIENTED_EDGE('',*,*,#16989,.T.) ;
#22786=ORIENTED_EDGE('',*,*,#16600,.T.) ;
#22787=ORIENTED_EDGE('',*,*,#16987,.F.) ;
#22788=ORIENTED_EDGE('',*,*,#16504,.T.) ;
#22789=ORIENTED_EDGE('',*,*,#16990,.T.) ;
#22790=ORIENTED_EDGE('',*,*,#16601,.T.) ;
#22791=ORIENTED_EDGE('',*,*,#16989,.F.) ;
#22792=ORIENTED_EDGE('',*,*,#16503,.T.) ;
#22793=ORIENTED_EDGE('',*,*,#16988,.F.) ;
#22794=ORIENTED_EDGE('',*,*,#16602,.T.) ;
#22795=ORIENTED_EDGE('',*,*,#16990,.F.) ;
#22796=ORIENTED_EDGE('',*,*,#16506,.T.) ;
#22797=ORIENTED_EDGE('',*,*,#16991,.T.) ;
#22798=ORIENTED_EDGE('',*,*,#16603,.F.) ;
#22799=ORIENTED_EDGE('',*,*,#16992,.T.) ;
#22800=ORIENTED_EDGE('',*,*,#16930,.F.) ;
#22801=ORIENTED_EDGE('',*,*,#16993,.F.) ;
#22802=ORIENTED_EDGE('',*,*,#16604,.T.) ;
#22803=ORIENTED_EDGE('',*,*,#16991,.F.) ;
#22804=ORIENTED_EDGE('',*,*,#16929,.T.) ;
#22805=ORIENTED_EDGE('',*,*,#16994,.T.) ;
#22806=ORIENTED_EDGE('',*,*,#16605,.F.) ;
#22807=ORIENTED_EDGE('',*,*,#16993,.T.) ;
#22808=ORIENTED_EDGE('',*,*,#16928,.F.) ;
#22809=ORIENTED_EDGE('',*,*,#16995,.T.) ;
#22810=ORIENTED_EDGE('',*,*,#16996,.F.) ;
#22811=ORIENTED_EDGE('',*,*,#16580,.F.) ;
#22812=ORIENTED_EDGE('',*,*,#16711,.F.) ;
#22813=ORIENTED_EDGE('',*,*,#16693,.F.) ;
#22814=ORIENTED_EDGE('',*,*,#16473,.F.) ;
#22815=ORIENTED_EDGE('',*,*,#16980,.F.) ;
#22816=ORIENTED_EDGE('',*,*,#16581,.F.) ;
#22817=ORIENTED_EDGE('',*,*,#16996,.T.) ;
#22818=ORIENTED_EDGE('',*,*,#16997,.F.) ;
#22819=ORIENTED_EDGE('',*,*,#16856,.F.) ;
#22820=ORIENTED_EDGE('',*,*,#16998,.F.) ;
#22821=ORIENTED_EDGE('',*,*,#16999,.F.) ;
#22822=ORIENTED_EDGE('',*,*,#17000,.F.) ;
#22823=ORIENTED_EDGE('',*,*,#16966,.F.) ;
#22824=ORIENTED_EDGE('',*,*,#16584,.T.) ;
#22825=ORIENTED_EDGE('',*,*,#17001,.F.) ;
#22826=ORIENTED_EDGE('',*,*,#16854,.F.) ;
#22827=ORIENTED_EDGE('',*,*,#17002,.F.) ;
#22828=ORIENTED_EDGE('',*,*,#16999,.T.) ;
#22829=ORIENTED_EDGE('',*,*,#16583,.T.) ;
#22830=ORIENTED_EDGE('',*,*,#16979,.F.) ;
#22831=ORIENTED_EDGE('',*,*,#16471,.F.) ;
#22832=ORIENTED_EDGE('',*,*,#16807,.F.) ;
#22833=ORIENTED_EDGE('',*,*,#16963,.T.) ;
#22834=ORIENTED_EDGE('',*,*,#16921,.T.) ;
#22835=ORIENTED_EDGE('',*,*,#17003,.F.) ;
#22836=ORIENTED_EDGE('',*,*,#16977,.T.) ;
#22837=ORIENTED_EDGE('',*,*,#17004,.F.) ;
#22838=ORIENTED_EDGE('',*,*,#16931,.T.) ;
#22839=ORIENTED_EDGE('',*,*,#16992,.F.) ;
#22840=ORIENTED_EDGE('',*,*,#16608,.T.) ;
#22841=ORIENTED_EDGE('',*,*,#16981,.F.) ;
#22842=ORIENTED_EDGE('',*,*,#16479,.T.) ;
#22843=ORIENTED_EDGE('',*,*,#16481,.T.) ;
#22844=ORIENTED_EDGE('',*,*,#16982,.F.) ;
#22845=ORIENTED_EDGE('',*,*,#16606,.T.) ;
#22846=ORIENTED_EDGE('',*,*,#16994,.F.) ;
#22847=ORIENTED_EDGE('',*,*,#16927,.T.) ;
#22848=ORIENTED_EDGE('',*,*,#16964,.F.) ;
#22849=ORIENTED_EDGE('',*,*,#17005,.T.) ;
#22850=ORIENTED_EDGE('',*,*,#17006,.T.) ;
#22851=ORIENTED_EDGE('',*,*,#16833,.F.) ;
#22852=ORIENTED_EDGE('',*,*,#16868,.F.) ;
#22853=ORIENTED_EDGE('',*,*,#16866,.T.) ;
#22854=ORIENTED_EDGE('',*,*,#16909,.F.) ;
#22855=ORIENTED_EDGE('',*,*,#16911,.T.) ;
#22856=ORIENTED_EDGE('',*,*,#16912,.F.) ;
#22857=ORIENTED_EDGE('',*,*,#16831,.F.) ;
#22858=ORIENTED_EDGE('',*,*,#17007,.F.) ;
#22859=ORIENTED_EDGE('',*,*,#16840,.F.) ;
#22860=ORIENTED_EDGE('',*,*,#17008,.F.) ;
#22861=ORIENTED_EDGE('',*,*,#17009,.T.) ;
#22862=ORIENTED_EDGE('',*,*,#16535,.T.) ;
#22863=ORIENTED_EDGE('',*,*,#17009,.F.) ;
#22864=ORIENTED_EDGE('',*,*,#17010,.F.) ;
#22865=ORIENTED_EDGE('',*,*,#17008,.T.) ;
#22866=ORIENTED_EDGE('',*,*,#17011,.T.) ;
#22867=ORIENTED_EDGE('',*,*,#16674,.T.) ;
#22868=ORIENTED_EDGE('',*,*,#17011,.F.) ;
#22869=ORIENTED_EDGE('',*,*,#17010,.T.) ;
#22870=ORIENTED_EDGE('',*,*,#16555,.F.) ;
#22871=ORIENTED_EDGE('',*,*,#16372,.F.) ;
#22872=ORIENTED_EDGE('',*,*,#16396,.F.) ;
#22873=ORIENTED_EDGE('',*,*,#16380,.F.) ;
#22874=ORIENTED_EDGE('',*,*,#16379,.F.) ;
#22875=ORIENTED_EDGE('',*,*,#16647,.F.) ;
#22876=ORIENTED_EDGE('',*,*,#16646,.F.) ;
#22877=ORIENTED_EDGE('',*,*,#16365,.T.) ;
#22878=ORIENTED_EDGE('',*,*,#16364,.T.) ;
#22879=ORIENTED_EDGE('',*,*,#16399,.T.) ;
#22880=ORIENTED_EDGE('',*,*,#16362,.T.) ;
#22881=ORIENTED_EDGE('',*,*,#16358,.T.) ;
#22882=ORIENTED_EDGE('',*,*,#16553,.F.) ;
#22883=ORIENTED_EDGE('',*,*,#16356,.F.) ;
#22884=ORIENTED_EDGE('',*,*,#16361,.F.) ;
#22885=ORIENTED_EDGE('',*,*,#16360,.F.) ;
#22886=ORIENTED_EDGE('',*,*,#16398,.F.) ;
#22887=ORIENTED_EDGE('',*,*,#16367,.F.) ;
#22888=ORIENTED_EDGE('',*,*,#16645,.F.) ;
#22889=ORIENTED_EDGE('',*,*,#16377,.F.) ;
#22890=ORIENTED_EDGE('',*,*,#16376,.F.) ;
#22891=ORIENTED_EDGE('',*,*,#16397,.F.) ;
#22892=ORIENTED_EDGE('',*,*,#16374,.F.) ;
#22893=ORIENTED_EDGE('',*,*,#16370,.F.) ;
#22894=ORIENTED_EDGE('',*,*,#16554,.F.) ;
#22895=ORIENTED_EDGE('',*,*,#16558,.F.) ;
#22896=ORIENTED_EDGE('',*,*,#16385,.F.) ;
#22897=ORIENTED_EDGE('',*,*,#16394,.F.) ;
#22898=ORIENTED_EDGE('',*,*,#16393,.F.) ;
#22899=ORIENTED_EDGE('',*,*,#16392,.F.) ;
#22900=ORIENTED_EDGE('',*,*,#16650,.F.) ;
#22901=ORIENTED_EDGE('',*,*,#16649,.F.) ;
#22902=ORIENTED_EDGE('',*,*,#16352,.T.) ;
#22903=ORIENTED_EDGE('',*,*,#16351,.T.) ;
#22904=ORIENTED_EDGE('',*,*,#16401,.T.) ;
#22905=ORIENTED_EDGE('',*,*,#16349,.T.) ;
#22906=ORIENTED_EDGE('',*,*,#16345,.T.) ;
#22907=ORIENTED_EDGE('',*,*,#16556,.F.) ;
#22908=ORIENTED_EDGE('',*,*,#16343,.F.) ;
#22909=ORIENTED_EDGE('',*,*,#16348,.F.) ;
#22910=ORIENTED_EDGE('',*,*,#16347,.F.) ;
#22911=ORIENTED_EDGE('',*,*,#16400,.F.) ;
#22912=ORIENTED_EDGE('',*,*,#16354,.F.) ;
#22913=ORIENTED_EDGE('',*,*,#16648,.F.) ;
#22914=ORIENTED_EDGE('',*,*,#16390,.F.) ;
#22915=ORIENTED_EDGE('',*,*,#16389,.F.) ;
#22916=ORIENTED_EDGE('',*,*,#16395,.F.) ;
#22917=ORIENTED_EDGE('',*,*,#16387,.F.) ;
#22918=ORIENTED_EDGE('',*,*,#16383,.F.) ;
#22919=ORIENTED_EDGE('',*,*,#16557,.F.) ;
#22920=ORIENTED_EDGE('',*,*,#16497,.F.) ;
#22921=ORIENTED_EDGE('',*,*,#16320,.F.) ;
#22922=ORIENTED_EDGE('',*,*,#16404,.F.) ;
#22923=ORIENTED_EDGE('',*,*,#16328,.F.) ;
#22924=ORIENTED_EDGE('',*,*,#16327,.F.) ;
#22925=ORIENTED_EDGE('',*,*,#16615,.F.) ;
#22926=ORIENTED_EDGE('',*,*,#16614,.F.) ;
#22927=ORIENTED_EDGE('',*,*,#16312,.T.) ;
#22928=ORIENTED_EDGE('',*,*,#16311,.T.) ;
#22929=ORIENTED_EDGE('',*,*,#16408,.T.) ;
#22930=ORIENTED_EDGE('',*,*,#16309,.T.) ;
#22931=ORIENTED_EDGE('',*,*,#16305,.T.) ;
#22932=ORIENTED_EDGE('',*,*,#16495,.F.) ;
#22933=ORIENTED_EDGE('',*,*,#16303,.F.) ;
#22934=ORIENTED_EDGE('',*,*,#16308,.F.) ;
#22935=ORIENTED_EDGE('',*,*,#16307,.F.) ;
#22936=ORIENTED_EDGE('',*,*,#16407,.F.) ;
#22937=ORIENTED_EDGE('',*,*,#16406,.F.) ;
#22938=ORIENTED_EDGE('',*,*,#16315,.F.) ;
#22939=ORIENTED_EDGE('',*,*,#16314,.F.) ;
#22940=ORIENTED_EDGE('',*,*,#16613,.F.) ;
#22941=ORIENTED_EDGE('',*,*,#16325,.F.) ;
#22942=ORIENTED_EDGE('',*,*,#16324,.F.) ;
#22943=ORIENTED_EDGE('',*,*,#16405,.F.) ;
#22944=ORIENTED_EDGE('',*,*,#16322,.F.) ;
#22945=ORIENTED_EDGE('',*,*,#16318,.F.) ;
#22946=ORIENTED_EDGE('',*,*,#16496,.F.) ;
#22947=ORIENTED_EDGE('',*,*,#16494,.F.) ;
#22948=ORIENTED_EDGE('',*,*,#16333,.F.) ;
#22949=ORIENTED_EDGE('',*,*,#16402,.F.) ;
#22950=ORIENTED_EDGE('',*,*,#16341,.F.) ;
#22951=ORIENTED_EDGE('',*,*,#16340,.F.) ;
#22952=ORIENTED_EDGE('',*,*,#16612,.F.) ;
#22953=ORIENTED_EDGE('',*,*,#16611,.F.) ;
#22954=ORIENTED_EDGE('',*,*,#16299,.T.) ;
#22955=ORIENTED_EDGE('',*,*,#16298,.T.) ;
#22956=ORIENTED_EDGE('',*,*,#16410,.T.) ;
#22957=ORIENTED_EDGE('',*,*,#16296,.T.) ;
#22958=ORIENTED_EDGE('',*,*,#16292,.T.) ;
#22959=ORIENTED_EDGE('',*,*,#16492,.F.) ;
#22960=ORIENTED_EDGE('',*,*,#16290,.F.) ;
#22961=ORIENTED_EDGE('',*,*,#16295,.F.) ;
#22962=ORIENTED_EDGE('',*,*,#16294,.F.) ;
#22963=ORIENTED_EDGE('',*,*,#16409,.F.) ;
#22964=ORIENTED_EDGE('',*,*,#16301,.F.) ;
#22965=ORIENTED_EDGE('',*,*,#16610,.F.) ;
#22966=ORIENTED_EDGE('',*,*,#16338,.F.) ;
#22967=ORIENTED_EDGE('',*,*,#16337,.F.) ;
#22968=ORIENTED_EDGE('',*,*,#16403,.F.) ;
#22969=ORIENTED_EDGE('',*,*,#16335,.F.) ;
#22970=ORIENTED_EDGE('',*,*,#16331,.F.) ;
#22971=ORIENTED_EDGE('',*,*,#16493,.F.) ;
#22972=ORIENTED_EDGE('',*,*,#17012,.F.) ;
#22973=ORIENTED_EDGE('',*,*,#16565,.F.) ;
#22974=ORIENTED_EDGE('',*,*,#17013,.F.) ;
#22975=ORIENTED_EDGE('',*,*,#17014,.F.) ;
#22976=ORIENTED_EDGE('',*,*,#17015,.F.) ;
#22977=ORIENTED_EDGE('',*,*,#16563,.F.) ;
#22978=ORIENTED_EDGE('',*,*,#17016,.F.) ;
#22979=ORIENTED_EDGE('',*,*,#17017,.F.) ;
#22980=ORIENTED_EDGE('',*,*,#17018,.F.) ;
#22981=ORIENTED_EDGE('',*,*,#17019,.F.) ;
#22982=ORIENTED_EDGE('',*,*,#17020,.F.) ;
#22983=ORIENTED_EDGE('',*,*,#16561,.F.) ;
#22984=ORIENTED_EDGE('',*,*,#17021,.F.) ;
#22985=ORIENTED_EDGE('',*,*,#17022,.F.) ;
#22986=ORIENTED_EDGE('',*,*,#17023,.F.) ;
#22987=ORIENTED_EDGE('',*,*,#16559,.F.) ;
#22988=ORIENTED_EDGE('',*,*,#16562,.T.) ;
#22989=ORIENTED_EDGE('',*,*,#17020,.T.) ;
#22990=ORIENTED_EDGE('',*,*,#17024,.T.) ;
#22991=ORIENTED_EDGE('',*,*,#17016,.T.) ;
#22992=ORIENTED_EDGE('',*,*,#16560,.T.) ;
#22993=ORIENTED_EDGE('',*,*,#17023,.T.) ;
#22994=ORIENTED_EDGE('',*,*,#17025,.T.) ;
#22995=ORIENTED_EDGE('',*,*,#17018,.T.) ;
#22996=ORIENTED_EDGE('',*,*,#17026,.T.) ;
#22997=ORIENTED_EDGE('',*,*,#16642,.T.) ;
#22998=ORIENTED_EDGE('',*,*,#17027,.T.) ;
#22999=ORIENTED_EDGE('',*,*,#17019,.T.) ;
#23000=ORIENTED_EDGE('',*,*,#16564,.T.) ;
#23001=ORIENTED_EDGE('',*,*,#17015,.T.) ;
#23002=ORIENTED_EDGE('',*,*,#17028,.T.) ;
#23003=ORIENTED_EDGE('',*,*,#17013,.T.) ;
#23004=ORIENTED_EDGE('',*,*,#17029,.T.) ;
#23005=ORIENTED_EDGE('',*,*,#16638,.T.) ;
#23006=ORIENTED_EDGE('',*,*,#17030,.T.) ;
#23007=ORIENTED_EDGE('',*,*,#17014,.T.) ;
#23008=ORIENTED_EDGE('',*,*,#16566,.T.) ;
#23009=ORIENTED_EDGE('',*,*,#17012,.T.) ;
#23010=ORIENTED_EDGE('',*,*,#17031,.T.) ;
#23011=ORIENTED_EDGE('',*,*,#17021,.T.) ;
#23012=ORIENTED_EDGE('',*,*,#17032,.T.) ;
#23013=ORIENTED_EDGE('',*,*,#16644,.T.) ;
#23014=ORIENTED_EDGE('',*,*,#17033,.T.) ;
#23015=ORIENTED_EDGE('',*,*,#17022,.T.) ;
#23016=ORIENTED_EDGE('',*,*,#16637,.T.) ;
#23017=ORIENTED_EDGE('',*,*,#17032,.F.) ;
#23018=ORIENTED_EDGE('',*,*,#17031,.F.) ;
#23019=ORIENTED_EDGE('',*,*,#17030,.F.) ;
#23020=ORIENTED_EDGE('',*,*,#17034,.T.) ;
#23021=ORIENTED_EDGE('',*,*,#16640,.T.) ;
#23022=ORIENTED_EDGE('',*,*,#17035,.T.) ;
#23023=ORIENTED_EDGE('',*,*,#17017,.T.) ;
#23024=ORIENTED_EDGE('',*,*,#17028,.F.) ;
#23025=ORIENTED_EDGE('',*,*,#17035,.F.) ;
#23026=ORIENTED_EDGE('',*,*,#16639,.T.) ;
#23027=ORIENTED_EDGE('',*,*,#17029,.F.) ;
#23028=ORIENTED_EDGE('',*,*,#17025,.F.) ;
#23029=ORIENTED_EDGE('',*,*,#17033,.F.) ;
#23030=ORIENTED_EDGE('',*,*,#16643,.T.) ;
#23031=ORIENTED_EDGE('',*,*,#17026,.F.) ;
#23032=ORIENTED_EDGE('',*,*,#17024,.F.) ;
#23033=ORIENTED_EDGE('',*,*,#17027,.F.) ;
#23034=ORIENTED_EDGE('',*,*,#16641,.T.) ;
#23035=ORIENTED_EDGE('',*,*,#17034,.F.) ;
#23036=ORIENTED_EDGE('',*,*,#17036,.F.) ;
#23037=ORIENTED_EDGE('',*,*,#17037,.F.) ;
#23038=ORIENTED_EDGE('',*,*,#17038,.F.) ;
#23039=ORIENTED_EDGE('',*,*,#17005,.F.) ;
#23040=ORIENTED_EDGE('',*,*,#17039,.F.) ;
#23041=ORIENTED_EDGE('',*,*,#16962,.T.) ;
#23042=ORIENTED_EDGE('',*,*,#17004,.T.) ;
#23043=ORIENTED_EDGE('',*,*,#16976,.F.) ;
#23044=ORIENTED_EDGE('',*,*,#16488,.F.) ;
#23045=ORIENTED_EDGE('',*,*,#16733,.T.) ;
#23046=ORIENTED_EDGE('',*,*,#16737,.F.) ;
#23047=ORIENTED_EDGE('',*,*,#17040,.F.) ;
#23048=ORIENTED_EDGE('',*,*,#17041,.T.) ;
#23049=ORIENTED_EDGE('',*,*,#17039,.T.) ;
#23050=ORIENTED_EDGE('',*,*,#16736,.T.) ;
#23051=ORIENTED_EDGE('',*,*,#17042,.F.) ;
#23052=ORIENTED_EDGE('',*,*,#16721,.F.) ;
#23053=ORIENTED_EDGE('',*,*,#16718,.F.) ;
#23054=ORIENTED_EDGE('',*,*,#16490,.F.) ;
#23055=ORIENTED_EDGE('',*,*,#16978,.T.) ;
#23056=ORIENTED_EDGE('',*,*,#17003,.T.) ;
#23057=ORIENTED_EDGE('',*,*,#16961,.T.) ;
#23058=ORIENTED_EDGE('',*,*,#16937,.T.) ;
#23059=ORIENTED_EDGE('',*,*,#16923,.T.) ;
#23060=ORIENTED_EDGE('',*,*,#16722,.T.) ;
#23061=ORIENTED_EDGE('',*,*,#17042,.T.) ;
#23062=ORIENTED_EDGE('',*,*,#17043,.T.) ;
#23063=ORIENTED_EDGE('',*,*,#17044,.F.) ;
#23064=ORIENTED_EDGE('',*,*,#16767,.T.) ;
#23065=ORIENTED_EDGE('',*,*,#17006,.F.) ;
#23066=ORIENTED_EDGE('',*,*,#17038,.T.) ;
#23067=ORIENTED_EDGE('',*,*,#17045,.T.) ;
#23068=ORIENTED_EDGE('',*,*,#17046,.F.) ;
#23069=ORIENTED_EDGE('',*,*,#16745,.T.) ;
#23070=ORIENTED_EDGE('',*,*,#16925,.T.) ;
#23071=ORIENTED_EDGE('',*,*,#16939,.T.) ;
#23072=ORIENTED_EDGE('',*,*,#17047,.T.) ;
#23073=ORIENTED_EDGE('',*,*,#17048,.F.) ;
#23074=ORIENTED_EDGE('',*,*,#17049,.F.) ;
#23075=ORIENTED_EDGE('',*,*,#17050,.F.) ;
#23076=ORIENTED_EDGE('',*,*,#17047,.F.) ;
#23077=ORIENTED_EDGE('',*,*,#16938,.T.) ;
#23078=ORIENTED_EDGE('',*,*,#17043,.F.) ;
#23079=ORIENTED_EDGE('',*,*,#16960,.F.) ;
#23080=ORIENTED_EDGE('',*,*,#17041,.F.) ;
#23081=ORIENTED_EDGE('',*,*,#16945,.T.) ;
#23082=ORIENTED_EDGE('',*,*,#16950,.T.) ;
#23083=ORIENTED_EDGE('',*,*,#16955,.T.) ;
#23084=ORIENTED_EDGE('',*,*,#16940,.T.) ;
#23085=ORIENTED_EDGE('',*,*,#17046,.T.) ;
#23086=ORIENTED_EDGE('',*,*,#17050,.T.) ;
#23087=ORIENTED_EDGE('',*,*,#17051,.F.) ;
#23088=ORIENTED_EDGE('',*,*,#16743,.T.) ;
#23089=ORIENTED_EDGE('',*,*,#17051,.T.) ;
#23090=ORIENTED_EDGE('',*,*,#17049,.T.) ;
#23091=ORIENTED_EDGE('',*,*,#17052,.F.) ;
#23092=ORIENTED_EDGE('',*,*,#16741,.T.) ;
#23093=ORIENTED_EDGE('',*,*,#17040,.T.) ;
#23094=ORIENTED_EDGE('',*,*,#16739,.T.) ;
#23095=ORIENTED_EDGE('',*,*,#17052,.T.) ;
#23096=ORIENTED_EDGE('',*,*,#17048,.T.) ;
#23097=ORIENTED_EDGE('',*,*,#17053,.F.) ;
#23098=ORIENTED_EDGE('',*,*,#17045,.F.) ;
#23099=ORIENTED_EDGE('',*,*,#17037,.T.) ;
#23100=ORIENTED_EDGE('',*,*,#17054,.F.) ;
#23101=ORIENTED_EDGE('',*,*,#17055,.F.) ;
#23102=ORIENTED_EDGE('',*,*,#17056,.F.) ;
#23103=ORIENTED_EDGE('',*,*,#16835,.T.) ;
#23104=ORIENTED_EDGE('',*,*,#17057,.F.) ;
#23105=ORIENTED_EDGE('',*,*,#17054,.T.) ;
#23106=ORIENTED_EDGE('',*,*,#17036,.T.) ;
#23107=ORIENTED_EDGE('',*,*,#17007,.T.) ;
#23108=ORIENTED_EDGE('',*,*,#16758,.T.) ;
#23109=ORIENTED_EDGE('',*,*,#17044,.T.) ;
#23110=ORIENTED_EDGE('',*,*,#17053,.T.) ;
#23111=ORIENTED_EDGE('',*,*,#17058,.F.) ;
#23112=ORIENTED_EDGE('',*,*,#16765,.T.) ;
#23113=ORIENTED_EDGE('',*,*,#17058,.T.) ;
#23114=ORIENTED_EDGE('',*,*,#17056,.T.) ;
#23115=ORIENTED_EDGE('',*,*,#17059,.F.) ;
#23116=ORIENTED_EDGE('',*,*,#16763,.T.) ;
#23117=ORIENTED_EDGE('',*,*,#17059,.T.) ;
#23118=ORIENTED_EDGE('',*,*,#17055,.T.) ;
#23119=ORIENTED_EDGE('',*,*,#17057,.T.) ;
#23120=ORIENTED_EDGE('',*,*,#16761,.T.) ;
#23121=ORIENTED_EDGE('',*,*,#17060,.F.) ;
#23122=ORIENTED_EDGE('',*,*,#16280,.F.) ;
#23123=ORIENTED_EDGE('',*,*,#16411,.F.) ;
#23124=ORIENTED_EDGE('',*,*,#16288,.F.) ;
#23125=ORIENTED_EDGE('',*,*,#16287,.F.) ;
#23126=ORIENTED_EDGE('',*,*,#17061,.F.) ;
#23127=ORIENTED_EDGE('',*,*,#17062,.F.) ;
#23128=ORIENTED_EDGE('',*,*,#16234,.T.) ;
#23129=ORIENTED_EDGE('',*,*,#16233,.T.) ;
#23130=ORIENTED_EDGE('',*,*,#16420,.T.) ;
#23131=ORIENTED_EDGE('',*,*,#16231,.T.) ;
#23132=ORIENTED_EDGE('',*,*,#16227,.T.) ;
#23133=ORIENTED_EDGE('',*,*,#17063,.F.) ;
#23134=ORIENTED_EDGE('',*,*,#16225,.F.) ;
#23135=ORIENTED_EDGE('',*,*,#16230,.F.) ;
#23136=ORIENTED_EDGE('',*,*,#16229,.F.) ;
#23137=ORIENTED_EDGE('',*,*,#16419,.F.) ;
#23138=ORIENTED_EDGE('',*,*,#16236,.F.) ;
#23139=ORIENTED_EDGE('',*,*,#17064,.F.) ;
#23140=ORIENTED_EDGE('',*,*,#16285,.F.) ;
#23141=ORIENTED_EDGE('',*,*,#16284,.F.) ;
#23142=ORIENTED_EDGE('',*,*,#16412,.F.) ;
#23143=ORIENTED_EDGE('',*,*,#16282,.F.) ;
#23144=ORIENTED_EDGE('',*,*,#16278,.F.) ;
#23145=ORIENTED_EDGE('',*,*,#17065,.F.) ;
#23146=ORIENTED_EDGE('',*,*,#17066,.F.) ;
#23147=ORIENTED_EDGE('',*,*,#16254,.F.) ;
#23148=ORIENTED_EDGE('',*,*,#16415,.F.) ;
#23149=ORIENTED_EDGE('',*,*,#16262,.F.) ;
#23150=ORIENTED_EDGE('',*,*,#16261,.F.) ;
#23151=ORIENTED_EDGE('',*,*,#17067,.F.) ;
#23152=ORIENTED_EDGE('',*,*,#17068,.F.) ;
#23153=ORIENTED_EDGE('',*,*,#16220,.T.) ;
#23154=ORIENTED_EDGE('',*,*,#16219,.T.) ;
#23155=ORIENTED_EDGE('',*,*,#16423,.T.) ;
#23156=ORIENTED_EDGE('',*,*,#16217,.T.) ;
#23157=ORIENTED_EDGE('',*,*,#16213,.T.) ;
#23158=ORIENTED_EDGE('',*,*,#17069,.F.) ;
#23159=ORIENTED_EDGE('',*,*,#16211,.F.) ;
#23160=ORIENTED_EDGE('',*,*,#16216,.F.) ;
#23161=ORIENTED_EDGE('',*,*,#16215,.F.) ;
#23162=ORIENTED_EDGE('',*,*,#16422,.F.) ;
#23163=ORIENTED_EDGE('',*,*,#16421,.F.) ;
#23164=ORIENTED_EDGE('',*,*,#16223,.F.) ;
#23165=ORIENTED_EDGE('',*,*,#16222,.F.) ;
#23166=ORIENTED_EDGE('',*,*,#17070,.F.) ;
#23167=ORIENTED_EDGE('',*,*,#16259,.F.) ;
#23168=ORIENTED_EDGE('',*,*,#16258,.F.) ;
#23169=ORIENTED_EDGE('',*,*,#16416,.F.) ;
#23170=ORIENTED_EDGE('',*,*,#16256,.F.) ;
#23171=ORIENTED_EDGE('',*,*,#16252,.F.) ;
#23172=ORIENTED_EDGE('',*,*,#17071,.F.) ;
#23173=ORIENTED_EDGE('',*,*,#17072,.F.) ;
#23174=ORIENTED_EDGE('',*,*,#16241,.F.) ;
#23175=ORIENTED_EDGE('',*,*,#16417,.F.) ;
#23176=ORIENTED_EDGE('',*,*,#16249,.F.) ;
#23177=ORIENTED_EDGE('',*,*,#16248,.F.) ;
#23178=ORIENTED_EDGE('',*,*,#17073,.F.) ;
#23179=ORIENTED_EDGE('',*,*,#17074,.F.) ;
#23180=ORIENTED_EDGE('',*,*,#16206,.T.) ;
#23181=ORIENTED_EDGE('',*,*,#16205,.T.) ;
#23182=ORIENTED_EDGE('',*,*,#16204,.T.) ;
#23183=ORIENTED_EDGE('',*,*,#16425,.T.) ;
#23184=ORIENTED_EDGE('',*,*,#16202,.T.) ;
#23185=ORIENTED_EDGE('',*,*,#16201,.T.) ;
#23186=ORIENTED_EDGE('',*,*,#16197,.T.) ;
#23187=ORIENTED_EDGE('',*,*,#17075,.F.) ;
#23188=ORIENTED_EDGE('',*,*,#16195,.F.) ;
#23189=ORIENTED_EDGE('',*,*,#16200,.F.) ;
#23190=ORIENTED_EDGE('',*,*,#16199,.F.) ;
#23191=ORIENTED_EDGE('',*,*,#16424,.F.) ;
#23192=ORIENTED_EDGE('',*,*,#16209,.F.) ;
#23193=ORIENTED_EDGE('',*,*,#16208,.F.) ;
#23194=ORIENTED_EDGE('',*,*,#17076,.F.) ;
#23195=ORIENTED_EDGE('',*,*,#16246,.F.) ;
#23196=ORIENTED_EDGE('',*,*,#16245,.F.) ;
#23197=ORIENTED_EDGE('',*,*,#16418,.F.) ;
#23198=ORIENTED_EDGE('',*,*,#16243,.F.) ;
#23199=ORIENTED_EDGE('',*,*,#16239,.F.) ;
#23200=ORIENTED_EDGE('',*,*,#17077,.F.) ;
#23201=ORIENTED_EDGE('',*,*,#16453,.T.) ;
#23202=ORIENTED_EDGE('',*,*,#16692,.F.) ;
#23203=ORIENTED_EDGE('',*,*,#16970,.T.) ;
#23204=ORIENTED_EDGE('',*,*,#16849,.T.) ;
#23205=ORIENTED_EDGE('',*,*,#16967,.T.) ;
#23206=ORIENTED_EDGE('',*,*,#17000,.T.) ;
#23207=ORIENTED_EDGE('',*,*,#17002,.T.) ;
#23208=ORIENTED_EDGE('',*,*,#16853,.T.) ;
#23209=ORIENTED_EDGE('',*,*,#16997,.T.) ;
#23210=ORIENTED_EDGE('',*,*,#16995,.F.) ;
#23211=ORIENTED_EDGE('',*,*,#16710,.T.) ;
#23212=ORIENTED_EDGE('',*,*,#16706,.T.) ;
#23213=ORIENTED_EDGE('',*,*,#16460,.T.) ;
#23214=ORIENTED_EDGE('',*,*,#16714,.T.) ;
#23215=ORIENTED_EDGE('',*,*,#16676,.T.) ;
#23216=ORIENTED_EDGE('',*,*,#16688,.T.) ;
#23217=ORIENTED_EDGE('',*,*,#16820,.T.) ;
#23218=ORIENTED_EDGE('',*,*,#16857,.F.) ;
#23219=ORIENTED_EDGE('',*,*,#16919,.T.) ;
#23220=ORIENTED_EDGE('',*,*,#16901,.T.) ;
#23221=ORIENTED_EDGE('',*,*,#16894,.T.) ;
#23222=ORIENTED_EDGE('',*,*,#16860,.F.) ;
#23223=ORIENTED_EDGE('',*,*,#16917,.T.) ;
#23224=ORIENTED_EDGE('',*,*,#16906,.T.) ;
#23225=ORIENTED_EDGE('',*,*,#16904,.T.) ;
#23226=ORIENTED_EDGE('',*,*,#16843,.T.) ;
#23227=ORIENTED_EDGE('',*,*,#16914,.T.) ;
#23228=ORIENTED_EDGE('',*,*,#16900,.F.) ;
#23229=ORIENTED_EDGE('',*,*,#16897,.T.) ;
#23230=ORIENTED_EDGE('',*,*,#16847,.T.) ;
#23231=ORIENTED_EDGE('',*,*,#16916,.T.) ;
#23232=ORIENTED_EDGE('',*,*,#16689,.T.) ;
#23233=ORIENTED_EDGE('',*,*,#17078,.T.) ;
#23234=ORIENTED_EDGE('',*,*,#17079,.T.) ;
#23235=ORIENTED_EDGE('',*,*,#17080,.T.) ;
#23236=ORIENTED_EDGE('',*,*,#17081,.T.) ;
#23237=ORIENTED_EDGE('',*,*,#17082,.T.) ;
#23238=ORIENTED_EDGE('',*,*,#17083,.T.) ;
#23239=ORIENTED_EDGE('',*,*,#16803,.T.) ;
#23240=ORIENTED_EDGE('',*,*,#16797,.T.) ;
#23241=ORIENTED_EDGE('',*,*,#16794,.T.) ;
#23242=ORIENTED_EDGE('',*,*,#16791,.T.) ;
#23243=ORIENTED_EDGE('',*,*,#16788,.T.) ;
#23244=ORIENTED_EDGE('',*,*,#16801,.T.) ;
#23245=ORIENTED_EDGE('',*,*,#16785,.T.) ;
#23246=ORIENTED_EDGE('',*,*,#16779,.T.) ;
#23247=ORIENTED_EDGE('',*,*,#16776,.T.) ;
#23248=ORIENTED_EDGE('',*,*,#16773,.T.) ;
#23249=ORIENTED_EDGE('',*,*,#16770,.T.) ;
#23250=ORIENTED_EDGE('',*,*,#16783,.T.) ;
#23251=ORIENTED_EDGE('',*,*,#17084,.T.) ;
#23252=ORIENTED_EDGE('',*,*,#17085,.T.) ;
#23253=ORIENTED_EDGE('',*,*,#17086,.T.) ;
#23254=ORIENTED_EDGE('',*,*,#17087,.T.) ;
#23255=ORIENTED_EDGE('',*,*,#17088,.T.) ;
#23256=ORIENTED_EDGE('',*,*,#17089,.T.) ;
#23257=ORIENTED_EDGE('',*,*,#17090,.T.) ;
#23258=ORIENTED_EDGE('',*,*,#17091,.T.) ;
#23259=ORIENTED_EDGE('',*,*,#17092,.T.) ;
#23260=ORIENTED_EDGE('',*,*,#17093,.T.) ;
#23261=ORIENTED_EDGE('',*,*,#17094,.T.) ;
#23262=ORIENTED_EDGE('',*,*,#17095,.T.) ;
#23263=ORIENTED_EDGE('',*,*,#17076,.T.) ;
#23264=ORIENTED_EDGE('',*,*,#16207,.T.) ;
#23265=ORIENTED_EDGE('',*,*,#17074,.T.) ;
#23266=ORIENTED_EDGE('',*,*,#17073,.T.) ;
#23267=ORIENTED_EDGE('',*,*,#16247,.T.) ;
#23268=ORIENTED_EDGE('',*,*,#17070,.T.) ;
#23269=ORIENTED_EDGE('',*,*,#16221,.T.) ;
#23270=ORIENTED_EDGE('',*,*,#17068,.T.) ;
#23271=ORIENTED_EDGE('',*,*,#17067,.T.) ;
#23272=ORIENTED_EDGE('',*,*,#16260,.T.) ;
#23273=ORIENTED_EDGE('',*,*,#17096,.T.) ;
#23274=ORIENTED_EDGE('',*,*,#16192,.T.) ;
#23275=ORIENTED_EDGE('',*,*,#17097,.T.) ;
#23276=ORIENTED_EDGE('',*,*,#17098,.T.) ;
#23277=ORIENTED_EDGE('',*,*,#16273,.T.) ;
#23278=ORIENTED_EDGE('',*,*,#17064,.T.) ;
#23279=ORIENTED_EDGE('',*,*,#16235,.T.) ;
#23280=ORIENTED_EDGE('',*,*,#17062,.T.) ;
#23281=ORIENTED_EDGE('',*,*,#17061,.T.) ;
#23282=ORIENTED_EDGE('',*,*,#16286,.T.) ;
#23283=ORIENTED_EDGE('',*,*,#17099,.F.) ;
#23284=ORIENTED_EDGE('',*,*,#16267,.F.) ;
#23285=ORIENTED_EDGE('',*,*,#16413,.F.) ;
#23286=ORIENTED_EDGE('',*,*,#16275,.F.) ;
#23287=ORIENTED_EDGE('',*,*,#16274,.F.) ;
#23288=ORIENTED_EDGE('',*,*,#17098,.F.) ;
#23289=ORIENTED_EDGE('',*,*,#17097,.F.) ;
#23290=ORIENTED_EDGE('',*,*,#16191,.T.) ;
#23291=ORIENTED_EDGE('',*,*,#16190,.T.) ;
#23292=ORIENTED_EDGE('',*,*,#16427,.T.) ;
#23293=ORIENTED_EDGE('',*,*,#16188,.T.) ;
#23294=ORIENTED_EDGE('',*,*,#16184,.T.) ;
#23295=ORIENTED_EDGE('',*,*,#17100,.F.) ;
#23296=ORIENTED_EDGE('',*,*,#16182,.F.) ;
#23297=ORIENTED_EDGE('',*,*,#16187,.F.) ;
#23298=ORIENTED_EDGE('',*,*,#16186,.F.) ;
#23299=ORIENTED_EDGE('',*,*,#16426,.F.) ;
#23300=ORIENTED_EDGE('',*,*,#16193,.F.) ;
#23301=ORIENTED_EDGE('',*,*,#17096,.F.) ;
#23302=ORIENTED_EDGE('',*,*,#16272,.F.) ;
#23303=ORIENTED_EDGE('',*,*,#16271,.F.) ;
#23304=ORIENTED_EDGE('',*,*,#16414,.F.) ;
#23305=ORIENTED_EDGE('',*,*,#16269,.F.) ;
#23306=ORIENTED_EDGE('',*,*,#16265,.F.) ;
#23307=ORIENTED_EDGE('',*,*,#17101,.F.) ;
#23308=ORIENTED_EDGE('',*,*,#17102,.F.) ;
#23309=ORIENTED_EDGE('',*,*,#17103,.T.) ;
#23310=ORIENTED_EDGE('',*,*,#17095,.F.) ;
#23311=ORIENTED_EDGE('',*,*,#17104,.F.) ;
#23312=ORIENTED_EDGE('',*,*,#17105,.F.) ;
#23313=ORIENTED_EDGE('',*,*,#17104,.T.) ;
#23314=ORIENTED_EDGE('',*,*,#17094,.F.) ;
#23315=ORIENTED_EDGE('',*,*,#17106,.F.) ;
#23316=ORIENTED_EDGE('',*,*,#17107,.F.) ;
#23317=ORIENTED_EDGE('',*,*,#17108,.T.) ;
#23318=ORIENTED_EDGE('',*,*,#17090,.F.) ;
#23319=ORIENTED_EDGE('',*,*,#17103,.F.) ;
#23320=ORIENTED_EDGE('',*,*,#17109,.F.) ;
#23321=ORIENTED_EDGE('',*,*,#17110,.T.) ;
#23322=ORIENTED_EDGE('',*,*,#17091,.F.) ;
#23323=ORIENTED_EDGE('',*,*,#17108,.F.) ;
#23324=ORIENTED_EDGE('',*,*,#17111,.F.) ;
#23325=ORIENTED_EDGE('',*,*,#17112,.T.) ;
#23326=ORIENTED_EDGE('',*,*,#17092,.F.) ;
#23327=ORIENTED_EDGE('',*,*,#17110,.F.) ;
#23328=ORIENTED_EDGE('',*,*,#17113,.F.) ;
#23329=ORIENTED_EDGE('',*,*,#17106,.T.) ;
#23330=ORIENTED_EDGE('',*,*,#17093,.F.) ;
#23331=ORIENTED_EDGE('',*,*,#17112,.F.) ;
#23332=ORIENTED_EDGE('',*,*,#17114,.F.) ;
#23333=ORIENTED_EDGE('',*,*,#17115,.T.) ;
#23334=ORIENTED_EDGE('',*,*,#17083,.F.) ;
#23335=ORIENTED_EDGE('',*,*,#17116,.F.) ;
#23336=ORIENTED_EDGE('',*,*,#17117,.F.) ;
#23337=ORIENTED_EDGE('',*,*,#17116,.T.) ;
#23338=ORIENTED_EDGE('',*,*,#17082,.F.) ;
#23339=ORIENTED_EDGE('',*,*,#17118,.F.) ;
#23340=ORIENTED_EDGE('',*,*,#17119,.F.) ;
#23341=ORIENTED_EDGE('',*,*,#17120,.T.) ;
#23342=ORIENTED_EDGE('',*,*,#17078,.F.) ;
#23343=ORIENTED_EDGE('',*,*,#17115,.F.) ;
#23344=ORIENTED_EDGE('',*,*,#17121,.F.) ;
#23345=ORIENTED_EDGE('',*,*,#17122,.T.) ;
#23346=ORIENTED_EDGE('',*,*,#17079,.F.) ;
#23347=ORIENTED_EDGE('',*,*,#17120,.F.) ;
#23348=ORIENTED_EDGE('',*,*,#17123,.F.) ;
#23349=ORIENTED_EDGE('',*,*,#17124,.T.) ;
#23350=ORIENTED_EDGE('',*,*,#17080,.F.) ;
#23351=ORIENTED_EDGE('',*,*,#17122,.F.) ;
#23352=ORIENTED_EDGE('',*,*,#17125,.F.) ;
#23353=ORIENTED_EDGE('',*,*,#17118,.T.) ;
#23354=ORIENTED_EDGE('',*,*,#17081,.F.) ;
#23355=ORIENTED_EDGE('',*,*,#17124,.F.) ;
#23356=ORIENTED_EDGE('',*,*,#16448,.T.) ;
#23357=ORIENTED_EDGE('',*,*,#16431,.F.) ;
#23358=ORIENTED_EDGE('',*,*,#16915,.F.) ;
#23359=ORIENTED_EDGE('',*,*,#16845,.T.) ;
#23360=ORIENTED_EDGE('',*,*,#16896,.F.) ;
#23361=ORIENTED_EDGE('',*,*,#16814,.F.) ;
#23362=ORIENTED_EDGE('',*,*,#16913,.F.) ;
#23363=ORIENTED_EDGE('',*,*,#16841,.T.) ;
#23364=ORIENTED_EDGE('',*,*,#16903,.T.) ;
#23365=ORIENTED_EDGE('',*,*,#16816,.F.) ;
#23366=ORIENTED_EDGE('',*,*,#16918,.T.) ;
#23367=ORIENTED_EDGE('',*,*,#16862,.T.) ;
#23368=ORIENTED_EDGE('',*,*,#16893,.T.) ;
#23369=ORIENTED_EDGE('',*,*,#16806,.F.) ;
#23370=ORIENTED_EDGE('',*,*,#16920,.T.) ;
#23371=ORIENTED_EDGE('',*,*,#16858,.T.) ;
#23372=ORIENTED_EDGE('',*,*,#16818,.T.) ;
#23373=ORIENTED_EDGE('',*,*,#16513,.F.) ;
#23374=ORIENTED_EDGE('',*,*,#16678,.F.) ;
#23375=ORIENTED_EDGE('',*,*,#16462,.F.) ;
#23376=ORIENTED_EDGE('',*,*,#16709,.F.) ;
#23377=ORIENTED_EDGE('',*,*,#16694,.T.) ;
#23378=ORIENTED_EDGE('',*,*,#16998,.T.) ;
#23379=ORIENTED_EDGE('',*,*,#16855,.T.) ;
#23380=ORIENTED_EDGE('',*,*,#17001,.T.) ;
#23381=ORIENTED_EDGE('',*,*,#16809,.F.) ;
#23382=ORIENTED_EDGE('',*,*,#16968,.T.) ;
#23383=ORIENTED_EDGE('',*,*,#16851,.T.) ;
#23384=ORIENTED_EDGE('',*,*,#16969,.T.) ;
#23385=ORIENTED_EDGE('',*,*,#16810,.F.) ;
#23386=ORIENTED_EDGE('',*,*,#16778,.T.) ;
#23387=ORIENTED_EDGE('',*,*,#16784,.T.) ;
#23388=ORIENTED_EDGE('',*,*,#16781,.T.) ;
#23389=ORIENTED_EDGE('',*,*,#16768,.T.) ;
#23390=ORIENTED_EDGE('',*,*,#16772,.T.) ;
#23391=ORIENTED_EDGE('',*,*,#16775,.T.) ;
#23392=ORIENTED_EDGE('',*,*,#16796,.T.) ;
#23393=ORIENTED_EDGE('',*,*,#16802,.T.) ;
#23394=ORIENTED_EDGE('',*,*,#16799,.T.) ;
#23395=ORIENTED_EDGE('',*,*,#16786,.T.) ;
#23396=ORIENTED_EDGE('',*,*,#16790,.T.) ;
#23397=ORIENTED_EDGE('',*,*,#16793,.T.) ;
#23398=ORIENTED_EDGE('',*,*,#17063,.T.) ;
#23399=ORIENTED_EDGE('',*,*,#17065,.T.) ;
#23400=ORIENTED_EDGE('',*,*,#16277,.T.) ;
#23401=ORIENTED_EDGE('',*,*,#16281,.T.) ;
#23402=ORIENTED_EDGE('',*,*,#17060,.T.) ;
#23403=ORIENTED_EDGE('',*,*,#16226,.T.) ;
#23404=ORIENTED_EDGE('',*,*,#17069,.T.) ;
#23405=ORIENTED_EDGE('',*,*,#17071,.T.) ;
#23406=ORIENTED_EDGE('',*,*,#16251,.T.) ;
#23407=ORIENTED_EDGE('',*,*,#16255,.T.) ;
#23408=ORIENTED_EDGE('',*,*,#17066,.T.) ;
#23409=ORIENTED_EDGE('',*,*,#16212,.T.) ;
#23410=ORIENTED_EDGE('',*,*,#17075,.T.) ;
#23411=ORIENTED_EDGE('',*,*,#17077,.T.) ;
#23412=ORIENTED_EDGE('',*,*,#16238,.T.) ;
#23413=ORIENTED_EDGE('',*,*,#16242,.T.) ;
#23414=ORIENTED_EDGE('',*,*,#17072,.T.) ;
#23415=ORIENTED_EDGE('',*,*,#16196,.T.) ;
#23416=ORIENTED_EDGE('',*,*,#17100,.T.) ;
#23417=ORIENTED_EDGE('',*,*,#17101,.T.) ;
#23418=ORIENTED_EDGE('',*,*,#16264,.T.) ;
#23419=ORIENTED_EDGE('',*,*,#16268,.T.) ;
#23420=ORIENTED_EDGE('',*,*,#17099,.T.) ;
#23421=ORIENTED_EDGE('',*,*,#16183,.T.) ;
#23422=ORIENTED_EDGE('',*,*,#17107,.T.) ;
#23423=ORIENTED_EDGE('',*,*,#17102,.T.) ;
#23424=ORIENTED_EDGE('',*,*,#17105,.T.) ;
#23425=ORIENTED_EDGE('',*,*,#17113,.T.) ;
#23426=ORIENTED_EDGE('',*,*,#17111,.T.) ;
#23427=ORIENTED_EDGE('',*,*,#17109,.T.) ;
#23428=ORIENTED_EDGE('',*,*,#17119,.T.) ;
#23429=ORIENTED_EDGE('',*,*,#17114,.T.) ;
#23430=ORIENTED_EDGE('',*,*,#17117,.T.) ;
#23431=ORIENTED_EDGE('',*,*,#17125,.T.) ;
#23432=ORIENTED_EDGE('',*,*,#17123,.T.) ;
#23433=ORIENTED_EDGE('',*,*,#17121,.T.) ;
#23434=ORIENTED_EDGE('',*,*,#17126,.T.) ;
#23435=ORIENTED_EDGE('',*,*,#17127,.T.) ;
#23436=ORIENTED_EDGE('',*,*,#17128,.T.) ;
#23437=ORIENTED_EDGE('',*,*,#17129,.T.) ;
#23438=ORIENTED_EDGE('',*,*,#17130,.T.) ;
#23439=ORIENTED_EDGE('',*,*,#17131,.T.) ;
#23440=ORIENTED_EDGE('',*,*,#17127,.F.) ;
#23441=ORIENTED_EDGE('',*,*,#17132,.T.) ;
#23442=ORIENTED_EDGE('',*,*,#17089,.F.) ;
#23443=ORIENTED_EDGE('',*,*,#17133,.F.) ;
#23444=ORIENTED_EDGE('',*,*,#17128,.F.) ;
#23445=ORIENTED_EDGE('',*,*,#17133,.T.) ;
#23446=ORIENTED_EDGE('',*,*,#17088,.F.) ;
#23447=ORIENTED_EDGE('',*,*,#17134,.F.) ;
#23448=ORIENTED_EDGE('',*,*,#17126,.F.) ;
#23449=ORIENTED_EDGE('',*,*,#17135,.T.) ;
#23450=ORIENTED_EDGE('',*,*,#17084,.F.) ;
#23451=ORIENTED_EDGE('',*,*,#17132,.F.) ;
#23452=ORIENTED_EDGE('',*,*,#17131,.F.) ;
#23453=ORIENTED_EDGE('',*,*,#17136,.T.) ;
#23454=ORIENTED_EDGE('',*,*,#17085,.F.) ;
#23455=ORIENTED_EDGE('',*,*,#17135,.F.) ;
#23456=ORIENTED_EDGE('',*,*,#17130,.F.) ;
#23457=ORIENTED_EDGE('',*,*,#17137,.T.) ;
#23458=ORIENTED_EDGE('',*,*,#17086,.F.) ;
#23459=ORIENTED_EDGE('',*,*,#17136,.F.) ;
#23460=ORIENTED_EDGE('',*,*,#17129,.F.) ;
#23461=ORIENTED_EDGE('',*,*,#17134,.T.) ;
#23462=ORIENTED_EDGE('',*,*,#17087,.F.) ;
#23463=ORIENTED_EDGE('',*,*,#17137,.F.) ;
#30056=CYLINDRICAL_SURFACE('',#33201,2.05475) ;
#30057=CYLINDRICAL_SURFACE('',#33203,2.05475) ;
#30058=CYLINDRICAL_SURFACE('',#33204,2.05475) ;
#30059=CYLINDRICAL_SURFACE('',#33206,2.05475000000001) ;
#30060=CYLINDRICAL_SURFACE('',#33208,2.05475000000001) ;
#30061=CYLINDRICAL_SURFACE('',#33209,2.05475000000001) ;
#30062=CYLINDRICAL_SURFACE('',#33211,2.05475000000001) ;
#30063=CYLINDRICAL_SURFACE('',#33213,2.05475000000001) ;
#30064=CYLINDRICAL_SURFACE('',#33214,2.05475000000001) ;
#30065=CYLINDRICAL_SURFACE('',#33216,2.05474999999993) ;
#30066=CYLINDRICAL_SURFACE('',#33218,2.05474999999993) ;
#30067=CYLINDRICAL_SURFACE('',#33219,2.05474999999993) ;
#30068=CYLINDRICAL_SURFACE('',#33221,1.66599999999999) ;
#30069=CYLINDRICAL_SURFACE('',#33223,1.66599999999999) ;
#30070=CYLINDRICAL_SURFACE('',#33225,1.66599999999999) ;
#30071=CYLINDRICAL_SURFACE('',#33227,1.66599999999999) ;
#30072=CYLINDRICAL_SURFACE('',#33229,1.66599999999999) ;
#30073=CYLINDRICAL_SURFACE('',#33231,1.66599999999999) ;
#30074=CYLINDRICAL_SURFACE('',#33233,1.66599999999999) ;
#30075=CYLINDRICAL_SURFACE('',#33235,1.66599999999999) ;
#30076=CYLINDRICAL_SURFACE('',#33237,1.66599999999999) ;
#30077=CYLINDRICAL_SURFACE('',#33239,1.66599999999998) ;
#30078=CYLINDRICAL_SURFACE('',#33241,1.66599999999998) ;
#30079=CYLINDRICAL_SURFACE('',#33243,1.66599999999998) ;
#30080=CYLINDRICAL_SURFACE('',#33245,2.05475) ;
#30081=CYLINDRICAL_SURFACE('',#33247,2.05475) ;
#30082=CYLINDRICAL_SURFACE('',#33248,2.05475) ;
#30083=CYLINDRICAL_SURFACE('',#33250,2.05475) ;
#30084=CYLINDRICAL_SURFACE('',#33252,2.05475) ;
#30085=CYLINDRICAL_SURFACE('',#33253,2.05475) ;
#30086=CYLINDRICAL_SURFACE('',#33255,1.666) ;
#30087=CYLINDRICAL_SURFACE('',#33257,1.666) ;
#30088=CYLINDRICAL_SURFACE('',#33259,1.666) ;
#30089=CYLINDRICAL_SURFACE('',#33261,1.666) ;
#30090=CYLINDRICAL_SURFACE('',#33263,1.666) ;
#30091=CYLINDRICAL_SURFACE('',#33265,1.666) ;
#30092=CYLINDRICAL_SURFACE('',#33267,2.05475) ;
#30093=CYLINDRICAL_SURFACE('',#33269,2.05475) ;
#30094=CYLINDRICAL_SURFACE('',#33270,2.05475) ;
#30095=CYLINDRICAL_SURFACE('',#33272,2.05475) ;
#30096=CYLINDRICAL_SURFACE('',#33274,2.05475) ;
#30097=CYLINDRICAL_SURFACE('',#33275,2.05475) ;
#30098=CYLINDRICAL_SURFACE('',#33277,1.66600000000001) ;
#30099=CYLINDRICAL_SURFACE('',#33279,1.66600000000001) ;
#30100=CYLINDRICAL_SURFACE('',#33281,1.66600000000001) ;
#30101=CYLINDRICAL_SURFACE('',#33283,1.66600000000001) ;
#30102=CYLINDRICAL_SURFACE('',#33285,1.66600000000001) ;
#30103=CYLINDRICAL_SURFACE('',#33287,1.66600000000001) ;
#30104=CYLINDRICAL_SURFACE('',#33289,1.66600000000001) ;
#30105=CYLINDRICAL_SURFACE('',#33290,1.66600000000001) ;
#30106=CYLINDRICAL_SURFACE('',#33291,2.05475) ;
#30107=CYLINDRICAL_SURFACE('',#33292,2.05475) ;
#30108=CYLINDRICAL_SURFACE('',#33293,1.666) ;
#30109=CYLINDRICAL_SURFACE('',#33294,1.666) ;
#30110=CYLINDRICAL_SURFACE('',#33295,2.05475) ;
#30111=CYLINDRICAL_SURFACE('',#33296,2.05475) ;
#30112=CYLINDRICAL_SURFACE('',#33297,1.66599999999998) ;
#30113=CYLINDRICAL_SURFACE('',#33298,1.66599999999999) ;
#30114=CYLINDRICAL_SURFACE('',#33299,1.66599999999999) ;
#30115=CYLINDRICAL_SURFACE('',#33300,1.66599999999999) ;
#30116=CYLINDRICAL_SURFACE('',#33301,2.05474999999993) ;
#30117=CYLINDRICAL_SURFACE('',#33302,2.05475000000001) ;
#30118=CYLINDRICAL_SURFACE('',#33303,2.05475000000001) ;
#30119=CYLINDRICAL_SURFACE('',#33304,2.05475) ;
#30120=CYLINDRICAL_SURFACE('',#33305,0.5) ;
#30121=CYLINDRICAL_SURFACE('',#33308,2.) ;
#30122=CYLINDRICAL_SURFACE('',#33311,2.) ;
#30123=CYLINDRICAL_SURFACE('',#33314,2.) ;
#30124=CYLINDRICAL_SURFACE('',#33317,2.) ;
#30125=CYLINDRICAL_SURFACE('',#33324,2.) ;
#30126=CYLINDRICAL_SURFACE('',#33327,1.) ;
#30127=CYLINDRICAL_SURFACE('',#33337,0.5) ;
#30128=CYLINDRICAL_SURFACE('',#33376,2.) ;
#30129=CYLINDRICAL_SURFACE('',#33378,2.) ;
#30130=CYLINDRICAL_SURFACE('',#33380,2.) ;
#30131=CYLINDRICAL_SURFACE('',#33382,0.5) ;
#30132=CYLINDRICAL_SURFACE('',#33396,1.) ;
#30133=CYLINDRICAL_SURFACE('',#33400,1.) ;
#30134=CYLINDRICAL_SURFACE('',#33406,1.) ;
#30135=CYLINDRICAL_SURFACE('',#33411,1.) ;
#30136=CYLINDRICAL_SURFACE('',#33414,4.) ;
#30137=CYLINDRICAL_SURFACE('',#33417,4.) ;
#30138=CYLINDRICAL_SURFACE('',#33420,1.) ;
#30139=CYLINDRICAL_SURFACE('',#33426,1.) ;
#30140=CYLINDRICAL_SURFACE('',#33431,1.) ;
#30141=CYLINDRICAL_SURFACE('',#33434,4.) ;
#30142=CYLINDRICAL_SURFACE('',#33437,4.) ;
#30143=CYLINDRICAL_SURFACE('',#33454,0.5) ;
#30144=CYLINDRICAL_SURFACE('',#33457,0.5) ;
#30145=CYLINDRICAL_SURFACE('',#33460,0.5) ;
#30146=CYLINDRICAL_SURFACE('',#33462,0.5) ;
#30147=CYLINDRICAL_SURFACE('',#33465,0.5) ;
#30148=CYLINDRICAL_SURFACE('',#33471,1.65) ;
#30149=CYLINDRICAL_SURFACE('',#33474,1.65) ;
#30150=CYLINDRICAL_SURFACE('',#33477,1.65) ;
#30151=CYLINDRICAL_SURFACE('',#33482,1.75) ;
#30152=CYLINDRICAL_SURFACE('',#33488,2.) ;
#30153=CYLINDRICAL_SURFACE('',#33491,2.) ;
#30154=CYLINDRICAL_SURFACE('',#33494,2.) ;
#30155=CYLINDRICAL_SURFACE('',#33497,2.) ;
#30156=CYLINDRICAL_SURFACE('',#33500,2.) ;
#30157=CYLINDRICAL_SURFACE('',#33503,2.) ;
#30158=CYLINDRICAL_SURFACE('',#33510,3.25) ;
#30159=CYLINDRICAL_SURFACE('',#33512,2.) ;
#30160=CYLINDRICAL_SURFACE('',#33513,2.) ;
#30161=CYLINDRICAL_SURFACE('',#33514,2.) ;
#30162=CYLINDRICAL_SURFACE('',#33516,2.) ;
#30163=CYLINDRICAL_SURFACE('',#33539,2.) ;
#30164=CYLINDRICAL_SURFACE('',#33541,2.) ;
#30165=CYLINDRICAL_SURFACE('',#33545,2.) ;
#30166=CYLINDRICAL_SURFACE('',#33547,3.25) ;
#30167=CYLINDRICAL_SURFACE('',#33552,3.25) ;
#30168=CYLINDRICAL_SURFACE('',#33567,1.75) ;
#30169=CYLINDRICAL_SURFACE('',#33572,1.75) ;
#30170=CYLINDRICAL_SURFACE('',#33577,1.75) ;
#30171=CYLINDRICAL_SURFACE('',#33582,1.75) ;
#30172=CYLINDRICAL_SURFACE('',#33600,2.) ;
#30173=CYLINDRICAL_SURFACE('',#33601,2.) ;
#30174=CYLINDRICAL_SURFACE('',#33617,3.25) ;
#30175=CYLINDRICAL_SURFACE('',#33621,2.) ;
#30176=CYLINDRICAL_SURFACE('',#33624,2.) ;
#30177=CYLINDRICAL_SURFACE('',#33627,3.25) ;
#30178=CYLINDRICAL_SURFACE('',#33630,3.25) ;
#30179=CYLINDRICAL_SURFACE('',#33632,1.65) ;
#30180=CYLINDRICAL_SURFACE('',#33640,0.125) ;
#30181=CYLINDRICAL_SURFACE('',#33642,0.125) ;
#30182=CYLINDRICAL_SURFACE('',#33644,0.125) ;
#30183=CYLINDRICAL_SURFACE('',#33647,0.125) ;
#30184=CYLINDRICAL_SURFACE('',#33649,0.125) ;
#30185=CYLINDRICAL_SURFACE('',#33652,0.125) ;
#30186=CYLINDRICAL_SURFACE('',#33654,0.125) ;
#30187=CYLINDRICAL_SURFACE('',#33658,0.125) ;
#30188=CYLINDRICAL_SURFACE('',#33669,2.) ;
#30189=CYLINDRICAL_SURFACE('',#33673,2.) ;
#30190=CYLINDRICAL_SURFACE('',#33674,2.) ;
#30191=CYLINDRICAL_SURFACE('',#33676,2.) ;
#30192=CYLINDRICAL_SURFACE('',#33682,2.) ;
#30193=CYLINDRICAL_SURFACE('',#33687,2.) ;
#30194=CYLINDRICAL_SURFACE('',#33690,2.) ;
#30958=ADVANCED_FACE('',(#2479),#30056,.F.) ;
#30959=ADVANCED_FACE('',(#2480),#30057,.F.) ;
#30960=ADVANCED_FACE('',(#2481),#30058,.F.) ;
#30961=ADVANCED_FACE('',(#2482),#30059,.F.) ;
#30962=ADVANCED_FACE('',(#2483),#30060,.F.) ;
#30963=ADVANCED_FACE('',(#2484),#30061,.F.) ;
#30964=ADVANCED_FACE('',(#2485),#30062,.F.) ;
#30965=ADVANCED_FACE('',(#2486),#30063,.F.) ;
#30966=ADVANCED_FACE('',(#2487),#30064,.F.) ;
#30967=ADVANCED_FACE('',(#2488),#30065,.F.) ;
#30968=ADVANCED_FACE('',(#2489),#30066,.F.) ;
#30969=ADVANCED_FACE('',(#2490),#30067,.F.) ;
#30970=ADVANCED_FACE('',(#2491),#30068,.F.) ;
#30971=ADVANCED_FACE('',(#2492),#30069,.F.) ;
#30972=ADVANCED_FACE('',(#2493),#30070,.F.) ;
#30973=ADVANCED_FACE('',(#2494),#30071,.F.) ;
#30974=ADVANCED_FACE('',(#2495),#30072,.F.) ;
#30975=ADVANCED_FACE('',(#2496),#30073,.F.) ;
#30976=ADVANCED_FACE('',(#2497),#30074,.F.) ;
#30977=ADVANCED_FACE('',(#2498),#30075,.F.) ;
#30978=ADVANCED_FACE('',(#2499),#30076,.F.) ;
#30979=ADVANCED_FACE('',(#2500),#30077,.F.) ;
#30980=ADVANCED_FACE('',(#2501),#30078,.F.) ;
#30981=ADVANCED_FACE('',(#2502),#30079,.F.) ;
#30982=ADVANCED_FACE('',(#2503),#30080,.F.) ;
#30983=ADVANCED_FACE('',(#2504),#30081,.F.) ;
#30984=ADVANCED_FACE('',(#2505),#30082,.F.) ;
#30985=ADVANCED_FACE('',(#2506),#30083,.F.) ;
#30986=ADVANCED_FACE('',(#2507),#30084,.F.) ;
#30987=ADVANCED_FACE('',(#2508),#30085,.F.) ;
#30988=ADVANCED_FACE('',(#2509),#30086,.F.) ;
#30989=ADVANCED_FACE('',(#2510),#30087,.F.) ;
#30990=ADVANCED_FACE('',(#2511),#30088,.F.) ;
#30991=ADVANCED_FACE('',(#2512),#30089,.F.) ;
#30992=ADVANCED_FACE('',(#2513),#30090,.F.) ;
#30993=ADVANCED_FACE('',(#2514),#30091,.F.) ;
#30994=ADVANCED_FACE('',(#2515),#30092,.F.) ;
#30995=ADVANCED_FACE('',(#2516),#30093,.F.) ;
#30996=ADVANCED_FACE('',(#2517),#30094,.F.) ;
#30997=ADVANCED_FACE('',(#2518),#30095,.F.) ;
#30998=ADVANCED_FACE('',(#2519),#30096,.F.) ;
#30999=ADVANCED_FACE('',(#2520),#30097,.F.) ;
#31000=ADVANCED_FACE('',(#2521),#30098,.F.) ;
#31001=ADVANCED_FACE('',(#2522),#30099,.F.) ;
#31002=ADVANCED_FACE('',(#2523),#30100,.F.) ;
#31003=ADVANCED_FACE('',(#2524),#30101,.F.) ;
#31004=ADVANCED_FACE('',(#2525),#30102,.F.) ;
#31005=ADVANCED_FACE('',(#2526),#30103,.F.) ;
#31006=ADVANCED_FACE('',(#2527),#30104,.F.) ;
#31007=ADVANCED_FACE('',(#2528),#30105,.F.) ;
#31008=ADVANCED_FACE('',(#2529),#30106,.F.) ;
#31009=ADVANCED_FACE('',(#2530),#30107,.F.) ;
#31010=ADVANCED_FACE('',(#2531),#30108,.F.) ;
#31011=ADVANCED_FACE('',(#2532),#30109,.F.) ;
#31012=ADVANCED_FACE('',(#2533),#30110,.F.) ;
#31013=ADVANCED_FACE('',(#2534),#30111,.F.) ;
#31014=ADVANCED_FACE('',(#2535),#30112,.F.) ;
#31015=ADVANCED_FACE('',(#2536),#30113,.F.) ;
#31016=ADVANCED_FACE('',(#2537),#30114,.F.) ;
#31017=ADVANCED_FACE('',(#2538),#30115,.F.) ;
#31018=ADVANCED_FACE('',(#2539),#30116,.F.) ;
#31019=ADVANCED_FACE('',(#2540),#30117,.F.) ;
#31020=ADVANCED_FACE('',(#2541),#30118,.F.) ;
#31021=ADVANCED_FACE('',(#2542),#30119,.F.) ;
#31022=ADVANCED_FACE('',(#2543),#30120,.F.) ;
#31023=ADVANCED_FACE('',(#2544),#30121,.T.) ;
#31024=ADVANCED_FACE('',(#2545),#30122,.T.) ;
#31025=ADVANCED_FACE('',(#2546),#30123,.T.) ;
#31026=ADVANCED_FACE('',(#2547),#30124,.T.) ;
#31027=ADVANCED_FACE('',(#2548),#1779,.T.) ;
#31028=ADVANCED_FACE('',(#2549),#30125,.T.) ;
#31029=ADVANCED_FACE('',(#2550),#30126,.F.) ;
#31030=ADVANCED_FACE('',(#2551,#1051,#1052,#1053,#1054,#1055,#1056,#1057,
#1058),#1780,.T.) ;
#31031=ADVANCED_FACE('',(#2552),#30127,.F.) ;
#31032=ADVANCED_FACE('',(#2553,#1059,#1060,#1061,#1062,#1063,#1064,#1065,
#1066,#1067,#1068),#1781,.T.) ;
#31033=ADVANCED_FACE('',(#2554,#1069,#1070,#1071,#1072,#1073,#1074,#1075,
#1076),#1782,.F.) ;
#31034=ADVANCED_FACE('',(#2555,#1077,#1078,#1079,#1080,#1081,#1082,#1083,
#1084,#1085,#1086),#1783,.F.) ;
#31035=ADVANCED_FACE('',(#2556),#1784,.T.) ;
#31036=ADVANCED_FACE('',(#2557),#1785,.F.) ;
#31037=ADVANCED_FACE('',(#2558),#30128,.T.) ;
#31038=ADVANCED_FACE('',(#2559),#30129,.T.) ;
#31039=ADVANCED_FACE('',(#2560),#30130,.T.) ;
#31040=ADVANCED_FACE('',(#2561),#30131,.F.) ;
#31041=ADVANCED_FACE('',(#2562),#1786,.F.) ;
#31042=ADVANCED_FACE('',(#2563),#1787,.F.) ;
#31043=ADVANCED_FACE('',(#2564),#1788,.F.) ;
#31044=ADVANCED_FACE('',(#2565),#905,.T.) ;
#31045=ADVANCED_FACE('',(#2566),#1789,.T.) ;
#31046=ADVANCED_FACE('',(#2567),#1790,.F.) ;
#31047=ADVANCED_FACE('',(#2568),#1791,.T.) ;
#31048=ADVANCED_FACE('',(#2569),#1792,.T.) ;
#31049=ADVANCED_FACE('',(#2570),#1793,.T.) ;
#31050=ADVANCED_FACE('',(#2571),#1794,.T.) ;
#31051=ADVANCED_FACE('',(#2572),#1795,.T.) ;
#31052=ADVANCED_FACE('',(#2573),#30132,.F.) ;
#31053=ADVANCED_FACE('',(#2574),#1796,.T.) ;
#31054=ADVANCED_FACE('',(#2575),#30133,.F.) ;
#31055=ADVANCED_FACE('',(#2576),#227,.F.) ;
#31056=ADVANCED_FACE('',(#2577),#30134,.F.) ;
#31057=ADVANCED_FACE('',(#2578),#228,.F.) ;
#31058=ADVANCED_FACE('',(#2579),#30135,.F.) ;
#31059=ADVANCED_FACE('',(#2580),#1797,.T.) ;
#31060=ADVANCED_FACE('',(#2581),#30136,.T.) ;
#31061=ADVANCED_FACE('',(#2582),#1798,.F.) ;
#31062=ADVANCED_FACE('',(#2583),#30137,.T.) ;
#31063=ADVANCED_FACE('',(#2584),#1799,.T.) ;
#31064=ADVANCED_FACE('',(#2585),#30138,.F.) ;
#31065=ADVANCED_FACE('',(#2586),#229,.F.) ;
#31066=ADVANCED_FACE('',(#2587),#30139,.F.) ;
#31067=ADVANCED_FACE('',(#2588),#230,.F.) ;
#31068=ADVANCED_FACE('',(#2589),#30140,.F.) ;
#31069=ADVANCED_FACE('',(#2590),#1800,.T.) ;
#31070=ADVANCED_FACE('',(#2591),#30141,.T.) ;
#31071=ADVANCED_FACE('',(#2592),#1801,.F.) ;
#31072=ADVANCED_FACE('',(#2593),#30142,.T.) ;
#31073=ADVANCED_FACE('',(#2594),#1802,.T.) ;
#31074=ADVANCED_FACE('',(#2595),#1803,.T.) ;
#31075=ADVANCED_FACE('',(#2596),#1804,.T.) ;
#31076=ADVANCED_FACE('',(#2597),#1805,.T.) ;
#31077=ADVANCED_FACE('',(#2598),#1806,.T.) ;
#31078=ADVANCED_FACE('',(#2599),#1807,.T.) ;
#31079=ADVANCED_FACE('',(#2600),#1808,.T.) ;
#31080=ADVANCED_FACE('',(#2601),#1809,.T.) ;
#31081=ADVANCED_FACE('',(#2602),#1810,.T.) ;
#31082=ADVANCED_FACE('',(#2603),#1811,.T.) ;
#31083=ADVANCED_FACE('',(#2604),#1812,.T.) ;
#31084=ADVANCED_FACE('',(#2605),#1813,.T.) ;
#31085=ADVANCED_FACE('',(#2606),#1814,.T.) ;
#31086=ADVANCED_FACE('',(#2607),#1815,.F.) ;
#31087=ADVANCED_FACE('',(#2608),#1816,.F.) ;
#31088=ADVANCED_FACE('',(#2609),#30143,.F.) ;
#31089=ADVANCED_FACE('',(#2610),#30144,.F.) ;
#31090=ADVANCED_FACE('',(#2611),#30145,.F.) ;
#31091=ADVANCED_FACE('',(#2612),#30146,.F.) ;
#31092=ADVANCED_FACE('',(#2613),#30147,.F.) ;
#31093=ADVANCED_FACE('',(#2614),#1817,.F.) ;
#31094=ADVANCED_FACE('',(#2615),#883,.F.) ;
#31095=ADVANCED_FACE('',(#2616),#30148,.F.) ;
#31096=ADVANCED_FACE('',(#2617),#884,.F.) ;
#31097=ADVANCED_FACE('',(#2618),#30149,.F.) ;
#31098=ADVANCED_FACE('',(#2619),#885,.F.) ;
#31099=ADVANCED_FACE('',(#2620),#30150,.F.) ;
#31100=ADVANCED_FACE('',(#2621),#1818,.F.) ;
#31101=ADVANCED_FACE('',(#2622),#1819,.F.) ;
#31102=ADVANCED_FACE('',(#2623),#30151,.F.) ;
#31103=ADVANCED_FACE('',(#2624),#886,.F.) ;
#31104=ADVANCED_FACE('',(#2625),#30152,.F.) ;
#31105=ADVANCED_FACE('',(#2626),#30153,.F.) ;
#31106=ADVANCED_FACE('',(#2627),#30154,.F.) ;
#31107=ADVANCED_FACE('',(#2628),#30155,.F.) ;
#31108=ADVANCED_FACE('',(#2629),#30156,.F.) ;
#31109=ADVANCED_FACE('',(#2630),#30157,.F.) ;
#31110=ADVANCED_FACE('',(#2631),#231,.T.) ;
#31111=ADVANCED_FACE('',(#2632),#30158,.T.) ;
#31112=ADVANCED_FACE('',(#2633),#30159,.F.) ;
#31113=ADVANCED_FACE('',(#2634),#30160,.F.) ;
#31114=ADVANCED_FACE('',(#2635),#30161,.F.) ;
#31115=ADVANCED_FACE('',(#2636),#1820,.F.) ;
#31116=ADVANCED_FACE('',(#2637),#30162,.F.) ;
#31117=ADVANCED_FACE('',(#2638),#1821,.F.) ;
#31118=ADVANCED_FACE('',(#2639),#1822,.F.) ;
#31119=ADVANCED_FACE('',(#2640),#1823,.F.) ;
#31120=ADVANCED_FACE('',(#2641),#1824,.F.) ;
#31121=ADVANCED_FACE('',(#2642),#1825,.F.) ;
#31122=ADVANCED_FACE('',(#2643),#1826,.F.) ;
#31123=ADVANCED_FACE('',(#2644),#1827,.F.) ;
#31124=ADVANCED_FACE('',(#2645),#1828,.F.) ;
#31125=ADVANCED_FACE('',(#2646),#1829,.F.) ;
#31126=ADVANCED_FACE('',(#2647),#1830,.F.) ;
#31127=ADVANCED_FACE('',(#2648),#1831,.F.) ;
#31128=ADVANCED_FACE('',(#2649),#1832,.F.) ;
#31129=ADVANCED_FACE('',(#2650),#1833,.F.) ;
#31130=ADVANCED_FACE('',(#2651),#1834,.F.) ;
#31131=ADVANCED_FACE('',(#2652),#1835,.F.) ;
#31132=ADVANCED_FACE('',(#2653),#1836,.F.) ;
#31133=ADVANCED_FACE('',(#2654),#1837,.F.) ;
#31134=ADVANCED_FACE('',(#2655),#1838,.F.) ;
#31135=ADVANCED_FACE('',(#2656),#1839,.T.) ;
#31136=ADVANCED_FACE('',(#2657),#30163,.T.) ;
#31137=ADVANCED_FACE('',(#2658),#30164,.T.) ;
#31138=ADVANCED_FACE('',(#2659),#1840,.T.) ;
#31139=ADVANCED_FACE('',(#2660),#30165,.T.) ;
#31140=ADVANCED_FACE('',(#2661),#30166,.T.) ;
#31141=ADVANCED_FACE('',(#2662),#232,.T.) ;
#31142=ADVANCED_FACE('',(#2663),#30167,.T.) ;
#31143=ADVANCED_FACE('',(#2664),#1841,.F.) ;
#31144=ADVANCED_FACE('',(#2665),#1842,.F.) ;
#31145=ADVANCED_FACE('',(#2666),#1843,.F.) ;
#31146=ADVANCED_FACE('',(#2667),#1844,.F.) ;
#31147=ADVANCED_FACE('',(#2668,#1087,#1088,#1089,#1090),#1845,.F.) ;
#31148=ADVANCED_FACE('',(#2669),#1846,.T.) ;
#31149=ADVANCED_FACE('',(#2670),#30168,.F.) ;
#31150=ADVANCED_FACE('',(#2671),#887,.F.) ;
#31151=ADVANCED_FACE('',(#2672),#30169,.F.) ;
#31152=ADVANCED_FACE('',(#2673),#888,.F.) ;
#31153=ADVANCED_FACE('',(#2674),#30170,.F.) ;
#31154=ADVANCED_FACE('',(#2675),#889,.F.) ;
#31155=ADVANCED_FACE('',(#2676),#30171,.F.) ;
#31156=ADVANCED_FACE('',(#2677),#890,.F.) ;
#31157=ADVANCED_FACE('',(#2678),#1847,.F.) ;
#31158=ADVANCED_FACE('',(#2679),#1848,.F.) ;
#31159=ADVANCED_FACE('',(#2680),#1849,.F.) ;
#31160=ADVANCED_FACE('',(#2681),#1850,.T.) ;
#31161=ADVANCED_FACE('',(#2682),#1851,.F.) ;
#31162=ADVANCED_FACE('',(#2683),#1852,.F.) ;
#31163=ADVANCED_FACE('',(#2684),#1853,.F.) ;
#31164=ADVANCED_FACE('',(#2685),#1854,.F.) ;
#31165=ADVANCED_FACE('',(#2686),#1855,.F.) ;
#31166=ADVANCED_FACE('',(#2687),#1856,.F.) ;
#31167=ADVANCED_FACE('',(#2688),#30172,.F.) ;
#31168=ADVANCED_FACE('',(#2689),#30173,.F.) ;
#31169=ADVANCED_FACE('',(#2690),#1857,.F.) ;
#31170=ADVANCED_FACE('',(#2691),#1858,.F.) ;
#31171=ADVANCED_FACE('',(#2692),#1859,.F.) ;
#31172=ADVANCED_FACE('',(#2693),#1860,.F.) ;
#31173=ADVANCED_FACE('',(#2694),#1861,.F.) ;
#31174=ADVANCED_FACE('',(#2695),#1862,.F.) ;
#31175=ADVANCED_FACE('',(#2696),#1863,.F.) ;
#31176=ADVANCED_FACE('',(#2697),#1864,.F.) ;
#31177=ADVANCED_FACE('',(#2698),#1865,.F.) ;
#31178=ADVANCED_FACE('',(#2699),#1866,.F.) ;
#31179=ADVANCED_FACE('',(#2700),#233,.T.) ;
#31180=ADVANCED_FACE('',(#2701),#30174,.T.) ;
#31181=ADVANCED_FACE('',(#2702),#234,.T.) ;
#31182=ADVANCED_FACE('',(#2703),#30175,.T.) ;
#31183=ADVANCED_FACE('',(#2704),#1867,.T.) ;
#31184=ADVANCED_FACE('',(#2705),#30176,.T.) ;
#31185=ADVANCED_FACE('',(#2706),#1868,.F.) ;
#31186=ADVANCED_FACE('',(#2707),#30177,.T.) ;
#31187=ADVANCED_FACE('',(#2708),#30178,.T.) ;
#31188=ADVANCED_FACE('',(#2709,#1091),#1869,.F.) ;
#31189=ADVANCED_FACE('',(#2710),#30179,.F.) ;
#31190=ADVANCED_FACE('',(#2711),#891,.F.) ;
#31191=ADVANCED_FACE('',(#2712),#906,.F.) ;
#31192=ADVANCED_FACE('',(#2713),#907,.F.) ;
#31193=ADVANCED_FACE('',(#2714),#908,.F.) ;
#31194=ADVANCED_FACE('',(#2715),#909,.F.) ;
#31195=ADVANCED_FACE('',(#2716),#910,.F.) ;
#31196=ADVANCED_FACE('',(#2717),#911,.F.) ;
#31197=ADVANCED_FACE('',(#2718),#912,.F.) ;
#31198=ADVANCED_FACE('',(#2719),#913,.F.) ;
#31199=ADVANCED_FACE('',(#2720),#1870,.F.) ;
#31200=ADVANCED_FACE('',(#2721),#1871,.F.) ;
#31201=ADVANCED_FACE('',(#2722),#1872,.F.) ;
#31202=ADVANCED_FACE('',(#2723),#1873,.F.) ;
#31203=ADVANCED_FACE('',(#2724),#30180,.F.) ;
#31204=ADVANCED_FACE('',(#2725),#30181,.F.) ;
#31205=ADVANCED_FACE('',(#2726),#30182,.T.) ;
#31206=ADVANCED_FACE('',(#2727),#30183,.F.) ;
#31207=ADVANCED_FACE('',(#2728),#30184,.T.) ;
#31208=ADVANCED_FACE('',(#2729),#30185,.F.) ;
#31209=ADVANCED_FACE('',(#2730),#30186,.T.) ;
#31210=ADVANCED_FACE('',(#2731),#235,.T.) ;
#31211=ADVANCED_FACE('',(#2732),#30187,.T.) ;
#31212=ADVANCED_FACE('',(#2733),#236,.T.) ;
#31213=ADVANCED_FACE('',(#2734),#237,.T.) ;
#31214=ADVANCED_FACE('',(#2735),#238,.T.) ;
#31215=ADVANCED_FACE('',(#2736),#1874,.T.) ;
#31216=ADVANCED_FACE('',(#2737),#1875,.F.) ;
#31217=ADVANCED_FACE('',(#2738),#30188,.T.) ;
#31218=ADVANCED_FACE('',(#2739),#1876,.F.) ;
#31219=ADVANCED_FACE('',(#2740),#30189,.T.) ;
#31220=ADVANCED_FACE('',(#2741),#30190,.T.) ;
#31221=ADVANCED_FACE('',(#2742),#30191,.T.) ;
#31222=ADVANCED_FACE('',(#2743,#1092,#1093,#1094,#1095),#1877,.T.) ;
#31223=ADVANCED_FACE('',(#2744),#740,.F.) ;
#31224=ADVANCED_FACE('',(#2745),#30192,.T.) ;
#31225=ADVANCED_FACE('',(#2746),#741,.F.) ;
#31226=ADVANCED_FACE('',(#2747,#1096),#1878,.T.) ;
#31227=ADVANCED_FACE('',(#2748),#30193,.T.) ;
#31228=ADVANCED_FACE('',(#2749),#742,.F.) ;
#31229=ADVANCED_FACE('',(#2750),#30194,.T.) ;
#31230=ADVANCED_FACE('',(#2751),#743,.F.) ;
#31231=ADVANCED_FACE('',(#2752),#914,.F.) ;
#31232=ADVANCED_FACE('',(#2753),#915,.F.) ;
#31233=ADVANCED_FACE('',(#2754),#916,.F.) ;
#31234=ADVANCED_FACE('',(#2755),#917,.F.) ;
#31235=ADVANCED_FACE('',(#2756),#918,.F.) ;
#31236=ADVANCED_FACE('',(#2757),#919,.F.) ;
#31237=ADVANCED_FACE('',(#2758,#1097,#1098,#1099,#1100,#1101,#1102,#1103,
#1104,#1105),#1879,.F.) ;
#31238=ADVANCED_FACE('',(#2759),#920,.F.) ;
#31239=ADVANCED_FACE('',(#2760),#921,.F.) ;
#31240=ADVANCED_FACE('',(#2761),#1880,.T.) ;
#31241=ADVANCED_FACE('',(#2762),#1881,.T.) ;
#31242=ADVANCED_FACE('',(#2763),#1882,.T.) ;
#31243=ADVANCED_FACE('',(#2764),#1883,.T.) ;
#31244=ADVANCED_FACE('',(#2765),#1884,.T.) ;
#31245=ADVANCED_FACE('',(#2766),#1885,.T.) ;
#31246=ADVANCED_FACE('',(#2767),#1886,.T.) ;
#31247=ADVANCED_FACE('',(#2768),#1887,.T.) ;
#31248=ADVANCED_FACE('',(#2769),#1888,.T.) ;
#31249=ADVANCED_FACE('',(#2770),#1889,.T.) ;
#31250=ADVANCED_FACE('',(#2771),#1890,.T.) ;
#31251=ADVANCED_FACE('',(#2772),#1891,.T.) ;
#31252=ADVANCED_FACE('',(#2773,#1106,#1107,#1108,#1109,#1110,#1111,#1112,
#1113,#1114),#1892,.T.) ;
#31253=ADVANCED_FACE('',(#2774),#1893,.T.) ;
#31254=ADVANCED_FACE('',(#2775),#1894,.T.) ;
#31255=ADVANCED_FACE('',(#2776),#1895,.T.) ;
#31256=ADVANCED_FACE('',(#2777),#1896,.T.) ;
#31257=ADVANCED_FACE('',(#2778),#1897,.T.) ;
#31258=ADVANCED_FACE('',(#2779),#1898,.T.) ;
#32640=CLOSED_SHELL('',(#30958,#30959,#30960,#30961,#30962,#30963,#30964,
#30965,#30966,#30967,#30968,#30969,#30970,#30971,#30972,#30973,#30974,#30975,
#30976,#30977,#30978,#30979,#30980,#30981,#30982,#30983,#30984,#30985,#30986,
#30987,#30988,#30989,#30990,#30991,#30992,#30993,#30994,#30995,#30996,#30997,
#30998,#30999,#31000,#31001,#31002,#31003,#31004,#31005,#31006,#31007,#31008,
#31009,#31010,#31011,#31012,#31013,#31014,#31015,#31016,#31017,#31018,#31019,
#31020,#31021,#31022,#31023,#31024,#31025,#31026,#31027,#31028,#31029,#31030,
#31031,#31032,#31033,#31034,#31035,#31036,#31037,#31038,#31039,#31040,#31041,
#31042,#31043,#31044,#31045,#31046,#31047,#31048,#31049,#31050,#31051,#31052,
#31053,#31054,#31055,#31056,#31057,#31058,#31059,#31060,#31061,#31062,#31063,
#31064,#31065,#31066,#31067,#31068,#31069,#31070,#31071,#31072,#31073,#31074,
#31075,#31076,#31077,#31078,#31079,#31080,#31081,#31082,#31083,#31084,#31085,
#31086,#31087,#31088,#31089,#31090,#31091,#31092,#31093,#31094,#31095,#31096,
#31097,#31098,#31099,#31100,#31101,#31102,#31103,#31104,#31105,#31106,#31107,
#31108,#31109,#31110,#31111,#31112,#31113,#31114,#31115,#31116,#31117,#31118,
#31119,#31120,#31121,#31122,#31123,#31124,#31125,#31126,#31127,#31128,#31129,
#31130,#31131,#31132,#31133,#31134,#31135,#31136,#31137,#31138,#31139,#31140,
#31141,#31142,#31143,#31144,#31145,#31146,#31147,#31148,#31149,#31150,#31151,
#31152,#31153,#31154,#31155,#31156,#31157,#31158,#31159,#31160,#31161,#31162,
#31163,#31164,#31165,#31166,#31167,#31168,#31169,#31170,#31171,#31172,#31173,
#31174,#31175,#31176,#31177,#31178,#31179,#31180,#31181,#31182,#31183,#31184,
#31185,#31186,#31187,#31188,#31189,#31190,#31191,#31192,#31193,#31194,#31195,
#31196,#31197,#31198,#31199,#31200,#31201,#31202,#31203,#31204,#31205,#31206,
#31207,#31208,#31209,#31210,#31211,#31212,#31213,#31214,#31215,#31216,#31217,
#31218,#31219,#31220,#31221,#31222,#31223,#31224,#31225,#31226,#31227,#31228,
#31229,#31230,#31231,#31232,#31233,#31234,#31235,#31236,#31237,#31238,#31239,
#31240,#31241,#31242,#31243,#31244,#31245,#31246,#31247,#31248,#31249,#31250,
#31251,#31252,#31253,#31254,#31255,#31256,#31257,#31258)) ;
#33060=AXIS2_PLACEMENT_3D('',#47173,#37309,#37310) ;
#33201=AXIS2_PLACEMENT_3D('',#50225,#37653,#37654) ;
#33202=AXIS2_PLACEMENT_3D('',#50259,#37656,#37657) ;
#33203=AXIS2_PLACEMENT_3D('',#50296,#37658,#37659) ;
#33204=AXIS2_PLACEMENT_3D('',#50535,#37661,#37662) ;
#33205=AXIS2_PLACEMENT_3D('',#50673,#37664,#37665) ;
#33206=AXIS2_PLACEMENT_3D('',#50748,#37666,#37667) ;
#33207=AXIS2_PLACEMENT_3D('',#50760,#37669,#37670) ;
#33208=AXIS2_PLACEMENT_3D('',#50779,#37671,#37672) ;
#33209=AXIS2_PLACEMENT_3D('',#51021,#37674,#37675) ;
#33210=AXIS2_PLACEMENT_3D('',#51184,#37677,#37678) ;
#33211=AXIS2_PLACEMENT_3D('',#51286,#37679,#37680) ;
#33212=AXIS2_PLACEMENT_3D('',#51320,#37682,#37683) ;
#33213=AXIS2_PLACEMENT_3D('',#51357,#37684,#37685) ;
#33214=AXIS2_PLACEMENT_3D('',#51598,#37687,#37688) ;
#33215=AXIS2_PLACEMENT_3D('',#51736,#37690,#37691) ;
#33216=AXIS2_PLACEMENT_3D('',#51822,#37692,#37693) ;
#33217=AXIS2_PLACEMENT_3D('',#51854,#37695,#37696) ;
#33218=AXIS2_PLACEMENT_3D('',#51891,#37697,#37698) ;
#33219=AXIS2_PLACEMENT_3D('',#52130,#37700,#37701) ;
#33220=AXIS2_PLACEMENT_3D('',#52268,#37703,#37704) ;
#33221=AXIS2_PLACEMENT_3D('',#52345,#37705,#37706) ;
#33222=AXIS2_PLACEMENT_3D('',#52350,#37708,#37709) ;
#33223=AXIS2_PLACEMENT_3D('',#52394,#37710,#37711) ;
#33224=AXIS2_PLACEMENT_3D('',#52598,#37713,#37714) ;
#33225=AXIS2_PLACEMENT_3D('',#52703,#37715,#37716) ;
#33226=AXIS2_PLACEMENT_3D('',#52850,#37718,#37719) ;
#33227=AXIS2_PLACEMENT_3D('',#53059,#37720,#37721) ;
#33228=AXIS2_PLACEMENT_3D('',#53064,#37723,#37724) ;
#33229=AXIS2_PLACEMENT_3D('',#53108,#37725,#37726) ;
#33230=AXIS2_PLACEMENT_3D('',#53312,#37728,#37729) ;
#33231=AXIS2_PLACEMENT_3D('',#53417,#37730,#37731) ;
#33232=AXIS2_PLACEMENT_3D('',#53564,#37733,#37734) ;
#33233=AXIS2_PLACEMENT_3D('',#53773,#37735,#37736) ;
#33234=AXIS2_PLACEMENT_3D('',#53778,#37738,#37739) ;
#33235=AXIS2_PLACEMENT_3D('',#53822,#37740,#37741) ;
#33236=AXIS2_PLACEMENT_3D('',#54026,#37743,#37744) ;
#33237=AXIS2_PLACEMENT_3D('',#54131,#37745,#37746) ;
#33238=AXIS2_PLACEMENT_3D('',#54278,#37748,#37749) ;
#33239=AXIS2_PLACEMENT_3D('',#54487,#37750,#37751) ;
#33240=AXIS2_PLACEMENT_3D('',#54492,#37753,#37754) ;
#33241=AXIS2_PLACEMENT_3D('',#54536,#37755,#37756) ;
#33242=AXIS2_PLACEMENT_3D('',#54740,#37758,#37759) ;
#33243=AXIS2_PLACEMENT_3D('',#54845,#37760,#37761) ;
#33244=AXIS2_PLACEMENT_3D('',#54992,#37763,#37764) ;
#33245=AXIS2_PLACEMENT_3D('',#55201,#37765,#37766) ;
#33246=AXIS2_PLACEMENT_3D('',#55235,#37768,#37769) ;
#33247=AXIS2_PLACEMENT_3D('',#55272,#37770,#37771) ;
#33248=AXIS2_PLACEMENT_3D('',#55507,#37773,#37774) ;
#33249=AXIS2_PLACEMENT_3D('',#55645,#37776,#37777) ;
#33250=AXIS2_PLACEMENT_3D('',#55720,#37778,#37779) ;
#33251=AXIS2_PLACEMENT_3D('',#55754,#37781,#37782) ;
#33252=AXIS2_PLACEMENT_3D('',#55791,#37783,#37784) ;
#33253=AXIS2_PLACEMENT_3D('',#56032,#37786,#37787) ;
#33254=AXIS2_PLACEMENT_3D('',#56170,#37789,#37790) ;
#33255=AXIS2_PLACEMENT_3D('',#56256,#37791,#37792) ;
#33256=AXIS2_PLACEMENT_3D('',#56261,#37794,#37795) ;
#33257=AXIS2_PLACEMENT_3D('',#56305,#37796,#37797) ;
#33258=AXIS2_PLACEMENT_3D('',#56509,#37799,#37800) ;
#33259=AXIS2_PLACEMENT_3D('',#56614,#37801,#37802) ;
#33260=AXIS2_PLACEMENT_3D('',#56761,#37804,#37805) ;
#33261=AXIS2_PLACEMENT_3D('',#56970,#37806,#37807) ;
#33262=AXIS2_PLACEMENT_3D('',#56975,#37809,#37810) ;
#33263=AXIS2_PLACEMENT_3D('',#57019,#37811,#37812) ;
#33264=AXIS2_PLACEMENT_3D('',#57223,#37814,#37815) ;
#33265=AXIS2_PLACEMENT_3D('',#57326,#37816,#37817) ;
#33266=AXIS2_PLACEMENT_3D('',#57473,#37819,#37820) ;
#33267=AXIS2_PLACEMENT_3D('',#57682,#37821,#37822) ;
#33268=AXIS2_PLACEMENT_3D('',#57714,#37824,#37825) ;
#33269=AXIS2_PLACEMENT_3D('',#57751,#37826,#37827) ;
#33270=AXIS2_PLACEMENT_3D('',#57994,#37829,#37830) ;
#33271=AXIS2_PLACEMENT_3D('',#58132,#37832,#37833) ;
#33272=AXIS2_PLACEMENT_3D('',#58211,#37834,#37835) ;
#33273=AXIS2_PLACEMENT_3D('',#58243,#37837,#37838) ;
#33274=AXIS2_PLACEMENT_3D('',#58280,#37839,#37840) ;
#33275=AXIS2_PLACEMENT_3D('',#58521,#37842,#37843) ;
#33276=AXIS2_PLACEMENT_3D('',#58659,#37845,#37846) ;
#33277=AXIS2_PLACEMENT_3D('',#58734,#37847,#37848) ;
#33278=AXIS2_PLACEMENT_3D('',#58739,#37850,#37851) ;
#33279=AXIS2_PLACEMENT_3D('',#58783,#37852,#37853) ;
#33280=AXIS2_PLACEMENT_3D('',#58987,#37855,#37856) ;
#33281=AXIS2_PLACEMENT_3D('',#59092,#37857,#37858) ;
#33282=AXIS2_PLACEMENT_3D('',#59239,#37860,#37861) ;
#33283=AXIS2_PLACEMENT_3D('',#59448,#37862,#37863) ;
#33284=AXIS2_PLACEMENT_3D('',#59453,#37865,#37866) ;
#33285=AXIS2_PLACEMENT_3D('',#59497,#37867,#37868) ;
#33286=AXIS2_PLACEMENT_3D('',#59701,#37870,#37871) ;
#33287=AXIS2_PLACEMENT_3D('',#59806,#37872,#37873) ;
#33288=AXIS2_PLACEMENT_3D('',#59953,#37875,#37876) ;
#33289=AXIS2_PLACEMENT_3D('',#60162,#37877,#37878) ;
#33290=AXIS2_PLACEMENT_3D('',#60371,#37879,#37880) ;
#33291=AXIS2_PLACEMENT_3D('',#60584,#37881,#37882) ;
#33292=AXIS2_PLACEMENT_3D('',#60805,#37883,#37884) ;
#33293=AXIS2_PLACEMENT_3D('',#61032,#37885,#37886) ;
#33294=AXIS2_PLACEMENT_3D('',#61243,#37887,#37888) ;
#33295=AXIS2_PLACEMENT_3D('',#61454,#37889,#37890) ;
#33296=AXIS2_PLACEMENT_3D('',#61684,#37891,#37892) ;
#33297=AXIS2_PLACEMENT_3D('',#61911,#37893,#37894) ;
#33298=AXIS2_PLACEMENT_3D('',#62122,#37895,#37896) ;
#33299=AXIS2_PLACEMENT_3D('',#62331,#37897,#37898) ;
#33300=AXIS2_PLACEMENT_3D('',#62544,#37899,#37900) ;
#33301=AXIS2_PLACEMENT_3D('',#62755,#37901,#37902) ;
#33302=AXIS2_PLACEMENT_3D('',#62980,#37903,#37904) ;
#33303=AXIS2_PLACEMENT_3D('',#63206,#37905,#37906) ;
#33304=AXIS2_PLACEMENT_3D('',#63431,#37907,#37908) ;
#33305=AXIS2_PLACEMENT_3D('',#63656,#37909,#37910) ;
#33306=AXIS2_PLACEMENT_3D('',#63659,#37911,#37912) ;
#33307=AXIS2_PLACEMENT_3D('',#63663,#37914,#37915) ;
#33308=AXIS2_PLACEMENT_3D('',#63665,#37917,#37918) ;
#33309=AXIS2_PLACEMENT_3D('',#63668,#37919,#37920) ;
#33310=AXIS2_PLACEMENT_3D('',#63672,#37922,#37923) ;
#33311=AXIS2_PLACEMENT_3D('',#63674,#37925,#37926) ;
#33312=AXIS2_PLACEMENT_3D('',#63677,#37927,#37928) ;
#33313=AXIS2_PLACEMENT_3D('',#63681,#37930,#37931) ;
#33314=AXIS2_PLACEMENT_3D('',#63683,#37933,#37934) ;
#33315=AXIS2_PLACEMENT_3D('',#63686,#37935,#37936) ;
#33316=AXIS2_PLACEMENT_3D('',#63690,#37938,#37939) ;
#33317=AXIS2_PLACEMENT_3D('',#63692,#37941,#37942) ;
#33318=AXIS2_PLACEMENT_3D('',#63695,#37943,#37944) ;
#33319=AXIS2_PLACEMENT_3D('',#63699,#37946,#37947) ;
#33320=AXIS2_PLACEMENT_3D('',#63701,#37949,#37950) ;
#33321=AXIS2_PLACEMENT_3D('',#63705,#37952,#37953) ;
#33322=AXIS2_PLACEMENT_3D('',#63710,#37956,#37957) ;
#33323=AXIS2_PLACEMENT_3D('',#63714,#37959,#37960) ;
#33324=AXIS2_PLACEMENT_3D('',#63717,#37963,#37964) ;
#33325=AXIS2_PLACEMENT_3D('',#63720,#37965,#37966) ;
#33326=AXIS2_PLACEMENT_3D('',#63724,#37968,#37969) ;
#33327=AXIS2_PLACEMENT_3D('',#63726,#37971,#37972) ;
#33328=AXIS2_PLACEMENT_3D('',#63729,#37973,#37974) ;
#33329=AXIS2_PLACEMENT_3D('',#63733,#37976,#37977) ;
#33330=AXIS2_PLACEMENT_3D('',#63735,#37979,#37980) ;
#33331=AXIS2_PLACEMENT_3D('',#63742,#37984,#37985) ;
#33332=AXIS2_PLACEMENT_3D('',#63750,#37989,#37990) ;
#33333=AXIS2_PLACEMENT_3D('',#63774,#38002,#38003) ;
#33334=AXIS2_PLACEMENT_3D('',#63778,#38005,#38006) ;
#33335=AXIS2_PLACEMENT_3D('',#64139,#38012,#38013) ;
#33336=AXIS2_PLACEMENT_3D('',#64165,#38026,#38027) ;
#33337=AXIS2_PLACEMENT_3D('',#64166,#38028,#38029) ;
#33338=AXIS2_PLACEMENT_3D('',#64169,#38030,#38031) ;
#33339=AXIS2_PLACEMENT_3D('',#64173,#38033,#38034) ;
#33340=AXIS2_PLACEMENT_3D('',#64175,#38036,#38037) ;
#33341=AXIS2_PLACEMENT_3D('',#64185,#38043,#38044) ;
#33342=AXIS2_PLACEMENT_3D('',#64193,#38048,#38049) ;
#33343=AXIS2_PLACEMENT_3D('',#64201,#38053,#38054) ;
#33344=AXIS2_PLACEMENT_3D('',#64209,#38058,#38059) ;
#33345=AXIS2_PLACEMENT_3D('',#64212,#38061,#38062) ;
#33346=AXIS2_PLACEMENT_3D('',#64246,#38079,#38080) ;
#33347=AXIS2_PLACEMENT_3D('',#64601,#38082,#38083) ;
#33348=AXIS2_PLACEMENT_3D('',#64605,#38085,#38086) ;
#33349=AXIS2_PLACEMENT_3D('',#64609,#38088,#38089) ;
#33350=AXIS2_PLACEMENT_3D('',#64612,#38091,#38092) ;
#33351=AXIS2_PLACEMENT_3D('',#64627,#38099,#38100) ;
#33352=AXIS2_PLACEMENT_3D('',#64631,#38102,#38103) ;
#33353=AXIS2_PLACEMENT_3D('',#64633,#38105,#38106) ;
#33354=AXIS2_PLACEMENT_3D('',#64645,#38112,#38113) ;
#33355=AXIS2_PLACEMENT_3D('',#64653,#38117,#38118) ;
#33356=AXIS2_PLACEMENT_3D('',#64659,#38122,#38123) ;
#33357=AXIS2_PLACEMENT_3D('',#64686,#38136,#38137) ;
#33358=AXIS2_PLACEMENT_3D('',#64690,#38139,#38140) ;
#33359=AXIS2_PLACEMENT_3D('',#64697,#38144,#38145) ;
#33360=AXIS2_PLACEMENT_3D('',#65048,#38146,#38147) ;
#33361=AXIS2_PLACEMENT_3D('',#65054,#38150,#38151) ;
#33362=AXIS2_PLACEMENT_3D('',#65062,#38155,#38156) ;
#33363=AXIS2_PLACEMENT_3D('',#65070,#38160,#38161) ;
#33364=AXIS2_PLACEMENT_3D('',#65078,#38165,#38166) ;
#33365=AXIS2_PLACEMENT_3D('',#65091,#38173,#38174) ;
#33366=AXIS2_PLACEMENT_3D('',#65095,#38176,#38177) ;
#33367=AXIS2_PLACEMENT_3D('',#65099,#38179,#38180) ;
#33368=AXIS2_PLACEMENT_3D('',#65103,#38182,#38183) ;
#33369=AXIS2_PLACEMENT_3D('',#65457,#38185,#38186) ;
#33370=AXIS2_PLACEMENT_3D('',#65461,#38188,#38189) ;
#33371=AXIS2_PLACEMENT_3D('',#65500,#38209,#38210) ;
#33372=AXIS2_PLACEMENT_3D('',#65502,#38211,#38212) ;
#33373=AXIS2_PLACEMENT_3D('',#65503,#38213,#38214) ;
#33374=AXIS2_PLACEMENT_3D('',#65505,#38215,#38216) ;
#33375=AXIS2_PLACEMENT_3D('',#65511,#38221,#38222) ;
#33376=AXIS2_PLACEMENT_3D('',#65534,#38229,#38230) ;
#33377=AXIS2_PLACEMENT_3D('',#65536,#38231,#38232) ;
#33378=AXIS2_PLACEMENT_3D('',#65538,#38234,#38235) ;
#33379=AXIS2_PLACEMENT_3D('',#65541,#38237,#38238) ;
#33380=AXIS2_PLACEMENT_3D('',#65542,#38239,#38240) ;
#33381=AXIS2_PLACEMENT_3D('',#65544,#38241,#38242) ;
#33382=AXIS2_PLACEMENT_3D('',#65546,#38244,#38245) ;
#33383=AXIS2_PLACEMENT_3D('',#65548,#38246,#38247) ;
#33384=AXIS2_PLACEMENT_3D('',#65551,#38249,#38250) ;
#33385=AXIS2_PLACEMENT_3D('',#65552,#38251,#38252) ;
#33386=AXIS2_PLACEMENT_3D('',#65554,#38254,#38255) ;
#33387=AXIS2_PLACEMENT_3D('',#65560,#38259,#38260) ;
#33388=AXIS2_PLACEMENT_3D('',#65620,#38264,#38265) ;
#33389=AXIS2_PLACEMENT_3D('',#65624,#38268,#38269) ;
#33390=AXIS2_PLACEMENT_3D('',#65629,#38273,#38274) ;
#33391=AXIS2_PLACEMENT_3D('',#65633,#38277,#38278) ;
#33392=AXIS2_PLACEMENT_3D('',#65635,#38280,#38281) ;
#33393=AXIS2_PLACEMENT_3D('',#65636,#38282,#38283) ;
#33394=AXIS2_PLACEMENT_3D('',#65638,#38285,#38286) ;
#33395=AXIS2_PLACEMENT_3D('',#65643,#38290,#38291) ;
#33396=AXIS2_PLACEMENT_3D('',#65645,#38293,#38294) ;
#33397=AXIS2_PLACEMENT_3D('',#65647,#38295,#38296) ;
#33398=AXIS2_PLACEMENT_3D('',#65650,#38298,#38299) ;
#33399=AXIS2_PLACEMENT_3D('',#65651,#38300,#38301) ;
#33400=AXIS2_PLACEMENT_3D('',#65657,#38305,#38306) ;
#33401=AXIS2_PLACEMENT_3D('',#65659,#38307,#38308) ;
#33402=AXIS2_PLACEMENT_3D('',#65661,#38309,#38310) ;
#33403=AXIS2_PLACEMENT_3D('',#65663,#38312,#38313) ;
#33404=AXIS2_PLACEMENT_3D('',#65665,#38314,#38315) ;
#33405=AXIS2_PLACEMENT_3D('',#65666,#38316,#38317) ;
#33406=AXIS2_PLACEMENT_3D('',#65667,#38318,#38319) ;
#33407=AXIS2_PLACEMENT_3D('',#65669,#38320,#38321) ;
#33408=AXIS2_PLACEMENT_3D('',#65671,#38323,#38324) ;
#33409=AXIS2_PLACEMENT_3D('',#65673,#38325,#38326) ;
#33410=AXIS2_PLACEMENT_3D('',#65674,#38327,#38328) ;
#33411=AXIS2_PLACEMENT_3D('',#65675,#38329,#38330) ;
#33412=AXIS2_PLACEMENT_3D('',#65677,#38331,#38332) ;
#33413=AXIS2_PLACEMENT_3D('',#65679,#38334,#38335) ;
#33414=AXIS2_PLACEMENT_3D('',#65685,#38339,#38340) ;
#33415=AXIS2_PLACEMENT_3D('',#65688,#38342,#38343) ;
#33416=AXIS2_PLACEMENT_3D('',#65689,#38344,#38345) ;
#33417=AXIS2_PLACEMENT_3D('',#65693,#38348,#38349) ;
#33418=AXIS2_PLACEMENT_3D('',#65696,#38351,#38352) ;
#33419=AXIS2_PLACEMENT_3D('',#65697,#38353,#38354) ;
#33420=AXIS2_PLACEMENT_3D('',#65701,#38357,#38358) ;
#33421=AXIS2_PLACEMENT_3D('',#65703,#38359,#38360) ;
#33422=AXIS2_PLACEMENT_3D('',#65705,#38361,#38362) ;
#33423=AXIS2_PLACEMENT_3D('',#65707,#38364,#38365) ;
#33424=AXIS2_PLACEMENT_3D('',#65709,#38366,#38367) ;
#33425=AXIS2_PLACEMENT_3D('',#65710,#38368,#38369) ;
#33426=AXIS2_PLACEMENT_3D('',#65711,#38370,#38371) ;
#33427=AXIS2_PLACEMENT_3D('',#65713,#38372,#38373) ;
#33428=AXIS2_PLACEMENT_3D('',#65715,#38375,#38376) ;
#33429=AXIS2_PLACEMENT_3D('',#65717,#38377,#38378) ;
#33430=AXIS2_PLACEMENT_3D('',#65718,#38379,#38380) ;
#33431=AXIS2_PLACEMENT_3D('',#65719,#38381,#38382) ;
#33432=AXIS2_PLACEMENT_3D('',#65721,#38383,#38384) ;
#33433=AXIS2_PLACEMENT_3D('',#65723,#38386,#38387) ;
#33434=AXIS2_PLACEMENT_3D('',#65729,#38391,#38392) ;
#33435=AXIS2_PLACEMENT_3D('',#65732,#38394,#38395) ;
#33436=AXIS2_PLACEMENT_3D('',#65733,#38396,#38397) ;
#33437=AXIS2_PLACEMENT_3D('',#65737,#38400,#38401) ;
#33438=AXIS2_PLACEMENT_3D('',#65740,#38403,#38404) ;
#33439=AXIS2_PLACEMENT_3D('',#65741,#38405,#38406) ;
#33440=AXIS2_PLACEMENT_3D('',#65745,#38409,#38410) ;
#33441=AXIS2_PLACEMENT_3D('',#65754,#38415,#38416) ;
#33442=AXIS2_PLACEMENT_3D('',#65760,#38420,#38421) ;
#33443=AXIS2_PLACEMENT_3D('',#65766,#38425,#38426) ;
#33444=AXIS2_PLACEMENT_3D('',#65772,#38430,#38431) ;
#33445=AXIS2_PLACEMENT_3D('',#65778,#38435,#38436) ;
#33446=AXIS2_PLACEMENT_3D('',#65781,#38439,#38440) ;
#33447=AXIS2_PLACEMENT_3D('',#65790,#38445,#38446) ;
#33448=AXIS2_PLACEMENT_3D('',#65796,#38450,#38451) ;
#33449=AXIS2_PLACEMENT_3D('',#65802,#38455,#38456) ;
#33450=AXIS2_PLACEMENT_3D('',#65808,#38460,#38461) ;
#33451=AXIS2_PLACEMENT_3D('',#65814,#38465,#38466) ;
#33452=AXIS2_PLACEMENT_3D('',#65817,#38469,#38470) ;
#33453=AXIS2_PLACEMENT_3D('',#65818,#38471,#38472) ;
#33454=AXIS2_PLACEMENT_3D('',#65819,#38473,#38474) ;
#33455=AXIS2_PLACEMENT_3D('',#65821,#38475,#38476) ;
#33456=AXIS2_PLACEMENT_3D('',#65823,#38477,#38478) ;
#33457=AXIS2_PLACEMENT_3D('',#65825,#38480,#38481) ;
#33458=AXIS2_PLACEMENT_3D('',#65827,#38482,#38483) ;
#33459=AXIS2_PLACEMENT_3D('',#65829,#38484,#38485) ;
#33460=AXIS2_PLACEMENT_3D('',#65831,#38487,#38488) ;
#33461=AXIS2_PLACEMENT_3D('',#65834,#38490,#38491) ;
#33462=AXIS2_PLACEMENT_3D('',#65835,#38492,#38493) ;
#33463=AXIS2_PLACEMENT_3D('',#65837,#38494,#38495) ;
#33464=AXIS2_PLACEMENT_3D('',#65839,#38496,#38497) ;
#33465=AXIS2_PLACEMENT_3D('',#65841,#38499,#38500) ;
#33466=AXIS2_PLACEMENT_3D('',#65843,#38501,#38502) ;
#33467=AXIS2_PLACEMENT_3D('',#65846,#38504,#38505) ;
#33468=AXIS2_PLACEMENT_3D('',#65847,#38506,#38507) ;
#33469=AXIS2_PLACEMENT_3D('',#65854,#38512,#38513) ;
#33470=AXIS2_PLACEMENT_3D('',#65856,#38514,#38515) ;
#33471=AXIS2_PLACEMENT_3D('',#65858,#38517,#38518) ;
#33472=AXIS2_PLACEMENT_3D('',#65860,#38520,#38521) ;
#33473=AXIS2_PLACEMENT_3D('',#65862,#38522,#38523) ;
#33474=AXIS2_PLACEMENT_3D('',#65864,#38525,#38526) ;
#33475=AXIS2_PLACEMENT_3D('',#65866,#38528,#38529) ;
#33476=AXIS2_PLACEMENT_3D('',#65868,#38530,#38531) ;
#33477=AXIS2_PLACEMENT_3D('',#65870,#38533,#38534) ;
#33478=AXIS2_PLACEMENT_3D('',#65872,#38536,#38537) ;
#33479=AXIS2_PLACEMENT_3D('',#65875,#38539,#38540) ;
#33480=AXIS2_PLACEMENT_3D('',#65876,#38541,#38542) ;
#33481=AXIS2_PLACEMENT_3D('',#65879,#38544,#38545) ;
#33482=AXIS2_PLACEMENT_3D('',#65880,#38546,#38547) ;
#33483=AXIS2_PLACEMENT_3D('',#65882,#38548,#38549) ;
#33484=AXIS2_PLACEMENT_3D('',#65886,#38551,#38552) ;
#33485=AXIS2_PLACEMENT_3D('',#65887,#38553,#38554) ;
#33486=AXIS2_PLACEMENT_3D('',#65888,#38555,#38556) ;
#33487=AXIS2_PLACEMENT_3D('',#65891,#38558,#38559) ;
#33488=AXIS2_PLACEMENT_3D('',#65892,#38560,#38561) ;
#33489=AXIS2_PLACEMENT_3D('',#65895,#38562,#38563) ;
#33490=AXIS2_PLACEMENT_3D('',#65899,#38565,#38566) ;
#33491=AXIS2_PLACEMENT_3D('',#65901,#38568,#38569) ;
#33492=AXIS2_PLACEMENT_3D('',#65904,#38570,#38571) ;
#33493=AXIS2_PLACEMENT_3D('',#65908,#38573,#38574) ;
#33494=AXIS2_PLACEMENT_3D('',#65910,#38576,#38577) ;
#33495=AXIS2_PLACEMENT_3D('',#65913,#38578,#38579) ;
#33496=AXIS2_PLACEMENT_3D('',#65917,#38581,#38582) ;
#33497=AXIS2_PLACEMENT_3D('',#65919,#38584,#38585) ;
#33498=AXIS2_PLACEMENT_3D('',#65922,#38586,#38587) ;
#33499=AXIS2_PLACEMENT_3D('',#65926,#38589,#38590) ;
#33500=AXIS2_PLACEMENT_3D('',#65928,#38592,#38593) ;
#33501=AXIS2_PLACEMENT_3D('',#65930,#38594,#38595) ;
#33502=AXIS2_PLACEMENT_3D('',#65932,#38596,#38597) ;
#33503=AXIS2_PLACEMENT_3D('',#65934,#38599,#38600) ;
#33504=AXIS2_PLACEMENT_3D('',#65937,#38601,#38602) ;
#33505=AXIS2_PLACEMENT_3D('',#65941,#38604,#38605) ;
#33506=AXIS2_PLACEMENT_3D('',#65943,#38607,#38608) ;
#33507=AXIS2_PLACEMENT_3D('',#65945,#38609,#38610) ;
#33508=AXIS2_PLACEMENT_3D('',#65947,#38611,#38612) ;
#33509=AXIS2_PLACEMENT_3D('',#65948,#38613,#38614) ;
#33510=AXIS2_PLACEMENT_3D('',#65949,#38615,#38616) ;
#33511=AXIS2_PLACEMENT_3D('',#65950,#38617,#38618) ;
#33512=AXIS2_PLACEMENT_3D('',#65952,#38620,#38621) ;
#33513=AXIS2_PLACEMENT_3D('',#65955,#38624,#38625) ;
#33514=AXIS2_PLACEMENT_3D('',#65958,#38628,#38629) ;
#33515=AXIS2_PLACEMENT_3D('',#65961,#38632,#38633) ;
#33516=AXIS2_PLACEMENT_3D('',#65962,#38634,#38635) ;
#33517=AXIS2_PLACEMENT_3D('',#65964,#38637,#38638) ;
#33518=AXIS2_PLACEMENT_3D('',#65967,#38641,#38642) ;
#33519=AXIS2_PLACEMENT_3D('',#65969,#38644,#38645) ;
#33520=AXIS2_PLACEMENT_3D('',#65971,#38647,#38648) ;
#33521=AXIS2_PLACEMENT_3D('',#65972,#38649,#38650) ;
#33522=AXIS2_PLACEMENT_3D('',#65975,#38653,#38654) ;
#33523=AXIS2_PLACEMENT_3D('',#65977,#38656,#38657) ;
#33524=AXIS2_PLACEMENT_3D('',#65979,#38659,#38660) ;
#33525=AXIS2_PLACEMENT_3D('',#65980,#38661,#38662) ;
#33526=AXIS2_PLACEMENT_3D('',#65983,#38665,#38666) ;
#33527=AXIS2_PLACEMENT_3D('',#65985,#38668,#38669) ;
#33528=AXIS2_PLACEMENT_3D('',#65987,#38671,#38672) ;
#33529=AXIS2_PLACEMENT_3D('',#65988,#38673,#38674) ;
#33530=AXIS2_PLACEMENT_3D('',#65989,#38675,#38676) ;
#33531=AXIS2_PLACEMENT_3D('',#65990,#38677,#38678) ;
#33532=AXIS2_PLACEMENT_3D('',#65993,#38681,#38682) ;
#33533=AXIS2_PLACEMENT_3D('',#65995,#38684,#38685) ;
#33534=AXIS2_PLACEMENT_3D('',#65997,#38687,#38688) ;
#33535=AXIS2_PLACEMENT_3D('',#65998,#38689,#38690) ;
#33536=AXIS2_PLACEMENT_3D('',#66002,#38693,#38694) ;
#33537=AXIS2_PLACEMENT_3D('',#66003,#38695,#38696) ;
#33538=AXIS2_PLACEMENT_3D('',#66007,#38699,#38700) ;
#33539=AXIS2_PLACEMENT_3D('',#66008,#38701,#38702) ;
#33540=AXIS2_PLACEMENT_3D('',#66010,#38703,#38704) ;
#33541=AXIS2_PLACEMENT_3D('',#66012,#38706,#38707) ;
#33542=AXIS2_PLACEMENT_3D('',#66015,#38709,#38710) ;
#33543=AXIS2_PLACEMENT_3D('',#66016,#38711,#38712) ;
#33544=AXIS2_PLACEMENT_3D('',#66020,#38715,#38716) ;
#33545=AXIS2_PLACEMENT_3D('',#66021,#38717,#38718) ;
#33546=AXIS2_PLACEMENT_3D('',#66024,#38720,#38721) ;
#33547=AXIS2_PLACEMENT_3D('',#66025,#38722,#38723) ;
#33548=AXIS2_PLACEMENT_3D('',#66027,#38724,#38725) ;
#33549=AXIS2_PLACEMENT_3D('',#66029,#38727,#38728) ;
#33550=AXIS2_PLACEMENT_3D('',#66031,#38729,#38730) ;
#33551=AXIS2_PLACEMENT_3D('',#66032,#38731,#38732) ;
#33552=AXIS2_PLACEMENT_3D('',#66033,#38733,#38734) ;
#33553=AXIS2_PLACEMENT_3D('',#66035,#38736,#38737) ;
#33554=AXIS2_PLACEMENT_3D('',#66038,#38740,#38741) ;
#33555=AXIS2_PLACEMENT_3D('',#66041,#38744,#38745) ;
#33556=AXIS2_PLACEMENT_3D('',#66044,#38748,#38749) ;
#33557=AXIS2_PLACEMENT_3D('',#66047,#38752,#38753) ;
#33558=AXIS2_PLACEMENT_3D('',#66062,#38761,#38762) ;
#33559=AXIS2_PLACEMENT_3D('',#66066,#38764,#38765) ;
#33560=AXIS2_PLACEMENT_3D('',#66071,#38768,#38769) ;
#33561=AXIS2_PLACEMENT_3D('',#66073,#38770,#38771) ;
#33562=AXIS2_PLACEMENT_3D('',#66075,#38772,#38773) ;
#33563=AXIS2_PLACEMENT_3D('',#66077,#38774,#38775) ;
#33564=AXIS2_PLACEMENT_3D('',#66078,#38776,#38777) ;
#33565=AXIS2_PLACEMENT_3D('',#66080,#38778,#38779) ;
#33566=AXIS2_PLACEMENT_3D('',#66083,#38781,#38782) ;
#33567=AXIS2_PLACEMENT_3D('',#66084,#38783,#38784) ;
#33568=AXIS2_PLACEMENT_3D('',#66086,#38785,#38786) ;
#33569=AXIS2_PLACEMENT_3D('',#66090,#38788,#38789) ;
#33570=AXIS2_PLACEMENT_3D('',#66091,#38790,#38791) ;
#33571=AXIS2_PLACEMENT_3D('',#66092,#38792,#38793) ;
#33572=AXIS2_PLACEMENT_3D('',#66094,#38795,#38796) ;
#33573=AXIS2_PLACEMENT_3D('',#66096,#38797,#38798) ;
#33574=AXIS2_PLACEMENT_3D('',#66100,#38800,#38801) ;
#33575=AXIS2_PLACEMENT_3D('',#66101,#38802,#38803) ;
#33576=AXIS2_PLACEMENT_3D('',#66102,#38804,#38805) ;
#33577=AXIS2_PLACEMENT_3D('',#66104,#38807,#38808) ;
#33578=AXIS2_PLACEMENT_3D('',#66106,#38809,#38810) ;
#33579=AXIS2_PLACEMENT_3D('',#66110,#38812,#38813) ;
#33580=AXIS2_PLACEMENT_3D('',#66111,#38814,#38815) ;
#33581=AXIS2_PLACEMENT_3D('',#66112,#38816,#38817) ;
#33582=AXIS2_PLACEMENT_3D('',#66114,#38819,#38820) ;
#33583=AXIS2_PLACEMENT_3D('',#66116,#38821,#38822) ;
#33584=AXIS2_PLACEMENT_3D('',#66120,#38824,#38825) ;
#33585=AXIS2_PLACEMENT_3D('',#66121,#38826,#38827) ;
#33586=AXIS2_PLACEMENT_3D('',#66122,#38828,#38829) ;
#33587=AXIS2_PLACEMENT_3D('',#66124,#38831,#38832) ;
#33588=AXIS2_PLACEMENT_3D('',#66130,#38836,#38837) ;
#33589=AXIS2_PLACEMENT_3D('',#66131,#38838,#38839) ;
#33590=AXIS2_PLACEMENT_3D('',#66132,#38840,#38841) ;
#33591=AXIS2_PLACEMENT_3D('',#66133,#38842,#38843) ;
#33592=AXIS2_PLACEMENT_3D('',#66134,#38844,#38845) ;
#33593=AXIS2_PLACEMENT_3D('',#66137,#38847,#38848) ;
#33594=AXIS2_PLACEMENT_3D('',#66140,#38851,#38852) ;
#33595=AXIS2_PLACEMENT_3D('',#66144,#38856,#38857) ;
#33596=AXIS2_PLACEMENT_3D('',#66147,#38860,#38861) ;
#33597=AXIS2_PLACEMENT_3D('',#66149,#38863,#38864) ;
#33598=AXIS2_PLACEMENT_3D('',#66151,#38866,#38867) ;
#33599=AXIS2_PLACEMENT_3D('',#66152,#38868,#38869) ;
#33600=AXIS2_PLACEMENT_3D('',#66158,#38873,#38874) ;
#33601=AXIS2_PLACEMENT_3D('',#66161,#38877,#38878) ;
#33602=AXIS2_PLACEMENT_3D('',#66162,#38879,#38880) ;
#33603=AXIS2_PLACEMENT_3D('',#66163,#38881,#38882) ;
#33604=AXIS2_PLACEMENT_3D('',#66164,#38883,#38884) ;
#33605=AXIS2_PLACEMENT_3D('',#66165,#38885,#38886) ;
#33606=AXIS2_PLACEMENT_3D('',#66166,#38887,#38888) ;
#33607=AXIS2_PLACEMENT_3D('',#66169,#38891,#38892) ;
#33608=AXIS2_PLACEMENT_3D('',#66171,#38894,#38895) ;
#33609=AXIS2_PLACEMENT_3D('',#66173,#38897,#38898) ;
#33610=AXIS2_PLACEMENT_3D('',#66174,#38899,#38900) ;
#33611=AXIS2_PLACEMENT_3D('',#66177,#38903,#38904) ;
#33612=AXIS2_PLACEMENT_3D('',#66179,#38906,#38907) ;
#33613=AXIS2_PLACEMENT_3D('',#66181,#38909,#38910) ;
#33614=AXIS2_PLACEMENT_3D('',#66182,#38911,#38912) ;
#33615=AXIS2_PLACEMENT_3D('',#66183,#38913,#38914) ;
#33616=AXIS2_PLACEMENT_3D('',#66184,#38915,#38916) ;
#33617=AXIS2_PLACEMENT_3D('',#66185,#38917,#38918) ;
#33618=AXIS2_PLACEMENT_3D('',#66186,#38919,#38920) ;
#33619=AXIS2_PLACEMENT_3D('',#66187,#38921,#38922) ;
#33620=AXIS2_PLACEMENT_3D('',#66188,#38923,#38924) ;
#33621=AXIS2_PLACEMENT_3D('',#66189,#38925,#38926) ;
#33622=AXIS2_PLACEMENT_3D('',#66192,#38928,#38929) ;
#33623=AXIS2_PLACEMENT_3D('',#66193,#38930,#38931) ;
#33624=AXIS2_PLACEMENT_3D('',#66196,#38934,#38935) ;
#33625=AXIS2_PLACEMENT_3D('',#66198,#38936,#38937) ;
#33626=AXIS2_PLACEMENT_3D('',#66200,#38939,#38940) ;
#33627=AXIS2_PLACEMENT_3D('',#66203,#38943,#38944) ;
#33628=AXIS2_PLACEMENT_3D('',#66204,#38945,#38946) ;
#33629=AXIS2_PLACEMENT_3D('',#66205,#38947,#38948) ;
#33630=AXIS2_PLACEMENT_3D('',#66206,#38949,#38950) ;
#33631=AXIS2_PLACEMENT_3D('',#66207,#38951,#38952) ;
#33632=AXIS2_PLACEMENT_3D('',#66213,#38956,#38957) ;
#33633=AXIS2_PLACEMENT_3D('',#66216,#38958,#38959) ;
#33634=AXIS2_PLACEMENT_3D('',#66218,#38961,#38962) ;
#33635=AXIS2_PLACEMENT_3D('',#66219,#38963,#38964) ;
#33636=AXIS2_PLACEMENT_3D('',#66957,#38966,#38967) ;
#33637=AXIS2_PLACEMENT_3D('',#66963,#38971,#38972) ;
#33638=AXIS2_PLACEMENT_3D('',#66969,#38976,#38977) ;
#33639=AXIS2_PLACEMENT_3D('',#66975,#38981,#38982) ;
#33640=AXIS2_PLACEMENT_3D('',#66981,#38986,#38987) ;
#33641=AXIS2_PLACEMENT_3D('',#66982,#38988,#38989) ;
#33642=AXIS2_PLACEMENT_3D('',#66983,#38990,#38991) ;
#33643=AXIS2_PLACEMENT_3D('',#66984,#38992,#38993) ;
#33644=AXIS2_PLACEMENT_3D('',#66985,#38994,#38995) ;
#33645=AXIS2_PLACEMENT_3D('',#66986,#38996,#38997) ;
#33646=AXIS2_PLACEMENT_3D('',#66987,#38998,#38999) ;
#33647=AXIS2_PLACEMENT_3D('',#66988,#39000,#39001) ;
#33648=AXIS2_PLACEMENT_3D('',#66989,#39002,#39003) ;
#33649=AXIS2_PLACEMENT_3D('',#66990,#39004,#39005) ;
#33650=AXIS2_PLACEMENT_3D('',#66991,#39006,#39007) ;
#33651=AXIS2_PLACEMENT_3D('',#66992,#39008,#39009) ;
#33652=AXIS2_PLACEMENT_3D('',#66993,#39010,#39011) ;
#33653=AXIS2_PLACEMENT_3D('',#66994,#39012,#39013) ;
#33654=AXIS2_PLACEMENT_3D('',#66995,#39014,#39015) ;
#33655=AXIS2_PLACEMENT_3D('',#66996,#39016,#39017) ;
#33656=AXIS2_PLACEMENT_3D('',#66997,#39018,#39019) ;
#33657=AXIS2_PLACEMENT_3D('',#66998,#39020,#39021) ;
#33658=AXIS2_PLACEMENT_3D('',#66999,#39022,#39023) ;
#33659=AXIS2_PLACEMENT_3D('',#67000,#39024,#39025) ;
#33660=AXIS2_PLACEMENT_3D('',#67001,#39026,#39027) ;
#33661=AXIS2_PLACEMENT_3D('',#67002,#39028,#39029) ;
#33662=AXIS2_PLACEMENT_3D('',#67003,#39030,#39031) ;
#33663=AXIS2_PLACEMENT_3D('',#67004,#39032,#39033) ;
#33664=AXIS2_PLACEMENT_3D('',#67005,#39034,#39035) ;
#33665=AXIS2_PLACEMENT_3D('',#67007,#39036,#39037) ;
#33666=AXIS2_PLACEMENT_3D('',#67010,#39039,#39040) ;
#33667=AXIS2_PLACEMENT_3D('',#67011,#39041,#39042) ;
#33668=AXIS2_PLACEMENT_3D('',#67012,#39043,#39044) ;
#33669=AXIS2_PLACEMENT_3D('',#67013,#39045,#39046) ;
#33670=AXIS2_PLACEMENT_3D('',#67015,#39047,#39048) ;
#33671=AXIS2_PLACEMENT_3D('',#67017,#39050,#39051) ;
#33672=AXIS2_PLACEMENT_3D('',#67018,#39052,#39053) ;
#33673=AXIS2_PLACEMENT_3D('',#67019,#39054,#39055) ;
#33674=AXIS2_PLACEMENT_3D('',#67021,#39057,#39058) ;
#33675=AXIS2_PLACEMENT_3D('',#67023,#39059,#39060) ;
#33676=AXIS2_PLACEMENT_3D('',#67025,#39062,#39063) ;
#33677=AXIS2_PLACEMENT_3D('',#67027,#39064,#39065) ;
#33678=AXIS2_PLACEMENT_3D('',#67029,#39067,#39068) ;
#33679=AXIS2_PLACEMENT_3D('',#67031,#39069,#39070) ;
#33680=AXIS2_PLACEMENT_3D('',#67034,#39072,#39073) ;
#33681=AXIS2_PLACEMENT_3D('',#67044,#39074,#39075) ;
#33682=AXIS2_PLACEMENT_3D('',#67045,#39076,#39077) ;
#33683=AXIS2_PLACEMENT_3D('',#67046,#39078,#39079) ;
#33684=AXIS2_PLACEMENT_3D('',#67056,#39080,#39081) ;
#33685=AXIS2_PLACEMENT_3D('',#67058,#39082,#39083) ;
#33686=AXIS2_PLACEMENT_3D('',#67062,#39085,#39086) ;
#33687=AXIS2_PLACEMENT_3D('',#67064,#39088,#39089) ;
#33688=AXIS2_PLACEMENT_3D('',#67065,#39090,#39091) ;
#33689=AXIS2_PLACEMENT_3D('',#67075,#39092,#39093) ;
#33690=AXIS2_PLACEMENT_3D('',#67076,#39094,#39095) ;
#33691=AXIS2_PLACEMENT_3D('',#67077,#39096,#39097) ;
#33692=AXIS2_PLACEMENT_3D('',#68689,#39098,#39099) ;
#33693=AXIS2_PLACEMENT_3D('',#69260,#39118,#39119) ;
#33694=AXIS2_PLACEMENT_3D('',#69266,#39123,#39124) ;
#33695=AXIS2_PLACEMENT_3D('',#69270,#39127,#39128) ;
#33696=AXIS2_PLACEMENT_3D('',#69274,#39131,#39132) ;
#33697=AXIS2_PLACEMENT_3D('',#69278,#39135,#39136) ;
#33698=AXIS2_PLACEMENT_3D('',#69282,#39139,#39140) ;
#33699=AXIS2_PLACEMENT_3D('',#69284,#39142,#39143) ;
#33700=AXIS2_PLACEMENT_3D('',#69290,#39147,#39148) ;
#33701=AXIS2_PLACEMENT_3D('',#69294,#39151,#39152) ;
#33702=AXIS2_PLACEMENT_3D('',#69298,#39155,#39156) ;
#33703=AXIS2_PLACEMENT_3D('',#69302,#39159,#39160) ;
#33704=AXIS2_PLACEMENT_3D('',#69306,#39163,#39164) ;
#33705=AXIS2_PLACEMENT_3D('',#69308,#39166,#39167) ;
#33706=AXIS2_PLACEMENT_3D('',#69321,#39174,#39175) ;
#33707=AXIS2_PLACEMENT_3D('',#69324,#39178,#39179) ;
#33708=AXIS2_PLACEMENT_3D('',#69326,#39181,#39182) ;
#33709=AXIS2_PLACEMENT_3D('',#69328,#39184,#39185) ;
#33710=AXIS2_PLACEMENT_3D('',#69330,#39187,#39188) ;
#33711=AXIS2_PLACEMENT_3D('',#69332,#39190,#39191) ;
#33712=AXIS2_PLACEMENT_3D('',#69333,#39192,#39193) ;
#33713=AXIS2_PLACEMENT_3D('',#69334,#39194,#39195) ;
#37309=DIRECTION('axis',(0.,0.,1.)) ;
#37310=DIRECTION('refdir',(1.,0.,0.)) ;
#37653=DIRECTION('center_axis',(4.54195640846217E-14,-1.66321791214601E-16,
1.)) ;
#37654=DIRECTION('ref_axis',(0.609352821942987,-0.792899198126797,-2.78084159612697E-14)) ;
#37655=DIRECTION('',(4.54195640846217E-14,-1.66321791214601E-16,1.)) ;
#37656=DIRECTION('center_axis',(-4.54195640846217E-14,1.66321791214601E-16,
-1.)) ;
#37657=DIRECTION('ref_axis',(-1.,-3.64900768663075E-31,4.54195640846217E-14)) ;
#37658=DIRECTION('center_axis',(4.54195640846217E-14,-1.66321791214601E-16,
1.)) ;
#37659=DIRECTION('ref_axis',(0.609352821942987,-0.792899198126797,-2.78084159612697E-14)) ;
#37660=DIRECTION('',(4.54195640846217E-14,-1.66321791214601E-16,1.)) ;
#37661=DIRECTION('center_axis',(4.54195640846217E-14,-1.66321791214601E-16,
1.)) ;
#37662=DIRECTION('ref_axis',(0.609352821942987,-0.792899198126797,-2.78084159612697E-14)) ;
#37663=DIRECTION('',(4.54195640846217E-14,-1.66321791214601E-16,1.)) ;
#37664=DIRECTION('center_axis',(4.54195640846217E-14,-1.66321791214601E-16,
1.)) ;
#37665=DIRECTION('ref_axis',(-1.,-3.64900768663092E-31,4.54195640846217E-14)) ;
#37666=DIRECTION('center_axis',(4.54195640846217E-14,-1.66321791214601E-16,
1.)) ;
#37667=DIRECTION('ref_axis',(0.980619819129883,0.195920316275966,-4.45067388996815E-14)) ;
#37668=DIRECTION('',(4.54195640846217E-14,-1.66321791214601E-16,1.)) ;
#37669=DIRECTION('center_axis',(-4.54195640846217E-14,1.66321791214601E-16,
-1.)) ;
#37670=DIRECTION('ref_axis',(-1.,3.4580495717732E-14,4.54195640846217E-14)) ;
#37671=DIRECTION('center_axis',(4.54195640846217E-14,-1.66321791214601E-16,
1.)) ;
#37672=DIRECTION('ref_axis',(0.980619819129883,0.195920316275966,-4.45067388996815E-14)) ;
#37673=DIRECTION('',(4.54195640846217E-14,-1.66321791214601E-16,1.)) ;
#37674=DIRECTION('center_axis',(4.54195640846217E-14,-1.66321791214601E-16,
1.)) ;
#37675=DIRECTION('ref_axis',(0.980619819129883,0.195920316275966,-4.45067388996815E-14)) ;
#37676=DIRECTION('',(4.54195640846217E-14,-1.66321791214601E-16,1.)) ;
#37677=DIRECTION('center_axis',(4.54195640846217E-14,-1.66321791214601E-16,
1.)) ;
#37678=DIRECTION('ref_axis',(-1.,3.4580495717732E-14,4.54195640846217E-14)) ;
#37679=DIRECTION('center_axis',(4.54195640846217E-14,-1.66321791214601E-16,
1.)) ;
#37680=DIRECTION('ref_axis',(0.609364319911517,-0.792890361663436,-2.78089367242917E-14)) ;
#37681=DIRECTION('',(4.54195640846217E-14,-1.66321791214601E-16,1.)) ;
#37682=DIRECTION('center_axis',(-4.54195640846217E-14,1.66321791214601E-16,
-1.)) ;
#37683=DIRECTION('ref_axis',(-1.,3.4580495717732E-14,4.54195640846217E-14)) ;
#37684=DIRECTION('center_axis',(4.54195640846217E-14,-1.66321791214601E-16,
1.)) ;
#37685=DIRECTION('ref_axis',(0.609364319911517,-0.792890361663436,-2.78089367242917E-14)) ;
#37686=DIRECTION('',(4.54195640846217E-14,-1.66321791214601E-16,1.)) ;
#37687=DIRECTION('center_axis',(4.54195640846217E-14,-1.66321791214601E-16,
1.)) ;
#37688=DIRECTION('ref_axis',(0.609364319911517,-0.792890361663436,-2.78089367242917E-14)) ;
#37689=DIRECTION('',(4.54195640846217E-14,-1.66321791214601E-16,1.)) ;
#37690=DIRECTION('center_axis',(4.54195640846217E-14,-1.66321791214601E-16,
1.)) ;
#37691=DIRECTION('ref_axis',(-1.,3.4580495717732E-14,4.54195640846217E-14)) ;
#37692=DIRECTION('center_axis',(4.54195640846217E-14,-1.66321791214601E-16,
1.)) ;
#37693=DIRECTION('ref_axis',(0.609355676053996,-0.792897004699083,-2.78085452289327E-14)) ;
#37694=DIRECTION('',(4.54195640846217E-14,-1.66321791214601E-16,1.)) ;
#37695=DIRECTION('center_axis',(-4.54195640846217E-14,1.66321791214601E-16,
-1.)) ;
#37696=DIRECTION('ref_axis',(-1.,3.54035479944944E-31,4.54195640846217E-14)) ;
#37697=DIRECTION('center_axis',(4.54195640846217E-14,-1.66321791214601E-16,
1.)) ;
#37698=DIRECTION('ref_axis',(0.609355676053996,-0.792897004699083,-2.78085452289327E-14)) ;
#37699=DIRECTION('',(4.54195640846217E-14,-1.66321791214601E-16,1.)) ;
#37700=DIRECTION('center_axis',(4.54195640846217E-14,-1.66321791214601E-16,
1.)) ;
#37701=DIRECTION('ref_axis',(0.609355676053996,-0.792897004699083,-2.78085452289327E-14)) ;
#37702=DIRECTION('',(4.54195640846217E-14,-1.66321791214601E-16,1.)) ;
#37703=DIRECTION('center_axis',(4.54195640846217E-14,-1.66321791214601E-16,
1.)) ;
#37704=DIRECTION('ref_axis',(-1.,3.54035479944944E-31,4.54195640846217E-14)) ;
#37705=DIRECTION('center_axis',(4.54195640846217E-14,-1.66321791214601E-16,
1.)) ;
#37706=DIRECTION('ref_axis',(-0.938429938932521,-0.345469607512881,4.25656196263415E-14)) ;
#37707=DIRECTION('',(4.54195640846217E-14,-1.66321791214601E-16,1.)) ;
#37708=DIRECTION('center_axis',(-4.54195640846217E-14,1.66321791214601E-16,
-1.)) ;
#37709=DIRECTION('ref_axis',(-1.,5.55236256206829E-46,4.54195640846217E-14)) ;
#37710=DIRECTION('center_axis',(4.54195640846217E-14,-1.66321791214601E-16,
1.)) ;
#37711=DIRECTION('ref_axis',(-0.938429938932521,-0.345469607512881,4.25656196263415E-14)) ;
#37712=DIRECTION('',(4.54195640846217E-14,-1.66321791214601E-16,1.)) ;
#37713=DIRECTION('center_axis',(-4.54195640846217E-14,1.66321791214601E-16,
-1.)) ;
#37714=DIRECTION('ref_axis',(-1.,5.55236256206829E-46,4.54195640846217E-14)) ;
#37715=DIRECTION('center_axis',(4.54195640846217E-14,-1.66321791214601E-16,
1.)) ;
#37716=DIRECTION('ref_axis',(-0.938429938932521,-0.345469607512881,4.25656196263415E-14)) ;
#37717=DIRECTION('',(4.54195640846217E-14,-1.66321791214601E-16,1.)) ;
#37718=DIRECTION('center_axis',(4.54195640846217E-14,-1.66321791214601E-16,
1.)) ;
#37719=DIRECTION('ref_axis',(-1.,5.55236256206829E-46,4.54195640846217E-14)) ;
#37720=DIRECTION('center_axis',(4.54195640846217E-14,-1.66321791214601E-16,
1.)) ;
#37721=DIRECTION('ref_axis',(-0.938428681849293,-0.345473022221127,4.25655619622289E-14)) ;
#37722=DIRECTION('',(4.54195640846217E-14,-1.66321791214601E-16,1.)) ;
#37723=DIRECTION('center_axis',(-4.54195640846217E-14,1.66321791214601E-16,
-1.)) ;
#37724=DIRECTION('ref_axis',(-1.,5.55236256206829E-46,4.54195640846217E-14)) ;
#37725=DIRECTION('center_axis',(4.54195640846217E-14,-1.66321791214601E-16,
1.)) ;
#37726=DIRECTION('ref_axis',(-0.938428681849293,-0.345473022221127,4.25655619622289E-14)) ;
#37727=DIRECTION('',(4.54195640846217E-14,-1.66321791214601E-16,1.)) ;
#37728=DIRECTION('center_axis',(-4.54195640846217E-14,1.66321791214601E-16,
-1.)) ;
#37729=DIRECTION('ref_axis',(-1.,5.55236256206829E-46,4.54195640846217E-14)) ;
#37730=DIRECTION('center_axis',(4.54195640846217E-14,-1.66321791214601E-16,
1.)) ;
#37731=DIRECTION('ref_axis',(-0.938428681849293,-0.345473022221127,4.25655619622289E-14)) ;
#37732=DIRECTION('',(4.54195640846217E-14,-1.66321791214601E-16,1.)) ;
#37733=DIRECTION('center_axis',(4.54195640846217E-14,-1.66321791214601E-16,
1.)) ;
#37734=DIRECTION('ref_axis',(-1.,5.55236256206829E-46,4.54195640846217E-14)) ;
#37735=DIRECTION('center_axis',(4.54195640846217E-14,-1.66321791214601E-16,
1.)) ;
#37736=DIRECTION('ref_axis',(-0.938433691542647,-0.345459413792185,4.25657917636955E-14)) ;
#37737=DIRECTION('',(4.54195640846217E-14,-1.66321791214601E-16,1.)) ;
#37738=DIRECTION('center_axis',(-4.54195640846217E-14,1.66321791214601E-16,
-1.)) ;
#37739=DIRECTION('ref_axis',(-1.,5.55236256206829E-46,4.54195640846217E-14)) ;
#37740=DIRECTION('center_axis',(4.54195640846217E-14,-1.66321791214601E-16,
1.)) ;
#37741=DIRECTION('ref_axis',(-0.938433691542647,-0.345459413792185,4.25657917636955E-14)) ;
#37742=DIRECTION('',(4.54195640846217E-14,-1.66321791214601E-16,1.)) ;
#37743=DIRECTION('center_axis',(-4.54195640846217E-14,1.66321791214601E-16,
-1.)) ;
#37744=DIRECTION('ref_axis',(-1.,5.55236256206829E-46,4.54195640846217E-14)) ;
#37745=DIRECTION('center_axis',(4.54195640846217E-14,-1.66321791214601E-16,
1.)) ;
#37746=DIRECTION('ref_axis',(-0.938433691542647,-0.345459413792185,4.25657917636955E-14)) ;
#37747=DIRECTION('',(4.54195640846217E-14,-1.66321791214601E-16,1.)) ;
#37748=DIRECTION('center_axis',(4.54195640846217E-14,-1.66321791214601E-16,
1.)) ;
#37749=DIRECTION('ref_axis',(-1.,5.55236256206829E-46,4.54195640846217E-14)) ;
#37750=DIRECTION('center_axis',(4.54195640846217E-14,-1.66321791214601E-16,
1.)) ;
#37751=DIRECTION('ref_axis',(-0.938432448023048,-0.345462791769924,4.25657347217461E-14)) ;
#37752=DIRECTION('',(4.54195640846217E-14,-1.66321791214601E-16,1.)) ;
#37753=DIRECTION('center_axis',(-4.54195640846217E-14,1.66321791214601E-16,
-1.)) ;
#37754=DIRECTION('ref_axis',(-1.,5.55236256206829E-46,4.54195640846217E-14)) ;
#37755=DIRECTION('center_axis',(4.54195640846217E-14,-1.66321791214601E-16,
1.)) ;
#37756=DIRECTION('ref_axis',(-0.938432448023048,-0.345462791769924,4.25657347217461E-14)) ;
#37757=DIRECTION('',(4.54195640846217E-14,-1.66321791214601E-16,1.)) ;
#37758=DIRECTION('center_axis',(-4.54195640846217E-14,1.66321791214601E-16,
-1.)) ;
#37759=DIRECTION('ref_axis',(-1.,5.55236256206829E-46,4.54195640846217E-14)) ;
#37760=DIRECTION('center_axis',(4.54195640846217E-14,-1.66321791214601E-16,
1.)) ;
#37761=DIRECTION('ref_axis',(-0.938432448023048,-0.345462791769924,4.25657347217461E-14)) ;
#37762=DIRECTION('',(4.54195640846217E-14,-1.66321791214601E-16,1.)) ;
#37763=DIRECTION('center_axis',(4.54195640846217E-14,-1.66321791214601E-16,
1.)) ;
#37764=DIRECTION('ref_axis',(-1.,5.55236256206829E-46,4.54195640846217E-14)) ;
#37765=DIRECTION('center_axis',(1.75658099177411E-13,1.,1.66321791206623E-16)) ;
#37766=DIRECTION('ref_axis',(-0.792895134159569,1.39177102581146E-13,0.609358110002713)) ;
#37767=DIRECTION('',(1.75658099177411E-13,1.,1.66321791206623E-16)) ;
#37768=DIRECTION('center_axis',(-1.75658099177411E-13,-1.,-1.66321791206623E-16)) ;
#37769=DIRECTION('ref_axis',(1.72902478588661E-14,1.66321791203586E-16,
-1.)) ;
#37770=DIRECTION('center_axis',(1.75658099177411E-13,1.,1.66321791206623E-16)) ;
#37771=DIRECTION('ref_axis',(-0.792895134159569,1.39177102581146E-13,0.609358110002713)) ;
#37772=DIRECTION('',(1.75658099177411E-13,1.,1.66321791206623E-16)) ;
#37773=DIRECTION('center_axis',(1.75658099177411E-13,1.,1.66321791206623E-16)) ;
#37774=DIRECTION('ref_axis',(0.195317858763442,-3.44722822381472E-14,0.980739993090964)) ;
#37775=DIRECTION('',(1.75658099177411E-13,1.,1.66321791206623E-16)) ;
#37776=DIRECTION('center_axis',(1.75658099177411E-13,1.,1.66321791206623E-16)) ;
#37777=DIRECTION('ref_axis',(1.72902478588661E-14,1.66321791203586E-16,
-1.)) ;
#37778=DIRECTION('center_axis',(1.75658099177411E-13,1.,1.66321791206623E-16)) ;
#37779=DIRECTION('ref_axis',(-0.792888490970559,1.39175934213506E-13,0.609366754004868)) ;
#37780=DIRECTION('',(1.75658099177411E-13,1.,1.66321791206623E-16)) ;
#37781=DIRECTION('center_axis',(-1.75658099177411E-13,-1.,-1.66321791206623E-16)) ;
#37782=DIRECTION('ref_axis',(2.16128098235828E-15,1.66321791206243E-16,
-1.)) ;
#37783=DIRECTION('center_axis',(1.75658099177411E-13,1.,1.66321791206623E-16)) ;
#37784=DIRECTION('ref_axis',(-0.792888490970559,1.39175934213506E-13,0.609366754004868)) ;
#37785=DIRECTION('',(1.75658099177411E-13,1.,1.66321791206623E-16)) ;
#37786=DIRECTION('center_axis',(1.75658099177411E-13,1.,1.66321791206623E-16)) ;
#37787=DIRECTION('ref_axis',(-0.792888490970559,1.39175934213506E-13,0.609366754004868)) ;
#37788=DIRECTION('',(1.75658099177411E-13,1.,1.66321791206623E-16)) ;
#37789=DIRECTION('center_axis',(1.75658099177411E-13,1.,1.66321791206623E-16)) ;
#37790=DIRECTION('ref_axis',(2.16128098235828E-15,1.66321791206243E-16,
-1.)) ;
#37791=DIRECTION('center_axis',(1.75658099177411E-13,1.,1.66321791206623E-16)) ;
#37792=DIRECTION('ref_axis',(-0.345475903104034,6.08417214137425E-14,-0.938427621276384)) ;
#37793=DIRECTION('',(1.75658099177411E-13,1.,1.66321791206623E-16)) ;
#37794=DIRECTION('center_axis',(-1.75658099177411E-13,-1.,-1.66321791206623E-16)) ;
#37795=DIRECTION('ref_axis',(2.14929886997261E-46,1.66321791206623E-16,
-1.)) ;
#37796=DIRECTION('center_axis',(1.75658099177411E-13,1.,1.66321791206623E-16)) ;
#37797=DIRECTION('ref_axis',(-0.345475903104034,6.08417214137425E-14,-0.938427621276384)) ;
#37798=DIRECTION('',(1.75658099177411E-13,1.,1.66321791206623E-16)) ;
#37799=DIRECTION('center_axis',(-1.75658099177411E-13,-1.,-1.66321791206623E-16)) ;
#37800=DIRECTION('ref_axis',(2.14929886997261E-46,1.66321791206623E-16,
-1.)) ;
#37801=DIRECTION('center_axis',(1.75658099177411E-13,1.,1.66321791206623E-16)) ;
#37802=DIRECTION('ref_axis',(-0.345475903104034,6.08417214137425E-14,-0.938427621276384)) ;
#37803=DIRECTION('',(1.75658099177411E-13,1.,1.66321791206623E-16)) ;
#37804=DIRECTION('center_axis',(1.75658099177411E-13,1.,1.66321791206623E-16)) ;
#37805=DIRECTION('ref_axis',(2.14929886997261E-46,1.66321791206623E-16,
-1.)) ;
#37806=DIRECTION('center_axis',(1.75658099177411E-13,1.,1.66321791206623E-16)) ;
#37807=DIRECTION('ref_axis',(-0.345465672469094,6.08399249462695E-14,-0.938431387553441)) ;
#37808=DIRECTION('',(1.75658099177411E-13,1.,1.66321791206623E-16)) ;
#37809=DIRECTION('center_axis',(-1.75658099177411E-13,-1.,-1.66321791206623E-16)) ;
#37810=DIRECTION('ref_axis',(2.14929886997261E-46,1.66321791206623E-16,
-1.)) ;
#37811=DIRECTION('center_axis',(1.75658099177411E-13,1.,1.66321791206623E-16)) ;
#37812=DIRECTION('ref_axis',(-0.345465672469094,6.08399249462695E-14,-0.938431387553441)) ;
#37813=DIRECTION('',(1.75658099177411E-13,1.,1.66321791206623E-16)) ;
#37814=DIRECTION('center_axis',(-1.75658099177411E-13,-1.,-1.66321791206623E-16)) ;
#37815=DIRECTION('ref_axis',(2.14929886997261E-46,1.66321791206623E-16,
-1.)) ;
#37816=DIRECTION('center_axis',(1.75658099177411E-13,1.,1.66321791206623E-16)) ;
#37817=DIRECTION('ref_axis',(-0.345465672469094,6.08399249462695E-14,-0.938431387553441)) ;
#37818=DIRECTION('',(1.75658099177411E-13,1.,1.66321791206623E-16)) ;
#37819=DIRECTION('center_axis',(1.75658099177411E-13,1.,1.66321791206623E-16)) ;
#37820=DIRECTION('ref_axis',(2.14929886997261E-46,1.66321791206623E-16,
-1.)) ;
#37821=DIRECTION('center_axis',(-1.75658099177411E-13,-1.,-1.66321791206623E-16)) ;
#37822=DIRECTION('ref_axis',(-0.792900091868732,1.39380671434654E-13,-0.609351658990567)) ;
#37823=DIRECTION('',(-1.75658099177411E-13,-1.,-1.66321791206623E-16)) ;
#37824=DIRECTION('center_axis',(1.75658099177411E-13,1.,1.66321791206623E-16)) ;
#37825=DIRECTION('ref_axis',(-1.72902478588661E-14,-1.66321791203586E-16,
1.)) ;
#37826=DIRECTION('center_axis',(-1.75658099177411E-13,-1.,-1.66321791206623E-16)) ;
#37827=DIRECTION('ref_axis',(-0.792900091868732,1.39380671434654E-13,-0.609351658990567)) ;
#37828=DIRECTION('',(-1.75658099177411E-13,-1.,-1.66321791206623E-16)) ;
#37829=DIRECTION('center_axis',(-1.75658099177411E-13,-1.,-1.66321791206623E-16)) ;
#37830=DIRECTION('ref_axis',(-0.792900091868732,1.39380671434654E-13,-0.609351658990567)) ;
#37831=DIRECTION('',(-1.75658099177411E-13,-1.,-1.66321791206623E-16)) ;
#37832=DIRECTION('center_axis',(-1.75658099177411E-13,-1.,-1.66321791206623E-16)) ;
#37833=DIRECTION('ref_axis',(-1.72902478588661E-14,-1.66321791203586E-16,
1.)) ;
#37834=DIRECTION('center_axis',(-1.75658099177411E-13,-1.,-1.66321791206623E-16)) ;
#37835=DIRECTION('ref_axis',(-0.792893488573911,1.39379512941514E-13,-0.609360251228363)) ;
#37836=DIRECTION('',(-1.75658099177411E-13,-1.,-1.66321791206623E-16)) ;
#37837=DIRECTION('center_axis',(1.75658099177411E-13,1.,1.66321791206623E-16)) ;
#37838=DIRECTION('ref_axis',(6.48384294707473E-15,-1.66321791207762E-16,
1.)) ;
#37839=DIRECTION('center_axis',(-1.75658099177411E-13,-1.,-1.66321791206623E-16)) ;
#37840=DIRECTION('ref_axis',(-0.792893488573911,1.39379512941514E-13,-0.609360251228363)) ;
#37841=DIRECTION('',(-1.75658099177411E-13,-1.,-1.66321791206623E-16)) ;
#37842=DIRECTION('center_axis',(-1.75658099177411E-13,-1.,-1.66321791206623E-16)) ;
#37843=DIRECTION('ref_axis',(-0.792893488573911,1.39379512941514E-13,-0.609360251228363)) ;
#37844=DIRECTION('',(-1.75658099177411E-13,-1.,-1.66321791206623E-16)) ;
#37845=DIRECTION('center_axis',(-1.75658099177411E-13,-1.,-1.66321791206623E-16)) ;
#37846=DIRECTION('ref_axis',(6.48384294707473E-15,-1.66321791207762E-16,
1.)) ;
#37847=DIRECTION('center_axis',(-1.75658099177411E-13,-1.,-1.66321791206623E-16)) ;
#37848=DIRECTION('ref_axis',(-0.345468206718894,6.05282070843357E-14,0.938430454613676)) ;
#37849=DIRECTION('',(-1.75658099177411E-13,-1.,-1.66321791206623E-16)) ;
#37850=DIRECTION('center_axis',(1.75658099177411E-13,1.,1.66321791206623E-16)) ;
#37851=DIRECTION('ref_axis',(-2.14929886997261E-46,-1.66321791206623E-16,
1.)) ;
#37852=DIRECTION('center_axis',(-1.75658099177411E-13,-1.,-1.66321791206623E-16)) ;
#37853=DIRECTION('ref_axis',(-0.345468206718894,6.05282070843357E-14,0.938430454613676)) ;
#37854=DIRECTION('',(-1.75658099177411E-13,-1.,-1.66321791206623E-16)) ;
#37855=DIRECTION('center_axis',(1.75658099177411E-13,1.,1.66321791206623E-16)) ;
#37856=DIRECTION('ref_axis',(-2.14929886997261E-46,-1.66321791206623E-16,
1.)) ;
#37857=DIRECTION('center_axis',(-1.75658099177411E-13,-1.,-1.66321791206623E-16)) ;
#37858=DIRECTION('ref_axis',(-0.345468206718894,6.05282070843357E-14,0.938430454613676)) ;
#37859=DIRECTION('',(-1.75658099177411E-13,-1.,-1.66321791206623E-16)) ;
#37860=DIRECTION('center_axis',(-1.75658099177411E-13,-1.,-1.66321791206623E-16)) ;
#37861=DIRECTION('ref_axis',(-2.14929886997261E-46,-1.66321791206623E-16,
1.)) ;
#37862=DIRECTION('center_axis',(-1.75658099177411E-13,-1.,-1.66321791206623E-16)) ;
#37863=DIRECTION('ref_axis',(-0.345458037383117,6.05264201354982E-14,0.938434198229905)) ;
#37864=DIRECTION('',(-1.75658099177411E-13,-1.,-1.66321791206623E-16)) ;
#37865=DIRECTION('center_axis',(1.75658099177411E-13,1.,1.66321791206623E-16)) ;
#37866=DIRECTION('ref_axis',(-2.14929886997261E-46,-1.66321791206623E-16,
1.)) ;
#37867=DIRECTION('center_axis',(-1.75658099177411E-13,-1.,-1.66321791206623E-16)) ;
#37868=DIRECTION('ref_axis',(-0.345458037383117,6.05264201354982E-14,0.938434198229905)) ;
#37869=DIRECTION('',(-1.75658099177411E-13,-1.,-1.66321791206623E-16)) ;
#37870=DIRECTION('center_axis',(1.75658099177411E-13,1.,1.66321791206623E-16)) ;
#37871=DIRECTION('ref_axis',(-2.14929886997261E-46,-1.66321791206623E-16,
1.)) ;
#37872=DIRECTION('center_axis',(-1.75658099177411E-13,-1.,-1.66321791206623E-16)) ;
#37873=DIRECTION('ref_axis',(-0.345458037383117,6.05264201354982E-14,0.938434198229905)) ;
#37874=DIRECTION('',(-1.75658099177411E-13,-1.,-1.66321791206623E-16)) ;
#37875=DIRECTION('center_axis',(-1.75658099177411E-13,-1.,-1.66321791206623E-16)) ;
#37876=DIRECTION('ref_axis',(-2.14929886997261E-46,-1.66321791206623E-16,
1.)) ;
#37877=DIRECTION('center_axis',(-1.75658099177411E-13,-1.,-1.66321791206623E-16)) ;
#37878=DIRECTION('ref_axis',(-0.345458037383117,6.05264201354982E-14,0.938434198229905)) ;
#37879=DIRECTION('center_axis',(-1.75658099177411E-13,-1.,-1.66321791206623E-16)) ;
#37880=DIRECTION('ref_axis',(-0.345468206718894,6.05282070843357E-14,0.938430454613676)) ;
#37881=DIRECTION('center_axis',(-1.75658099177411E-13,-1.,-1.66321791206623E-16)) ;
#37882=DIRECTION('ref_axis',(-0.792893488573911,1.39379512941514E-13,-0.609360251228363)) ;
#37883=DIRECTION('center_axis',(-1.75658099177411E-13,-1.,-1.66321791206623E-16)) ;
#37884=DIRECTION('ref_axis',(-0.792900091868732,1.39380671434654E-13,-0.609351658990567)) ;
#37885=DIRECTION('center_axis',(1.75658099177411E-13,1.,1.66321791206623E-16)) ;
#37886=DIRECTION('ref_axis',(-0.345465672469094,6.08399249462695E-14,-0.938431387553441)) ;
#37887=DIRECTION('center_axis',(1.75658099177411E-13,1.,1.66321791206623E-16)) ;
#37888=DIRECTION('ref_axis',(-0.345475903104034,6.08417214137425E-14,-0.938427621276384)) ;
#37889=DIRECTION('center_axis',(1.75658099177411E-13,1.,1.66321791206623E-16)) ;
#37890=DIRECTION('ref_axis',(-0.792888490970559,1.39175934213506E-13,0.609366754004868)) ;
#37891=DIRECTION('center_axis',(1.75658099177411E-13,1.,1.66321791206623E-16)) ;
#37892=DIRECTION('ref_axis',(-0.792895134159569,1.39177102581146E-13,0.609358110002713)) ;
#37893=DIRECTION('center_axis',(4.54195640846217E-14,-1.66321791214601E-16,
1.)) ;
#37894=DIRECTION('ref_axis',(-0.938432448023048,-0.345462791769924,4.25657347217461E-14)) ;
#37895=DIRECTION('center_axis',(4.54195640846217E-14,-1.66321791214601E-16,
1.)) ;
#37896=DIRECTION('ref_axis',(-0.938433691542647,-0.345459413792185,4.25657917636955E-14)) ;
#37897=DIRECTION('center_axis',(4.54195640846217E-14,-1.66321791214601E-16,
1.)) ;
#37898=DIRECTION('ref_axis',(-0.938428681849293,-0.345473022221127,4.25655619622289E-14)) ;
#37899=DIRECTION('center_axis',(4.54195640846217E-14,-1.66321791214601E-16,
1.)) ;
#37900=DIRECTION('ref_axis',(-0.938429938932521,-0.345469607512881,4.25656196263415E-14)) ;
#37901=DIRECTION('center_axis',(4.54195640846217E-14,-1.66321791214601E-16,
1.)) ;
#37902=DIRECTION('ref_axis',(0.609355676053996,-0.792897004699083,-2.78085452289327E-14)) ;
#37903=DIRECTION('center_axis',(4.54195640846217E-14,-1.66321791214601E-16,
1.)) ;
#37904=DIRECTION('ref_axis',(0.609364319911517,-0.792890361663436,-2.78089367242917E-14)) ;
#37905=DIRECTION('center_axis',(4.54195640846217E-14,-1.66321791214601E-16,
1.)) ;
#37906=DIRECTION('ref_axis',(0.980619819129883,0.195920316275966,-4.45067388996815E-14)) ;
#37907=DIRECTION('center_axis',(4.54195640846217E-14,-1.66321791214601E-16,
1.)) ;
#37908=DIRECTION('ref_axis',(0.609352821942987,-0.792899198126797,-2.78084159612697E-14)) ;
#37909=DIRECTION('center_axis',(-1.,1.75658099177411E-13,4.54195640846217E-14)) ;
#37910=DIRECTION('ref_axis',(9.20925513359107E-14,0.707106781186535,-0.70710678118656)) ;
#37911=DIRECTION('center_axis',(-1.,1.75658099177411E-13,4.54195640846217E-14)) ;
#37912=DIRECTION('ref_axis',(9.20925513359107E-14,0.707106781186535,-0.70710678118656)) ;
#37913=DIRECTION('',(-1.,1.75658099177411E-13,4.54195640846217E-14)) ;
#37914=DIRECTION('center_axis',(-1.,1.75658099177411E-13,4.54195640846217E-14)) ;
#37915=DIRECTION('ref_axis',(9.20925513359107E-14,0.707106781186535,-0.70710678118656)) ;
#37916=DIRECTION('',(1.,-1.75658099177411E-13,-4.54195640846217E-14)) ;
#37917=DIRECTION('center_axis',(-1.75658099177411E-13,-1.,-1.66321791206623E-16)) ;
#37918=DIRECTION('ref_axis',(4.54195640846217E-14,-1.66321791214601E-16,
1.)) ;
#37919=DIRECTION('center_axis',(1.75658099177411E-13,1.,1.66321791206623E-16)) ;
#37920=DIRECTION('ref_axis',(4.54195640846217E-14,-1.66321791214601E-16,
1.)) ;
#37921=DIRECTION('',(-1.75658099177413E-13,-1.,-4.27988859368166E-14)) ;
#37922=DIRECTION('center_axis',(-1.75658099177411E-13,-1.,-1.66321791206623E-16)) ;
#37923=DIRECTION('ref_axis',(4.54195640846217E-14,-1.66321791214601E-16,
1.)) ;
#37924=DIRECTION('',(1.63182045051861E-13,1.,1.66321791207189E-16)) ;
#37925=DIRECTION('center_axis',(-1.75658099177411E-13,-1.,-1.66321791206623E-16)) ;
#37926=DIRECTION('ref_axis',(1.,-1.75658099177411E-13,-4.54195640846217E-14)) ;
#37927=DIRECTION('center_axis',(1.75658099177411E-13,1.,1.66321791206623E-16)) ;
#37928=DIRECTION('ref_axis',(1.,-1.75658099177411E-13,-4.54195640846217E-14)) ;
#37929=DIRECTION('',(-1.75658099177411E-13,-1.,-1.66321791206623E-16)) ;
#37930=DIRECTION('center_axis',(-1.75658099177411E-13,-1.,-1.66321791206623E-16)) ;
#37931=DIRECTION('ref_axis',(1.,-1.75658099177411E-13,-4.54195640846217E-14)) ;
#37932=DIRECTION('',(1.75658099177411E-13,1.,1.66321791206623E-16)) ;
#37933=DIRECTION('center_axis',(1.75658099177411E-13,1.,1.66321791206623E-16)) ;
#37934=DIRECTION('ref_axis',(4.54195640846217E-14,-1.66321791214601E-16,
1.)) ;
#37935=DIRECTION('center_axis',(-1.75658099177411E-13,-1.,-1.66321791206623E-16)) ;
#37936=DIRECTION('ref_axis',(4.54195640846217E-14,-1.66321791214601E-16,
1.)) ;
#37937=DIRECTION('',(1.75658099177411E-13,1.,1.66321791206623E-16)) ;
#37938=DIRECTION('center_axis',(1.75658099177411E-13,1.,1.66321791206623E-16)) ;
#37939=DIRECTION('ref_axis',(4.54195640846217E-14,-1.66321791214601E-16,
1.)) ;
#37940=DIRECTION('',(-1.75658099177411E-13,-1.,-1.66321791206623E-16)) ;
#37941=DIRECTION('center_axis',(1.75658099177411E-13,1.,1.66321791206623E-16)) ;
#37942=DIRECTION('ref_axis',(-1.,1.75658099177411E-13,4.54195640846217E-14)) ;
#37943=DIRECTION('center_axis',(-1.75658099177411E-13,-1.,-1.66321791206623E-16)) ;
#37944=DIRECTION('ref_axis',(-1.,1.75658099177411E-13,4.54195640846217E-14)) ;
#37945=DIRECTION('',(1.63182045051861E-13,1.,1.66321791207189E-16)) ;
#37946=DIRECTION('center_axis',(1.75658099177411E-13,1.,1.66321791206623E-16)) ;
#37947=DIRECTION('ref_axis',(-1.,1.75658099177411E-13,4.54195640846217E-14)) ;
#37948=DIRECTION('',(-1.75658099177411E-13,-1.,-1.66321791206623E-16)) ;
#37949=DIRECTION('center_axis',(1.,-1.75658099177411E-13,-4.54195640846217E-14)) ;
#37950=DIRECTION('ref_axis',(4.54195640846217E-14,-1.66321791214601E-16,
1.)) ;
#37951=DIRECTION('',(1.75658099177411E-13,1.,1.66321791206623E-16)) ;
#37952=DIRECTION('center_axis',(1.,-1.75658099177411E-13,-4.54195640846217E-14)) ;
#37953=DIRECTION('ref_axis',(-1.56325514861458E-13,-0.707106781186535,-0.70710678118656)) ;
#37954=DIRECTION('',(-4.54195640846217E-14,1.66321791214601E-16,-1.)) ;
#37955=DIRECTION('',(4.54195640846217E-14,-1.66321791214601E-16,1.)) ;
#37956=DIRECTION('center_axis',(-1.,1.75658099177411E-13,4.54195640846217E-14)) ;
#37957=DIRECTION('ref_axis',(-1.75658099177411E-13,-1.,-1.66321791206623E-16)) ;
#37958=DIRECTION('',(-1.75658099177411E-13,-1.,-1.66321791206623E-16)) ;
#37959=DIRECTION('center_axis',(-1.,1.75658099177411E-13,4.54195640846217E-14)) ;
#37960=DIRECTION('ref_axis',(-4.54195640846217E-14,1.66321791214601E-16,
-1.)) ;
#37961=DIRECTION('',(-4.54195640846217E-14,1.66321791214601E-16,-1.)) ;
#37962=DIRECTION('',(4.54195640846217E-14,-1.66321791214601E-16,1.)) ;
#37963=DIRECTION('center_axis',(1.75658099177411E-13,1.,1.66321791206623E-16)) ;
#37964=DIRECTION('ref_axis',(-4.54195640846217E-14,1.66321791214601E-16,
-1.)) ;
#37965=DIRECTION('center_axis',(-1.63182045051861E-13,-1.,0.)) ;
#37966=DIRECTION('ref_axis',(-4.54195640846217E-14,7.41165735269263E-27,
-1.)) ;
#37967=DIRECTION('',(1.75658099177411E-13,1.,1.66321791206623E-16)) ;
#37968=DIRECTION('center_axis',(1.63182045051861E-13,1.,0.)) ;
#37969=DIRECTION('ref_axis',(-4.54195640846217E-14,7.41165735269263E-27,
-1.)) ;
#37970=DIRECTION('',(1.75658099177411E-13,1.,1.66321791206623E-16)) ;
#37971=DIRECTION('center_axis',(-1.63182045051861E-13,-1.,-1.66321791207189E-16)) ;
#37972=DIRECTION('ref_axis',(-0.707106781186566,1.15504737890484E-13,-0.707106781186529)) ;
#37973=DIRECTION('center_axis',(-1.63182045051861E-13,-1.,0.)) ;
#37974=DIRECTION('ref_axis',(-0.707106781186566,1.15387130624063E-13,-0.707106781186529)) ;
#37975=DIRECTION('',(1.63182045051861E-13,1.,1.66321791207189E-16)) ;
#37976=DIRECTION('center_axis',(-1.63182045051861E-13,-1.,0.)) ;
#37977=DIRECTION('ref_axis',(-0.707106781186566,1.15387130624063E-13,-0.707106781186529)) ;
#37978=DIRECTION('',(-1.63182045051861E-13,-1.,-1.66321791207189E-16)) ;
#37979=DIRECTION('center_axis',(1.75658099177411E-13,1.,1.66321791206623E-16)) ;
#37980=DIRECTION('ref_axis',(-4.54195640846217E-14,1.66321791214601E-16,
-1.)) ;
#37981=DIRECTION('',(-1.,1.75658099177411E-13,4.54195640846217E-14)) ;
#37982=DIRECTION('',(1.,-1.75658099177411E-13,-4.54195640846217E-14)) ;
#37983=DIRECTION('',(-4.54195640846217E-14,1.66321791214601E-16,-1.)) ;
#37984=DIRECTION('center_axis',(1.75658099177411E-13,1.,1.66321791206623E-16)) ;
#37985=DIRECTION('ref_axis',(-1.,1.75658099177411E-13,4.54195640846217E-14)) ;
#37986=DIRECTION('',(-4.54195640846217E-14,1.66321791214601E-16,-1.)) ;
#37987=DIRECTION('',(1.,-1.75658099177411E-13,-4.54195640846217E-14)) ;
#37988=DIRECTION('',(-4.54195640846217E-14,1.66321791214601E-16,-1.)) ;
#37989=DIRECTION('center_axis',(1.75658099177411E-13,1.,1.66321791206623E-16)) ;
#37990=DIRECTION('ref_axis',(-1.,1.75658099177411E-13,4.54195640846217E-14)) ;
#37991=DIRECTION('',(-4.54195640846217E-14,1.66321791214601E-16,-1.)) ;
#37992=DIRECTION('',(1.,-1.75658099177411E-13,-4.54195640846217E-14)) ;
#37993=DIRECTION('',(2.71407300257853E-29,1.66321791206623E-16,-1.)) ;
#37994=DIRECTION('',(1.,-1.75658099177411E-13,0.)) ;
#37995=DIRECTION('',(-4.54195640846217E-14,1.66321791214601E-16,-1.)) ;
#37996=DIRECTION('',(-1.,1.75658099177411E-13,4.54195640846217E-14)) ;
#37997=DIRECTION('',(-4.54195640846217E-14,1.66321791214601E-16,-1.)) ;
#37998=DIRECTION('',(-1.,1.75658099177411E-13,4.54195640846217E-14)) ;
#37999=DIRECTION('',(4.54195640846217E-14,-1.66321791214601E-16,1.)) ;
#38000=DIRECTION('',(-1.,1.75658099177411E-13,4.54195640846217E-14)) ;
#38001=DIRECTION('',(4.54195640846217E-14,-1.66321791214601E-16,1.)) ;
#38002=DIRECTION('center_axis',(1.75658099177411E-13,1.,1.66321791206623E-16)) ;
#38003=DIRECTION('ref_axis',(-0.707106781186586,1.24326640365114E-13,-0.707106781186509)) ;
#38004=DIRECTION('',(-1.,1.75658099177411E-13,4.54195640846217E-14)) ;
#38005=DIRECTION('center_axis',(1.75658099177411E-13,1.,1.66321791206623E-16)) ;
#38006=DIRECTION('ref_axis',(0.707106781186528,-1.24091425832262E-13,-0.707106781186567)) ;
#38007=DIRECTION('',(-4.54195640846217E-14,1.66321791214601E-16,-1.)) ;
#38008=DIRECTION('',(-1.,1.75658099177411E-13,4.54195640846217E-14)) ;
#38009=DIRECTION('',(-4.54195640846217E-14,1.66321791214601E-16,-1.)) ;
#38010=DIRECTION('',(1.,-1.75658099177411E-13,-4.54195640846217E-14)) ;
#38011=DIRECTION('',(-4.54195640846217E-14,1.66321791214601E-16,-1.)) ;
#38012=DIRECTION('center_axis',(1.75658099177411E-13,1.,1.66321791206623E-16)) ;
#38013=DIRECTION('ref_axis',(1.,-1.75658099177411E-13,-4.54195640846217E-14)) ;
#38014=DIRECTION('',(1.,-1.75658099177411E-13,-4.54195640846217E-14)) ;
#38015=DIRECTION('',(4.54195640846217E-14,-1.66321791214601E-16,1.)) ;
#38016=DIRECTION('',(-1.,1.75658099177411E-13,4.54195640846217E-14)) ;
#38017=DIRECTION('',(-4.54195640846217E-14,1.66321791214601E-16,-1.)) ;
#38018=DIRECTION('',(1.,-1.75658099177411E-13,-4.54195640846217E-14)) ;
#38019=DIRECTION('',(4.54195640846217E-14,-1.66321791214601E-16,1.)) ;
#38020=DIRECTION('',(-1.,1.75658099177411E-13,4.54195640846217E-14)) ;
#38021=DIRECTION('',(-4.54195640846217E-14,1.66321791214601E-16,-1.)) ;
#38022=DIRECTION('',(1.,-1.75658099177411E-13,-4.54195640846217E-14)) ;
#38023=DIRECTION('',(4.54195640846217E-14,-1.66321791214601E-16,1.)) ;
#38024=DIRECTION('',(-1.,1.75658099177411E-13,4.54195640846217E-14)) ;
#38025=DIRECTION('',(-4.54195640846217E-14,1.66321791214601E-16,-1.)) ;
#38026=DIRECTION('center_axis',(1.75658099177411E-13,1.,1.66321791206623E-16)) ;
#38027=DIRECTION('ref_axis',(0.99999997726804,-1.75658059720776E-13,-0.000213222701069828)) ;
#38028=DIRECTION('center_axis',(1.,-1.75658099177411E-13,-4.54195640846217E-14)) ;
#38029=DIRECTION('ref_axis',(9.20925513359107E-14,0.707106781186535,-0.70710678118656)) ;
#38030=DIRECTION('center_axis',(1.,-1.63182045051861E-13,0.)) ;
#38031=DIRECTION('ref_axis',(1.15387130624058E-13,0.707106781186535,-0.70710678118656)) ;
#38032=DIRECTION('',(1.,-1.75658099177411E-13,-4.54195640846217E-14)) ;
#38033=DIRECTION('center_axis',(1.,-1.75658099177411E-13,-4.54195640846217E-14)) ;
#38034=DIRECTION('ref_axis',(9.20925513359107E-14,0.707106781186535,-0.70710678118656)) ;
#38035=DIRECTION('',(-1.,1.75658099177411E-13,4.54195640846217E-14)) ;
#38036=DIRECTION('center_axis',(-1.75658099177411E-13,-1.,-1.66321791206623E-16)) ;
#38037=DIRECTION('ref_axis',(4.54195640846217E-14,-1.66321791214601E-16,
1.)) ;
#38038=DIRECTION('',(1.,-1.75658099177411E-13,-4.54195640846217E-14)) ;
#38039=DIRECTION('',(4.54195640846217E-14,-1.66321791214601E-16,1.)) ;
#38040=DIRECTION('',(-1.,1.75658099177411E-13,0.)) ;
#38041=DIRECTION('',(-2.71407300257853E-29,-1.66321791206623E-16,1.)) ;
#38042=DIRECTION('',(-4.54195640846217E-14,1.66321791214601E-16,-1.)) ;
#38043=DIRECTION('center_axis',(-1.75658099177411E-13,-1.,-1.66321791206623E-16)) ;
#38044=DIRECTION('ref_axis',(1.,-1.75658099177411E-13,-4.54195640846217E-14)) ;
#38045=DIRECTION('',(4.54195640846217E-14,-1.66321791214601E-16,1.)) ;
#38046=DIRECTION('',(-1.,1.75658099177411E-13,4.54195640846217E-14)) ;
#38047=DIRECTION('',(-4.54195640846217E-14,1.66321791214601E-16,-1.)) ;
#38048=DIRECTION('center_axis',(-1.75658099177411E-13,-1.,-1.66321791206623E-16)) ;
#38049=DIRECTION('ref_axis',(1.,-1.75658099177411E-13,-4.54195640846217E-14)) ;
#38050=DIRECTION('',(4.54195640846217E-14,-1.66321791214601E-16,1.)) ;
#38051=DIRECTION('',(-1.,1.75658099177411E-13,4.54195640846217E-14)) ;
#38052=DIRECTION('',(4.54195640846217E-14,-1.66321791214601E-16,1.)) ;
#38053=DIRECTION('center_axis',(-1.75658099177411E-13,-1.,-1.66321791206623E-16)) ;
#38054=DIRECTION('ref_axis',(-1.,1.75658099177411E-13,4.54195640846217E-14)) ;
#38055=DIRECTION('',(4.54195640846217E-14,-1.66321791214601E-16,1.)) ;
#38056=DIRECTION('',(-1.,1.75658099177411E-13,4.54195640846217E-14)) ;
#38057=DIRECTION('',(4.54195640846217E-14,-1.66321791214601E-16,1.)) ;
#38058=DIRECTION('center_axis',(-1.75658099177411E-13,-1.,-1.66321791206623E-16)) ;
#38059=DIRECTION('ref_axis',(-1.,1.75658099177411E-13,4.54195640846217E-14)) ;
#38060=DIRECTION('',(4.54195640846217E-14,-1.66321791214601E-16,1.)) ;
#38061=DIRECTION('center_axis',(-1.75658099177411E-13,-1.,-1.66321791206623E-16)) ;
#38062=DIRECTION('ref_axis',(1.,-1.75658099177411E-13,-4.54195640846217E-14)) ;
#38063=DIRECTION('',(1.,-1.75658099177411E-13,-4.54195640846217E-14)) ;
#38064=DIRECTION('',(-4.54195640846217E-14,1.66321791214601E-16,-1.)) ;
#38065=DIRECTION('',(-1.,1.75658099177411E-13,4.54195640846217E-14)) ;
#38066=DIRECTION('',(4.54195640846217E-14,-1.66321791214601E-16,1.)) ;
#38067=DIRECTION('',(1.,-1.75658099177411E-13,-4.54195640846217E-14)) ;
#38068=DIRECTION('',(-4.54195640846217E-14,1.66321791214601E-16,-1.)) ;
#38069=DIRECTION('',(-1.,1.75658099177411E-13,4.54195640846217E-14)) ;
#38070=DIRECTION('',(4.54195640846217E-14,-1.66321791214601E-16,1.)) ;
#38071=DIRECTION('',(1.,-1.75658099177411E-13,-4.54195640846217E-14)) ;
#38072=DIRECTION('',(-4.54195640846217E-14,1.66321791214601E-16,-1.)) ;
#38073=DIRECTION('',(-1.,1.75658099177411E-13,4.54195640846217E-14)) ;
#38074=DIRECTION('',(4.54195640846217E-14,-1.66321791214601E-16,1.)) ;
#38075=DIRECTION('',(1.,-1.75658099177411E-13,-4.54195640846217E-14)) ;
#38076=DIRECTION('',(-4.54195640846217E-14,1.66321791214601E-16,-1.)) ;
#38077=DIRECTION('',(-1.,1.75658099177411E-13,4.54195640846217E-14)) ;
#38078=DIRECTION('',(4.54195640846217E-14,-1.66321791214601E-16,1.)) ;
#38079=DIRECTION('center_axis',(-1.75658099177411E-13,-1.,-1.66321791206623E-16)) ;
#38080=DIRECTION('ref_axis',(0.00363593456997526,-8.05002047109562E-16,
0.999993389968055)) ;
#38081=DIRECTION('',(2.92157696951376E-29,1.66321791206623E-16,-1.)) ;
#38082=DIRECTION('center_axis',(-1.75658099177411E-13,-1.,-1.66321791206623E-16)) ;
#38083=DIRECTION('ref_axis',(0.707106781186522,-1.24091425832261E-13,-0.707106781186573)) ;
#38084=DIRECTION('',(-1.,1.75658099177411E-13,6.34413156928661E-16)) ;
#38085=DIRECTION('center_axis',(-1.75658099177411E-13,-1.,-1.66321791206623E-16)) ;
#38086=DIRECTION('ref_axis',(-0.707106781186573,1.24326640365112E-13,-0.707106781186523)) ;
#38087=DIRECTION('',(-2.92157696951376E-29,-1.66321791206623E-16,1.)) ;
#38088=DIRECTION('center_axis',(-1.75658099177411E-13,-1.,-1.66321791206623E-16)) ;
#38089=DIRECTION('ref_axis',(-0.707106781186573,1.2409142583227E-13,0.707106781186523)) ;
#38090=DIRECTION('',(1.,-1.75658099177411E-13,-3.1720657846433E-16)) ;
#38091=DIRECTION('center_axis',(-1.75658099177411E-13,-1.,-1.66321791206623E-16)) ;
#38092=DIRECTION('ref_axis',(0.707106781186522,-1.24326640365103E-13,0.707106781186573)) ;
#38093=DIRECTION('',(1.,-1.75658099177411E-13,-4.54195640846217E-14)) ;
#38094=DIRECTION('',(-4.54195640846217E-14,1.66321791214601E-16,-1.)) ;
#38095=DIRECTION('',(1.,-1.75658099177411E-13,-4.54195640846217E-14)) ;
#38096=DIRECTION('',(4.54195640846217E-14,-1.66321791214601E-16,1.)) ;
#38097=DIRECTION('',(1.,-1.75658099177411E-13,-4.54195640846217E-14)) ;
#38098=DIRECTION('',(4.54195640846217E-14,-1.66321791214601E-16,1.)) ;
#38099=DIRECTION('center_axis',(-1.75658099177411E-13,-1.,-1.66321791206623E-16)) ;
#38100=DIRECTION('ref_axis',(0.70710678118651,-1.24091425832259E-13,-0.707106781186585)) ;
#38101=DIRECTION('',(1.,-1.75658099177411E-13,-4.54195640846217E-14)) ;
#38102=DIRECTION('center_axis',(-1.75658099177411E-13,-1.,-1.66321791206623E-16)) ;
#38103=DIRECTION('ref_axis',(-0.707106781186573,1.24326640365112E-13,-0.707106781186522)) ;
#38104=DIRECTION('',(-4.54195640846217E-14,1.66321791214601E-16,-1.)) ;
#38105=DIRECTION('center_axis',(1.75658099177411E-13,1.,1.66321791206623E-16)) ;
#38106=DIRECTION('ref_axis',(-4.54195640846217E-14,1.66321791214601E-16,
-1.)) ;
#38107=DIRECTION('',(4.54195640846217E-14,-1.66321791214601E-16,1.)) ;
#38108=DIRECTION('',(-1.,1.75658099177411E-13,0.)) ;
#38109=DIRECTION('',(-2.71407300257853E-29,-1.66321791206623E-16,1.)) ;
#38110=DIRECTION('',(1.,-1.75658099177411E-13,-4.54195640846217E-14)) ;
#38111=DIRECTION('',(4.54195640846217E-14,-1.66321791214601E-16,1.)) ;
#38112=DIRECTION('center_axis',(1.75658099177411E-13,1.,1.66321791206623E-16)) ;
#38113=DIRECTION('ref_axis',(-1.,1.75658099177411E-13,4.54195640846217E-14)) ;
#38114=DIRECTION('',(4.54195640846217E-14,-1.66321791214601E-16,1.)) ;
#38115=DIRECTION('',(-1.,1.75658099177411E-13,4.54195640846217E-14)) ;
#38116=DIRECTION('',(4.54195640846217E-14,-1.66321791214601E-16,1.)) ;
#38117=DIRECTION('center_axis',(1.75658099177411E-13,1.,1.66321791206623E-16)) ;
#38118=DIRECTION('ref_axis',(-1.,1.75658099177411E-13,4.54195640846217E-14)) ;
#38119=DIRECTION('',(-4.54195640846217E-14,1.66321791214601E-16,-1.)) ;
#38120=DIRECTION('',(1.,-1.75658099177411E-13,-4.54195640846217E-14)) ;
#38121=DIRECTION('',(1.,-1.75658099177411E-13,-4.54195640846217E-14)) ;
#38122=DIRECTION('center_axis',(-1.75658099177411E-13,-1.,-1.66321791206623E-16)) ;
#38123=DIRECTION('ref_axis',(1.,-1.75658099177411E-13,-4.54195640846217E-14)) ;
#38124=DIRECTION('',(1.,-1.75658099177411E-13,-4.54195640846217E-14)) ;
#38125=DIRECTION('',(-4.54195640846217E-14,1.66321791214601E-16,-1.)) ;
#38126=DIRECTION('',(-1.,1.75658099177411E-13,4.54195640846217E-14)) ;
#38127=DIRECTION('',(4.54195640846217E-14,-1.66321791214601E-16,1.)) ;
#38128=DIRECTION('',(1.,-1.75658099177411E-13,-4.54195640846217E-14)) ;
#38129=DIRECTION('',(-4.54195640846217E-14,1.66321791214601E-16,-1.)) ;
#38130=DIRECTION('',(-1.,1.75658099177411E-13,4.54195640846217E-14)) ;
#38131=DIRECTION('',(4.54195640846217E-14,-1.66321791214601E-16,1.)) ;
#38132=DIRECTION('',(1.,-1.75658099177411E-13,-4.54195640846217E-14)) ;
#38133=DIRECTION('',(-4.54195640846217E-14,1.66321791214601E-16,-1.)) ;
#38134=DIRECTION('',(-1.,1.75658099177411E-13,4.54195640846217E-14)) ;
#38135=DIRECTION('',(4.54195640846217E-14,-1.66321791214601E-16,1.)) ;
#38136=DIRECTION('center_axis',(1.75658099177411E-13,1.,1.66321791206623E-16)) ;
#38137=DIRECTION('ref_axis',(1.,-1.75658099177411E-13,-4.54195640846217E-14)) ;
#38138=DIRECTION('',(1.,-1.75658099177411E-13,-4.54195640846217E-14)) ;
#38139=DIRECTION('center_axis',(1.75658099177411E-13,1.,1.66321791206623E-16)) ;
#38140=DIRECTION('ref_axis',(-8.60220061280517E-14,1.66321791221733E-16,
-1.)) ;
#38141=DIRECTION('',(-4.54195640846217E-14,1.66321791214602E-16,-1.)) ;
#38142=DIRECTION('',(-1.,1.75658099177411E-13,4.54195640846217E-14)) ;
#38143=DIRECTION('',(4.54195640846217E-14,-1.66321791214601E-16,1.)) ;
#38144=DIRECTION('center_axis',(-1.75658099177411E-13,-1.,-1.66321791206623E-16)) ;
#38145=DIRECTION('ref_axis',(0.99999997726804,-1.75658059720776E-13,-0.000213222701069828)) ;
#38146=DIRECTION('center_axis',(-1.75658099177411E-13,-1.,-1.66321791206623E-16)) ;
#38147=DIRECTION('ref_axis',(4.54195640846217E-14,-1.66321791214601E-16,
1.)) ;
#38148=DIRECTION('',(1.,-1.75658099177411E-13,-4.54195640846217E-14)) ;
#38149=DIRECTION('',(4.54195640846217E-14,-1.66321791214601E-16,1.)) ;
#38150=DIRECTION('center_axis',(-1.75658099177411E-13,-1.,-1.66321791206623E-16)) ;
#38151=DIRECTION('ref_axis',(1.,-1.75658099177411E-13,-4.54195640846217E-14)) ;
#38152=DIRECTION('',(-4.54195640846217E-14,1.66321791214601E-16,-1.)) ;
#38153=DIRECTION('',(-1.,1.75658099177411E-13,4.54195640846217E-14)) ;
#38154=DIRECTION('',(4.54195640846217E-14,-1.66321791214601E-16,1.)) ;
#38155=DIRECTION('center_axis',(-1.75658099177411E-13,-1.,-1.66321791206623E-16)) ;
#38156=DIRECTION('ref_axis',(1.,-1.75658099177411E-13,-4.54195640846217E-14)) ;
#38157=DIRECTION('',(4.54195640846217E-14,-1.66321791214601E-16,1.)) ;
#38158=DIRECTION('',(1.,-1.75658099177411E-13,-4.54195640846217E-14)) ;
#38159=DIRECTION('',(4.54195640846217E-14,-1.66321791214601E-16,1.)) ;
#38160=DIRECTION('center_axis',(-1.75658099177411E-13,-1.,-1.66321791206623E-16)) ;
#38161=DIRECTION('ref_axis',(1.,-1.75658099177411E-13,-4.54195640846217E-14)) ;
#38162=DIRECTION('',(-4.54195640846217E-14,1.66321791214601E-16,-1.)) ;
#38163=DIRECTION('',(1.,-1.75658099177411E-13,-4.54195640846217E-14)) ;
#38164=DIRECTION('',(4.54195640846217E-14,-1.66321791214601E-16,1.)) ;
#38165=DIRECTION('center_axis',(-1.75658099177411E-13,-1.,-1.66321791206623E-16)) ;
#38166=DIRECTION('ref_axis',(1.,-1.75658099177411E-13,-4.54195640846217E-14)) ;
#38167=DIRECTION('',(-4.54195640846217E-14,1.66321791214601E-16,-1.)) ;
#38168=DIRECTION('',(1.,-1.75658099177411E-13,-4.54195640846217E-14)) ;
#38169=DIRECTION('',(2.71407300257853E-29,1.66321791206623E-16,-1.)) ;
#38170=DIRECTION('',(1.,-1.75658099177411E-13,0.)) ;
#38171=DIRECTION('',(-4.54195640846217E-14,1.66321791214601E-16,-1.)) ;
#38172=DIRECTION('',(-1.,1.75658099177411E-13,4.54195640846217E-14)) ;
#38173=DIRECTION('center_axis',(1.75658099177411E-13,1.,1.66321791206623E-16)) ;
#38174=DIRECTION('ref_axis',(0.707106781186522,-1.24326640365103E-13,0.707106781186573)) ;
#38175=DIRECTION('',(1.,-1.75658099177411E-13,-3.1720657846433E-16)) ;
#38176=DIRECTION('center_axis',(1.75658099177411E-13,1.,1.66321791206623E-16)) ;
#38177=DIRECTION('ref_axis',(-0.707106781186548,1.24091425832265E-13,0.707106781186548)) ;
#38178=DIRECTION('',(-2.92157696951376E-29,-1.66321791206623E-16,1.)) ;
#38179=DIRECTION('center_axis',(1.75658099177411E-13,1.,1.66321791206623E-16)) ;
#38180=DIRECTION('ref_axis',(-0.707106781186548,1.24326640365108E-13,-0.707106781186548)) ;
#38181=DIRECTION('',(-1.,1.75658099177411E-13,6.34413156928661E-16)) ;
#38182=DIRECTION('center_axis',(1.75658099177411E-13,1.,1.66321791206623E-16)) ;
#38183=DIRECTION('ref_axis',(0.707106781186522,-1.24091425832261E-13,-0.707106781186573)) ;
#38184=DIRECTION('',(2.92157696951376E-29,1.66321791206623E-16,-1.)) ;
#38185=DIRECTION('center_axis',(-1.75658099177411E-13,-1.,-1.66321791206623E-16)) ;
#38186=DIRECTION('ref_axis',(-1.,1.75658099177411E-13,4.54195640846217E-14)) ;
#38187=DIRECTION('',(-1.,1.75658099177411E-13,4.54195640846217E-14)) ;
#38188=DIRECTION('center_axis',(-1.75658099177411E-13,-1.,-1.66321791206623E-16)) ;
#38189=DIRECTION('ref_axis',(-4.54195640846217E-14,1.66321791214601E-16,
-1.)) ;
#38190=DIRECTION('',(-4.54195640846217E-14,1.66321791214602E-16,-1.)) ;
#38191=DIRECTION('',(1.,-1.75658099177411E-13,-4.54195640846217E-14)) ;
#38192=DIRECTION('',(4.54195640846217E-14,-1.66321791214601E-16,1.)) ;
#38193=DIRECTION('',(1.,-1.75658099177411E-13,-4.54195640846217E-14)) ;
#38194=DIRECTION('',(4.54195640846217E-14,-1.66321791214601E-16,1.)) ;
#38195=DIRECTION('',(-1.,1.75658099177411E-13,4.54195640846217E-14)) ;
#38196=DIRECTION('',(-4.54195640846217E-14,1.66321791214601E-16,-1.)) ;
#38197=DIRECTION('',(1.,-1.75658099177411E-13,-4.54195640846217E-14)) ;
#38198=DIRECTION('',(4.54195640846217E-14,-1.66321791214601E-16,1.)) ;
#38199=DIRECTION('',(-1.,1.75658099177411E-13,4.54195640846217E-14)) ;
#38200=DIRECTION('',(-4.54195640846217E-14,1.66321791214601E-16,-1.)) ;
#38201=DIRECTION('',(1.,-1.75658099177411E-13,-4.54195640846217E-14)) ;
#38202=DIRECTION('',(4.54195640846217E-14,-1.66321791214601E-16,1.)) ;
#38203=DIRECTION('',(-1.,1.75658099177411E-13,4.54195640846217E-14)) ;
#38204=DIRECTION('',(-4.54195640846217E-14,1.66321791214601E-16,-1.)) ;
#38205=DIRECTION('',(1.,-1.75658099177411E-13,-4.54195640846217E-14)) ;
#38206=DIRECTION('',(4.54195640846217E-14,-1.66321791214601E-16,1.)) ;
#38207=DIRECTION('',(-1.,1.75658099177411E-13,4.54195640846217E-14)) ;
#38208=DIRECTION('',(-4.54195640846217E-14,1.66321791214601E-16,-1.)) ;
#38209=DIRECTION('center_axis',(1.75658099177411E-13,1.,1.66321791206623E-16)) ;
#38210=DIRECTION('ref_axis',(0.00363593456997526,-8.05002047109562E-16,
0.999993389968055)) ;
#38211=DIRECTION('center_axis',(1.75658099177411E-13,1.,1.66321791206623E-16)) ;
#38212=DIRECTION('ref_axis',(0.00363593456997526,-8.05002047109562E-16,
0.999993389968055)) ;
#38213=DIRECTION('center_axis',(-1.,1.63182045051861E-13,0.)) ;
#38214=DIRECTION('ref_axis',(-1.63182045051861E-13,-1.,0.)) ;
#38215=DIRECTION('center_axis',(-1.,1.63182045051861E-13,0.)) ;
#38216=DIRECTION('ref_axis',(2.71407300258777E-29,1.66321791207189E-16,
-1.)) ;
#38217=DIRECTION('',(1.63182045051861E-13,1.,1.66321791207189E-16)) ;
#38218=DIRECTION('',(0.,0.,-1.)) ;
#38219=DIRECTION('',(1.63182045051861E-13,1.,1.66321791207189E-16)) ;
#38220=DIRECTION('',(1.63182045051861E-13,1.,0.)) ;
#38221=DIRECTION('center_axis',(-1.,1.63182045051861E-13,0.)) ;
#38222=DIRECTION('ref_axis',(-1.63182045051861E-13,-1.,0.)) ;
#38223=DIRECTION('',(0.,0.,-1.)) ;
#38224=DIRECTION('',(0.,0.,1.)) ;
#38225=DIRECTION('',(1.63182045051861E-13,1.,0.)) ;
#38226=DIRECTION('',(1.63182045051861E-13,1.,1.66321791207189E-16)) ;
#38227=DIRECTION('',(2.71407300257853E-29,1.66321791206623E-16,-1.)) ;
#38228=DIRECTION('',(1.63182045051861E-13,1.,0.)) ;
#38229=DIRECTION('center_axis',(1.,-1.75658099177411E-13,-4.54195640846217E-14)) ;
#38230=DIRECTION('ref_axis',(-4.54195640846217E-14,1.66321791214601E-16,
-1.)) ;
#38231=DIRECTION('center_axis',(1.,-1.75658099177411E-13,-4.54195640846217E-14)) ;
#38232=DIRECTION('ref_axis',(-4.54195640846217E-14,1.66321791214601E-16,
-1.)) ;
#38233=DIRECTION('',(1.,-1.75658099177411E-13,-4.54195640846217E-14)) ;
#38234=DIRECTION('center_axis',(1.,-1.75658099177411E-13,-4.54195640846217E-14)) ;
#38235=DIRECTION('ref_axis',(-4.54195640846217E-14,1.66321791214601E-16,
-1.)) ;
#38236=DIRECTION('',(1.,-1.75658099177411E-13,-4.54195640846217E-14)) ;
#38237=DIRECTION('center_axis',(-1.,1.75658099177411E-13,4.54195640846217E-14)) ;
#38238=DIRECTION('ref_axis',(1.75658099177411E-13,1.,1.66321791206623E-16)) ;
#38239=DIRECTION('center_axis',(1.,-1.75658099177411E-13,-4.54195640846217E-14)) ;
#38240=DIRECTION('ref_axis',(-1.75658099177411E-13,-1.,-1.66321791206623E-16)) ;
#38241=DIRECTION('center_axis',(-1.,1.75658099177411E-13,4.54195640846217E-14)) ;
#38242=DIRECTION('ref_axis',(-4.54195640846217E-14,1.66321791214601E-16,
-1.)) ;
#38243=DIRECTION('',(1.,-1.75658099177411E-13,-4.54195640846217E-14)) ;
#38244=DIRECTION('center_axis',(1.,-1.75658099177411E-13,-4.54195640846217E-14)) ;
#38245=DIRECTION('ref_axis',(-1.56325514861458E-13,-0.707106781186535,-0.70710678118656)) ;
#38246=DIRECTION('center_axis',(1.,-1.75658099177411E-13,-4.54195640846217E-14)) ;
#38247=DIRECTION('ref_axis',(-1.56325514861458E-13,-0.707106781186535,-0.70710678118656)) ;
#38248=DIRECTION('',(1.,-1.75658099177411E-13,-4.54195640846217E-14)) ;
#38249=DIRECTION('center_axis',(1.,-1.63182045051861E-13,0.)) ;
#38250=DIRECTION('ref_axis',(-1.15387130624058E-13,-0.707106781186535,-0.70710678118656)) ;
#38251=DIRECTION('center_axis',(1.,-1.75658099177411E-13,-4.54195640846217E-14)) ;
#38252=DIRECTION('ref_axis',(-4.54195640846217E-14,1.66321791214601E-16,
-1.)) ;
#38253=DIRECTION('',(-1.75658099177411E-13,-1.,0.)) ;
#38254=DIRECTION('center_axis',(-4.54195640846217E-14,1.66321791214601E-16,
-1.)) ;
#38255=DIRECTION('ref_axis',(-1.75658099177411E-13,-1.,-1.66321791206623E-16)) ;
#38256=DIRECTION('',(-1.,-4.97379915027563E-13,5.10702591322944E-14)) ;
#38257=DIRECTION('',(-1.75658099177411E-13,-1.,-1.66321791206623E-16)) ;
#38258=DIRECTION('',(1.,-1.75658099177411E-13,-4.54195640846217E-14)) ;
#38259=DIRECTION('center_axis',(1.75658099177411E-13,1.,1.66321791206623E-16)) ;
#38260=DIRECTION('ref_axis',(-4.54195640846217E-14,1.66321791214601E-16,
-1.)) ;
#38261=DIRECTION('',(1.,-1.75658099177411E-13,0.)) ;
#38262=DIRECTION('',(4.54195640846217E-14,-1.66321791214601E-16,1.)) ;
#38263=DIRECTION('',(-1.,0.,1.46549439249113E-13)) ;
#38264=DIRECTION('center_axis',(0.,0.,-1.)) ;
#38265=DIRECTION('ref_axis',(1.63182045051861E-13,1.,0.)) ;
#38266=DIRECTION('',(-1.,1.63182045051861E-13,0.)) ;
#38267=DIRECTION('',(-1.75658099177411E-13,-1.,0.)) ;
#38268=DIRECTION('center_axis',(1.63182045051861E-13,1.,0.)) ;
#38269=DIRECTION('ref_axis',(0.,0.,1.)) ;
#38270=DIRECTION('',(-1.,1.63182045051861E-13,4.54195640846217E-14)) ;
#38271=DIRECTION('',(0.,0.,1.)) ;
#38272=DIRECTION('',(4.54195640846217E-14,-7.41165735269262E-27,1.)) ;
#38273=DIRECTION('center_axis',(-1.,1.63182045051861E-13,0.)) ;
#38274=DIRECTION('ref_axis',(-1.63182045051861E-13,-1.,0.)) ;
#38275=DIRECTION('',(1.63182045051861E-13,1.,1.66321791207189E-16)) ;
#38276=DIRECTION('',(1.63182045051861E-13,1.,1.66321791207189E-16)) ;
#38277=DIRECTION('center_axis',(-1.,1.63182045051861E-13,0.)) ;
#38278=DIRECTION('ref_axis',(-1.63182045051861E-13,-1.,-1.66321791206623E-16)) ;
#38279=DIRECTION('',(1.63182045051861E-13,1.,0.)) ;
#38280=DIRECTION('center_axis',(0.,0.,-1.)) ;
#38281=DIRECTION('ref_axis',(1.63182045051861E-13,1.,0.)) ;
#38282=DIRECTION('center_axis',(0.,0.,-1.)) ;
#38283=DIRECTION('ref_axis',(1.63182045051861E-13,1.,0.)) ;
#38284=DIRECTION('',(-1.75658099177411E-13,-1.,0.)) ;
#38285=DIRECTION('center_axis',(1.63182045051861E-13,1.,0.)) ;
#38286=DIRECTION('ref_axis',(0.,0.,1.)) ;
#38287=DIRECTION('',(1.,-1.63182045051861E-13,-4.54195640846217E-14)) ;
#38288=DIRECTION('',(-4.54195640846217E-14,7.41165735269262E-27,-1.)) ;
#38289=DIRECTION('',(1.,-1.63182045051861E-13,0.)) ;
#38290=DIRECTION('center_axis',(0.,0.,-1.)) ;
#38291=DIRECTION('ref_axis',(1.63182045051861E-13,1.,0.)) ;
#38292=DIRECTION('',(-1.75658099177411E-13,-1.,0.)) ;
#38293=DIRECTION('center_axis',(4.54195640846217E-14,-1.66321791214601E-16,
1.)) ;
#38294=DIRECTION('ref_axis',(-0.707106781186698,-0.707106781186397,3.19988744963529E-14)) ;
#38295=DIRECTION('center_axis',(-4.54195640846217E-14,1.66321791214601E-16,
-1.)) ;
#38296=DIRECTION('ref_axis',(-0.707106781186698,-0.707106781186397,3.19988744963529E-14)) ;
#38297=DIRECTION('',(4.54195640846217E-14,-1.66321791214601E-16,1.)) ;
#38298=DIRECTION('center_axis',(4.54195640846217E-14,-1.66321791214601E-16,
1.)) ;
#38299=DIRECTION('ref_axis',(-0.707106781186698,-0.707106781186397,3.19988744963529E-14)) ;
#38300=DIRECTION('center_axis',(1.,-1.75658099177411E-13,-4.54195640846217E-14)) ;
#38301=DIRECTION('ref_axis',(4.54195640846217E-14,-1.66321791214601E-16,
1.)) ;
#38302=DIRECTION('',(1.75658099177411E-13,1.,1.66321791206623E-16)) ;
#38303=DIRECTION('',(-4.54195640846217E-14,1.66321791214601E-16,-1.)) ;
#38304=DIRECTION('',(1.75658099177411E-13,1.,1.66321791206623E-16)) ;
#38305=DIRECTION('center_axis',(-4.54195640846217E-14,1.66321791214601E-16,
-1.)) ;
#38306=DIRECTION('ref_axis',(0.707106781186409,-0.707106781186686,-3.22340890291936E-14)) ;
#38307=DIRECTION('center_axis',(-3.99680288865058E-14,7.09974814698903E-27,
-1.)) ;
#38308=DIRECTION('ref_axis',(1.,-1.42108547152021E-13,-3.99680288865058E-14)) ;
#38309=DIRECTION('center_axis',(4.54195640846217E-14,-1.66321791214601E-16,
1.)) ;
#38310=DIRECTION('ref_axis',(0.707106781186409,-0.707106781186686,-3.22340890291936E-14)) ;
#38311=DIRECTION('',(-4.54195640846217E-14,1.66321791214601E-16,-1.)) ;
#38312=DIRECTION('center_axis',(-1.75658099177411E-13,-1.,-1.66321791206623E-16)) ;
#38313=DIRECTION('ref_axis',(0.,0.,-1.)) ;
#38314=DIRECTION('center_axis',(1.,-1.77635683940023E-13,-3.55271579388434E-14)) ;
#38315=DIRECTION('ref_axis',(3.55271579388434E-14,0.,1.)) ;
#38316=DIRECTION('center_axis',(-1.75658099177411E-13,-1.,-1.66321791206623E-16)) ;
#38317=DIRECTION('ref_axis',(-0.707106781186586,1.24326640365114E-13,-0.707106781186509)) ;
#38318=DIRECTION('center_axis',(1.,-1.75658099177411E-13,-4.54195640846217E-14)) ;
#38319=DIRECTION('ref_axis',(-9.20925513359094E-14,-0.707106781186529,0.707106781186566)) ;
#38320=DIRECTION('center_axis',(1.,-2.13162820728042E-13,-3.55271156371924E-14)) ;
#38321=DIRECTION('ref_axis',(3.55271156371924E-14,0.,1.)) ;
#38322=DIRECTION('',(1.,-1.75658099177411E-13,-4.54195640846217E-14)) ;
#38323=DIRECTION('center_axis',(-1.75658099177411E-13,-1.,-1.66321791206623E-16)) ;
#38324=DIRECTION('ref_axis',(0.,0.,-1.)) ;
#38325=DIRECTION('center_axis',(3.99680288865051E-14,-7.0997481469889E-27,
1.)) ;
#38326=DIRECTION('ref_axis',(-1.,1.42108547152018E-13,3.99680288865051E-14)) ;
#38327=DIRECTION('center_axis',(-1.75658099177411E-13,-1.,-1.66321791206623E-16)) ;
#38328=DIRECTION('ref_axis',(0.707106781186528,-1.24091425832262E-13,-0.707106781186567)) ;
#38329=DIRECTION('center_axis',(4.54195640846217E-14,-1.66321791214601E-16,
1.)) ;
#38330=DIRECTION('ref_axis',(-0.707106781186698,-0.707106781186397,3.19988744963529E-14)) ;
#38331=DIRECTION('center_axis',(4.54195640846217E-14,-1.66321791214601E-16,
1.)) ;
#38332=DIRECTION('ref_axis',(-0.707106781186698,-0.707106781186397,3.19988744963529E-14)) ;
#38333=DIRECTION('',(4.54195640846217E-14,-1.66321791214601E-16,1.)) ;
#38334=DIRECTION('center_axis',(1.,-1.75658099177411E-13,-4.54195640846217E-14)) ;
#38335=DIRECTION('ref_axis',(4.54195640846217E-14,-1.66321791214601E-16,
1.)) ;
#38336=DIRECTION('',(-1.75658099177411E-13,-1.,-1.66321791206623E-16)) ;
#38337=DIRECTION('',(-4.54195640846217E-14,1.66321791214601E-16,-1.)) ;
#38338=DIRECTION('',(-1.75658099177411E-13,-1.,-1.66321791206623E-16)) ;
#38339=DIRECTION('center_axis',(1.75658099177411E-13,1.,1.66321791206623E-16)) ;
#38340=DIRECTION('ref_axis',(1.,-1.75658099177411E-13,-4.54195640846217E-14)) ;
#38341=DIRECTION('',(-2.79089251708989E-13,1.,1.66321791227277E-16)) ;
#38342=DIRECTION('center_axis',(1.75658099177411E-13,1.,1.66321791206623E-16)) ;
#38343=DIRECTION('ref_axis',(0.258819045102331,-4.53030069799869E-14,-0.965925826289119)) ;
#38344=DIRECTION('center_axis',(4.54195640846217E-14,-1.66321791214601E-16,
1.)) ;
#38345=DIRECTION('ref_axis',(1.75658099177411E-13,1.,1.66321791206623E-16)) ;
#38346=DIRECTION('',(-1.75658099177411E-13,-1.,-1.66321791206623E-16)) ;
#38347=DIRECTION('',(-1.,1.75658099177411E-13,4.54195640846217E-14)) ;
#38348=DIRECTION('center_axis',(-1.75658099177411E-13,-1.,-1.66321791206623E-16)) ;
#38349=DIRECTION('ref_axis',(-1.,1.75658099177411E-13,4.54195640846217E-14)) ;
#38350=DIRECTION('',(1.87026782949573E-13,1.,4.56410568798561E-14)) ;
#38351=DIRECTION('center_axis',(1.75658099177411E-13,1.,1.66321791206623E-16)) ;
#38352=DIRECTION('ref_axis',(-0.258819045102564,4.56243160072301E-14,-0.965925826289057)) ;
#38353=DIRECTION('center_axis',(-1.,1.75658099177411E-13,4.54195640846217E-14)) ;
#38354=DIRECTION('ref_axis',(-4.54195640846217E-14,1.66321791214601E-16,
-1.)) ;
#38355=DIRECTION('',(1.75658099177411E-13,1.,1.66321791206623E-16)) ;
#38356=DIRECTION('',(4.54195640846217E-14,-1.66321791214601E-16,1.)) ;
#38357=DIRECTION('center_axis',(-4.54195640846217E-14,1.66321791214601E-16,
-1.)) ;
#38358=DIRECTION('ref_axis',(-0.707106781186397,0.707106781186698,3.22340890291931E-14)) ;
#38359=DIRECTION('center_axis',(-4.44089209850056E-14,7.88860905220989E-27,
-1.)) ;
#38360=DIRECTION('ref_axis',(-1.,1.42108547152018E-13,4.44089209850056E-14)) ;
#38361=DIRECTION('center_axis',(4.54195640846217E-14,-1.66321791214601E-16,
1.)) ;
#38362=DIRECTION('ref_axis',(-0.707106781186397,0.707106781186698,3.22340890291931E-14)) ;
#38363=DIRECTION('',(-4.54195640846217E-14,1.66321791214601E-16,-1.)) ;
#38364=DIRECTION('center_axis',(1.75658099177411E-13,1.,1.66321791206623E-16)) ;
#38365=DIRECTION('ref_axis',(0.,0.,1.)) ;
#38366=DIRECTION('center_axis',(-1.,1.77635683940022E-13,3.5527157938743E-14)) ;
#38367=DIRECTION('ref_axis',(3.5527157938743E-14,0.,1.)) ;
#38368=DIRECTION('center_axis',(1.75658099177411E-13,1.,1.66321791206623E-16)) ;
#38369=DIRECTION('ref_axis',(0.70710678118651,-1.24091425832259E-13,-0.707106781186585)) ;
#38370=DIRECTION('center_axis',(1.,-1.75658099177411E-13,-4.54195640846217E-14)) ;
#38371=DIRECTION('ref_axis',(1.56325514861457E-13,0.707106781186529,0.707106781186566)) ;
#38372=DIRECTION('center_axis',(-1.,1.77635683940023E-13,5.32906734559391E-14)) ;
#38373=DIRECTION('ref_axis',(5.32906734559391E-14,0.,1.)) ;
#38374=DIRECTION('',(-1.,1.75658099177411E-13,4.54195640846217E-14)) ;
#38375=DIRECTION('center_axis',(1.75658099177411E-13,1.,1.66321791206623E-16)) ;
#38376=DIRECTION('ref_axis',(0.,0.,1.)) ;
#38377=DIRECTION('center_axis',(4.88498130835079E-14,-8.67746995743119E-27,
1.)) ;
#38378=DIRECTION('ref_axis',(1.,-1.42108547152023E-13,-4.88498130835079E-14)) ;
#38379=DIRECTION('center_axis',(1.75658099177411E-13,1.,1.66321791206623E-16)) ;
#38380=DIRECTION('ref_axis',(-0.707106781186573,1.24326640365112E-13,-0.707106781186522)) ;
#38381=DIRECTION('center_axis',(4.54195640846217E-14,-1.66321791214601E-16,
1.)) ;
#38382=DIRECTION('ref_axis',(0.707106781186636,0.70710678118646,-3.199887449635E-14)) ;
#38383=DIRECTION('center_axis',(4.54195640846217E-14,-1.66321791214601E-16,
1.)) ;
#38384=DIRECTION('ref_axis',(0.707106781186636,0.70710678118646,-3.199887449635E-14)) ;
#38385=DIRECTION('',(4.54195640846217E-14,-1.66321791214601E-16,1.)) ;
#38386=DIRECTION('center_axis',(-1.,1.75658099177411E-13,4.54195640846217E-14)) ;
#38387=DIRECTION('ref_axis',(4.54195640846217E-14,-1.66321791214601E-16,
1.)) ;
#38388=DIRECTION('',(1.75658099177411E-13,1.,1.66321791206623E-16)) ;
#38389=DIRECTION('',(-4.54195640846217E-14,1.66321791214601E-16,-1.)) ;
#38390=DIRECTION('',(1.75658099177411E-13,1.,1.66321791206623E-16)) ;
#38391=DIRECTION('center_axis',(-1.75658099177411E-13,-1.,-1.66321791206623E-16)) ;
#38392=DIRECTION('ref_axis',(-1.,1.75658099177411E-13,4.54195640846217E-14)) ;
#38393=DIRECTION('',(-1.75658099177411E-13,-1.,-1.66321791206623E-16)) ;
#38394=DIRECTION('center_axis',(-1.75658099177411E-13,-1.,-1.66321791206623E-16)) ;
#38395=DIRECTION('ref_axis',(-0.258819045102557,4.56243160072289E-14,-0.965925826289059)) ;
#38396=DIRECTION('center_axis',(4.54195640846217E-14,-1.66321791214601E-16,
1.)) ;
#38397=DIRECTION('ref_axis',(1.75658099177411E-13,1.,1.66321791206623E-16)) ;
#38398=DIRECTION('',(1.75658099177411E-13,1.,1.66321791206623E-16)) ;
#38399=DIRECTION('',(1.,-1.75658099177411E-13,-4.54195640846217E-14)) ;
#38400=DIRECTION('center_axis',(1.75658099177411E-13,1.,1.66321791206623E-16)) ;
#38401=DIRECTION('ref_axis',(1.,-1.75658099177411E-13,-4.54195640846217E-14)) ;
#38402=DIRECTION('',(-1.75658099177411E-13,-1.,-1.66321791206623E-16)) ;
#38403=DIRECTION('center_axis',(-1.75658099177411E-13,-1.,-1.66321791206623E-16)) ;
#38404=DIRECTION('ref_axis',(0.258819045102475,-4.53030069800122E-14,-0.965925826289081)) ;
#38405=DIRECTION('center_axis',(1.,-1.75658099177411E-13,-4.54195640846217E-14)) ;
#38406=DIRECTION('ref_axis',(-4.54195640846217E-14,1.66321791214601E-16,
-1.)) ;
#38407=DIRECTION('',(-1.75658099177411E-13,-1.,-1.66321791206623E-16)) ;
#38408=DIRECTION('',(4.54195640846217E-14,-1.66321791214601E-16,1.)) ;
#38409=DIRECTION('center_axis',(-0.5,0.866025403784438,7.35649810170484E-14)) ;
#38410=DIRECTION('ref_axis',(-0.866025403784438,-0.5,-4.2407782439997E-14)) ;
#38411=DIRECTION('',(-0.866025403784438,-0.5,3.92513354304904E-14)) ;
#38412=DIRECTION('',(-5.62735973232286E-17,8.49130336096823E-14,-1.)) ;
#38413=DIRECTION('',(0.866025403784438,0.5,-3.92513354304904E-14)) ;
#38414=DIRECTION('',(-5.62735973232286E-17,8.49130336096823E-14,-1.)) ;
#38415=DIRECTION('center_axis',(0.5,0.866025403784439,7.35087074197251E-14)) ;
#38416=DIRECTION('ref_axis',(-0.866025403784439,0.5,4.25052511696854E-14)) ;
#38417=DIRECTION('',(-0.866025403784438,0.5,3.9417657221705E-14)) ;
#38418=DIRECTION('',(0.866025403784438,-0.5,-3.9417657221705E-14)) ;
#38419=DIRECTION('',(-5.62735973232286E-17,8.49130336096823E-14,-1.)) ;
#38420=DIRECTION('center_axis',(1.,8.10629031994436E-17,-5.62735973232217E-17)) ;
#38421=DIRECTION('ref_axis',(-8.10629031994388E-17,1.,8.49130336096823E-14)) ;
#38422=DIRECTION('',(-8.10629031994436E-17,1.,1.66321791214605E-16)) ;
#38423=DIRECTION('',(8.10629031994341E-17,-1.,-1.66321791214605E-16)) ;
#38424=DIRECTION('',(-5.62735973232286E-17,8.49130336096823E-14,-1.)) ;
#38425=DIRECTION('center_axis',(0.5,-0.866025403784439,-7.35649810170484E-14)) ;
#38426=DIRECTION('ref_axis',(0.866025403784439,0.5,4.24077824399969E-14)) ;
#38427=DIRECTION('',(0.866025403784439,0.5,-3.92513354304904E-14)) ;
#38428=DIRECTION('',(-0.866025403784439,-0.5,3.92513354304904E-14)) ;
#38429=DIRECTION('',(-5.62735973232286E-17,8.49130336096823E-14,-1.)) ;
#38430=DIRECTION('center_axis',(-1.,5.55111512312073E-17,5.62735973232333E-17)) ;
#38431=DIRECTION('ref_axis',(-5.55111512312121E-17,-1.,-8.49130336096823E-14)) ;
#38432=DIRECTION('',(-5.55111512312074E-17,-1.,-1.66321791214598E-16)) ;
#38433=DIRECTION('',(-5.62735973232286E-17,8.49130336096823E-14,-1.)) ;
#38434=DIRECTION('',(5.55111512312168E-17,1.,1.66321791214598E-16)) ;
#38435=DIRECTION('center_axis',(-0.5,-0.866025403784439,-7.35087074197251E-14)) ;
#38436=DIRECTION('ref_axis',(0.866025403784439,-0.5,-4.25052511696854E-14)) ;
#38437=DIRECTION('',(0.866025403784439,-0.5,-3.9417657221705E-14)) ;
#38438=DIRECTION('',(-0.866025403784439,0.5,3.9417657221705E-14)) ;
#38439=DIRECTION('center_axis',(-0.5,0.866025403784438,7.35750690713851E-14)) ;
#38440=DIRECTION('ref_axis',(-0.866025403784438,-0.5,-4.24144871777968E-14)) ;
#38441=DIRECTION('',(-0.866025403784438,-0.5,3.92513354304904E-14)) ;
#38442=DIRECTION('',(-5.55111512312515E-17,8.49251224899127E-14,-1.)) ;
#38443=DIRECTION('',(0.866025403784438,0.5,-3.92513354304904E-14)) ;
#38444=DIRECTION('',(-5.55111512312515E-17,8.49251224899126E-14,-1.)) ;
#38445=DIRECTION('center_axis',(0.5,0.866025403784439,7.35195579201539E-14)) ;
#38446=DIRECTION('ref_axis',(-0.866025403784439,0.5,4.25106353121159E-14)) ;
#38447=DIRECTION('',(-0.866025403784438,0.5,3.9417657221705E-14)) ;
#38448=DIRECTION('',(0.866025403784438,-0.5,-3.9417657221705E-14)) ;
#38449=DIRECTION('',(-5.55111512312515E-17,8.49251224899127E-14,-1.)) ;
#38450=DIRECTION('center_axis',(1.,1.36574054430676E-16,-5.55111512312399E-17)) ;
#38451=DIRECTION('ref_axis',(-1.36574054430671E-16,1.,8.49251224899126E-14)) ;
#38452=DIRECTION('',(-1.36574054430676E-16,1.,1.66321791214607E-16)) ;
#38453=DIRECTION('',(1.36574054430667E-16,-1.,-1.66321791214607E-16)) ;
#38454=DIRECTION('',(-5.55111512312515E-17,8.49251224899127E-14,-1.)) ;
#38455=DIRECTION('center_axis',(0.5,-0.866025403784439,-7.35750690713851E-14)) ;
#38456=DIRECTION('ref_axis',(0.866025403784439,0.5,4.24144871777967E-14)) ;
#38457=DIRECTION('',(0.866025403784439,0.5,-3.92513354304904E-14)) ;
#38458=DIRECTION('',(-0.866025403784439,-0.5,3.92513354304904E-14)) ;
#38459=DIRECTION('',(-5.55111512312515E-17,8.49251224899126E-14,-1.)) ;
#38460=DIRECTION('center_axis',(-1.,-2.52435489670719E-29,5.55111512312515E-17)) ;
#38461=DIRECTION('ref_axis',(2.05292576492018E-29,-1.,-8.49251224899126E-14)) ;
#38462=DIRECTION('',(2.52343162529668E-29,-1.,-1.66321791214601E-16)) ;
#38463=DIRECTION('',(-5.55111512312515E-17,8.49251224899127E-14,-1.)) ;
#38464=DIRECTION('',(-1.58057336172267E-29,1.,1.66321791214601E-16)) ;
#38465=DIRECTION('center_axis',(-0.5,-0.866025403784439,-7.35195579201539E-14)) ;
#38466=DIRECTION('ref_axis',(0.866025403784439,-0.5,-4.25106353121159E-14)) ;
#38467=DIRECTION('',(0.866025403784439,-0.5,-3.9417657221705E-14)) ;
#38468=DIRECTION('',(-0.866025403784439,0.5,3.9417657221705E-14)) ;
#38469=DIRECTION('center_axis',(1.,-1.75658099177411E-13,-4.54195640846217E-14)) ;
#38470=DIRECTION('ref_axis',(-4.54195640846217E-14,1.66321791214601E-16,
-1.)) ;
#38471=DIRECTION('center_axis',(1.,-1.75658099177411E-13,-4.54195640846217E-14)) ;
#38472=DIRECTION('ref_axis',(-4.54195640846217E-14,1.66321791214601E-16,
-1.)) ;
#38473=DIRECTION('center_axis',(-1.,1.75658099177411E-13,4.54195640846217E-14)) ;
#38474=DIRECTION('ref_axis',(9.20925513359107E-14,0.707106781186535,-0.70710678118656)) ;
#38475=DIRECTION('center_axis',(1.,-1.75658099177411E-13,-4.54195640846217E-14)) ;
#38476=DIRECTION('ref_axis',(9.20925513359107E-14,0.707106781186535,-0.70710678118656)) ;
#38477=DIRECTION('center_axis',(-1.,1.75658099177411E-13,4.54195640846217E-14)) ;
#38478=DIRECTION('ref_axis',(9.20925513359107E-14,0.707106781186535,-0.70710678118656)) ;
#38479=DIRECTION('',(1.,-1.75658099177411E-13,-4.54195640846217E-14)) ;
#38480=DIRECTION('center_axis',(1.,-1.75658099177411E-13,-4.54195640846217E-14)) ;
#38481=DIRECTION('ref_axis',(-1.56325514861458E-13,-0.707106781186535,-0.70710678118656)) ;
#38482=DIRECTION('center_axis',(-1.,1.75658099177411E-13,4.54195640846217E-14)) ;
#38483=DIRECTION('ref_axis',(-1.56325514861458E-13,-0.707106781186535,-0.70710678118656)) ;
#38484=DIRECTION('center_axis',(1.,-1.75658099177411E-13,-4.54195640846217E-14)) ;
#38485=DIRECTION('ref_axis',(-1.56325514861458E-13,-0.707106781186535,-0.70710678118656)) ;
#38486=DIRECTION('',(-1.,1.75658099177411E-13,4.54195640846217E-14)) ;
#38487=DIRECTION('center_axis',(1.,-1.75658099177411E-13,-4.54195640846217E-14)) ;
#38488=DIRECTION('ref_axis',(-1.56325514861458E-13,-0.707106781186535,-0.70710678118656)) ;
#38489=DIRECTION('',(-1.,1.75658099177411E-13,4.54195640846217E-14)) ;
#38490=DIRECTION('center_axis',(-1.,1.75658099177411E-13,4.54195640846217E-14)) ;
#38491=DIRECTION('ref_axis',(-1.56325514861458E-13,-0.707106781186535,-0.70710678118656)) ;
#38492=DIRECTION('center_axis',(-1.,1.75658099177411E-13,4.54195640846217E-14)) ;
#38493=DIRECTION('ref_axis',(9.20925513359107E-14,0.707106781186535,-0.70710678118656)) ;
#38494=DIRECTION('center_axis',(1.,-1.75658099177411E-13,-4.54195640846217E-14)) ;
#38495=DIRECTION('ref_axis',(9.20925513359107E-14,0.707106781186535,-0.70710678118656)) ;
#38496=DIRECTION('center_axis',(-1.,1.75658099177411E-13,4.54195640846217E-14)) ;
#38497=DIRECTION('ref_axis',(9.20925513359107E-14,0.707106781186535,-0.70710678118656)) ;
#38498=DIRECTION('',(1.,-1.75658099177411E-13,-4.54195640846217E-14)) ;
#38499=DIRECTION('center_axis',(1.,-1.75658099177411E-13,-4.54195640846217E-14)) ;
#38500=DIRECTION('ref_axis',(9.20925513359107E-14,0.707106781186535,-0.70710678118656)) ;
#38501=DIRECTION('center_axis',(-1.,1.75658099177411E-13,4.54195640846217E-14)) ;
#38502=DIRECTION('ref_axis',(9.20925513359107E-14,0.707106781186535,-0.70710678118656)) ;
#38503=DIRECTION('',(1.,-1.75658099177411E-13,-4.54195640846217E-14)) ;
#38504=DIRECTION('center_axis',(1.,-1.75658099177411E-13,-4.54195640846217E-14)) ;
#38505=DIRECTION('ref_axis',(9.20925513359107E-14,0.707106781186535,-0.70710678118656)) ;
#38506=DIRECTION('center_axis',(-1.,1.75658099177411E-13,4.54195640846217E-14)) ;
#38507=DIRECTION('ref_axis',(4.54195640846217E-14,-1.66321791214601E-16,
1.)) ;
#38508=DIRECTION('',(1.75658099177411E-13,1.,1.66321791206623E-16)) ;
#38509=DIRECTION('',(4.54195640846217E-14,-1.66321791214601E-16,1.)) ;
#38510=DIRECTION('',(-1.75658099177411E-13,-1.,-1.66321791206623E-16)) ;
#38511=DIRECTION('',(1.75658099177411E-13,1.,1.66321791206623E-16)) ;
#38512=DIRECTION('center_axis',(-1.61486985400024E-13,-1.,0.)) ;
#38513=DIRECTION('ref_axis',(0.99999997726804,-1.61486981729108E-13,-0.000213222701069828)) ;
#38514=DIRECTION('center_axis',(1.75658099177411E-13,1.,1.66321791206623E-16)) ;
#38515=DIRECTION('ref_axis',(0.99999997726804,-1.75658059720776E-13,-0.000213222701069828)) ;
#38516=DIRECTION('',(-0.707106765112755,-0.707106781186416,0.000150771217829304)) ;
#38517=DIRECTION('center_axis',(-1.75658099177411E-13,-1.,-1.66321791206623E-16)) ;
#38518=DIRECTION('ref_axis',(0.99999997726804,-1.75658059720776E-13,-0.000213222701069828)) ;
#38519=DIRECTION('',(-1.75658099177411E-13,-1.,-1.66321791206623E-16)) ;
#38520=DIRECTION('center_axis',(1.61486985400024E-13,1.,0.)) ;
#38521=DIRECTION('ref_axis',(0.00363593456997526,-5.87156112817037E-16,
0.999993389968055)) ;
#38522=DIRECTION('center_axis',(-1.75658099177411E-13,-1.,-1.66321791206623E-16)) ;
#38523=DIRECTION('ref_axis',(0.00363593456997526,-8.05002047109562E-16,
0.999993389968055)) ;
#38524=DIRECTION('',(-0.002570993990266,0.707106781186547,-0.707102107188137)) ;
#38525=DIRECTION('center_axis',(-1.75658099177411E-13,-1.,-1.66321791206623E-16)) ;
#38526=DIRECTION('ref_axis',(0.00363593456997526,-8.05002047109562E-16,
0.999993389968055)) ;
#38527=DIRECTION('',(-1.75658099177411E-13,-1.,-1.66321791206623E-16)) ;
#38528=DIRECTION('center_axis',(-1.75617096622526E-13,-1.,0.)) ;
#38529=DIRECTION('ref_axis',(1.,-1.75617096622526E-13,-4.54195640846217E-14)) ;
#38530=DIRECTION('center_axis',(1.75658099177411E-13,1.,1.66321791206623E-16)) ;
#38531=DIRECTION('ref_axis',(1.,-1.75658099177411E-13,-4.54195640846217E-14)) ;
#38532=DIRECTION('',(-0.707106781186674,-0.707106781186421,3.20298861571495E-14)) ;
#38533=DIRECTION('center_axis',(-1.75658099177411E-13,-1.,-1.66321791206623E-16)) ;
#38534=DIRECTION('ref_axis',(1.,-1.75658099177411E-13,-4.54195640846217E-14)) ;
#38535=DIRECTION('',(-1.75658099177411E-13,-1.,-1.66321791206623E-16)) ;
#38536=DIRECTION('center_axis',(-4.54195640846217E-14,1.66321791214601E-16,
-1.)) ;
#38537=DIRECTION('ref_axis',(-1.,5.55236256206829E-46,4.54195640846217E-14)) ;
#38538=DIRECTION('',(1.,-1.75658099177411E-13,-4.54195640846217E-14)) ;
#38539=DIRECTION('center_axis',(-4.54195640846217E-14,1.66321791214601E-16,
-1.)) ;
#38540=DIRECTION('ref_axis',(0.923076923076982,0.384615384615244,-4.18617815430325E-14)) ;
#38541=DIRECTION('center_axis',(-4.54195640846217E-14,1.66321791214601E-16,
-1.)) ;
#38542=DIRECTION('ref_axis',(-1.,5.55236256206829E-46,4.54195640846217E-14)) ;
#38543=DIRECTION('',(1.,-1.75658099177411E-13,-4.54195640846217E-14)) ;
#38544=DIRECTION('center_axis',(4.54195640846217E-14,-1.66321791214601E-16,
1.)) ;
#38545=DIRECTION('ref_axis',(-0.923076923076847,0.384615384615568,4.19897213824222E-14)) ;
#38546=DIRECTION('center_axis',(1.75658099177411E-13,1.,1.66321791206623E-16)) ;
#38547=DIRECTION('ref_axis',(-1.,1.75658099177411E-13,4.54195640846217E-14)) ;
#38548=DIRECTION('center_axis',(-1.75658099177411E-13,-1.,-1.66321791206623E-16)) ;
#38549=DIRECTION('ref_axis',(-1.,1.75658099177411E-13,4.54195640846217E-14)) ;
#38550=DIRECTION('',(1.75658099177411E-13,1.,1.66321791206623E-16)) ;
#38551=DIRECTION('center_axis',(1.75658099177411E-13,1.,1.66321791206623E-16)) ;
#38552=DIRECTION('ref_axis',(-1.,1.75658099173691E-13,2.23674678734541E-8)) ;
#38553=DIRECTION('center_axis',(1.75658099177411E-13,1.,1.66321791206623E-16)) ;
#38554=DIRECTION('ref_axis',(-1.,1.75658099173691E-13,2.23674678734541E-8)) ;
#38555=DIRECTION('center_axis',(1.75658099177411E-13,1.,1.66321791206623E-16)) ;
#38556=DIRECTION('ref_axis',(-4.54195640846217E-14,1.66321791214601E-16,
-1.)) ;
#38557=DIRECTION('',(1.56412110467083E-13,0.707106781186548,0.707106781186547)) ;
#38558=DIRECTION('center_axis',(1.75658099177411E-13,1.,1.66321791206623E-16)) ;
#38559=DIRECTION('ref_axis',(1.,-1.75658099177411E-13,-4.54195640846217E-14)) ;
#38560=DIRECTION('center_axis',(4.54195640846217E-14,-1.66321791214601E-16,
1.)) ;
#38561=DIRECTION('ref_axis',(-1.,1.75658099177411E-13,4.54195640846217E-14)) ;
#38562=DIRECTION('center_axis',(-4.54195640846217E-14,1.66321791214601E-16,
-1.)) ;
#38563=DIRECTION('ref_axis',(1.,-1.75658099177411E-13,-4.54195640846217E-14)) ;
#38564=DIRECTION('',(-4.54195640846217E-14,1.66321791214601E-16,-1.)) ;
#38565=DIRECTION('center_axis',(4.54195640846217E-14,-1.66321791214601E-16,
1.)) ;
#38566=DIRECTION('ref_axis',(-1.,1.75658099177411E-13,4.54195640846217E-14)) ;
#38567=DIRECTION('',(4.54195640846217E-14,-1.66321791214601E-16,1.)) ;
#38568=DIRECTION('center_axis',(4.54195640846217E-14,-1.66321791214601E-16,
1.)) ;
#38569=DIRECTION('ref_axis',(-1.,1.75658099177411E-13,4.54195640846217E-14)) ;
#38570=DIRECTION('center_axis',(-4.54195640846217E-14,1.66321791214601E-16,
-1.)) ;
#38571=DIRECTION('ref_axis',(1.,-1.75658099177411E-13,-4.54195640846217E-14)) ;
#38572=DIRECTION('',(-4.54195640846217E-14,1.66321791214601E-16,-1.)) ;
#38573=DIRECTION('center_axis',(4.54195640846217E-14,-1.66321791214601E-16,
1.)) ;
#38574=DIRECTION('ref_axis',(-1.,1.75658099177411E-13,4.54195640846217E-14)) ;
#38575=DIRECTION('',(4.54195640846217E-14,-1.66321791214601E-16,1.)) ;
#38576=DIRECTION('center_axis',(-4.54195640846217E-14,1.66321791214601E-16,
-1.)) ;
#38577=DIRECTION('ref_axis',(-1.,1.75658099177411E-13,4.54195640846217E-14)) ;
#38578=DIRECTION('center_axis',(4.54195640846217E-14,-1.66321791214601E-16,
1.)) ;
#38579=DIRECTION('ref_axis',(1.,-1.75658099177411E-13,-4.54195640846217E-14)) ;
#38580=DIRECTION('',(4.54195640846217E-14,-1.66321791214601E-16,1.)) ;
#38581=DIRECTION('center_axis',(-4.54195640846217E-14,1.66321791214601E-16,
-1.)) ;
#38582=DIRECTION('ref_axis',(-1.,1.75658099177411E-13,4.54195640846217E-14)) ;
#38583=DIRECTION('',(-4.54195640846217E-14,1.66321791214601E-16,-1.)) ;
#38584=DIRECTION('center_axis',(-4.54195640846217E-14,1.66321791214601E-16,
-1.)) ;
#38585=DIRECTION('ref_axis',(-1.,1.75658099177411E-13,4.54195640846217E-14)) ;
#38586=DIRECTION('center_axis',(4.54195640846217E-14,-1.66321791214601E-16,
1.)) ;
#38587=DIRECTION('ref_axis',(1.,-1.75658099177411E-13,-4.54195640846217E-14)) ;
#38588=DIRECTION('',(4.54195640846217E-14,-1.66321791214601E-16,1.)) ;
#38589=DIRECTION('center_axis',(-4.54195640846217E-14,1.66321791214601E-16,
-1.)) ;
#38590=DIRECTION('ref_axis',(-1.,1.75658099177411E-13,4.54195640846217E-14)) ;
#38591=DIRECTION('',(-4.54195640846217E-14,1.66321791214601E-16,-1.)) ;
#38592=DIRECTION('center_axis',(4.54195640846217E-14,-1.66321791214601E-16,
1.)) ;
#38593=DIRECTION('ref_axis',(-1.75658099177411E-13,-1.,-1.66321791206623E-16)) ;
#38594=DIRECTION('center_axis',(-4.54195640846217E-14,1.66321791214601E-16,
-1.)) ;
#38595=DIRECTION('ref_axis',(1.,-1.75658099177411E-13,-4.54195640846217E-14)) ;
#38596=DIRECTION('center_axis',(-4.54195640846217E-14,1.66321791214601E-16,
-1.)) ;
#38597=DIRECTION('ref_axis',(1.,-1.75658099177411E-13,-4.54195640846217E-14)) ;
#38598=DIRECTION('',(-4.54195640846217E-14,1.66321791214601E-16,-1.)) ;
#38599=DIRECTION('center_axis',(4.54195640846217E-14,-1.66321791214601E-16,
1.)) ;
#38600=DIRECTION('ref_axis',(-1.75658099177411E-13,-1.,-1.66321791206623E-16)) ;
#38601=DIRECTION('center_axis',(-4.54195640846217E-14,1.66321791214601E-16,
-1.)) ;
#38602=DIRECTION('ref_axis',(1.,-1.75658099177411E-13,-4.54195640846217E-14)) ;
#38603=DIRECTION('',(4.54195640846217E-14,-1.66321791214601E-16,1.)) ;
#38604=DIRECTION('center_axis',(-4.54195640846217E-14,1.66321791214601E-16,
-1.)) ;
#38605=DIRECTION('ref_axis',(1.,-1.75658099177411E-13,-4.54195640846217E-14)) ;
#38606=DIRECTION('',(-4.54195640846217E-14,1.66321791214601E-16,-1.)) ;
#38607=DIRECTION('center_axis',(1.75658099177411E-13,1.,1.66321791206623E-16)) ;
#38608=DIRECTION('ref_axis',(-0.268757454585954,4.0124766254688E-14,-0.963207885455927)) ;
#38609=DIRECTION('center_axis',(-4.54195640846217E-14,1.66321791214601E-16,
-1.)) ;
#38610=DIRECTION('ref_axis',(-1.,1.75658099177411E-13,4.54195640846217E-14)) ;
#38611=DIRECTION('center_axis',(1.,-1.75658099177411E-13,-4.54195640846217E-14)) ;
#38612=DIRECTION('ref_axis',(1.75658099177411E-13,1.,1.66321791206622E-16)) ;
#38613=DIRECTION('center_axis',(1.75658099177411E-13,1.,1.66321791206623E-16)) ;
#38614=DIRECTION('ref_axis',(1.,-1.75658099177198E-13,-1.28004463729308E-9)) ;
#38615=DIRECTION('center_axis',(4.54195640846217E-14,-1.66321791214601E-16,
1.)) ;
#38616=DIRECTION('ref_axis',(1.75658099177411E-13,1.,1.66321791206623E-16)) ;
#38617=DIRECTION('center_axis',(4.54195640846217E-14,-1.66321791214601E-16,
1.)) ;
#38618=DIRECTION('ref_axis',(1.75658099177411E-13,1.,1.66321791206623E-16)) ;
#38619=DIRECTION('',(4.54195640846217E-14,-1.66321791214601E-16,1.)) ;
#38620=DIRECTION('center_axis',(-1.75658099177411E-13,-1.,-1.66321791206623E-16)) ;
#38621=DIRECTION('ref_axis',(1.,-1.75658099177411E-13,-4.54195640846217E-14)) ;
#38622=DIRECTION('',(1.75658099177411E-13,1.,1.66321791206623E-16)) ;
#38623=DIRECTION('',(-1.75658099177411E-13,-1.,-1.66321791206623E-16)) ;
#38624=DIRECTION('center_axis',(1.75658099177411E-13,1.,1.66321791206623E-16)) ;
#38625=DIRECTION('ref_axis',(-1.,1.75658099177411E-13,4.54195640846217E-14)) ;
#38626=DIRECTION('',(-1.75658099177411E-13,-1.,-1.66321791206623E-16)) ;
#38627=DIRECTION('',(1.75658099177411E-13,1.,1.66321791206623E-16)) ;
#38628=DIRECTION('center_axis',(1.75658099177411E-13,1.,1.66321791206623E-16)) ;
#38629=DIRECTION('ref_axis',(-1.,1.75658099177411E-13,4.54195640846217E-14)) ;
#38630=DIRECTION('',(-1.75658099177411E-13,-1.,-1.66321791206623E-16)) ;
#38631=DIRECTION('',(1.75658099177411E-13,1.,1.66321791206623E-16)) ;
#38632=DIRECTION('center_axis',(-4.54195640846217E-14,1.66321791214601E-16,
-1.)) ;
#38633=DIRECTION('ref_axis',(-1.75658099177411E-13,-1.,-1.66321791206623E-16)) ;
#38634=DIRECTION('center_axis',(-1.75658099177411E-13,-1.,-1.66321791206623E-16)) ;
#38635=DIRECTION('ref_axis',(1.,-1.75658099177411E-13,-4.54195640846217E-14)) ;
#38636=DIRECTION('',(-1.75658099177411E-13,-1.,-1.66321791206623E-16)) ;
#38637=DIRECTION('center_axis',(1.,-1.75658099177411E-13,-4.54195640846217E-14)) ;
#38638=DIRECTION('ref_axis',(-4.54195640846217E-14,1.66321791214601E-16,
-1.)) ;
#38639=DIRECTION('',(-1.75658099177411E-13,-1.,-1.66321791206623E-16)) ;
#38640=DIRECTION('',(1.75658099177411E-13,1.,1.66321791206623E-16)) ;
#38641=DIRECTION('center_axis',(-4.54195640846217E-14,1.66321791214601E-16,
-1.)) ;
#38642=DIRECTION('ref_axis',(-1.,1.75658099177411E-13,4.54195640846217E-14)) ;
#38643=DIRECTION('',(1.75658099177411E-13,1.,1.66321791206623E-16)) ;
#38644=DIRECTION('center_axis',(-1.,1.75658099177411E-13,4.54195640846217E-14)) ;
#38645=DIRECTION('ref_axis',(4.54195640846217E-14,-1.66321791214601E-16,
1.)) ;
#38646=DIRECTION('',(1.75658099177411E-13,1.,1.66321791206623E-16)) ;
#38647=DIRECTION('center_axis',(4.54195640846217E-14,-1.66321791214601E-16,
1.)) ;
#38648=DIRECTION('ref_axis',(1.,-1.75658099177411E-13,-4.54195640846217E-14)) ;
#38649=DIRECTION('center_axis',(1.,-1.75658099177411E-13,-4.54195640846217E-14)) ;
#38650=DIRECTION('ref_axis',(-4.54195640846217E-14,1.66321791214601E-16,
-1.)) ;
#38651=DIRECTION('',(-1.75658099177411E-13,-1.,-1.66321791206623E-16)) ;
#38652=DIRECTION('',(1.75658099177411E-13,1.,1.66321791206623E-16)) ;
#38653=DIRECTION('center_axis',(-4.54195640846217E-14,1.66321791214601E-16,
-1.)) ;
#38654=DIRECTION('ref_axis',(-1.,1.75658099177411E-13,4.54195640846217E-14)) ;
#38655=DIRECTION('',(1.75658099177411E-13,1.,1.66321791206623E-16)) ;
#38656=DIRECTION('center_axis',(-1.,1.75658099177411E-13,4.54195640846217E-14)) ;
#38657=DIRECTION('ref_axis',(4.54195640846217E-14,-1.66321791214601E-16,
1.)) ;
#38658=DIRECTION('',(1.75658099177411E-13,1.,1.66321791206623E-16)) ;
#38659=DIRECTION('center_axis',(4.54195640846217E-14,-1.66321791214601E-16,
1.)) ;
#38660=DIRECTION('ref_axis',(1.,-1.75658099177411E-13,-4.54195640846217E-14)) ;
#38661=DIRECTION('center_axis',(1.,-1.75658099177411E-13,-4.54195640846217E-14)) ;
#38662=DIRECTION('ref_axis',(-4.54195640846217E-14,1.66321791214601E-16,
-1.)) ;
#38663=DIRECTION('',(-1.75658099177411E-13,-1.,-1.66321791206623E-16)) ;
#38664=DIRECTION('',(1.75658099177411E-13,1.,1.66321791206623E-16)) ;
#38665=DIRECTION('center_axis',(-4.54195640846217E-14,1.66321791214601E-16,
-1.)) ;
#38666=DIRECTION('ref_axis',(-1.,1.75658099177411E-13,4.54195640846217E-14)) ;
#38667=DIRECTION('',(1.75658099177411E-13,1.,1.66321791206623E-16)) ;
#38668=DIRECTION('center_axis',(-1.,1.75658099177411E-13,4.54195640846217E-14)) ;
#38669=DIRECTION('ref_axis',(4.54195640846217E-14,-1.66321791214601E-16,
1.)) ;
#38670=DIRECTION('',(1.75658099177411E-13,1.,1.66321791206623E-16)) ;
#38671=DIRECTION('center_axis',(4.54195640846217E-14,-1.66321791214601E-16,
1.)) ;
#38672=DIRECTION('ref_axis',(1.,-1.75658099177411E-13,-4.54195640846217E-14)) ;
#38673=DIRECTION('center_axis',(4.54195640846217E-14,-1.66321791214601E-16,
1.)) ;
#38674=DIRECTION('ref_axis',(1.,-1.75658099177411E-13,-4.54195640846217E-14)) ;
#38675=DIRECTION('center_axis',(4.54195640846217E-14,-1.66321791214601E-16,
1.)) ;
#38676=DIRECTION('ref_axis',(0.923076923076982,0.384615384615244,-4.18617815430325E-14)) ;
#38677=DIRECTION('center_axis',(-1.,1.75658099177411E-13,4.54195640846217E-14)) ;
#38678=DIRECTION('ref_axis',(4.54195640846217E-14,-1.66321791214601E-16,
1.)) ;
#38679=DIRECTION('',(1.75658099177411E-13,1.,1.66321791206623E-16)) ;
#38680=DIRECTION('',(1.75658099177411E-13,1.,1.66321791206623E-16)) ;
#38681=DIRECTION('center_axis',(4.54195640846217E-14,-1.66321791214601E-16,
1.)) ;
#38682=DIRECTION('ref_axis',(1.,-1.75658099177411E-13,-4.54195640846217E-14)) ;
#38683=DIRECTION('',(-1.75658099177411E-13,-1.,-1.66321791206623E-16)) ;
#38684=DIRECTION('center_axis',(1.,-1.75658099177411E-13,-4.54195640846217E-14)) ;
#38685=DIRECTION('ref_axis',(-4.54195640846217E-14,1.66321791214601E-16,
-1.)) ;
#38686=DIRECTION('',(1.75658099177411E-13,1.,1.66321791206623E-16)) ;
#38687=DIRECTION('center_axis',(-4.54195640846217E-14,1.66321791214601E-16,
-1.)) ;
#38688=DIRECTION('ref_axis',(-1.,1.75658099177411E-13,4.54195640846217E-14)) ;
#38689=DIRECTION('center_axis',(-1.,1.75658099177411E-13,4.54195640846217E-14)) ;
#38690=DIRECTION('ref_axis',(4.54195640846217E-14,-1.66321791214601E-16,
1.)) ;
#38691=DIRECTION('',(1.75658099177411E-13,1.,1.66321791206623E-16)) ;
#38692=DIRECTION('',(-1.75658099177411E-13,-1.,-1.66321791206623E-16)) ;
#38693=DIRECTION('center_axis',(1.,-1.75658099177411E-13,-4.54195640846217E-14)) ;
#38694=DIRECTION('ref_axis',(-4.54195640846217E-14,1.66321791214601E-16,
-1.)) ;
#38695=DIRECTION('center_axis',(1.,-1.75658099177411E-13,-4.54195640846217E-14)) ;
#38696=DIRECTION('ref_axis',(1.75658099177411E-13,1.,1.66321791206623E-16)) ;
#38697=DIRECTION('',(-1.75658099177411E-13,-1.,-1.66321791206623E-16)) ;
#38698=DIRECTION('',(-1.75658099177411E-13,-1.,-1.66321791206622E-16)) ;
#38699=DIRECTION('center_axis',(1.,-1.75658099177411E-13,-4.54195640846217E-14)) ;
#38700=DIRECTION('ref_axis',(-4.54195640846217E-14,1.66321791214601E-16,
-1.)) ;
#38701=DIRECTION('center_axis',(-1.,1.75658099177411E-13,4.54195640846217E-14)) ;
#38702=DIRECTION('ref_axis',(1.75658099177411E-13,1.,1.66321791206623E-16)) ;
#38703=DIRECTION('center_axis',(-1.,1.75658099177411E-13,4.54195640846217E-14)) ;
#38704=DIRECTION('ref_axis',(1.75658099177411E-13,1.,1.66321791206623E-16)) ;
#38705=DIRECTION('',(-1.,1.75658099177411E-13,4.54195640846217E-14)) ;
#38706=DIRECTION('center_axis',(1.,-1.75658099177411E-13,-4.54195640846217E-14)) ;
#38707=DIRECTION('ref_axis',(-4.54195640846217E-14,1.66321791214601E-16,
-1.)) ;
#38708=DIRECTION('',(1.,-1.75658099177411E-13,-4.54195640846217E-14)) ;
#38709=DIRECTION('center_axis',(-1.,1.75658099177411E-13,4.54195640846217E-14)) ;
#38710=DIRECTION('ref_axis',(1.75658099177411E-13,1.,1.66321791206623E-16)) ;
#38711=DIRECTION('center_axis',(1.,-1.75658099177411E-13,-4.54195640846217E-14)) ;
#38712=DIRECTION('ref_axis',(1.75658099177411E-13,1.,1.66321791206623E-16)) ;
#38713=DIRECTION('',(1.75658099177411E-13,1.,1.66321791206623E-16)) ;
#38714=DIRECTION('',(-1.75658099177411E-13,-1.,-1.66321791206622E-16)) ;
#38715=DIRECTION('center_axis',(1.,-1.75658099177411E-13,-4.54195640846217E-14)) ;
#38716=DIRECTION('ref_axis',(-4.54195640846217E-14,1.66321791214601E-16,
-1.)) ;
#38717=DIRECTION('center_axis',(1.,-1.75658099177411E-13,-4.54195640846217E-14)) ;
#38718=DIRECTION('ref_axis',(-4.54195640846217E-14,1.66321791214601E-16,
-1.)) ;
#38719=DIRECTION('',(1.,-1.75658099177411E-13,-4.54195640846217E-14)) ;
#38720=DIRECTION('center_axis',(-1.,1.75658099177411E-13,4.54195640846217E-14)) ;
#38721=DIRECTION('ref_axis',(1.75658099177411E-13,1.,1.66321791206623E-16)) ;
#38722=DIRECTION('center_axis',(1.,-1.75658099177411E-13,-4.54195640846217E-14)) ;
#38723=DIRECTION('ref_axis',(1.75658099177411E-13,1.,1.66321791206622E-16)) ;
#38724=DIRECTION('center_axis',(-1.,1.75658099177411E-13,4.54195640846217E-14)) ;
#38725=DIRECTION('ref_axis',(4.54195640846217E-14,-1.66321791214601E-16,
1.)) ;
#38726=DIRECTION('',(1.,-1.75658099177411E-13,-4.54195640846217E-14)) ;
#38727=DIRECTION('center_axis',(1.75658099177411E-13,1.,1.66321791206623E-16)) ;
#38728=DIRECTION('ref_axis',(-0.963207885455927,1.73873987103648E-13,0.268757454585955)) ;
#38729=DIRECTION('center_axis',(-4.54195640846217E-14,1.66321791214601E-16,
-1.)) ;
#38730=DIRECTION('ref_axis',(1.75658099177411E-13,1.,1.66321791206623E-16)) ;
#38731=DIRECTION('center_axis',(1.75658099177411E-13,1.,1.66321791206623E-16)) ;
#38732=DIRECTION('ref_axis',(-1.28008105260808E-9,1.66322016063228E-16,
-1.)) ;
#38733=DIRECTION('center_axis',(-4.54195640846217E-14,1.66321791214601E-16,
-1.)) ;
#38734=DIRECTION('ref_axis',(1.75658099177411E-13,1.,1.66321791206623E-16)) ;
#38735=DIRECTION('',(-4.54195640846217E-14,1.66321791214601E-16,-1.)) ;
#38736=DIRECTION('center_axis',(1.,-1.75658099177411E-13,-4.54195640846217E-14)) ;
#38737=DIRECTION('ref_axis',(1.75658099177411E-13,1.,1.66321791206623E-16)) ;
#38738=DIRECTION('',(1.75658099177411E-13,1.,1.66321791206623E-16)) ;
#38739=DIRECTION('',(1.75658099177411E-13,1.,1.66321791206622E-16)) ;
#38740=DIRECTION('center_axis',(1.,-1.75658099177411E-13,-4.54195640846217E-14)) ;
#38741=DIRECTION('ref_axis',(1.75658099177411E-13,1.,1.66321791206623E-16)) ;
#38742=DIRECTION('',(1.75658099177411E-13,1.,1.66321791206623E-16)) ;
#38743=DIRECTION('',(1.75658099177411E-13,1.,1.66321791206622E-16)) ;
#38744=DIRECTION('center_axis',(1.,-1.75658099177411E-13,-4.54195640846217E-14)) ;
#38745=DIRECTION('ref_axis',(-4.54195640846217E-14,1.66321791214601E-16,
-1.)) ;
#38746=DIRECTION('',(1.75658099177411E-13,1.,1.66321791206623E-16)) ;
#38747=DIRECTION('',(-1.75658099177411E-13,-1.,-1.66321791206623E-16)) ;
#38748=DIRECTION('center_axis',(1.,-1.75658099177411E-13,-4.54195640846217E-14)) ;
#38749=DIRECTION('ref_axis',(-4.54195640846217E-14,1.66321791214601E-16,
-1.)) ;
#38750=DIRECTION('',(1.75658099177411E-13,1.,1.66321791206623E-16)) ;
#38751=DIRECTION('',(-1.75658099177411E-13,-1.,-1.66321791206623E-16)) ;
#38752=DIRECTION('center_axis',(1.75658099177411E-13,1.,1.66321791206623E-16)) ;
#38753=DIRECTION('ref_axis',(-1.,1.75658099177411E-13,4.54195640846217E-14)) ;
#38754=DIRECTION('',(-4.54195640846217E-14,1.663217912146E-16,-1.)) ;
#38755=DIRECTION('',(1.,-1.75658099177411E-13,-4.54195640846217E-14)) ;
#38756=DIRECTION('',(-4.54195640846217E-14,1.66321791214601E-16,-1.)) ;
#38757=DIRECTION('',(-1.,1.75658099177411E-13,4.54195640846217E-14)) ;
#38758=DIRECTION('',(4.54195640846217E-14,-1.66321791214601E-16,1.)) ;
#38759=DIRECTION('',(1.,-1.75658099177411E-13,-4.54195640846217E-14)) ;
#38760=DIRECTION('',(4.54195640846217E-14,-1.66321791214601E-16,1.)) ;
#38761=DIRECTION('center_axis',(-1.75658099177411E-13,-1.,-1.66321791206623E-16)) ;
#38762=DIRECTION('ref_axis',(-1.,1.75658099177624E-13,-1.27995379816492E-9)) ;
#38763=DIRECTION('',(-1.,1.75658099177411E-13,4.54195640846217E-14)) ;
#38764=DIRECTION('center_axis',(-1.75658099177411E-13,-1.,-1.66321791206623E-16)) ;
#38765=DIRECTION('ref_axis',(1.28005416232692E-9,1.66321566354742E-16,-1.)) ;
#38766=DIRECTION('',(-4.54195640846195E-14,1.25021331759346E-14,-1.)) ;
#38767=DIRECTION('',(4.54195640846217E-14,-1.66321791214601E-16,1.)) ;
#38768=DIRECTION('center_axis',(-1.75658099177411E-13,-1.,-1.66321791206623E-16)) ;
#38769=DIRECTION('ref_axis',(1.,-1.75658099177411E-13,-4.54195640846217E-14)) ;
#38770=DIRECTION('center_axis',(-1.75658099177411E-13,-1.,-1.66321791206623E-16)) ;
#38771=DIRECTION('ref_axis',(1.,-1.75658099177411E-13,-4.54195640846217E-14)) ;
#38772=DIRECTION('center_axis',(-1.75658099177411E-13,-1.,-1.66321791206623E-16)) ;
#38773=DIRECTION('ref_axis',(1.,-1.75658099177411E-13,-4.54195640846217E-14)) ;
#38774=DIRECTION('center_axis',(-1.75658099177411E-13,-1.,-1.66321791206623E-16)) ;
#38775=DIRECTION('ref_axis',(1.,-1.75658099177411E-13,-4.54195640846217E-14)) ;
#38776=DIRECTION('center_axis',(4.54195640846217E-14,-1.66321791214601E-16,
1.)) ;
#38777=DIRECTION('ref_axis',(-1.,1.75658099177411E-13,4.54195640846217E-14)) ;
#38778=DIRECTION('center_axis',(-4.54195640846217E-14,1.66321791214601E-16,
-1.)) ;
#38779=DIRECTION('ref_axis',(0.707106781186648,0.707106781186447,-3.19988744963506E-14)) ;
#38780=DIRECTION('',(1.,-1.75658099177411E-13,-4.54195640846217E-14)) ;
#38781=DIRECTION('center_axis',(-4.54195640846217E-14,1.66321791214601E-16,
-1.)) ;
#38782=DIRECTION('ref_axis',(-0.707106781186397,0.707106781186698,3.22340890291931E-14)) ;
#38783=DIRECTION('center_axis',(-1.75658099177411E-13,-1.,-1.66321791206623E-16)) ;
#38784=DIRECTION('ref_axis',(1.,-1.75658099177411E-13,-4.54195640846217E-14)) ;
#38785=DIRECTION('center_axis',(1.75658099177411E-13,1.,1.66321791206623E-16)) ;
#38786=DIRECTION('ref_axis',(1.,-1.75658099177411E-13,-4.54195640846217E-14)) ;
#38787=DIRECTION('',(-1.75658099177411E-13,-1.,-1.66321791206623E-16)) ;
#38788=DIRECTION('center_axis',(1.75658099177411E-13,1.,1.66321791206623E-16)) ;
#38789=DIRECTION('ref_axis',(-1.,1.75658099177411E-13,4.54195640846217E-14)) ;
#38790=DIRECTION('center_axis',(1.75658099177411E-13,1.,1.66321791206623E-16)) ;
#38791=DIRECTION('ref_axis',(-1.,1.75658099177411E-13,4.54195640846217E-14)) ;
#38792=DIRECTION('center_axis',(-1.75658099177411E-13,-1.,-1.66321791206623E-16)) ;
#38793=DIRECTION('ref_axis',(-4.54195640846217E-14,1.66321791214601E-16,
-1.)) ;
#38794=DIRECTION('',(-9.21791469415371E-14,-0.707106781186548,0.707106781186547)) ;
#38795=DIRECTION('center_axis',(-1.75658099177411E-13,-1.,-1.66321791206623E-16)) ;
#38796=DIRECTION('ref_axis',(1.,-1.75658099177411E-13,-4.54195640846217E-14)) ;
#38797=DIRECTION('center_axis',(1.75658099177411E-13,1.,1.66321791206623E-16)) ;
#38798=DIRECTION('ref_axis',(1.,-1.75658099177411E-13,-4.54195640846217E-14)) ;
#38799=DIRECTION('',(-1.75658099177411E-13,-1.,-1.66321791206623E-16)) ;
#38800=DIRECTION('center_axis',(1.75658099177411E-13,1.,1.66321791206623E-16)) ;
#38801=DIRECTION('ref_axis',(-1.,1.75658099177411E-13,4.54195640846217E-14)) ;
#38802=DIRECTION('center_axis',(1.75658099177411E-13,1.,1.66321791206623E-16)) ;
#38803=DIRECTION('ref_axis',(-1.,1.75658099177411E-13,4.54195640846217E-14)) ;
#38804=DIRECTION('center_axis',(-1.75658099177411E-13,-1.,-1.66321791206623E-16)) ;
#38805=DIRECTION('ref_axis',(-4.54195640846217E-14,1.66321791214601E-16,
-1.)) ;
#38806=DIRECTION('',(-9.21791469415371E-14,-0.707106781186548,0.707106781186547)) ;
#38807=DIRECTION('center_axis',(-1.75658099177411E-13,-1.,-1.66321791206623E-16)) ;
#38808=DIRECTION('ref_axis',(1.,-1.75658099177411E-13,-4.54195640846217E-14)) ;
#38809=DIRECTION('center_axis',(1.75658099177411E-13,1.,1.66321791206623E-16)) ;
#38810=DIRECTION('ref_axis',(1.,-1.75658099177411E-13,-4.54195640846217E-14)) ;
#38811=DIRECTION('',(-1.75658099177411E-13,-1.,-1.66321791206623E-16)) ;
#38812=DIRECTION('center_axis',(1.75658099177411E-13,1.,1.66321791206623E-16)) ;
#38813=DIRECTION('ref_axis',(-1.,1.75658099177411E-13,4.54195640846217E-14)) ;
#38814=DIRECTION('center_axis',(1.75658099177411E-13,1.,1.66321791206623E-16)) ;
#38815=DIRECTION('ref_axis',(-1.,1.75658099177411E-13,4.54195640846217E-14)) ;
#38816=DIRECTION('center_axis',(-1.75658099177411E-13,-1.,-1.66321791206623E-16)) ;
#38817=DIRECTION('ref_axis',(-4.54195640846217E-14,1.66321791214601E-16,
-1.)) ;
#38818=DIRECTION('',(-9.21791469415371E-14,-0.707106781186548,0.707106781186547)) ;
#38819=DIRECTION('center_axis',(-1.75658099177411E-13,-1.,-1.66321791206623E-16)) ;
#38820=DIRECTION('ref_axis',(1.,-1.75658099177411E-13,-4.54195640846217E-14)) ;
#38821=DIRECTION('center_axis',(1.75658099177411E-13,1.,1.66321791206623E-16)) ;
#38822=DIRECTION('ref_axis',(1.,-1.75658099177411E-13,-4.54195640846217E-14)) ;
#38823=DIRECTION('',(-1.75658099177411E-13,-1.,-1.66321791206623E-16)) ;
#38824=DIRECTION('center_axis',(1.75658099177411E-13,1.,1.66321791206623E-16)) ;
#38825=DIRECTION('ref_axis',(-1.,1.75658099177411E-13,4.54195640846217E-14)) ;
#38826=DIRECTION('center_axis',(1.75658099177411E-13,1.,1.66321791206623E-16)) ;
#38827=DIRECTION('ref_axis',(-1.,1.75658099177411E-13,4.54195640846217E-14)) ;
#38828=DIRECTION('center_axis',(-1.75658099177411E-13,-1.,-1.66321791206623E-16)) ;
#38829=DIRECTION('ref_axis',(-4.54195640846217E-14,1.66321791214601E-16,
-1.)) ;
#38830=DIRECTION('',(-9.21791469415371E-14,-0.707106781186548,0.707106781186547)) ;
#38831=DIRECTION('center_axis',(-1.,1.75658099177411E-13,4.54195640846217E-14)) ;
#38832=DIRECTION('ref_axis',(4.54195640846217E-14,-1.66321791214601E-16,
1.)) ;
#38833=DIRECTION('',(4.54195640846217E-14,-1.66321791214601E-16,1.)) ;
#38834=DIRECTION('',(1.75658099177411E-13,1.,1.66321791206623E-16)) ;
#38835=DIRECTION('',(-1.75658099177411E-13,-1.,-1.66321791206623E-16)) ;
#38836=DIRECTION('center_axis',(-4.54195640846217E-14,1.66321791214601E-16,
-1.)) ;
#38837=DIRECTION('ref_axis',(-1.,5.55236256206829E-46,4.54195640846217E-14)) ;
#38838=DIRECTION('center_axis',(-4.54195640846217E-14,1.66321791214601E-16,
-1.)) ;
#38839=DIRECTION('ref_axis',(-0.923076923076982,-0.384615384615244,4.18617815430325E-14)) ;
#38840=DIRECTION('center_axis',(-4.54195640846217E-14,1.66321791214601E-16,
-1.)) ;
#38841=DIRECTION('ref_axis',(-1.,5.55236256206829E-46,4.54195640846217E-14)) ;
#38842=DIRECTION('center_axis',(4.54195640846217E-14,-1.66321791214601E-16,
1.)) ;
#38843=DIRECTION('ref_axis',(0.923076923076847,-0.384615384615568,-4.19897213824222E-14)) ;
#38844=DIRECTION('center_axis',(1.,-1.75658099177411E-13,-4.54195640846217E-14)) ;
#38845=DIRECTION('ref_axis',(1.75658099177411E-13,1.,1.66321791206623E-16)) ;
#38846=DIRECTION('',(1.75658099177411E-13,1.,1.66321791206623E-16)) ;
#38847=DIRECTION('center_axis',(1.,-1.75658099177411E-13,-4.54195640846217E-14)) ;
#38848=DIRECTION('ref_axis',(-1.75658099177411E-13,-1.,-1.66321791206623E-16)) ;
#38849=DIRECTION('',(-1.75658099177411E-13,-1.,-1.66321791206622E-16)) ;
#38850=DIRECTION('',(1.75658099177411E-13,1.,1.66321791206623E-16)) ;
#38851=DIRECTION('center_axis',(1.,-1.75658099177411E-13,-4.54195640846217E-14)) ;
#38852=DIRECTION('ref_axis',(1.75658099177411E-13,1.,1.66321791206623E-16)) ;
#38853=DIRECTION('',(-1.75658099177411E-13,-1.,-1.66321791206623E-16)) ;
#38854=DIRECTION('',(1.75658099177411E-13,1.,1.66321791206622E-16)) ;
#38855=DIRECTION('',(-1.75658099177411E-13,-1.,-1.66321791206623E-16)) ;
#38856=DIRECTION('center_axis',(4.54195640846217E-14,-1.66321791214601E-16,
1.)) ;
#38857=DIRECTION('ref_axis',(1.,-1.75658099177411E-13,-4.54195640846217E-14)) ;
#38858=DIRECTION('',(-1.75658099177411E-13,-1.,-1.66321791206623E-16)) ;
#38859=DIRECTION('',(-1.75658099177411E-13,-1.,-1.66321791206623E-16)) ;
#38860=DIRECTION('center_axis',(1.,-1.75658099177411E-13,-4.54195640846217E-14)) ;
#38861=DIRECTION('ref_axis',(-4.54195640846217E-14,1.66321791214601E-16,
-1.)) ;
#38862=DIRECTION('',(1.75658099177411E-13,1.,1.66321791206623E-16)) ;
#38863=DIRECTION('center_axis',(-4.54195640846217E-14,1.66321791214601E-16,
-1.)) ;
#38864=DIRECTION('ref_axis',(-1.,1.75658099177411E-13,4.54195640846217E-14)) ;
#38865=DIRECTION('',(-1.75658099177411E-13,-1.,-1.66321791206623E-16)) ;
#38866=DIRECTION('center_axis',(-1.,1.75658099177411E-13,4.54195640846217E-14)) ;
#38867=DIRECTION('ref_axis',(4.54195640846217E-14,-1.66321791214601E-16,
1.)) ;
#38868=DIRECTION('center_axis',(1.,-1.75658099177411E-13,-4.54195640846217E-14)) ;
#38869=DIRECTION('ref_axis',(-4.54195640846217E-14,1.66321791214601E-16,
-1.)) ;
#38870=DIRECTION('',(-1.75658099177411E-13,-1.,-1.66321791206622E-16)) ;
#38871=DIRECTION('',(-4.54195640846217E-14,1.66321791214601E-16,-1.)) ;
#38872=DIRECTION('',(-1.75658099177411E-13,-1.,-1.66321791206622E-16)) ;
#38873=DIRECTION('center_axis',(1.75658099177411E-13,1.,1.66321791206623E-16)) ;
#38874=DIRECTION('ref_axis',(-1.,1.75658099177411E-13,4.54195640846217E-14)) ;
#38875=DIRECTION('',(-1.75658099177411E-13,-1.,-1.66321791206623E-16)) ;
#38876=DIRECTION('',(1.75658099177411E-13,1.,1.66321791206623E-16)) ;
#38877=DIRECTION('center_axis',(1.75658099177411E-13,1.,1.66321791206623E-16)) ;
#38878=DIRECTION('ref_axis',(-1.,1.75658099177411E-13,4.54195640846217E-14)) ;
#38879=DIRECTION('center_axis',(-4.54195640846217E-14,1.66321791214601E-16,
-1.)) ;
#38880=DIRECTION('ref_axis',(-1.75658099177411E-13,-1.,-1.66321791206623E-16)) ;
#38881=DIRECTION('center_axis',(4.54195640846217E-14,-1.66321791214601E-16,
1.)) ;
#38882=DIRECTION('ref_axis',(-1.,1.75658099177411E-13,4.54195640846217E-14)) ;
#38883=DIRECTION('center_axis',(4.54195640846217E-14,-1.66321791214601E-16,
1.)) ;
#38884=DIRECTION('ref_axis',(-0.923076923076982,-0.384615384615244,4.18617815430325E-14)) ;
#38885=DIRECTION('center_axis',(4.54195640846217E-14,-1.66321791214601E-16,
1.)) ;
#38886=DIRECTION('ref_axis',(-1.75658099177411E-13,-1.,-1.66321791206623E-16)) ;
#38887=DIRECTION('center_axis',(-4.54195640846217E-14,1.66321791214601E-16,
-1.)) ;
#38888=DIRECTION('ref_axis',(-1.,1.75658099177411E-13,4.54195640846217E-14)) ;
#38889=DIRECTION('',(-1.75658099177411E-13,-1.,-1.66321791206623E-16)) ;
#38890=DIRECTION('',(1.75658099177411E-13,1.,1.66321791206623E-16)) ;
#38891=DIRECTION('center_axis',(-1.,1.75658099177411E-13,4.54195640846217E-14)) ;
#38892=DIRECTION('ref_axis',(4.54195640846217E-14,-1.66321791214601E-16,
1.)) ;
#38893=DIRECTION('',(-1.75658099177411E-13,-1.,-1.66321791206623E-16)) ;
#38894=DIRECTION('center_axis',(4.54195640846217E-14,-1.66321791214601E-16,
1.)) ;
#38895=DIRECTION('ref_axis',(1.,-1.75658099177411E-13,-4.54195640846217E-14)) ;
#38896=DIRECTION('',(-1.75658099177411E-13,-1.,-1.66321791206623E-16)) ;
#38897=DIRECTION('center_axis',(1.,-1.75658099177411E-13,-4.54195640846217E-14)) ;
#38898=DIRECTION('ref_axis',(-4.54195640846217E-14,1.66321791214601E-16,
-1.)) ;
#38899=DIRECTION('center_axis',(-4.54195640846217E-14,1.66321791214601E-16,
-1.)) ;
#38900=DIRECTION('ref_axis',(-1.,1.75658099177411E-13,4.54195640846217E-14)) ;
#38901=DIRECTION('',(-1.75658099177411E-13,-1.,-1.66321791206623E-16)) ;
#38902=DIRECTION('',(1.75658099177411E-13,1.,1.66321791206623E-16)) ;
#38903=DIRECTION('center_axis',(-1.,1.75658099177411E-13,4.54195640846217E-14)) ;
#38904=DIRECTION('ref_axis',(4.54195640846217E-14,-1.66321791214601E-16,
1.)) ;
#38905=DIRECTION('',(-1.75658099177411E-13,-1.,-1.66321791206623E-16)) ;
#38906=DIRECTION('center_axis',(4.54195640846217E-14,-1.66321791214601E-16,
1.)) ;
#38907=DIRECTION('ref_axis',(1.,-1.75658099177411E-13,-4.54195640846217E-14)) ;
#38908=DIRECTION('',(-1.75658099177411E-13,-1.,-1.66321791206623E-16)) ;
#38909=DIRECTION('center_axis',(1.,-1.75658099177411E-13,-4.54195640846217E-14)) ;
#38910=DIRECTION('ref_axis',(-4.54195640846217E-14,1.66321791214601E-16,
-1.)) ;
#38911=DIRECTION('center_axis',(-1.75658099177411E-13,-1.,-1.66321791206623E-16)) ;
#38912=DIRECTION('ref_axis',(0.963207885455952,-1.73873987103648E-13,0.268757454585867)) ;
#38913=DIRECTION('center_axis',(1.,-1.75658099177411E-13,-4.54195640846217E-14)) ;
#38914=DIRECTION('ref_axis',(4.54195640846217E-14,-1.66321791214601E-16,
1.)) ;
#38915=DIRECTION('center_axis',(-4.54195640846217E-14,1.66321791214601E-16,
-1.)) ;
#38916=DIRECTION('ref_axis',(-1.75658099177411E-13,-1.,-1.66321791206623E-16)) ;
#38917=DIRECTION('center_axis',(-1.,1.75658099177411E-13,4.54195640846217E-14)) ;
#38918=DIRECTION('ref_axis',(-1.75658099177411E-13,-1.,-1.66321791206622E-16)) ;
#38919=DIRECTION('center_axis',(-1.,1.75658099177411E-13,4.54195640846217E-14)) ;
#38920=DIRECTION('ref_axis',(-1.75658099177411E-13,-1.,-1.66321791206622E-16)) ;
#38921=DIRECTION('center_axis',(-1.75658099177411E-13,-1.,-1.66321791206623E-16)) ;
#38922=DIRECTION('ref_axis',(0.268757454585866,-4.6812227297136E-14,-0.963207885455952)) ;
#38923=DIRECTION('center_axis',(-4.54195640846217E-14,1.66321791214601E-16,
-1.)) ;
#38924=DIRECTION('ref_axis',(1.,-1.75658099177411E-13,-4.54195640846217E-14)) ;
#38925=DIRECTION('center_axis',(1.,-1.75658099177411E-13,-4.54195640846217E-14)) ;
#38926=DIRECTION('ref_axis',(-1.75658099177411E-13,-1.,-1.66321791206623E-16)) ;
#38927=DIRECTION('',(1.,-1.75658099177411E-13,-4.54195640846217E-14)) ;
#38928=DIRECTION('center_axis',(1.,-1.75658099177411E-13,-4.54195640846217E-14)) ;
#38929=DIRECTION('ref_axis',(-1.75658099177411E-13,-1.,-1.66321791206623E-16)) ;
#38930=DIRECTION('center_axis',(1.,-1.75658099177411E-13,-4.54195640846217E-14)) ;
#38931=DIRECTION('ref_axis',(1.75658099177411E-13,1.,1.66321791206623E-16)) ;
#38932=DIRECTION('',(-1.75658099177411E-13,-1.,-1.66321791206622E-16)) ;
#38933=DIRECTION('',(1.75658099177411E-13,1.,1.66321791206623E-16)) ;
#38934=DIRECTION('center_axis',(-1.,1.75658099177411E-13,4.54195640846217E-14)) ;
#38935=DIRECTION('ref_axis',(-4.54195640846217E-14,1.66321791214601E-16,
-1.)) ;
#38936=DIRECTION('center_axis',(-1.,1.75658099177411E-13,4.54195640846217E-14)) ;
#38937=DIRECTION('ref_axis',(-4.54195640846217E-14,1.66321791214601E-16,
-1.)) ;
#38938=DIRECTION('',(-1.,1.75658099177411E-13,4.54195640846217E-14)) ;
#38939=DIRECTION('center_axis',(1.,-1.75658099177411E-13,-4.54195640846217E-14)) ;
#38940=DIRECTION('ref_axis',(1.75658099177411E-13,1.,1.66321791206623E-16)) ;
#38941=DIRECTION('',(-1.75658099177411E-13,-1.,-1.66321791206623E-16)) ;
#38942=DIRECTION('',(1.75658099177411E-13,1.,1.66321791206622E-16)) ;
#38943=DIRECTION('center_axis',(-4.54195640846217E-14,1.66321791214601E-16,
-1.)) ;
#38944=DIRECTION('ref_axis',(-1.75658099177411E-13,-1.,-1.66321791206623E-16)) ;
#38945=DIRECTION('center_axis',(-4.54195640846217E-14,1.66321791214601E-16,
-1.)) ;
#38946=DIRECTION('ref_axis',(-0.384615384615568,-0.923076923076847,1.73155353022032E-14)) ;
#38947=DIRECTION('center_axis',(4.54195640846217E-14,-1.66321791214601E-16,
1.)) ;
#38948=DIRECTION('ref_axis',(-1.,1.75658099177411E-13,4.54195640846217E-14)) ;
#38949=DIRECTION('center_axis',(4.54195640846217E-14,-1.66321791214601E-16,
1.)) ;
#38950=DIRECTION('ref_axis',(-1.75658099177411E-13,-1.,-1.66321791206623E-16)) ;
#38951=DIRECTION('center_axis',(-1.75658099177411E-13,-1.,-1.66321791206623E-16)) ;
#38952=DIRECTION('ref_axis',(2.14929886997261E-46,1.66321791206623E-16,
-1.)) ;
#38953=DIRECTION('',(1.,-1.75658099177411E-13,-4.54195640846217E-14)) ;
#38954=DIRECTION('',(-4.54195640846217E-14,1.66321791214601E-16,-1.)) ;
#38955=DIRECTION('',(-4.54195640846217E-14,1.66321791214601E-16,-1.)) ;
#38956=DIRECTION('center_axis',(-1.75658099177411E-13,-1.,-1.66321791206623E-16)) ;
#38957=DIRECTION('ref_axis',(1.,-1.75658099177411E-13,-4.54195640846217E-14)) ;
#38958=DIRECTION('center_axis',(0.000159104274938584,-0.999999372085354,
-0.00110928568305424)) ;
#38959=DIRECTION('ref_axis',(-0.00379983340424099,0.00110867311936705,-0.999992166024322)) ;
#38960=DIRECTION('',(-1.75658099177411E-13,-1.,-1.66321791206623E-16)) ;
#38961=DIRECTION('center_axis',(0.000159104274938584,-0.999999372085354,
-0.00110928568305424)) ;
#38962=DIRECTION('ref_axis',(-0.00379983340424099,0.00110867311936705,-0.999992166024322)) ;
#38963=DIRECTION('center_axis',(1.61486985400024E-13,1.,0.)) ;
#38964=DIRECTION('ref_axis',(0.00363593456997526,-5.87156112817037E-16,
0.999993389968055)) ;
#38965=DIRECTION('',(-0.002570993990266,0.707106781186547,-0.707102107188137)) ;
#38966=DIRECTION('center_axis',(3.1720657846433E-16,-5.63472075157877E-29,
1.)) ;
#38967=DIRECTION('ref_axis',(-1.,1.75658099177411E-13,3.1720657846433E-16)) ;
#38968=DIRECTION('',(1.77635683940029E-13,1.,0.)) ;
#38969=DIRECTION('',(-1.77635683940029E-13,-1.,0.)) ;
#38970=DIRECTION('',(-1.,1.75658099177411E-13,3.1720657846433E-16)) ;
#38971=DIRECTION('center_axis',(-1.,1.77635683940029E-13,3.28915439981538E-31)) ;
#38972=DIRECTION('ref_axis',(2.92157696951376E-29,1.66321791206623E-16,
-1.)) ;
#38973=DIRECTION('',(1.77635683940029E-13,1.,0.)) ;
#38974=DIRECTION('',(-1.77635683940029E-13,-1.,0.)) ;
#38975=DIRECTION('',(2.92157696951376E-29,1.66321791206623E-16,-1.)) ;
#38976=DIRECTION('center_axis',(-6.34413156928661E-16,1.12694415031575E-28,
-1.)) ;
#38977=DIRECTION('ref_axis',(1.,-1.75658099177411E-13,-6.34413156928661E-16)) ;
#38978=DIRECTION('',(-1.77635683940029E-13,-1.,0.)) ;
#38979=DIRECTION('',(1.,-1.75658099177411E-13,-6.34413156928661E-16)) ;
#38980=DIRECTION('',(1.77635683940029E-13,1.,0.)) ;
#38981=DIRECTION('center_axis',(1.,-1.77635683940029E-13,-3.28915439981538E-31)) ;
#38982=DIRECTION('ref_axis',(-2.92157696951376E-29,-1.66321791206623E-16,
1.)) ;
#38983=DIRECTION('',(-1.77635683940029E-13,-1.,0.)) ;
#38984=DIRECTION('',(-2.92157696951376E-29,-1.66321791206623E-16,1.)) ;
#38985=DIRECTION('',(1.77635683940029E-13,1.,0.)) ;
#38986=DIRECTION('center_axis',(-1.77635683940029E-13,-1.,0.)) ;
#38987=DIRECTION('ref_axis',(-0.707106781186573,1.25607396694709E-13,-0.707106781186523)) ;
#38988=DIRECTION('center_axis',(0.,-1.,0.)) ;
#38989=DIRECTION('ref_axis',(0.,0.,-1.)) ;
#38990=DIRECTION('center_axis',(-1.77635683940029E-13,-1.,0.)) ;
#38991=DIRECTION('ref_axis',(0.707106781186522,-1.256073966947E-13,-0.707106781186573)) ;
#38992=DIRECTION('center_axis',(0.,-1.,-5.68434188608072E-13)) ;
#38993=DIRECTION('ref_axis',(1.,0.,0.)) ;
#38994=DIRECTION('center_axis',(1.,-1.75658099177411E-13,-6.34413156928661E-16)) ;
#38995=DIRECTION('ref_axis',(1.24657630944033E-13,0.707106781186598,0.707106781186497)) ;
#38996=DIRECTION('center_axis',(-1.,1.42108547151988E-13,0.)) ;
#38997=DIRECTION('ref_axis',(0.,0.,1.)) ;
#38998=DIRECTION('center_axis',(1.,-1.42108547151988E-13,0.)) ;
#38999=DIRECTION('ref_axis',(1.42108547151988E-13,1.,0.)) ;
#39000=DIRECTION('center_axis',(-1.77635683940029E-13,-1.,0.)) ;
#39001=DIRECTION('ref_axis',(-0.707106781186573,1.25607396694709E-13,0.707106781186523)) ;
#39002=DIRECTION('center_axis',(0.,-1.,0.)) ;
#39003=DIRECTION('ref_axis',(-1.,0.,0.)) ;
#39004=DIRECTION('center_axis',(-1.,1.75658099177411E-13,3.1720657846433E-16)) ;
#39005=DIRECTION('ref_axis',(1.23984734176031E-13,0.707106781186623,-0.707106781186472)) ;
#39006=DIRECTION('center_axis',(1.,-1.42108547152069E-13,0.)) ;
#39007=DIRECTION('ref_axis',(0.,0.,-1.)) ;
#39008=DIRECTION('center_axis',(-1.,1.42108547152069E-13,0.)) ;
#39009=DIRECTION('ref_axis',(1.42108547152069E-13,1.,0.)) ;
#39010=DIRECTION('center_axis',(-1.77635683940029E-13,-1.,0.)) ;
#39011=DIRECTION('ref_axis',(0.707106781186522,-1.256073966947E-13,0.707106781186573)) ;
#39012=DIRECTION('center_axis',(-5.68434188608112E-13,-1.,0.)) ;
#39013=DIRECTION('ref_axis',(0.,0.,1.)) ;
#39014=DIRECTION('center_axis',(-2.92157696951376E-29,-1.66321791206623E-16,
1.)) ;
#39015=DIRECTION('ref_axis',(-0.707106781186347,0.707106781186749,1.17607266421309E-16)) ;
#39016=DIRECTION('center_axis',(0.,0.,-1.)) ;
#39017=DIRECTION('ref_axis',(-1.,0.,0.)) ;
#39018=DIRECTION('center_axis',(0.,0.,1.)) ;
#39019=DIRECTION('ref_axis',(1.42108547151988E-13,1.,0.)) ;
#39020=DIRECTION('center_axis',(1.42108547152069E-13,1.,0.)) ;
#39021=DIRECTION('ref_axis',(0.,0.,1.)) ;
#39022=DIRECTION('center_axis',(2.92157696951376E-29,1.66321791206623E-16,
-1.)) ;
#39023=DIRECTION('ref_axis',(0.707106781186548,0.707106781186548,1.17607266421317E-16)) ;
#39024=DIRECTION('center_axis',(0.,0.,1.)) ;
#39025=DIRECTION('ref_axis',(1.,0.,0.)) ;
#39026=DIRECTION('center_axis',(0.,0.,-1.)) ;
#39027=DIRECTION('ref_axis',(1.42108547151988E-13,1.,0.)) ;
#39028=DIRECTION('center_axis',(-1.42108547152069E-13,-1.,0.)) ;
#39029=DIRECTION('ref_axis',(0.,0.,-1.)) ;
#39030=DIRECTION('center_axis',(-1.42108547151988E-13,-1.,0.)) ;
#39031=DIRECTION('ref_axis',(0.,0.,-1.)) ;
#39032=DIRECTION('center_axis',(-1.42108547151988E-13,-1.,0.)) ;
#39033=DIRECTION('ref_axis',(0.,0.,-1.)) ;
#39034=DIRECTION('center_axis',(4.54195640846217E-14,-1.66321791214601E-16,
1.)) ;
#39035=DIRECTION('ref_axis',(1.,-1.75658099177411E-13,-4.54195640846217E-14)) ;
#39036=DIRECTION('center_axis',(-4.54195640846217E-14,1.66321791214601E-16,
-1.)) ;
#39037=DIRECTION('ref_axis',(-0.707106781186661,-0.707106781186434,3.19988744963512E-14)) ;
#39038=DIRECTION('',(-1.,1.75658099177411E-13,4.54195640846217E-14)) ;
#39039=DIRECTION('center_axis',(-4.54195640846217E-14,1.66321791214601E-16,
-1.)) ;
#39040=DIRECTION('ref_axis',(0.707106781186403,-0.707106781186692,-3.22340890291934E-14)) ;
#39041=DIRECTION('center_axis',(-4.54195640846217E-14,1.66321791214601E-16,
-1.)) ;
#39042=DIRECTION('ref_axis',(-1.,1.75658099177411E-13,4.54195640846217E-14)) ;
#39043=DIRECTION('center_axis',(-4.54195640846217E-14,1.66321791214601E-16,
-1.)) ;
#39044=DIRECTION('ref_axis',(0.707106781186648,0.707106781186447,-3.19988744963506E-14)) ;
#39045=DIRECTION('center_axis',(4.54195640846217E-14,-1.66321791214601E-16,
1.)) ;
#39046=DIRECTION('ref_axis',(0.707106781186648,0.707106781186447,-3.19988744963506E-14)) ;
#39047=DIRECTION('center_axis',(-3.10862446895045E-14,5.52202633654702E-27,
-1.)) ;
#39048=DIRECTION('ref_axis',(1.77635683940023E-13,1.,-2.00890147845606E-41)) ;
#39049=DIRECTION('',(4.54195640846217E-14,-1.66321791214601E-16,1.)) ;
#39050=DIRECTION('center_axis',(4.54195640846217E-14,-1.66321791214601E-16,
1.)) ;
#39051=DIRECTION('ref_axis',(1.,-1.75658099177411E-13,-4.54195640846217E-14)) ;
#39052=DIRECTION('center_axis',(4.54195640846217E-14,-1.66321791214601E-16,
1.)) ;
#39053=DIRECTION('ref_axis',(0.707106781186648,0.707106781186447,-3.19988744963506E-14)) ;
#39054=DIRECTION('center_axis',(4.54195640846217E-14,-1.66321791214601E-16,
1.)) ;
#39055=DIRECTION('ref_axis',(0.707106781186648,0.707106781186447,-3.19988744963506E-14)) ;
#39056=DIRECTION('',(4.54195640846217E-14,-1.66321791214601E-16,1.)) ;
#39057=DIRECTION('center_axis',(-4.54195640846217E-14,1.66321791214601E-16,
-1.)) ;
#39058=DIRECTION('ref_axis',(0.707106781186403,-0.707106781186692,-3.22340890291934E-14)) ;
#39059=DIRECTION('center_axis',(-3.77475828372543E-14,6.66133814775755E-15,
-1.)) ;
#39060=DIRECTION('ref_axis',(1.,-1.77635683940026E-13,-3.77475828372555E-14)) ;
#39061=DIRECTION('',(-4.54195640846217E-14,1.66321791214601E-16,-1.)) ;
#39062=DIRECTION('center_axis',(4.54195640846217E-14,-1.66321791214601E-16,
1.)) ;
#39063=DIRECTION('ref_axis',(-0.707106781186397,0.707106781186698,3.22340890291931E-14)) ;
#39064=DIRECTION('center_axis',(-5.1070259132759E-14,-6.66133814774199E-15,
-1.)) ;
#39065=DIRECTION('ref_axis',(-1.,1.77635683940027E-13,5.10702591327578E-14)) ;
#39066=DIRECTION('',(-4.54195640846217E-14,1.66321791214601E-16,-1.)) ;
#39067=DIRECTION('center_axis',(1.75658099177411E-13,1.,1.66321791206623E-16)) ;
#39068=DIRECTION('ref_axis',(-1.,1.75658099177411E-13,4.54195640846217E-14)) ;
#39069=DIRECTION('center_axis',(-1.75658099177411E-13,-1.,-1.66321791206623E-16)) ;
#39070=DIRECTION('ref_axis',(0.258819045102331,-4.53030069799869E-14,-0.965925826289119)) ;
#39071=DIRECTION('',(1.,-1.75658099177411E-13,-4.54195640846217E-14)) ;
#39072=DIRECTION('center_axis',(-1.75658099177411E-13,-1.,-1.66321791206623E-16)) ;
#39073=DIRECTION('ref_axis',(-0.258819045102564,4.56243160072301E-14,-0.965925826289057)) ;
#39074=DIRECTION('center_axis',(1.,-1.77635683940023E-13,-4.44089209850062E-14)) ;
#39075=DIRECTION('ref_axis',(-4.44089209850062E-14,0.,-1.)) ;
#39076=DIRECTION('center_axis',(-1.,1.75658099177411E-13,4.54195640846217E-14)) ;
#39077=DIRECTION('ref_axis',(9.20925513359143E-14,0.707106781186551,-0.707106781186544)) ;
#39078=DIRECTION('center_axis',(1.,-1.77635683940023E-13,-1.42108547152023E-13)) ;
#39079=DIRECTION('ref_axis',(-1.42108547152023E-13,0.,-1.)) ;
#39080=DIRECTION('center_axis',(-1.75658099177411E-13,-1.,-1.66321791206623E-16)) ;
#39081=DIRECTION('ref_axis',(1.,-1.75658099177411E-13,-4.54195640846217E-14)) ;
#39082=DIRECTION('center_axis',(1.75658099177411E-13,1.,1.66321791206623E-16)) ;
#39083=DIRECTION('ref_axis',(0.258819045102475,-4.53030069800122E-14,-0.965925826289081)) ;
#39084=DIRECTION('',(4.54195640846217E-14,-1.66321791214601E-16,1.)) ;
#39085=DIRECTION('center_axis',(1.75658099177411E-13,1.,1.66321791206623E-16)) ;
#39086=DIRECTION('ref_axis',(-0.258819045102557,4.56243160072289E-14,-0.965925826289059)) ;
#39087=DIRECTION('',(-1.,1.75658099177411E-13,4.54195640846217E-14)) ;
#39088=DIRECTION('center_axis',(-4.54195640846217E-14,1.66321791214601E-16,
-1.)) ;
#39089=DIRECTION('ref_axis',(-0.707106781186661,-0.707106781186434,3.19988744963512E-14)) ;
#39090=DIRECTION('center_axis',(-5.77315972805084E-14,8.71691300269209E-27,
-1.)) ;
#39091=DIRECTION('ref_axis',(-1.50990331349019E-13,-1.,-2.86985925493723E-42)) ;
#39092=DIRECTION('center_axis',(-1.,1.77635683940029E-13,4.44089209850064E-14)) ;
#39093=DIRECTION('ref_axis',(-4.44089209850064E-14,0.,-1.)) ;
#39094=DIRECTION('center_axis',(1.,-1.75658099177411E-13,-4.54195640846217E-14)) ;
#39095=DIRECTION('ref_axis',(-1.5632551486146E-13,-0.707106781186551,-0.707106781186544)) ;
#39096=DIRECTION('center_axis',(-1.,1.77635683940023E-13,2.66453525910034E-14)) ;
#39097=DIRECTION('ref_axis',(-2.66453525910034E-14,0.,-1.)) ;
#39098=DIRECTION('center_axis',(4.54195640846217E-14,-1.66321791214601E-16,
1.)) ;
#39099=DIRECTION('ref_axis',(1.75658099177411E-13,1.,1.66321791206623E-16)) ;
#39100=DIRECTION('',(-0.866025403784439,-0.5,3.92513354304904E-14)) ;
#39101=DIRECTION('',(1.36574054430667E-16,-1.,-1.66321791214607E-16)) ;
#39102=DIRECTION('',(0.866025403784438,-0.5,-3.9417657221705E-14)) ;
#39103=DIRECTION('',(0.866025403784438,0.5,-3.92513354304904E-14)) ;
#39104=DIRECTION('',(-1.58057336172267E-29,1.,1.66321791214601E-16)) ;
#39105=DIRECTION('',(-0.866025403784439,0.5,3.9417657221705E-14)) ;
#39106=DIRECTION('',(-0.866025403784439,-0.5,3.92513354304904E-14)) ;
#39107=DIRECTION('',(8.10629031994341E-17,-1.,-1.66321791214605E-16)) ;
#39108=DIRECTION('',(0.866025403784438,-0.5,-3.9417657221705E-14)) ;
#39109=DIRECTION('',(0.866025403784438,0.5,-3.92513354304904E-14)) ;
#39110=DIRECTION('',(5.55111512312168E-17,1.,1.66321791214598E-16)) ;
#39111=DIRECTION('',(-0.866025403784439,0.5,3.9417657221705E-14)) ;
#39112=DIRECTION('',(-0.866025403784439,-0.5,3.92513354304904E-14)) ;
#39113=DIRECTION('',(1.36574054430641E-16,-1.,-1.66321791214607E-16)) ;
#39114=DIRECTION('',(0.866025403784438,-0.5,-3.9417657221705E-14)) ;
#39115=DIRECTION('',(0.866025403784438,0.5,-3.92513354304904E-14)) ;
#39116=DIRECTION('',(9.43781534984571E-30,1.,1.66321791214601E-16)) ;
#39117=DIRECTION('',(-0.866025403784439,0.5,3.9417657221705E-14)) ;
#39118=DIRECTION('center_axis',(-0.5,-0.866025403784439,-7.35195579201608E-14)) ;
#39119=DIRECTION('ref_axis',(0.866025403784439,-0.5,-4.25106353121199E-14)) ;
#39120=DIRECTION('',(0.866025403784439,-0.5,-3.9417657221705E-14)) ;
#39121=DIRECTION('',(-5.55111512312578E-17,8.49251224899206E-14,-1.)) ;
#39122=DIRECTION('',(-5.55111512312578E-17,8.49251224899206E-14,-1.)) ;
#39123=DIRECTION('center_axis',(-1.,0.,5.55111512312578E-17)) ;
#39124=DIRECTION('ref_axis',(-4.71429131787108E-30,-1.,-8.49251224899206E-14)) ;
#39125=DIRECTION('',(-9.2327141051674E-33,-1.,-1.66321791214601E-16)) ;
#39126=DIRECTION('',(-5.55111512312578E-17,8.49251224899206E-14,-1.)) ;
#39127=DIRECTION('center_axis',(0.5,-0.866025403784439,-7.3575069071392E-14)) ;
#39128=DIRECTION('ref_axis',(0.866025403784439,0.5,4.24144871778007E-14)) ;
#39129=DIRECTION('',(0.866025403784439,0.5,-3.92513354304904E-14)) ;
#39130=DIRECTION('',(-5.55111512312578E-17,8.49251224899206E-14,-1.)) ;
#39131=DIRECTION('center_axis',(1.,1.36574054430651E-16,-5.55111512312462E-17)) ;
#39132=DIRECTION('ref_axis',(-1.36574054430646E-16,1.,8.49251224899206E-14)) ;
#39133=DIRECTION('',(-1.36574054430651E-16,1.,1.66321791214607E-16)) ;
#39134=DIRECTION('',(-5.55111512312578E-17,8.49251224899206E-14,-1.)) ;
#39135=DIRECTION('center_axis',(0.5,0.866025403784439,7.35195579201608E-14)) ;
#39136=DIRECTION('ref_axis',(-0.866025403784439,0.5,4.25106353121199E-14)) ;
#39137=DIRECTION('',(-0.866025403784438,0.5,3.9417657221705E-14)) ;
#39138=DIRECTION('',(-5.55111512312578E-17,8.49251224899206E-14,-1.)) ;
#39139=DIRECTION('center_axis',(-0.5,0.866025403784438,7.3575069071392E-14)) ;
#39140=DIRECTION('ref_axis',(-0.866025403784438,-0.5,-4.24144871778007E-14)) ;
#39141=DIRECTION('',(-0.866025403784438,-0.5,3.92513354304904E-14)) ;
#39142=DIRECTION('center_axis',(-0.5,-0.866025403784439,-7.35195579201539E-14)) ;
#39143=DIRECTION('ref_axis',(0.866025403784439,-0.5,-4.25106353121159E-14)) ;
#39144=DIRECTION('',(0.866025403784439,-0.5,-3.9417657221705E-14)) ;
#39145=DIRECTION('',(-5.55111512312187E-17,8.49251224899126E-14,-1.)) ;
#39146=DIRECTION('',(-5.55111512312187E-17,8.49251224899127E-14,-1.)) ;
#39147=DIRECTION('center_axis',(-1.,-2.52435489670719E-29,5.55111512312187E-17)) ;
#39148=DIRECTION('ref_axis',(2.05292576492046E-29,-1.,-8.49251224899126E-14)) ;
#39149=DIRECTION('',(2.52343162529668E-29,-1.,-1.66321791214601E-16)) ;
#39150=DIRECTION('',(-5.55111512312187E-17,8.49251224899127E-14,-1.)) ;
#39151=DIRECTION('center_axis',(0.5,-0.866025403784439,-7.35750690713851E-14)) ;
#39152=DIRECTION('ref_axis',(0.866025403784439,0.5,4.24144871777968E-14)) ;
#39153=DIRECTION('',(0.866025403784439,0.5,-3.92513354304904E-14)) ;
#39154=DIRECTION('',(-5.55111512312187E-17,8.49251224899127E-14,-1.)) ;
#39155=DIRECTION('center_axis',(1.,1.36574054430676E-16,-5.55111512312071E-17)) ;
#39156=DIRECTION('ref_axis',(-1.36574054430671E-16,1.,8.49251224899126E-14)) ;
#39157=DIRECTION('',(-1.36574054430676E-16,1.,1.66321791214607E-16)) ;
#39158=DIRECTION('',(-5.55111512312187E-17,8.49251224899127E-14,-1.)) ;
#39159=DIRECTION('center_axis',(0.5,0.866025403784439,7.35195579201539E-14)) ;
#39160=DIRECTION('ref_axis',(-0.866025403784439,0.5,4.25106353121159E-14)) ;
#39161=DIRECTION('',(-0.866025403784438,0.5,3.9417657221705E-14)) ;
#39162=DIRECTION('',(-5.55111512312187E-17,8.49251224899126E-14,-1.)) ;
#39163=DIRECTION('center_axis',(-0.5,0.866025403784438,7.35750690713851E-14)) ;
#39164=DIRECTION('ref_axis',(-0.866025403784438,-0.5,-4.24144871777968E-14)) ;
#39165=DIRECTION('',(-0.866025403784438,-0.5,3.92513354304904E-14)) ;
#39166=DIRECTION('center_axis',(4.54195640846217E-14,-1.66321791214601E-16,
1.)) ;
#39167=DIRECTION('ref_axis',(1.75658099177411E-13,1.,1.66321791206623E-16)) ;
#39168=DIRECTION('',(0.866025403784439,0.5,-3.92513354304904E-14)) ;
#39169=DIRECTION('',(0.866025403784439,-0.5,-3.9417657221705E-14)) ;
#39170=DIRECTION('',(-5.55111512312074E-17,-1.,-1.66321791214598E-16)) ;
#39171=DIRECTION('',(-0.866025403784438,-0.5,3.92513354304904E-14)) ;
#39172=DIRECTION('',(-0.866025403784438,0.5,3.9417657221705E-14)) ;
#39173=DIRECTION('',(-8.10629031994436E-17,1.,1.66321791214605E-16)) ;
#39174=DIRECTION('center_axis',(-0.5,-0.866025403784439,-7.34978569193033E-14)) ;
#39175=DIRECTION('ref_axis',(0.866025403784439,-0.5,-4.2499867027259E-14)) ;
#39176=DIRECTION('',(-5.70360434152559E-17,8.490094472946E-14,-1.)) ;
#39177=DIRECTION('',(-5.70360434152559E-17,8.490094472946E-14,-1.)) ;
#39178=DIRECTION('center_axis',(-1.,5.55111512312073E-17,5.70360434152606E-17)) ;
#39179=DIRECTION('ref_axis',(-5.55111512312121E-17,-1.,-8.490094472946E-14)) ;
#39180=DIRECTION('',(-5.70360434152559E-17,8.490094472946E-14,-1.)) ;
#39181=DIRECTION('center_axis',(0.5,-0.866025403784439,-7.35548929627185E-14)) ;
#39182=DIRECTION('ref_axis',(0.866025403784439,0.5,4.2401077702201E-14)) ;
#39183=DIRECTION('',(-5.70360434152559E-17,8.490094472946E-14,-1.)) ;
#39184=DIRECTION('center_axis',(1.,8.10629031994436E-17,-5.7036043415249E-17)) ;
#39185=DIRECTION('ref_axis',(-8.10629031994388E-17,1.,8.490094472946E-14)) ;
#39186=DIRECTION('',(-5.70360434152559E-17,8.490094472946E-14,-1.)) ;
#39187=DIRECTION('center_axis',(0.5,0.866025403784439,7.34978569193033E-14)) ;
#39188=DIRECTION('ref_axis',(-0.866025403784439,0.5,4.2499867027259E-14)) ;
#39189=DIRECTION('',(-5.70360434152559E-17,8.490094472946E-14,-1.)) ;
#39190=DIRECTION('center_axis',(-0.5,0.866025403784438,7.35548929627185E-14)) ;
#39191=DIRECTION('ref_axis',(-0.866025403784438,-0.5,-4.24010777022011E-14)) ;
#39192=DIRECTION('',(0.,0.,1.)) ;
#39193=DIRECTION('',(1.,0.,0.)) ;
#39194=DIRECTION('',(0.,0.,1.)) ;
#39195=DIRECTION('',(1.,0.,0.)) ;
#47173=CARTESIAN_POINT('',(0.,0.,0.)) ;
#50225=CARTESIAN_POINT('Origin',(179.888527625416,585.710565160536,-51.0680854522974)) ;
#50226=CARTESIAN_POINT('',(178.636459939217,587.33977480686,-47.7297342831525)) ;
#50227=CARTESIAN_POINT('',(178.636459895391,587.339774773179,-47.671523035887)) ;
#50228=CARTESIAN_POINT('',(178.636459914529,587.339774787887,-51.0680854522974)) ;
#50229=CARTESIAN_POINT('',(178.005900115752,584.887332980433,-47.5221601717597)) ;
#50230=CARTESIAN_POINT('Ctrl Pts',(178.636459895391,587.339774773179,-47.6715230358871)) ;
#50231=CARTESIAN_POINT('Ctrl Pts',(178.622051948503,587.328702087864,-47.6704668912743)) ;
#50232=CARTESIAN_POINT('Ctrl Pts',(178.607789560242,587.317437260344,-47.6694051968374)) ;
#50233=CARTESIAN_POINT('Ctrl Pts',(178.487045236967,587.219440421823,-47.6602809317652)) ;
#50234=CARTESIAN_POINT('Ctrl Pts',(178.389364918817,587.12243134586,-47.6519504773091)) ;
#50235=CARTESIAN_POINT('Ctrl Pts',(178.270018935768,586.97744097979,-47.6409601002178)) ;
#50236=CARTESIAN_POINT('Ctrl Pts',(178.239388517243,586.937302978343,-47.6380533492227)) ;
#50237=CARTESIAN_POINT('Ctrl Pts',(178.193017158957,586.87165754715,-47.6335619409714)) ;
#50238=CARTESIAN_POINT('Ctrl Pts',(178.176303322685,586.846865984155,-47.6319234492914)) ;
#50239=CARTESIAN_POINT('Ctrl Pts',(178.13743793732,586.786410828827,-47.6280712936817)) ;
#50240=CARTESIAN_POINT('Ctrl Pts',(178.11582742136,586.750417784659,-47.6258889309011)) ;
#50241=CARTESIAN_POINT('Ctrl Pts',(178.041476930324,586.61752088359,-47.6181384242265)) ;
#50242=CARTESIAN_POINT('Ctrl Pts',(177.99545548892,586.517067886397,-47.6128483931015)) ;
#50243=CARTESIAN_POINT('Ctrl Pts',(177.913341108927,586.291485316647,-47.601291085922)) ;
#50244=CARTESIAN_POINT('Ctrl Pts',(177.880612878398,586.165652951717,-47.5950305003944)) ;
#50245=CARTESIAN_POINT('Ctrl Pts',(177.850497749422,585.97884066761,-47.5853775866719)) ;
#50246=CARTESIAN_POINT('Ctrl Pts',(177.843585084823,585.919722142574,-47.5822759537453)) ;
#50247=CARTESIAN_POINT('Ctrl Pts',(177.835183898614,585.804812341749,-47.576118591322)) ;
#50248=CARTESIAN_POINT('Ctrl Pts',(177.833383449117,585.749095971256,-47.5730751020488)) ;
#50249=CARTESIAN_POINT('Ctrl Pts',(177.834968265367,585.559629255589,-47.5625121835925)) ;
#50250=CARTESIAN_POINT('Ctrl Pts',(177.849141441219,585.426323248145,-47.5546957485577)) ;
#50251=CARTESIAN_POINT('Ctrl Pts',(177.896728318326,585.1956967431,-47.5408154361288)) ;
#50252=CARTESIAN_POINT('Ctrl Pts',(177.924657234882,585.097736004592,-47.5348091115553)) ;
#50253=CARTESIAN_POINT('Ctrl Pts',(177.967607229132,584.980780886296,-47.527743521705)) ;
#50254=CARTESIAN_POINT('Ctrl Pts',(177.975846412108,584.95945204961,-47.5264597113805)) ;
#50255=CARTESIAN_POINT('Ctrl Pts',(177.991364576761,584.921192414976,-47.5241702591099)) ;
#50256=CARTESIAN_POINT('Ctrl Pts',(177.998518536886,584.904213714415,-47.5231591248557)) ;
#50257=CARTESIAN_POINT('Ctrl Pts',(178.005900115752,584.887332980433,-47.5221601717597)) ;
#50258=CARTESIAN_POINT('',(178.665796911972,584.056482856676,-47.523444591023)) ;
#50259=CARTESIAN_POINT('Origin',(179.888527625416,585.710565160536,-47.5221601717598)) ;
#50260=CARTESIAN_POINT('Ctrl Pts',(178.666885451598,584.058418689533,-47.5247290102857)) ;
#50261=CARTESIAN_POINT('Ctrl Pts',(178.653511313722,584.068307891946,-47.525627662434)) ;
#50262=CARTESIAN_POINT('Ctrl Pts',(178.640257270952,584.078359478669,-47.5265153396178)) ;
#50263=CARTESIAN_POINT('Ctrl Pts',(178.609645663288,584.102165685899,-47.5285624606179)) ;
#50264=CARTESIAN_POINT('Ctrl Pts',(178.592385307971,584.116042314304,-47.5297143830976)) ;
#50265=CARTESIAN_POINT('Ctrl Pts',(178.481292589341,584.20835253247,-47.5371376308387)) ;
#50266=CARTESIAN_POINT('Ctrl Pts',(178.394389987336,584.294757521546,-47.542999568097)) ;
#50267=CARTESIAN_POINT('Ctrl Pts',(178.239218126975,584.479347585433,-47.5546974006364)) ;
#50268=CARTESIAN_POINT('Ctrl Pts',(178.170792702272,584.576765419694,-47.5605112595867)) ;
#50269=CARTESIAN_POINT('Ctrl Pts',(178.084524128559,584.725481636807,-47.5693820913402)) ;
#50270=CARTESIAN_POINT('Ctrl Pts',(178.0596681154,584.772433838276,-47.5721793006139)) ;
#50271=CARTESIAN_POINT('Ctrl Pts',(178.013698342065,584.868056265502,-47.5778991786517)) ;
#50272=CARTESIAN_POINT('Ctrl Pts',(177.992594836705,584.916685944811,-47.5808193878186)) ;
#50273=CARTESIAN_POINT('Ctrl Pts',(177.933181634483,585.06952069295,-47.5900474878534)) ;
#50274=CARTESIAN_POINT('Ctrl Pts',(177.901420110829,585.176042772451,-47.596561393858)) ;
#50275=CARTESIAN_POINT('Ctrl Pts',(177.85864488408,585.377895156172,-47.6088857426835)) ;
#50276=CARTESIAN_POINT('Ctrl Pts',(177.845393105198,585.472458198085,-47.6146479075646)) ;
#50277=CARTESIAN_POINT('Ctrl Pts',(177.835876382909,585.60890486476,-47.6227188470256)) ;
#50278=CARTESIAN_POINT('Ctrl Pts',(177.834244503055,585.650289489834,-47.6251338894464)) ;
#50279=CARTESIAN_POINT('Ctrl Pts',(177.833548232647,585.726111104898,-47.629466674811)) ;
#50280=CARTESIAN_POINT('Ctrl Pts',(177.834096847837,585.760529887158,-47.6313988241779)) ;
#50281=CARTESIAN_POINT('Ctrl Pts',(177.836784129112,585.825931992355,-47.6349835616902)) ;
#50282=CARTESIAN_POINT('Ctrl Pts',(177.838760818321,585.856910608852,-47.6366427024279)) ;
#50283=CARTESIAN_POINT('Ctrl Pts',(177.847662721803,585.959709543268,-47.6420513037143)) ;
#50284=CARTESIAN_POINT('Ctrl Pts',(177.857668629265,586.031214532293,-47.6456573976396)) ;
#50285=CARTESIAN_POINT('Ctrl Pts',(177.903134627704,586.265476184802,-47.6573654666969)) ;
#50286=CARTESIAN_POINT('Ctrl Pts',(177.954593475042,586.424435928558,-47.6651906308011)) ;
#50287=CARTESIAN_POINT('Ctrl Pts',(178.049939653255,586.629910935619,-47.6766599426331)) ;
#50288=CARTESIAN_POINT('Ctrl Pts',(178.077584741966,586.683235374413,-47.6797657868005)) ;
#50289=CARTESIAN_POINT('Ctrl Pts',(178.132378598873,586.778470706083,-47.6856030880404)) ;
#50290=CARTESIAN_POINT('Ctrl Pts',(178.158796050686,586.820749708351,-47.6883063300768)) ;
#50291=CARTESIAN_POINT('Ctrl Pts',(178.22743122292,586.922189413675,-47.6950902412122)) ;
#50292=CARTESIAN_POINT('Ctrl Pts',(178.271297572279,586.980147673663,-47.699231731675)) ;
#50293=CARTESIAN_POINT('Ctrl Pts',(178.413054389223,587.148146249744,-47.7120490358254)) ;
#50294=CARTESIAN_POINT('Ctrl Pts',(178.519774316991,587.250100468531,-47.7210107004045)) ;
#50295=CARTESIAN_POINT('Ctrl Pts',(178.636459939217,587.33977480686,-47.7297342831524)) ;
#50296=CARTESIAN_POINT('Origin',(179.888527625416,585.710565160536,-51.0680854522974)) ;
#50297=CARTESIAN_POINT('',(178.636459914536,587.339774787892,-48.4293959864655)) ;
#50298=CARTESIAN_POINT('',(178.636459914529,587.339774787887,-48.3712343220044)) ;
#50299=CARTESIAN_POINT('',(178.636459914529,587.339774787887,-51.0680854522974)) ;
#50300=CARTESIAN_POINT('',(181.94327755488,585.71002676683,-47.9194602314969)) ;
#50301=CARTESIAN_POINT('Ctrl Pts',(178.636459914529,587.339774787887,-48.3712343220044)) ;
#50302=CARTESIAN_POINT('Ctrl Pts',(178.616732770872,587.324614234459,-48.3699812011576)) ;
#50303=CARTESIAN_POINT('Ctrl Pts',(178.597273587933,587.309089704676,-48.3687167206434)) ;
#50304=CARTESIAN_POINT('Ctrl Pts',(178.535957355158,587.258319596,-48.3646324682209)) ;
#50305=CARTESIAN_POINT('Ctrl Pts',(178.49523514045,587.221765161574,-48.3617663414953)) ;
#50306=CARTESIAN_POINT('Ctrl Pts',(178.418883875532,587.147516231435,-48.3560489276152)) ;
#50307=CARTESIAN_POINT('Ctrl Pts',(178.383127531142,587.110011835591,-48.3532070584353)) ;
#50308=CARTESIAN_POINT('Ctrl Pts',(178.285318242291,586.999330403391,-48.3449298370018)) ;
#50309=CARTESIAN_POINT('Ctrl Pts',(178.226925342831,586.923112147398,-48.3393511592422)) ;
#50310=CARTESIAN_POINT('Ctrl Pts',(178.098656363484,586.728936491659,-48.3255182844141)) ;
#50311=CARTESIAN_POINT('Ctrl Pts',(178.034833883732,586.607525688292,-48.3171593759884)) ;
#50312=CARTESIAN_POINT('Ctrl Pts',(177.966076214654,586.437443706439,-48.3064290896158)) ;
#50313=CARTESIAN_POINT('Ctrl Pts',(177.950075089051,586.393627581319,-48.303749038531)) ;
#50314=CARTESIAN_POINT('Ctrl Pts',(177.926513557381,586.321587738282,-48.2995201732169)) ;
#50315=CARTESIAN_POINT('Ctrl Pts',(177.918040449193,586.293684649819,-48.2979262294828)) ;
#50316=CARTESIAN_POINT('Ctrl Pts',(177.898407146047,586.223704463639,-48.2940379135337)) ;
#50317=CARTESIAN_POINT('Ctrl Pts',(177.887984843604,586.181437314423,-48.2917817422532)) ;
#50318=CARTESIAN_POINT('Ctrl Pts',(177.866532065166,586.080779991881,-48.2865581034063)) ;
#50319=CARTESIAN_POINT('Ctrl Pts',(177.856675638199,586.022179185615,-48.283633345089)) ;
#50320=CARTESIAN_POINT('Ctrl Pts',(177.828623120527,585.795779535687,-48.2725167961253)) ;
#50321=CARTESIAN_POINT('Ctrl Pts',(177.82857950266,585.626422692747,-48.2645227019426)) ;
#50322=CARTESIAN_POINT('Ctrl Pts',(177.85586501095,585.405265518843,-48.2530683432249)) ;
#50323=CARTESIAN_POINT('Ctrl Pts',(177.864608379056,585.351851706924,-48.2502282743187)) ;
#50324=CARTESIAN_POINT('Ctrl Pts',(177.885916441807,585.247666537071,-48.2445106014221)) ;
#50325=CARTESIAN_POINT('Ctrl Pts',(177.898331449846,585.196906556028,-48.2416398273973)) ;
#50326=CARTESIAN_POINT('Ctrl Pts',(177.940788212944,585.048138059375,-48.2329551796179)) ;
#50327=CARTESIAN_POINT('Ctrl Pts',(177.97623875876,584.951852304478,-48.2269703149639)) ;
#50328=CARTESIAN_POINT('Ctrl Pts',(178.074597442009,584.735978691476,-48.2128257421043)) ;
#50329=CARTESIAN_POINT('Ctrl Pts',(178.14240753163,584.619131848229,-48.204600120584)) ;
#50330=CARTESIAN_POINT('Ctrl Pts',(178.24625653502,584.474933400225,-48.1942621728566)) ;
#50331=CARTESIAN_POINT('Ctrl Pts',(178.272429697812,584.440892678788,-48.1918088082005)) ;
#50332=CARTESIAN_POINT('Ctrl Pts',(178.318180262506,584.385098984106,-48.1877999845216)) ;
#50333=CARTESIAN_POINT('Ctrl Pts',(178.337186839399,584.362902980642,-48.18621087511)) ;
#50334=CARTESIAN_POINT('Ctrl Pts',(178.388377929359,584.305640700901,-48.1821201130052)) ;
#50335=CARTESIAN_POINT('Ctrl Pts',(178.421317200854,584.271275027624,-48.1796696874536)) ;
#50336=CARTESIAN_POINT('Ctrl Pts',(178.504763121472,584.190060672954,-48.1737998996133)) ;
#50337=CARTESIAN_POINT('Ctrl Pts',(178.556488879704,584.144547337068,-48.1704397252974)) ;
#50338=CARTESIAN_POINT('Ctrl Pts',(178.729431106123,584.007156360584,-48.1597264770878)) ;
#50339=CARTESIAN_POINT('Ctrl Pts',(178.858572523721,583.926105746112,-48.1524478137044)) ;
#50340=CARTESIAN_POINT('Ctrl Pts',(179.044017713304,583.836610388659,-48.141857130019)) ;
#50341=CARTESIAN_POINT('Ctrl Pts',(179.093466176679,583.815102140579,-48.1390260709258)) ;
#50342=CARTESIAN_POINT('Ctrl Pts',(179.192436484254,583.776608278394,-48.133313773514)) ;
#50343=CARTESIAN_POINT('Ctrl Pts',(179.241874965903,583.759521407952,-48.1304387269888)) ;
#50344=CARTESIAN_POINT('Ctrl Pts',(179.391229339971,583.714202241957,-48.1216725489935)) ;
#50345=CARTESIAN_POINT('Ctrl Pts',(179.492678663355,583.691637391317,-48.1156042010222)) ;
#50346=CARTESIAN_POINT('Ctrl Pts',(179.728553311563,583.657638598557,-48.101381247454)) ;
#50347=CARTESIAN_POINT('Ctrl Pts',(179.863282043351,583.651569615006,-48.0931669054093)) ;
#50348=CARTESIAN_POINT('Ctrl Pts',(180.039958209376,583.660964602471,-48.0828789164744)) ;
#50349=CARTESIAN_POINT('Ctrl Pts',(180.082202386195,583.664524036193,-48.0804580024299)) ;
#50350=CARTESIAN_POINT('Ctrl Pts',(180.153271647572,583.672733423954,-48.0764846107144)) ;
#50351=CARTESIAN_POINT('Ctrl Pts',(180.182157092363,583.6766945972,-48.0748998497865)) ;
#50352=CARTESIAN_POINT('Ctrl Pts',(180.258192238367,583.688775492105,-48.0708011130373)) ;
#50353=CARTESIAN_POINT('Ctrl Pts',(180.305158046741,583.697928790143,-48.0683394527122)) ;
#50354=CARTESIAN_POINT('Ctrl Pts',(180.419476518232,583.724382584651,-48.0624282559596)) ;
#50355=CARTESIAN_POINT('Ctrl Pts',(180.486353181931,583.743477588543,-48.0590392477585)) ;
#50356=CARTESIAN_POINT('Ctrl Pts',(180.694272382868,583.814430075535,-48.0483888442308)) ;
#50357=CARTESIAN_POINT('Ctrl Pts',(180.830650194738,583.878365781271,-48.0411953677898)) ;
#50358=CARTESIAN_POINT('Ctrl Pts',(181.004812856034,583.984643594465,-48.0307080167695)) ;
#50359=CARTESIAN_POINT('Ctrl Pts',(181.04966096301,584.014491273626,-48.0278813501209)) ;
#50360=CARTESIAN_POINT('Ctrl Pts',(181.135276784856,584.076459447805,-48.0221990740497)) ;
#50361=CARTESIAN_POINT('Ctrl Pts',(181.176102652813,584.108430709867,-48.0193506201744)) ;
#50362=CARTESIAN_POINT('Ctrl Pts',(181.291326405921,584.205914651208,-48.0108786437663)) ;
#50363=CARTESIAN_POINT('Ctrl Pts',(181.362240599236,584.275300928053,-48.0050970984169)) ;
#50364=CARTESIAN_POINT('Ctrl Pts',(181.518388855748,584.451904723304,-47.9910442369297)) ;
#50365=CARTESIAN_POINT('Ctrl Pts',(181.598469878208,584.563058691308,-47.9826831206871)) ;
#50366=CARTESIAN_POINT('Ctrl Pts',(181.689454312248,584.720270284086,-47.9720696293225)) ;
#50367=CARTESIAN_POINT('Ctrl Pts',(181.710702755804,584.759934171019,-47.9694875488808)) ;
#50368=CARTESIAN_POINT('Ctrl Pts',(181.743589097101,584.826483883817,-47.965349145489)) ;
#50369=CARTESIAN_POINT('Ctrl Pts',(181.755982737469,584.852972977259,-47.9637529047783)) ;
#50370=CARTESIAN_POINT('Ctrl Pts',(181.786209978292,584.921343895791,-47.959757070883)) ;
#50371=CARTESIAN_POINT('Ctrl Pts',(181.803224687991,584.963568325523,-47.9574015053188)) ;
#50372=CARTESIAN_POINT('Ctrl Pts',(181.840670292856,585.066205485159,-47.9518637578263)) ;
#50373=CARTESIAN_POINT('Ctrl Pts',(181.859719488281,585.127072365383,-47.9487308504889)) ;
#50374=CARTESIAN_POINT('Ctrl Pts',(181.908742796499,585.313774658712,-47.9393219140778)) ;
#50375=CARTESIAN_POINT('Ctrl Pts',(181.929700552961,585.441634024675,-47.933129186118)) ;
#50376=CARTESIAN_POINT('Ctrl Pts',(181.94167411048,585.617020177267,-47.924269032645)) ;
#50377=CARTESIAN_POINT('Ctrl Pts',(181.943265368409,585.663517772867,-47.9218881440502)) ;
#50378=CARTESIAN_POINT('Ctrl Pts',(181.94327755488,585.71002676683,-47.9194602314969)) ;
#50379=CARTESIAN_POINT('Ctrl Pts',(181.943277555182,585.710027921507,-47.9194601712192)) ;
#50380=CARTESIAN_POINT('Ctrl Pts',(181.943288990901,585.753765513704,-47.9171769336477)) ;
#50381=CARTESIAN_POINT('Ctrl Pts',(181.941903931433,585.797490452821,-47.9148533307488)) ;
#50382=CARTESIAN_POINT('Ctrl Pts',(181.935789748451,585.893512517472,-47.9096434456928)) ;
#50383=CARTESIAN_POINT('Ctrl Pts',(181.93044953608,585.945737714692,-47.906739351913)) ;
#50384=CARTESIAN_POINT('Ctrl Pts',(181.899647721926,586.163995586748,-47.8942856313623)) ;
#50385=CARTESIAN_POINT('Ctrl Pts',(181.855881423971,586.326767122333,-47.8841510595223)) ;
#50386=CARTESIAN_POINT('Ctrl Pts',(181.75964674558,586.564209951801,-47.8687596087727)) ;
#50387=CARTESIAN_POINT('Ctrl Pts',(181.721231234971,586.643836981885,-47.8634994713564)) ;
#50388=CARTESIAN_POINT('Ctrl Pts',(181.661916626856,586.748897381278,-47.8566364834576)) ;
#50389=CARTESIAN_POINT('Ctrl Pts',(181.645362047115,586.77666813238,-47.8548307418738)) ;
#50390=CARTESIAN_POINT('Ctrl Pts',(181.610228564451,586.832562699905,-47.8512317357504)) ;
#50391=CARTESIAN_POINT('Ctrl Pts',(181.591599632597,586.860642824386,-47.8494417739713)) ;
#50392=CARTESIAN_POINT('Ctrl Pts',(181.499143100928,586.992829358914,-47.8410397257878)) ;
#50393=CARTESIAN_POINT('Ctrl Pts',(181.416407412661,587.090374540805,-47.8349004729119)) ;
#50394=CARTESIAN_POINT('Ctrl Pts',(181.238320119738,587.264529957423,-47.8227993555768)) ;
#50395=CARTESIAN_POINT('Ctrl Pts',(181.144140809479,587.341570526276,-47.816862729015)) ;
#50396=CARTESIAN_POINT('Ctrl Pts',(180.999202436521,587.440101645439,-47.8078192845947)) ;
#50397=CARTESIAN_POINT('Ctrl Pts',(180.953518174105,587.468600829704,-47.8049837135906)) ;
#50398=CARTESIAN_POINT('Ctrl Pts',(180.860202423943,587.521840987488,-47.7991886966417)) ;
#50399=CARTESIAN_POINT('Ctrl Pts',(180.81261595788,587.546574972235,-47.7962320466396)) ;
#50400=CARTESIAN_POINT('Ctrl Pts',(180.661739375481,587.617643700048,-47.7868355248201)) ;
#50401=CARTESIAN_POINT('Ctrl Pts',(180.555562932533,587.657322204198,-47.7801787748269)) ;
#50402=CARTESIAN_POINT('Ctrl Pts',(180.355034759728,587.713921164562,-47.7677030782489)) ;
#50403=CARTESIAN_POINT('Ctrl Pts',(180.261708858907,587.733385049441,-47.7619375674298)) ;
#50404=CARTESIAN_POINT('Ctrl Pts',(180.111160795272,587.754006052561,-47.7529542111146)) ;
#50405=CARTESIAN_POINT('Ctrl Pts',(180.054653005402,587.759374472618,-47.7496539479627)) ;
#50406=CARTESIAN_POINT('Ctrl Pts',(179.968584681763,587.763966155414,-47.7448051540227)) ;
#50407=CARTESIAN_POINT('Ctrl Pts',(179.939144838034,587.764902772479,-47.7431783160048)) ;
#50408=CARTESIAN_POINT('Ctrl Pts',(179.875210140234,587.765561347818,-47.7397285817788)) ;
#50409=CARTESIAN_POINT('Ctrl Pts',(179.840722482333,587.765048471467,-47.7379186989338)) ;
#50410=CARTESIAN_POINT('Ctrl Pts',(179.693339667233,587.759142986261,-47.7303405527453)) ;
#50411=CARTESIAN_POINT('Ctrl Pts',(179.580971023856,587.745309284466,-47.7249485680904)) ;
#50412=CARTESIAN_POINT('Ctrl Pts',(179.33415706429,587.693998335569,-47.7129334424596)) ;
#50413=CARTESIAN_POINT('Ctrl Pts',(179.201250395347,587.651951304077,-47.7063258665227)) ;
#50414=CARTESIAN_POINT('Ctrl Pts',(179.022503689492,587.574727072608,-47.6964391260437)) ;
#50415=CARTESIAN_POINT('Ctrl Pts',(178.972318281831,587.550580578585,-47.6935484885674)) ;
#50416=CARTESIAN_POINT('Ctrl Pts',(178.879111969972,587.500975565246,-47.6879243501719)) ;
#50417=CARTESIAN_POINT('Ctrl Pts',(178.835918336567,587.475927004888,-47.685207514099)) ;
#50418=CARTESIAN_POINT('Ctrl Pts',(178.739586813696,587.415270144877,-47.678880404289)) ;
#50419=CARTESIAN_POINT('Ctrl Pts',(178.687123423991,587.378710321286,-47.675236820593)) ;
#50420=CARTESIAN_POINT('Ctrl Pts',(178.636459895391,587.339774773179,-47.6715230358871)) ;
#50421=CARTESIAN_POINT('Ctrl Pts',(178.636459939217,587.33977480686,-47.7297342831524)) ;
#50422=CARTESIAN_POINT('Ctrl Pts',(178.685121246926,587.377171621376,-47.7333722715894)) ;
#50423=CARTESIAN_POINT('Ctrl Pts',(178.735429412256,587.412367062688,-47.7369561190645)) ;
#50424=CARTESIAN_POINT('Ctrl Pts',(178.809385083481,587.459317969666,-47.7418993910626)) ;
#50425=CARTESIAN_POINT('Ctrl Pts',(178.831788584265,587.472946435851,-47.743356368714)) ;
#50426=CARTESIAN_POINT('Ctrl Pts',(178.882639345079,587.502561434873,-47.7465626887374)) ;
#50427=CARTESIAN_POINT('Ctrl Pts',(178.91121922827,587.518306956344,-47.7482956410734)) ;
#50428=CARTESIAN_POINT('Ctrl Pts',(179.062994969881,587.597272621547,-47.757204387362)) ;
#50429=CARTESIAN_POINT('Ctrl Pts',(179.191986039724,587.648607440626,-47.7637955950988)) ;
#50430=CARTESIAN_POINT('Ctrl Pts',(179.403531539794,587.708918365324,-47.7744335276501)) ;
#50431=CARTESIAN_POINT('Ctrl Pts',(179.483146674648,587.726576573746,-47.7783973377741)) ;
#50432=CARTESIAN_POINT('Ctrl Pts',(179.627946151611,587.749766461961,-47.7857484251801)) ;
#50433=CARTESIAN_POINT('Ctrl Pts',(179.692744623988,587.757004154329,-47.7890872707027)) ;
#50434=CARTESIAN_POINT('Ctrl Pts',(179.806922777768,587.764284630978,-47.7951226952449)) ;
#50435=CARTESIAN_POINT('Ctrl Pts',(179.856165259636,587.76565034262,-47.7977745711824)) ;
#50436=CARTESIAN_POINT('Ctrl Pts',(179.969551834077,587.764718888585,-47.8040120431308)) ;
#50437=CARTESIAN_POINT('Ctrl Pts',(180.033631541949,587.761188487531,-47.8076345366458)) ;
#50438=CARTESIAN_POINT('Ctrl Pts',(180.244234576702,587.739664676921,-47.8198607373283)) ;
#50439=CARTESIAN_POINT('Ctrl Pts',(180.388978726142,587.70889252268,-47.8288161444471)) ;
#50440=CARTESIAN_POINT('Ctrl Pts',(180.602059547016,587.638972966298,-47.8422324087778)) ;
#50441=CARTESIAN_POINT('Ctrl Pts',(180.673570674285,587.610984552505,-47.8467682387898)) ;
#50442=CARTESIAN_POINT('Ctrl Pts',(180.77191781701,587.565991261117,-47.8529028490711)) ;
#50443=CARTESIAN_POINT('Ctrl Pts',(180.800181215274,587.552268814845,-47.8546528564018)) ;
#50444=CARTESIAN_POINT('Ctrl Pts',(180.857994067106,587.522542170704,-47.8581884581791)) ;
#50445=CARTESIAN_POINT('Ctrl Pts',(180.887487456895,587.506450850997,-47.8599687544073)) ;
#50446=CARTESIAN_POINT('Ctrl Pts',(181.027472061702,587.42556016813,-47.8683679266912)) ;
#50447=CARTESIAN_POINT('Ctrl Pts',(181.132146775073,587.351242068804,-47.8745059408282)) ;
#50448=CARTESIAN_POINT('Ctrl Pts',(181.322303135832,587.187511707329,-47.8866473468647)) ;
#50449=CARTESIAN_POINT('Ctrl Pts',(181.408000507189,587.099191091871,-47.8926264083878)) ;
#50450=CARTESIAN_POINT('Ctrl Pts',(181.518932709314,586.962217579984,-47.9016958987071)) ;
#50451=CARTESIAN_POINT('Ctrl Pts',(181.550936707775,586.91938684467,-47.9045039576313)) ;
#50452=CARTESIAN_POINT('Ctrl Pts',(181.610732168192,586.832490746178,-47.910178771066)) ;
#50453=CARTESIAN_POINT('Ctrl Pts',(181.638590046267,586.788519857356,-47.9130399002851)) ;
#50454=CARTESIAN_POINT('Ctrl Pts',(181.755704513453,586.587139645176,-47.9261227425133)) ;
#50455=CARTESIAN_POINT('Ctrl Pts',(181.825592849092,586.419429188602,-47.9370595229622)) ;
#50456=CARTESIAN_POINT('Ctrl Pts',(181.887379883498,586.189951930345,-47.9512949238449)) ;
#50457=CARTESIAN_POINT('Ctrl Pts',(181.89986481163,586.134529058559,-47.9546712369496)) ;
#50458=CARTESIAN_POINT('Ctrl Pts',(181.917608862202,586.037081332327,-47.9604290658585)) ;
#50459=CARTESIAN_POINT('Ctrl Pts',(181.923895539515,585.995278086389,-47.9628425815576)) ;
#50460=CARTESIAN_POINT('Ctrl Pts',(181.932320421659,585.924463173431,-47.9668031182439)) ;
#50461=CARTESIAN_POINT('Ctrl Pts',(181.935139833815,585.89555156452,-47.9683822080552)) ;
#50462=CARTESIAN_POINT('Ctrl Pts',(181.940953881478,585.819202681555,-47.972459522156)) ;
#50463=CARTESIAN_POINT('Ctrl Pts',(181.942917584158,585.771706060209,-47.974906408834)) ;
#50464=CARTESIAN_POINT('Ctrl Pts',(181.944140632089,585.587138683429,-47.9842104124131)) ;
#50465=CARTESIAN_POINT('Ctrl Pts',(181.931336410573,585.450342006926,-47.9906895499841)) ;
#50466=CARTESIAN_POINT('Ctrl Pts',(181.886883181918,585.223254546101,-48.0019933683402)) ;
#50467=CARTESIAN_POINT('Ctrl Pts',(181.862408409543,585.132042235162,-48.0066859319288)) ;
#50468=CARTESIAN_POINT('Ctrl Pts',(181.815029468638,584.99415895087,-48.0142488882546)) ;
#50469=CARTESIAN_POINT('Ctrl Pts',(181.796479679247,584.946127110689,-48.0169744114881)) ;
#50470=CARTESIAN_POINT('Ctrl Pts',(181.754646973934,584.848846994174,-48.0227102638407)) ;
#50471=CARTESIAN_POINT('Ctrl Pts',(181.731170387928,584.799726827208,-48.0257257385062)) ;
#50472=CARTESIAN_POINT('Ctrl Pts',(181.627255775538,584.602808025621,-48.0383298795153)) ;
#50473=CARTESIAN_POINT('Ctrl Pts',(181.530770202985,584.464241040989,-48.048497541916)) ;
#50474=CARTESIAN_POINT('Ctrl Pts',(181.379537424341,584.295540354759,-48.0620831337559)) ;
#50475=CARTESIAN_POINT('Ctrl Pts',(181.338733810148,584.253750790581,-48.0655596198017)) ;
#50476=CARTESIAN_POINT('Ctrl Pts',(181.264880107449,584.184295057971,-48.0714613126554)) ;
#50477=CARTESIAN_POINT('Ctrl Pts',(181.232636586987,584.15582459596,-48.0739205583258)) ;
#50478=CARTESIAN_POINT('Ctrl Pts',(181.177209693695,584.109897904425,-48.0779225835602)) ;
#50479=CARTESIAN_POINT('Ctrl Pts',(181.154511533064,584.091886053223,-48.0794998337636)) ;
#50480=CARTESIAN_POINT('Ctrl Pts',(181.094518301859,584.046313554621,-48.0835163547645)) ;
#50481=CARTESIAN_POINT('Ctrl Pts',(181.056659362174,584.019525305305,-48.0859079033304)) ;
#50482=CARTESIAN_POINT('Ctrl Pts',(180.903781206245,583.918938415685,-48.0951494693389)) ;
#50483=CARTESIAN_POINT('Ctrl Pts',(180.782425708051,583.855405453882,-48.101611621751)) ;
#50484=CARTESIAN_POINT('Ctrl Pts',(180.5665410488,583.768524288893,-48.1129684175069)) ;
#50485=CARTESIAN_POINT('Ctrl Pts',(180.475029262308,583.738957122749,-48.1177399653916)) ;
#50486=CARTESIAN_POINT('Ctrl Pts',(180.331724867342,583.703519135387,-48.1253929051634)) ;
#50487=CARTESIAN_POINT('Ctrl Pts',(180.281213082619,583.693028287582,-48.1281221150801)) ;
#50488=CARTESIAN_POINT('Ctrl Pts',(180.176939632221,583.675435836514,-48.1338470225872)) ;
#50489=CARTESIAN_POINT('Ctrl Pts',(180.123184838433,583.668539682639,-48.1368470084502)) ;
#50490=CARTESIAN_POINT('Ctrl Pts',(179.904729169015,583.649253826554,-48.149253612751)) ;
#50491=CARTESIAN_POINT('Ctrl Pts',(179.739103961346,583.654616901791,-48.1592159016528)) ;
#50492=CARTESIAN_POINT('Ctrl Pts',(179.489951376294,583.692966635994,-48.1743445615698)) ;
#50493=CARTESIAN_POINT('Ctrl Pts',(179.404882292459,583.711651318651,-48.1795206036668)) ;
#50494=CARTESIAN_POINT('Ctrl Pts',(179.290413414615,583.744532051245,-48.1862917883039)) ;
#50495=CARTESIAN_POINT('Ctrl Pts',(179.259787857356,583.754110862513,-48.1880833580417)) ;
#50496=CARTESIAN_POINT('Ctrl Pts',(179.198265249755,583.774947490261,-48.1916236081324)) ;
#50497=CARTESIAN_POINT('Ctrl Pts',(179.167389063839,583.786237391059,-48.1933700956937)) ;
#50498=CARTESIAN_POINT('Ctrl Pts',(179.009776680321,583.848195386809,-48.2021918055425)) ;
#50499=CARTESIAN_POINT('Ctrl Pts',(178.888034361432,583.91066348513,-48.2087065889619)) ;
#50500=CARTESIAN_POINT('Ctrl Pts',(178.673245011278,584.049451579728,-48.2210947512499)) ;
#50501=CARTESIAN_POINT('Ctrl Pts',(178.5789406374,584.122740061617,-48.2269230229882)) ;
#50502=CARTESIAN_POINT('Ctrl Pts',(178.452847466274,584.239646283619,-48.235795173972)) ;
#50503=CARTESIAN_POINT('Ctrl Pts',(178.415564827687,584.27698231178,-48.238573663469)) ;
#50504=CARTESIAN_POINT('Ctrl Pts',(178.343961353214,584.35443322779,-48.2442612720391)) ;
#50505=CARTESIAN_POINT('Ctrl Pts',(178.309667660239,584.39451832682,-48.2471682239792)) ;
#50506=CARTESIAN_POINT('Ctrl Pts',(178.175010798644,584.564763085197,-48.2593901721941)) ;
#50507=CARTESIAN_POINT('Ctrl Pts',(178.08890997158,584.705397593426,-48.2692667916853)) ;
#50508=CARTESIAN_POINT('Ctrl Pts',(177.993744151752,584.913122014472,-48.2829923187101)) ;
#50509=CARTESIAN_POINT('Ctrl Pts',(177.969751377576,584.972717998752,-48.2868315469812)) ;
#50510=CARTESIAN_POINT('Ctrl Pts',(177.93356250256,585.076382845395,-48.2932464649048)) ;
#50511=CARTESIAN_POINT('Ctrl Pts',(177.919972544042,585.119915217059,-48.2958636277839)) ;
#50512=CARTESIAN_POINT('Ctrl Pts',(177.900136405436,585.191781470052,-48.3000202988913)) ;
#50513=CARTESIAN_POINT('Ctrl Pts',(177.893022713931,585.219854914262,-48.3016021401449)) ;
#50514=CARTESIAN_POINT('Ctrl Pts',(177.876673238317,585.290628304369,-48.3054861972944)) ;
#50515=CARTESIAN_POINT('Ctrl Pts',(177.868201324395,585.333487955035,-48.3077492958369)) ;
#50516=CARTESIAN_POINT('Ctrl Pts',(177.839106260069,585.510111076727,-48.3168306450971)) ;
#50517=CARTESIAN_POINT('Ctrl Pts',(177.830353564614,585.645489593599,-48.3232400091894)) ;
#50518=CARTESIAN_POINT('Ctrl Pts',(177.838418384486,585.881447432622,-48.3347357433026)) ;
#50519=CARTESIAN_POINT('Ctrl Pts',(177.849261112119,585.981744041669,-48.3397224335615)) ;
#50520=CARTESIAN_POINT('Ctrl Pts',(177.876765189013,586.131875156197,-48.3476239015105)) ;
#50521=CARTESIAN_POINT('Ctrl Pts',(177.888045446498,586.182540388175,-48.3503660802006)) ;
#50522=CARTESIAN_POINT('Ctrl Pts',(177.914883102183,586.284682946268,-48.3560766796963)) ;
#50523=CARTESIAN_POINT('Ctrl Pts',(177.930567397288,586.336084872031,-48.359047485209)) ;
#50524=CARTESIAN_POINT('Ctrl Pts',(178.004139143522,586.547176825693,-48.371675885257)) ;
#50525=CARTESIAN_POINT('Ctrl Pts',(178.079691484335,586.699975624319,-48.3819321091802)) ;
#50526=CARTESIAN_POINT('Ctrl Pts',(178.219609065619,586.912159829085,-48.397173639217)) ;
#50527=CARTESIAN_POINT('Ctrl Pts',(178.270364970187,586.979687263092,-48.4021860179028)) ;
#50528=CARTESIAN_POINT('Ctrl Pts',(178.345864689751,587.068213582013,-48.4087972105741)) ;
#50529=CARTESIAN_POINT('Ctrl Pts',(178.367161054818,587.09203621,-48.4105802503613)) ;
#50530=CARTESIAN_POINT('Ctrl Pts',(178.411603574376,587.139475723884,-48.4141213908943)) ;
#50531=CARTESIAN_POINT('Ctrl Pts',(178.434781280395,587.163049892017,-48.4158765831591)) ;
#50532=CARTESIAN_POINT('Ctrl Pts',(178.51484535328,587.240645969364,-48.4216807330674)) ;
#50533=CARTESIAN_POINT('Ctrl Pts',(178.574255931544,587.291970259067,-48.4255669620015)) ;
#50534=CARTESIAN_POINT('Ctrl Pts',(178.636459914542,587.339774787898,-48.4293959864656)) ;
#50535=CARTESIAN_POINT('Origin',(179.888527625416,585.710565160536,-51.0680854522974)) ;
#50536=CARTESIAN_POINT('',(178.63687932657,587.339321169053,-49.1271827457828)) ;
#50537=CARTESIAN_POINT('',(178.636459914524,587.339774787883,-49.0681958067691)) ;
#50538=CARTESIAN_POINT('',(178.636459914529,587.339774787887,-51.0680854522974)) ;
#50539=CARTESIAN_POINT('',(181.943277589855,585.710182877802,-49.3762357656828)) ;
#50540=CARTESIAN_POINT('Ctrl Pts',(181.942731046524,585.710143815257,-49.375289272883)) ;
#50541=CARTESIAN_POINT('Ctrl Pts',(181.942609902982,585.781072616081,-49.3712166166913)) ;
#50542=CARTESIAN_POINT('Ctrl Pts',(181.938842933789,585.852042270409,-49.3671991813958)) ;
#50543=CARTESIAN_POINT('Ctrl Pts',(181.931456861355,585.922655946303,-49.3632663178078)) ;
#50544=CARTESIAN_POINT('Ctrl Pts',(181.924072660175,585.993251732304,-49.3593344506064)) ;
#50545=CARTESIAN_POINT('Ctrl Pts',(181.913071204659,586.063491698852,-49.3554871423331)) ;
#50546=CARTESIAN_POINT('Ctrl Pts',(181.898513657117,586.132983525398,-49.3517291276852)) ;
#50547=CARTESIAN_POINT('Ctrl Pts',(181.88395481418,586.202481535636,-49.3479707786323)) ;
#50548=CARTESIAN_POINT('Ctrl Pts',(181.865839152381,586.271231202506,-49.3443016663953)) ;
#50549=CARTESIAN_POINT('Ctrl Pts',(181.844262927951,586.338844996212,-49.3407022466588)) ;
#50550=CARTESIAN_POINT('Ctrl Pts',(181.822661713033,586.406537103051,-49.3370986579233)) ;
#50551=CARTESIAN_POINT('Ctrl Pts',(181.797591708343,586.473090572644,-49.333564737381)) ;
#50552=CARTESIAN_POINT('Ctrl Pts',(181.769186915986,586.538122925371,-49.3300584437495)) ;
#50553=CARTESIAN_POINT('Ctrl Pts',(181.740764472904,586.603195689168,-49.3265499713089)) ;
#50554=CARTESIAN_POINT('Ctrl Pts',(181.709002781512,586.666745209728,-49.3230688143823)) ;
#50555=CARTESIAN_POINT('Ctrl Pts',(181.674077437369,586.728397382294,-49.3195543533391)) ;
#50556=CARTESIAN_POINT('Ctrl Pts',(181.641178847481,586.786471814792,-49.3162438401467)) ;
#50557=CARTESIAN_POINT('Ctrl Pts',(181.605472728773,586.842862902337,-49.3129032840571)) ;
#50558=CARTESIAN_POINT('Ctrl Pts',(181.567145026093,586.897267996673,-49.3094721752712)) ;
#50559=CARTESIAN_POINT('Ctrl Pts',(181.564706940191,586.900728790934,-49.3092539170043)) ;
#50560=CARTESIAN_POINT('Ctrl Pts',(181.562258245026,586.904181566495,-49.309035292322)) ;
#50561=CARTESIAN_POINT('Ctrl Pts',(181.5597989878,586.907626252577,-49.308816285649)) ;
#50562=CARTESIAN_POINT('Ctrl Pts',(181.533601879691,586.944320589691,-49.3064833285961)) ;
#50563=CARTESIAN_POINT('Ctrl Pts',(181.506207383144,586.980095008409,-49.3041067928128)) ;
#50564=CARTESIAN_POINT('Ctrl Pts',(181.477684382118,587.014860414755,-49.3016672162806)) ;
#50565=CARTESIAN_POINT('Ctrl Pts',(181.477662093227,587.014887581684,-49.3016653099084)) ;
#50566=CARTESIAN_POINT('Ctrl Pts',(181.477639803647,587.014914747998,-49.3016634034977)) ;
#50567=CARTESIAN_POINT('Ctrl Pts',(181.477617513378,587.014941913696,-49.3016614970486)) ;
#50568=CARTESIAN_POINT('Ctrl Pts',(181.436792415083,587.064696463765,-49.298169795156)) ;
#50569=CARTESIAN_POINT('Ctrl Pts',(181.393498463665,587.112564995586,-49.2945396579515)) ;
#50570=CARTESIAN_POINT('Ctrl Pts',(181.347956768597,587.15831772393,-49.2908361813299)) ;
#50571=CARTESIAN_POINT('Ctrl Pts',(181.343340057968,587.162955827692,-49.290460747788)) ;
#50572=CARTESIAN_POINT('Ctrl Pts',(181.338700291656,587.16757217983,-49.2900845605706)) ;
#50573=CARTESIAN_POINT('Ctrl Pts',(181.33403772939,587.17216653593,-49.2897076874925)) ;
#50574=CARTESIAN_POINT('Ctrl Pts',(181.283458903455,587.222005470876,-49.2856194208424)) ;
#50575=CARTESIAN_POINT('Ctrl Pts',(181.230191784817,587.269257599862,-49.2814510605544)) ;
#50576=CARTESIAN_POINT('Ctrl Pts',(181.174555896109,587.313659051509,-49.2772769797148)) ;
#50577=CARTESIAN_POINT('Ctrl Pts',(181.118988717447,587.358005667584,-49.2731080538443)) ;
#50578=CARTESIAN_POINT('Ctrl Pts',(181.061058803437,587.399508975766,-49.2689337751207)) ;
#50579=CARTESIAN_POINT('Ctrl Pts',(181.00110188632,587.437942358132,-49.2648088811621)) ;
#50580=CARTESIAN_POINT('Ctrl Pts',(180.941185011684,587.476350072602,-49.2606867420313)) ;
#50581=CARTESIAN_POINT('Ctrl Pts',(180.879243905101,587.511692123099,-49.2566140905518)) ;
#50582=CARTESIAN_POINT('Ctrl Pts',(180.815629223576,587.543774893854,-49.2526223602738)) ;
#50583=CARTESIAN_POINT('Ctrl Pts',(180.752035650566,587.575847018959,-49.2486319545248)) ;
#50584=CARTESIAN_POINT('Ctrl Pts',(180.686769631124,587.604662042031,-49.2447224565592)) ;
#50585=CARTESIAN_POINT('Ctrl Pts',(180.620196491689,587.63005777694,-49.2409005518772)) ;
#50586=CARTESIAN_POINT('Ctrl Pts',(180.553623072081,587.655453618726,-49.2370786311107)) ;
#50587=CARTESIAN_POINT('Ctrl Pts',(180.485742520518,587.677430034423,-49.2333442395844)) ;
#50588=CARTESIAN_POINT('Ctrl Pts',(180.416935074601,587.695856798957,-49.2296795293261)) ;
#50589=CARTESIAN_POINT('Ctrl Pts',(180.348058708124,587.714302020548,-49.226011148333)) ;
#50590=CARTESIAN_POINT('Ctrl Pts',(180.278253579484,587.729190236431,-49.2224124098555)) ;
#50591=CARTESIAN_POINT('Ctrl Pts',(180.207916107238,587.740425467912,-49.2188426223026)) ;
#50592=CARTESIAN_POINT('Ctrl Pts',(180.137540745288,587.751666751639,-49.2152709117605)) ;
#50593=CARTESIAN_POINT('Ctrl Pts',(180.06663248392,587.759250723212,-49.2117278455962)) ;
#50594=CARTESIAN_POINT('Ctrl Pts',(179.995603422909,587.763120605311,-49.2081536905138)) ;
#50595=CARTESIAN_POINT('Ctrl Pts',(179.92834605237,587.766784994091,-49.204769325448)) ;
#50596=CARTESIAN_POINT('Ctrl Pts',(179.860980032854,587.767118982164,-49.2013565946411)) ;
#50597=CARTESIAN_POINT('Ctrl Pts',(179.793868461632,587.764113188371,-49.1978542829438)) ;
#50598=CARTESIAN_POINT('Ctrl Pts',(179.789983017362,587.76393916705,-49.197651515572)) ;
#50599=CARTESIAN_POINT('Ctrl Pts',(179.78609841312,587.763753958018,-49.1974484479372)) ;
#50600=CARTESIAN_POINT('Ctrl Pts',(179.782214714566,587.763557561845,-49.19724506816)) ;
#50601=CARTESIAN_POINT('Ctrl Pts',(179.739246410607,587.761384681962,-49.1949949233658)) ;
#50602=CARTESIAN_POINT('Ctrl Pts',(179.696391016001,587.757842438412,-49.1927063515351)) ;
#50603=CARTESIAN_POINT('Ctrl Pts',(179.653745543434,587.752938395067,-49.1903625908485)) ;
#50604=CARTESIAN_POINT('Ctrl Pts',(179.653711814989,587.752934516443,-49.1903607371604)) ;
#50605=CARTESIAN_POINT('Ctrl Pts',(179.653678086674,587.752930636967,-49.1903588834378)) ;
#50606=CARTESIAN_POINT('Ctrl Pts',(179.65364435849,587.75292675664,-49.1903570296806)) ;
#50607=CARTESIAN_POINT('Ctrl Pts',(179.589350160997,587.745529900698,-49.1868233135333)) ;
#50608=CARTESIAN_POINT('Ctrl Pts',(179.525312509616,587.735005549323,-49.1831554356994)) ;
#50609=CARTESIAN_POINT('Ctrl Pts',(179.46184773535,587.721416836011,-49.1794183432615)) ;
#50610=CARTESIAN_POINT('Ctrl Pts',(179.455646154714,587.72008898915,-49.1790531661949)) ;
#50611=CARTESIAN_POINT('Ctrl Pts',(179.449450072789,587.718731911477,-49.1786873282263)) ;
#50612=CARTESIAN_POINT('Ctrl Pts',(179.443259802766,587.717345681468,-49.1783208899553)) ;
#50613=CARTESIAN_POINT('Ctrl Pts',(179.374193897246,587.701879275243,-49.1742324752477)) ;
#50614=CARTESIAN_POINT('Ctrl Pts',(179.305847650325,587.682780044733,-49.1700700719711)) ;
#50615=CARTESIAN_POINT('Ctrl Pts',(179.238608498183,587.660172786892,-49.1659052769008)) ;
#50616=CARTESIAN_POINT('Ctrl Pts',(179.235036122816,587.658971676996,-49.165684003865)) ;
#50617=CARTESIAN_POINT('Ctrl Pts',(179.231466882203,587.657760672292,-49.1654627240778)) ;
#50618=CARTESIAN_POINT('Ctrl Pts',(179.227900837645,587.656539794077,-49.1652414482766)) ;
#50619=CARTESIAN_POINT('Ctrl Pts',(179.160499471941,587.633464126422,-49.1610591418145)) ;
#50620=CARTESIAN_POINT('Ctrl Pts',(179.094235691661,587.606858873681,-49.156878466474)) ;
#50621=CARTESIAN_POINT('Ctrl Pts',(179.029481540879,587.576886091707,-49.1527518854787)) ;
#50622=CARTESIAN_POINT('Ctrl Pts',(178.964770398448,587.546933217028,-49.1486280452721)) ;
#50623=CARTESIAN_POINT('Ctrl Pts',(178.901566786388,587.513617417541,-49.1445583855618)) ;
#50624=CARTESIAN_POINT('Ctrl Pts',(178.840223204897,587.477131031072,-49.1405719754824)) ;
#50625=CARTESIAN_POINT('Ctrl Pts',(178.77889638879,587.44065461644,-49.1365866549009)) ;
#50626=CARTESIAN_POINT('Ctrl Pts',(178.719428589935,587.401009363747,-49.1326845707494)) ;
#50627=CARTESIAN_POINT('Ctrl Pts',(178.662153901579,587.358416989177,-49.1288700914329)) ;
#50628=CARTESIAN_POINT('Ctrl Pts',(178.653680728366,587.35211590614,-49.1283057803054)) ;
#50629=CARTESIAN_POINT('Ctrl Pts',(178.645255520909,587.345750375093,-49.1277433423199)) ;
#50630=CARTESIAN_POINT('Ctrl Pts',(178.63687932657,587.339321169054,-49.1271827457828)) ;
#50631=CARTESIAN_POINT('',(180.418697842604,583.725390834864,-49.5221601717598)) ;
#50632=CARTESIAN_POINT('Ctrl Pts',(180.418697842604,583.725390834864,-49.5221601717598)) ;
#50633=CARTESIAN_POINT('Ctrl Pts',(180.488833687662,583.744121651461,-49.5182241312826)) ;
#50634=CARTESIAN_POINT('Ctrl Pts',(180.558043092019,583.766591466879,-49.5142880908053)) ;
#50635=CARTESIAN_POINT('Ctrl Pts',(180.625912157186,583.792685702696,-49.5103520503281)) ;
#50636=CARTESIAN_POINT('Ctrl Pts',(180.693726478774,583.818758890751,-49.5064191846838)) ;
#50637=CARTESIAN_POINT('Ctrl Pts',(180.760202181966,583.848450521621,-49.5024863190395)) ;
#50638=CARTESIAN_POINT('Ctrl Pts',(180.824941915912,583.881596642749,-49.4985534533952)) ;
#50639=CARTESIAN_POINT('Ctrl Pts',(180.889661927391,583.914732666164,-49.4946217858685)) ;
#50640=CARTESIAN_POINT('Ctrl Pts',(180.952646607951,583.951320884749,-49.4906901183417)) ;
#50641=CARTESIAN_POINT('Ctrl Pts',(181.01352096904,583.991150277705,-49.486758450815)) ;
#50642=CARTESIAN_POINT('Ctrl Pts',(181.074388214353,584.030975014891,-49.482827242872)) ;
#50643=CARTESIAN_POINT('Ctrl Pts',(181.133145244721,584.074039921525,-49.478896034929)) ;
#50644=CARTESIAN_POINT('Ctrl Pts',(181.189445268872,584.120090122239,-49.474964826986)) ;
#50645=CARTESIAN_POINT('Ctrl Pts',(181.245754646727,584.166147973749,-49.4710329659108)) ;
#50646=CARTESIAN_POINT('Ctrl Pts',(181.299605850614,584.215191813014,-49.4671011048356)) ;
#50647=CARTESIAN_POINT('Ctrl Pts',(181.350685554016,584.266926786727,-49.4631692437604)) ;
#50648=CARTESIAN_POINT('Ctrl Pts',(181.401788202959,584.318685000336,-49.4592356164518)) ;
#50649=CARTESIAN_POINT('Ctrl Pts',(181.450116553871,584.373136422868,-49.4553019891431)) ;
#50650=CARTESIAN_POINT('Ctrl Pts',(181.495395471567,584.429950742568,-49.4513683618344)) ;
#50651=CARTESIAN_POINT('Ctrl Pts',(181.540741306735,584.48684902785,-49.4474289210388)) ;
#50652=CARTESIAN_POINT('Ctrl Pts',(181.583028425668,584.546116819582,-49.4434894802433)) ;
#50653=CARTESIAN_POINT('Ctrl Pts',(181.622023487452,584.60739261791,-49.4395500394477)) ;
#50654=CARTESIAN_POINT('Ctrl Pts',(181.661050939679,584.668719313714,-49.4356073264369)) ;
#50655=CARTESIAN_POINT('Ctrl Pts',(181.69678066254,584.732056936852,-49.4316646134261)) ;
#50656=CARTESIAN_POINT('Ctrl Pts',(181.729025270704,584.797019332353,-49.4277219004154)) ;
#50657=CARTESIAN_POINT('Ctrl Pts',(181.761331269842,584.862105410695,-49.4237716808165)) ;
#50658=CARTESIAN_POINT('Ctrl Pts',(181.790138722435,584.928822015519,-49.4198214612176)) ;
#50659=CARTESIAN_POINT('Ctrl Pts',(181.815308509274,584.996763375656,-49.4158712416187)) ;
#50660=CARTESIAN_POINT('Ctrl Pts',(181.825786450384,585.025046712936,-49.4142268030466)) ;
#50661=CARTESIAN_POINT('Ctrl Pts',(181.835634593048,585.053542127974,-49.4125823644746)) ;
#50662=CARTESIAN_POINT('Ctrl Pts',(181.844845492613,585.082219742008,-49.4109379259025)) ;
#50663=CARTESIAN_POINT('Ctrl Pts',(181.870333237588,585.161574392204,-49.4063875526567)) ;
#50664=CARTESIAN_POINT('Ctrl Pts',(181.891016257104,585.242567282731,-49.4018371794109)) ;
#50665=CARTESIAN_POINT('Ctrl Pts',(181.906713128642,585.324657351507,-49.3972868061651)) ;
#50666=CARTESIAN_POINT('Ctrl Pts',(181.922242415703,585.40587100225,-49.3927850140597)) ;
#50667=CARTESIAN_POINT('Ctrl Pts',(181.932891369071,585.488158412433,-49.3882832219544)) ;
#50668=CARTESIAN_POINT('Ctrl Pts',(181.938530559059,585.570974564301,-49.3837814298491)) ;
#50669=CARTESIAN_POINT('Ctrl Pts',(181.941681262365,585.617245238656,-49.3812662084604)) ;
#50670=CARTESIAN_POINT('Ctrl Pts',(181.943268938184,585.663680597079,-49.3787509870716)) ;
#50671=CARTESIAN_POINT('Ctrl Pts',(181.943277589855,585.710182877802,-49.3762357656828)) ;
#50672=CARTESIAN_POINT('',(179.355546343215,583.723963875141,-49.5209457596381)) ;
#50673=CARTESIAN_POINT('Origin',(179.888527625416,585.710565160536,-49.5221601717598)) ;
#50674=CARTESIAN_POINT('Ctrl Pts',(179.356176202651,583.725974642273,-49.5197218953676)) ;
#50675=CARTESIAN_POINT('Ctrl Pts',(179.386889376523,583.717736065268,-49.5180018393397)) ;
#50676=CARTESIAN_POINT('Ctrl Pts',(179.417791541479,583.710211061965,-49.5163222483587)) ;
#50677=CARTESIAN_POINT('Ctrl Pts',(179.62291895486,583.665277731807,-49.5054338937319)) ;
#50678=CARTESIAN_POINT('Ctrl Pts',(179.8012184922,583.649948421268,-49.4971434324973)) ;
#50679=CARTESIAN_POINT('Ctrl Pts',(180.046299752696,583.660783124538,-49.485062778235)) ;
#50680=CARTESIAN_POINT('Ctrl Pts',(180.113133550294,583.667026643641,-49.4817057318923)) ;
#50681=CARTESIAN_POINT('Ctrl Pts',(180.232949061191,583.684168734103,-49.4754789283973)) ;
#50682=CARTESIAN_POINT('Ctrl Pts',(180.286033818234,583.693910325479,-49.4726452771753)) ;
#50683=CARTESIAN_POINT('Ctrl Pts',(180.38961266037,583.717166744821,-49.466936066763)) ;
#50684=CARTESIAN_POINT('Ctrl Pts',(180.44009631471,583.730541237049,-49.4640669709128)) ;
#50685=CARTESIAN_POINT('Ctrl Pts',(180.658536214026,583.797414324731,-49.4512467161314)) ;
#50686=CARTESIAN_POINT('Ctrl Pts',(180.819699315335,583.87046782969,-49.4406323481091)) ;
#50687=CARTESIAN_POINT('Ctrl Pts',(181.039578895036,584.00649269093,-49.4251737513292)) ;
#50688=CARTESIAN_POINT('Ctrl Pts',(181.106963343656,584.054002869783,-49.4202967402071)) ;
#50689=CARTESIAN_POINT('Ctrl Pts',(181.196194163741,584.125314438653,-49.4138177849933)) ;
#50690=CARTESIAN_POINT('Ctrl Pts',(181.220606829301,584.145772222574,-49.4120432686528)) ;
#50691=CARTESIAN_POINT('Ctrl Pts',(181.269515556757,584.188732282953,-49.4085018593836)) ;
#50692=CARTESIAN_POINT('Ctrl Pts',(181.293960615279,584.211278207407,-49.4067387469068)) ;
#50693=CARTESIAN_POINT('Ctrl Pts',(181.413096631273,584.326634341954,-49.398117883182)) ;
#50694=CARTESIAN_POINT('Ctrl Pts',(181.499205055676,584.427872260819,-49.3917808198691)) ;
#50695=CARTESIAN_POINT('Ctrl Pts',(181.622908773339,584.605593193042,-49.3813051619974)) ;
#50696=CARTESIAN_POINT('Ctrl Pts',(181.666587291408,584.677345034425,-49.3772266321849)) ;
#50697=CARTESIAN_POINT('Ctrl Pts',(181.736732034291,584.810263369691,-49.3696979435945)) ;
#50698=CARTESIAN_POINT('Ctrl Pts',(181.764844856385,584.870425085859,-49.3663001305553)) ;
#50699=CARTESIAN_POINT('Ctrl Pts',(181.808774185936,584.977690174157,-49.3601887408044)) ;
#50700=CARTESIAN_POINT('Ctrl Pts',(181.825886519072,585.024203356173,-49.3575224584785)) ;
#50701=CARTESIAN_POINT('Ctrl Pts',(181.861229729117,585.13216457032,-49.3512781347795)) ;
#50702=CARTESIAN_POINT('Ctrl Pts',(181.878299808622,585.193935477701,-49.3476646133698)) ;
#50703=CARTESIAN_POINT('Ctrl Pts',(181.924877811513,585.399452434824,-49.3355110738389)) ;
#50704=CARTESIAN_POINT('Ctrl Pts',(181.941885161974,585.545557198841,-49.3266292723503)) ;
#50705=CARTESIAN_POINT('Ctrl Pts',(181.94387725099,585.768487613464,-49.3133195289235)) ;
#50706=CARTESIAN_POINT('Ctrl Pts',(181.940310231736,585.844755901183,-49.308818262318)) ;
#50707=CARTESIAN_POINT('Ctrl Pts',(181.929291183026,585.951961391816,-49.3027124523943)) ;
#50708=CARTESIAN_POINT('Ctrl Pts',(181.925354210697,585.983192785691,-49.3009608130156)) ;
#50709=CARTESIAN_POINT('Ctrl Pts',(181.915760062096,586.047378507676,-49.2974340859969)) ;
#50710=CARTESIAN_POINT('Ctrl Pts',(181.91001315652,586.080309818826,-49.2956641350769)) ;
#50711=CARTESIAN_POINT('Ctrl Pts',(181.881733465697,586.221871392507,-49.2881706885986)) ;
#50712=CARTESIAN_POINT('Ctrl Pts',(181.851225742185,586.328727459923,-49.2828025136458)) ;
#50713=CARTESIAN_POINT('Ctrl Pts',(181.765035255342,586.558361766762,-49.2709509441333)) ;
#50714=CARTESIAN_POINT('Ctrl Pts',(181.705618529938,586.679181361807,-49.2644842935094)) ;
#50715=CARTESIAN_POINT('Ctrl Pts',(181.606007583798,586.839836828763,-49.2548131821556)) ;
#50716=CARTESIAN_POINT('Ctrl Pts',(181.575327955583,586.885169698002,-49.2519542820075)) ;
#50717=CARTESIAN_POINT('Ctrl Pts',(181.513046335847,586.969718204178,-49.2463318399926)) ;
#50718=CARTESIAN_POINT('Ctrl Pts',(181.48174035064,587.009102801363,-49.2435812871606)) ;
#50719=CARTESIAN_POINT('Ctrl Pts',(181.39353869084,587.112069056182,-49.2360100209409)) ;
#50720=CARTESIAN_POINT('Ctrl Pts',(181.334081765618,587.173316644171,-49.231084553678)) ;
#50721=CARTESIAN_POINT('Ctrl Pts',(181.163438823021,587.328507198668,-49.2174600850716)) ;
#50722=CARTESIAN_POINT('Ctrl Pts',(181.045809206581,587.414628392046,-49.2085624441057)) ;
#50723=CARTESIAN_POINT('Ctrl Pts',(180.876825266669,587.512721294467,-49.1970823189271)) ;
#50724=CARTESIAN_POINT('Ctrl Pts',(180.832664925807,587.536244346927,-49.1941935835968)) ;
#50725=CARTESIAN_POINT('Ctrl Pts',(180.761658948036,587.570800943084,-49.1897713126811)) ;
#50726=CARTESIAN_POINT('Ctrl Pts',(180.735365521296,587.582916992102,-49.1881814058169)) ;
#50727=CARTESIAN_POINT('Ctrl Pts',(180.672443125917,587.610314680613,-49.1844939719287)) ;
#50728=CARTESIAN_POINT('Ctrl Pts',(180.635612223257,587.625098206874,-49.1824234557031)) ;
#50729=CARTESIAN_POINT('Ctrl Pts',(180.494983306995,587.676868124178,-49.1747640503639)) ;
#50730=CARTESIAN_POINT('Ctrl Pts',(180.388690515493,587.706555339862,-49.1694648879953)) ;
#50731=CARTESIAN_POINT('Ctrl Pts',(180.154806656935,587.75200939133,-49.1579392175482)) ;
#50732=CARTESIAN_POINT('Ctrl Pts',(180.027088591908,587.764633356966,-49.1517160110635)) ;
#50733=CARTESIAN_POINT('Ctrl Pts',(179.846249286691,587.765558270212,-49.1423985175278)) ;
#50734=CARTESIAN_POINT('Ctrl Pts',(179.793474814603,587.763793941935,-49.1396220272722)) ;
#50735=CARTESIAN_POINT('Ctrl Pts',(179.689026453531,587.756266594903,-49.1339834551273)) ;
#50736=CARTESIAN_POINT('Ctrl Pts',(179.637387179636,587.750570762241,-49.1311255514424)) ;
#50737=CARTESIAN_POINT('Ctrl Pts',(179.480864991807,587.72727330979,-49.1222322948421)) ;
#50738=CARTESIAN_POINT('Ctrl Pts',(179.377094388892,587.703485526091,-49.1160073953665)) ;
#50739=CARTESIAN_POINT('Ctrl Pts',(179.133131826722,587.627246389328,-49.1007412704924)) ;
#50740=CARTESIAN_POINT('Ctrl Pts',(178.995899259555,587.567311496861,-49.0916085268589)) ;
#50741=CARTESIAN_POINT('Ctrl Pts',(178.837263816686,587.476341986995,-49.0811645232351)) ;
#50742=CARTESIAN_POINT('Ctrl Pts',(178.80856788964,587.458938879881,-49.0792820225989)) ;
#50743=CARTESIAN_POINT('Ctrl Pts',(178.758045081827,587.42657967757,-49.0759979476098)) ;
#50744=CARTESIAN_POINT('Ctrl Pts',(178.736057726286,587.411891056373,-49.0745802295068)) ;
#50745=CARTESIAN_POINT('Ctrl Pts',(178.687948631364,587.378391106045,-49.0714902426275)) ;
#50746=CARTESIAN_POINT('Ctrl Pts',(178.661980295812,587.359387515948,-49.0698303506149)) ;
#50747=CARTESIAN_POINT('Ctrl Pts',(178.636459914524,587.339774787883,-49.0681958067691)) ;
#50748=CARTESIAN_POINT('Origin',(29.8885276254155,585.710565160562,-51.0680854522906)) ;
#50749=CARTESIAN_POINT('',(27.873599051246,585.307997894761,-47.6045419700025)) ;
#50750=CARTESIAN_POINT('',(27.8735991218939,585.307997541154,-47.5475669749031)) ;
#50751=CARTESIAN_POINT('',(27.8735990520584,585.307997890694,-51.0680854522905)) ;
#50752=CARTESIAN_POINT('',(28.0059001157518,584.887332980459,-47.5221601717529)) ;
#50753=CARTESIAN_POINT('Ctrl Pts',(27.8735991218939,585.307997541154,-47.5475669749032)) ;
#50754=CARTESIAN_POINT('Ctrl Pts',(27.895951833801,585.196117911047,-47.5408462881297)) ;
#50755=CARTESIAN_POINT('Ctrl Pts',(27.9276066114201,585.086179402263,-47.5340931280632)) ;
#50756=CARTESIAN_POINT('Ctrl Pts',(27.9800846809023,584.948370365598,-47.525792691713)) ;
#50757=CARTESIAN_POINT('Ctrl Pts',(27.9926238383014,584.917694141937,-47.5239568576251)) ;
#50758=CARTESIAN_POINT('Ctrl Pts',(28.0059001157519,584.887332980459,-47.522160171753)) ;
#50759=CARTESIAN_POINT('',(28.665910763353,584.056452215556,-47.5234195439953)) ;
#50760=CARTESIAN_POINT('Origin',(29.8885276254157,585.710565160562,-47.522160171753)) ;
#50761=CARTESIAN_POINT('Ctrl Pts',(28.6669780822516,584.058350199942,-47.5246789162374)) ;
#50762=CARTESIAN_POINT('Ctrl Pts',(28.6536409221051,584.068210903466,-47.5255745090143)) ;
#50763=CARTESIAN_POINT('Ctrl Pts',(28.6404231746705,584.078233088099,-47.5264591946414)) ;
#50764=CARTESIAN_POINT('Ctrl Pts',(28.6099181024573,584.101950363772,-47.5284978961042)) ;
#50765=CARTESIAN_POINT('Ctrl Pts',(28.5927268286653,584.115766037774,-47.5296444808809)) ;
#50766=CARTESIAN_POINT('Ctrl Pts',(28.4803476990676,584.209096065911,-47.5371487358809)) ;
#50767=CARTESIAN_POINT('Ctrl Pts',(28.3922965013326,584.29681904309,-47.5430847582806)) ;
#50768=CARTESIAN_POINT('Ctrl Pts',(28.23723308194,584.482131450054,-47.5548023003805)) ;
#50769=CARTESIAN_POINT('Ctrl Pts',(28.1696609137121,584.578612473591,-47.5605572957726)) ;
#50770=CARTESIAN_POINT('Ctrl Pts',(28.0841276347631,584.726212641845,-47.569358114201)) ;
#50771=CARTESIAN_POINT('Ctrl Pts',(28.0593291575392,584.773099697532,-47.5721505613178)) ;
#50772=CARTESIAN_POINT('Ctrl Pts',(28.0134598379404,584.868592012861,-47.577861074877)) ;
#50773=CARTESIAN_POINT('Ctrl Pts',(27.9923997258961,584.917157164115,-47.5807767116811)) ;
#50774=CARTESIAN_POINT('Ctrl Pts',(27.9332548385845,585.069396801963,-47.5899668624736)) ;
#50775=CARTESIAN_POINT('Ctrl Pts',(27.9016364340812,585.175358181933,-47.5964448569719)) ;
#50776=CARTESIAN_POINT('Ctrl Pts',(27.8769385539296,585.291545532497,-47.6035380539106)) ;
#50777=CARTESIAN_POINT('Ctrl Pts',(27.8752435130242,585.299767039094,-47.6040398358064)) ;
#50778=CARTESIAN_POINT('Ctrl Pts',(27.8735990504334,585.307997898828,-47.6045419700025)) ;
#50779=CARTESIAN_POINT('Origin',(29.8885276254155,585.710565160562,-51.0680854522906)) ;
#50780=CARTESIAN_POINT('',(27.873599051992,585.307997891027,-48.3063633758768)) ;
#50781=CARTESIAN_POINT('',(27.8735990526509,585.307997887729,-48.2478302996211)) ;
#50782=CARTESIAN_POINT('',(27.8735990520584,585.307997890694,-51.0680854522905)) ;
#50783=CARTESIAN_POINT('',(31.94327712373,585.709998440692,-47.9195214922471)) ;
#50784=CARTESIAN_POINT('Ctrl Pts',(27.8735990532433,585.307997884764,-48.2478302996211)) ;
#50785=CARTESIAN_POINT('Ctrl Pts',(27.8791763621533,585.280082354232,-48.2463036433711)) ;
#50786=CARTESIAN_POINT('Ctrl Pts',(27.8853334487669,585.252284467362,-48.244758529309)) ;
#50787=CARTESIAN_POINT('Ctrl Pts',(27.9070920087431,585.16289103314,-48.2397045223047)) ;
#50788=CARTESIAN_POINT('Ctrl Pts',(27.9249711401828,585.101895516817,-48.2361228016622)) ;
#50789=CARTESIAN_POINT('Ctrl Pts',(27.9708782613911,584.968521068649,-48.2279904734401)) ;
#50790=CARTESIAN_POINT('Ctrl Pts',(28.0002381666779,584.896704121209,-48.223405743598)) ;
#50791=CARTESIAN_POINT('Ctrl Pts',(28.0943565480803,584.699175320679,-48.2103129966963)) ;
#50792=CARTESIAN_POINT('Ctrl Pts',(28.16812458387,584.578233238202,-48.2016933275169)) ;
#50793=CARTESIAN_POINT('Ctrl Pts',(28.2746238613887,584.438361233323,-48.1916354411103)) ;
#50794=CARTESIAN_POINT('Ctrl Pts',(28.2962166765566,584.411436855179,-48.1896964566119)) ;
#50795=CARTESIAN_POINT('Ctrl Pts',(28.3386926405478,584.361124179889,-48.1860883893746)) ;
#50796=CARTESIAN_POINT('Ctrl Pts',(28.3594518786549,584.337646045659,-48.1844129498431)) ;
#50797=CARTESIAN_POINT('Ctrl Pts',(28.4307882733337,584.260592521698,-48.1789081355011)) ;
#50798=CARTESIAN_POINT('Ctrl Pts',(28.4837116193195,584.209259542846,-48.1752287016001)) ;
#50799=CARTESIAN_POINT('Ctrl Pts',(28.6502667192815,584.064247376582,-48.1643964993453)) ;
#50800=CARTESIAN_POINT('Ctrl Pts',(28.7713071806064,583.979822089249,-48.1574409409065)) ;
#50801=CARTESIAN_POINT('Ctrl Pts',(28.9586369416767,583.877064778857,-48.14673438553)) ;
#50802=CARTESIAN_POINT('Ctrl Pts',(29.0184584731459,583.84793292598,-48.1433289198448)) ;
#50803=CARTESIAN_POINT('Ctrl Pts',(29.1253764569807,583.802141862425,-48.1371938378907)) ;
#50804=CARTESIAN_POINT('Ctrl Pts',(29.1718642480738,583.784202735805,-48.1345115149232)) ;
#50805=CARTESIAN_POINT('Ctrl Pts',(29.2801842777808,583.74686703889,-48.128208125788)) ;
#50806=CARTESIAN_POINT('Ctrl Pts',(29.3423712526496,583.728671157219,-48.1245498503397)) ;
#50807=CARTESIAN_POINT('Ctrl Pts',(29.4832857838523,583.694575836378,-48.1161735945466)) ;
#50808=CARTESIAN_POINT('Ctrl Pts',(29.5622947888377,583.680293189844,-48.1114170702281)) ;
#50809=CARTESIAN_POINT('Ctrl Pts',(29.7821550571299,583.653714991094,-48.098143462204)) ;
#50810=CARTESIAN_POINT('Ctrl Pts',(29.9237589071104,583.651266642562,-48.0895336769122)) ;
#50811=CARTESIAN_POINT('Ctrl Pts',(30.0969004817843,583.666149365845,-48.0796441104913)) ;
#50812=CARTESIAN_POINT('Ctrl Pts',(30.1292337505538,583.669703568193,-48.0778263956943)) ;
#50813=CARTESIAN_POINT('Ctrl Pts',(30.1939115380498,583.678371884333,-48.0742674485293)) ;
#50814=CARTESIAN_POINT('Ctrl Pts',(30.226245537593,583.683494433374,-48.0725272163753)) ;
#50815=CARTESIAN_POINT('Ctrl Pts',(30.3592048794961,583.707828772456,-48.0654823232685)) ;
#50816=CARTESIAN_POINT('Ctrl Pts',(30.4584549829245,583.73378062531,-48.0604835032138)) ;
#50817=CARTESIAN_POINT('Ctrl Pts',(30.6960009096934,583.815283694953,-48.0483141553702)) ;
#50818=CARTESIAN_POINT('Ctrl Pts',(30.8309737141318,583.878654430109,-48.0411895723705)) ;
#50819=CARTESIAN_POINT('Ctrl Pts',(31.0040371455349,583.984137549062,-48.0307774336922)) ;
#50820=CARTESIAN_POINT('Ctrl Pts',(31.0490198906013,584.01404791213,-48.0279445342932)) ;
#50821=CARTESIAN_POINT('Ctrl Pts',(31.1346951689422,584.076018931988,-48.0222621277005)) ;
#50822=CARTESIAN_POINT('Ctrl Pts',(31.1754568321568,584.107915029271,-48.0194203834038)) ;
#50823=CARTESIAN_POINT('Ctrl Pts',(31.2896151106487,584.204409594192,-48.0110342415765)) ;
#50824=CARTESIAN_POINT('Ctrl Pts',(31.3596551015355,584.272743679219,-48.0053376464281)) ;
#50825=CARTESIAN_POINT('Ctrl Pts',(31.5154689791388,584.448110285689,-47.9913658277476)) ;
#50826=CARTESIAN_POINT('Ctrl Pts',(31.5959248378698,584.559250743006,-47.982993681087)) ;
#50827=CARTESIAN_POINT('Ctrl Pts',(31.6877042577938,584.717061875886,-47.9723182844464)) ;
#50828=CARTESIAN_POINT('Ctrl Pts',(31.709353350906,584.757318266474,-47.9696931626625)) ;
#50829=CARTESIAN_POINT('Ctrl Pts',(31.7426187720382,584.824451387697,-47.9655136988059)) ;
#50830=CARTESIAN_POINT('Ctrl Pts',(31.7550332301088,584.850909049513,-47.9639172304712)) ;
#50831=CARTESIAN_POINT('Ctrl Pts',(31.7850205938924,584.918533387881,-47.959960490056)) ;
#50832=CARTESIAN_POINT('Ctrl Pts',(31.8018202341635,584.960024105956,-47.9576418861994)) ;
#50833=CARTESIAN_POINT('Ctrl Pts',(31.8386354329746,585.060240318765,-47.9522248476218)) ;
#50834=CARTESIAN_POINT('Ctrl Pts',(31.8573734922608,585.119388711621,-47.9491728441143)) ;
#50835=CARTESIAN_POINT('Ctrl Pts',(31.9078613298227,585.308017126589,-47.9396497905559)) ;
#50836=CARTESIAN_POINT('Ctrl Pts',(31.9297102836829,585.439777701415,-47.9332804013813)) ;
#50837=CARTESIAN_POINT('Ctrl Pts',(31.9417213650514,585.618420883782,-47.9242558801685)) ;
#50838=CARTESIAN_POINT('Ctrl Pts',(31.94326489026,585.664203639874,-47.9219118724121)) ;
#50839=CARTESIAN_POINT('Ctrl Pts',(31.9432775469358,585.709997258212,-47.9195222884686)) ;
#50840=CARTESIAN_POINT('Ctrl Pts',(31.9432775472728,585.709998478805,-47.9195222247762)) ;
#50841=CARTESIAN_POINT('Ctrl Pts',(31.9432895684224,585.753586358521,-47.9172477390332)) ;
#50842=CARTESIAN_POINT('Ctrl Pts',(31.9419146380902,585.797161735405,-47.9149331527379)) ;
#50843=CARTESIAN_POINT('Ctrl Pts',(31.9358506616059,585.892746243631,-47.909749736901)) ;
#50844=CARTESIAN_POINT('Ctrl Pts',(31.930563087351,585.944684850245,-47.9068634703778)) ;
#50845=CARTESIAN_POINT('Ctrl Pts',(31.9003772973783,586.159596891199,-47.8946101911145)) ;
#50846=CARTESIAN_POINT('Ctrl Pts',(31.8578935033976,586.319457659665,-47.8846822993874)) ;
#50847=CARTESIAN_POINT('Ctrl Pts',(31.7628877887553,586.557400188683,-47.8692846858374)) ;
#50848=CARTESIAN_POINT('Ctrl Pts',(31.7233554077588,586.639954947482,-47.863830861321)) ;
#50849=CARTESIAN_POINT('Ctrl Pts',(31.6625049858158,586.747896583627,-47.8567799774564)) ;
#50850=CARTESIAN_POINT('Ctrl Pts',(31.6458876683006,586.775806074372,-47.8549651672118)) ;
#50851=CARTESIAN_POINT('Ctrl Pts',(31.6107687354862,586.831729338061,-47.8513642082803)) ;
#50852=CARTESIAN_POINT('Ctrl Pts',(31.5922286585981,586.859706854857,-47.8495807371591)) ;
#50853=CARTESIAN_POINT('Ctrl Pts',(31.4990396814934,586.993114972238,-47.8411013358479)) ;
#50854=CARTESIAN_POINT('Ctrl Pts',(31.4152399003025,587.091810923917,-47.8348922752838)) ;
#50855=CARTESIAN_POINT('Ctrl Pts',(31.2365275719078,587.266000864805,-47.8227667067565)) ;
#50856=CARTESIAN_POINT('Ctrl Pts',(31.1431270040543,587.342270131788,-47.8168790170872)) ;
#50857=CARTESIAN_POINT('Ctrl Pts',(30.9991790775615,587.440112871951,-47.8078961187918)) ;
#50858=CARTESIAN_POINT('Ctrl Pts',(30.9535984076406,587.468548511161,-47.805066468503)) ;
#50859=CARTESIAN_POINT('Ctrl Pts',(30.8604330062125,587.521715931628,-47.7992796666911)) ;
#50860=CARTESIAN_POINT('Ctrl Pts',(30.8128901665524,587.546435612866,-47.7963251109806)) ;
#50861=CARTESIAN_POINT('Ctrl Pts',(30.6623647751032,587.617370489837,-47.786948339349)) ;
#50862=CARTESIAN_POINT('Ctrl Pts',(30.5565148256575,587.656976667338,-47.7803105145352)) ;
#50863=CARTESIAN_POINT('Ctrl Pts',(30.3558578954533,587.713753215226,-47.7678217929438)) ;
#50864=CARTESIAN_POINT('Ctrl Pts',(30.2620448222929,587.733346711718,-47.7620232198825)) ;
#50865=CARTESIAN_POINT('Ctrl Pts',(30.110847350709,587.754044411417,-47.7529976444087)) ;
#50866=CARTESIAN_POINT('Ctrl Pts',(30.0541867181453,587.759416452001,-47.7496872861673)) ;
#50867=CARTESIAN_POINT('Ctrl Pts',(29.9679728019198,587.763989806308,-47.7448290838786)) ;
#50868=CARTESIAN_POINT('Ctrl Pts',(29.9385405751248,587.764917459924,-47.7432022773115)) ;
#50869=CARTESIAN_POINT('Ctrl Pts',(29.8746247144214,587.765557282675,-47.7397526626701)) ;
#50870=CARTESIAN_POINT('Ctrl Pts',(29.8401484109236,587.765034845209,-47.7379427791917)) ;
#50871=CARTESIAN_POINT('Ctrl Pts',(29.6929166270205,587.759095008949,-47.7303693937815)) ;
#50872=CARTESIAN_POINT('Ctrl Pts',(29.5806884191535,587.745258862525,-47.7249803758292)) ;
#50873=CARTESIAN_POINT('Ctrl Pts',(29.3345856097655,587.694077198643,-47.7129907238908)) ;
#50874=CARTESIAN_POINT('Ctrl Pts',(29.2022252623547,587.652254408195,-47.7064054927449)) ;
#50875=CARTESIAN_POINT('Ctrl Pts',(29.0240310954337,587.575433414706,-47.6965489186305)) ;
#50876=CARTESIAN_POINT('Ctrl Pts',(28.9739003634705,587.551364997342,-47.6936617107901)) ;
#50877=CARTESIAN_POINT('Ctrl Pts',(28.8807610553989,587.501903095422,-47.6880428240056)) ;
#50878=CARTESIAN_POINT('Ctrl Pts',(28.8375816763748,587.47691649689,-47.6853276874536)) ;
#50879=CARTESIAN_POINT('Ctrl Pts',(28.725968023883,587.406786937141,-47.6779993969809)) ;
#50880=CARTESIAN_POINT('Ctrl Pts',(28.6592572347831,587.359081152255,-47.6732925638568)) ;
#50881=CARTESIAN_POINT('Ctrl Pts',(28.4895986556163,587.221720134921,-47.6604797202275)) ;
#50882=CARTESIAN_POINT('Ctrl Pts',(28.3924300419724,587.125584971483,-47.6522051418259)) ;
#50883=CARTESIAN_POINT('Ctrl Pts',(28.2722415573568,586.980344142012,-47.6411528064696)) ;
#50884=CARTESIAN_POINT('Ctrl Pts',(28.2405213517831,586.938895515114,-47.63814304934)) ;
#50885=CARTESIAN_POINT('Ctrl Pts',(28.1931909144416,586.871909861343,-47.6335563983695)) ;
#50886=CARTESIAN_POINT('Ctrl Pts',(28.1765029272481,586.847165294975,-47.6319196288005)) ;
#50887=CARTESIAN_POINT('Ctrl Pts',(28.1379146701452,586.787167736202,-47.6280933869951)) ;
#50888=CARTESIAN_POINT('Ctrl Pts',(28.116532481735,586.751599510589,-47.6259339184782)) ;
#50889=CARTESIAN_POINT('Ctrl Pts',(28.0428274433261,586.620135298275,-47.6182551168412)) ;
#50890=CARTESIAN_POINT('Ctrl Pts',(27.9970912172832,586.520749762445,-47.6130114496642)) ;
#50891=CARTESIAN_POINT('Ctrl Pts',(27.9138997018933,586.293962202881,-47.6013822923232)) ;
#50892=CARTESIAN_POINT('Ctrl Pts',(27.8804391956897,586.165630924532,-47.5950040210229)) ;
#50893=CARTESIAN_POINT('Ctrl Pts',(27.8501584134073,585.976245863917,-47.5852178133009)) ;
#50894=CARTESIAN_POINT('Ctrl Pts',(27.843322911764,585.917137363842,-47.5821164177999)) ;
#50895=CARTESIAN_POINT('Ctrl Pts',(27.8350567191064,585.802089177468,-47.5759510157502)) ;
#50896=CARTESIAN_POINT('Ctrl Pts',(27.8333276045775,585.746223199151,-47.5728988394472)) ;
#50897=CARTESIAN_POINT('Ctrl Pts',(27.8344573756436,585.631340513076,-47.5664927294243)) ;
#50898=CARTESIAN_POINT('Ctrl Pts',(27.8375803875382,585.572377758809,-47.5631343847387)) ;
#50899=CARTESIAN_POINT('Ctrl Pts',(27.849888613493,585.444546476883,-47.5557168352009)) ;
#50900=CARTESIAN_POINT('Ctrl Pts',(27.8600298425148,585.375914399032,-47.5516467875374)) ;
#50901=CARTESIAN_POINT('Ctrl Pts',(27.8735991218939,585.307997541154,-47.5475669749032)) ;
#50902=CARTESIAN_POINT('',(28.6364422247127,587.339761192919,-47.7296814414421)) ;
#50903=CARTESIAN_POINT('Ctrl Pts',(27.8735990504334,585.307997898828,-47.6045419700025)) ;
#50904=CARTESIAN_POINT('Ctrl Pts',(27.8564936227868,585.393613939248,-47.6097650867871)) ;
#50905=CARTESIAN_POINT('Ctrl Pts',(27.8448606829014,585.480241673589,-47.6150312344685)) ;
#50906=CARTESIAN_POINT('Ctrl Pts',(27.8358843342787,585.608720025698,-47.622630874679)) ;
#50907=CARTESIAN_POINT('Ctrl Pts',(27.8342469626353,585.650164533989,-47.6250494566789)) ;
#50908=CARTESIAN_POINT('Ctrl Pts',(27.8335474492433,585.726077930594,-47.6293875477471)) ;
#50909=CARTESIAN_POINT('Ctrl Pts',(27.8340962817061,585.760528524501,-47.6313215203702)) ;
#50910=CARTESIAN_POINT('Ctrl Pts',(27.8367863735249,585.825975415845,-47.6349087658605)) ;
#50911=CARTESIAN_POINT('Ctrl Pts',(27.8387646497125,585.856967034994,-47.636568643584)) ;
#50912=CARTESIAN_POINT('Ctrl Pts',(27.8476753019987,585.95982645283,-47.6419806542633)) ;
#50913=CARTESIAN_POINT('Ctrl Pts',(27.8576927934502,586.031378326314,-47.6455893746302)) ;
#50914=CARTESIAN_POINT('Ctrl Pts',(27.9032444872837,586.26595130639,-47.6573146546028)) ;
#50915=CARTESIAN_POINT('Ctrl Pts',(27.9548368867758,586.425158873018,-47.6651545488101)) ;
#50916=CARTESIAN_POINT('Ctrl Pts',(28.0502896792992,586.630593307613,-47.6766305303463)) ;
#50917=CARTESIAN_POINT('Ctrl Pts',(28.0778286365599,586.683672968718,-47.6797241666656)) ;
#50918=CARTESIAN_POINT('Ctrl Pts',(28.1324953542873,586.778662171874,-47.6855489862616)) ;
#50919=CARTESIAN_POINT('Ctrl Pts',(28.1589114778527,586.820929036927,-47.6882526683113)) ;
#50920=CARTESIAN_POINT('Ctrl Pts',(28.2277374707619,586.922629200175,-47.6950570249377)) ;
#50921=CARTESIAN_POINT('Ctrl Pts',(28.2718254573564,586.980838934933,-47.6992196674799)) ;
#50922=CARTESIAN_POINT('Ctrl Pts',(28.4136315333929,587.148696520203,-47.7120397130181)) ;
#50923=CARTESIAN_POINT('Ctrl Pts',(28.5200895330464,587.250341602668,-47.7209796683478)) ;
#50924=CARTESIAN_POINT('Ctrl Pts',(28.6364501397495,587.339767275828,-47.7296820333927)) ;
#50925=CARTESIAN_POINT('Ctrl Pts',(28.6364422247126,587.339761192919,-47.7296814414422)) ;
#50926=CARTESIAN_POINT('Ctrl Pts',(28.6824239637675,587.375099521165,-47.733120337256)) ;
#50927=CARTESIAN_POINT('Ctrl Pts',(28.7298764916139,587.408472467074,-47.7365108495857)) ;
#50928=CARTESIAN_POINT('Ctrl Pts',(28.8011066382216,587.454188607936,-47.7413072153448)) ;
#50929=CARTESIAN_POINT('Ctrl Pts',(28.8238032681358,587.468140002077,-47.7427942145078)) ;
#50930=CARTESIAN_POINT('Ctrl Pts',(28.8736065695272,587.497434626283,-47.7459576724762)) ;
#50931=CARTESIAN_POINT('Ctrl Pts',(28.9008028245355,587.512610394951,-47.7476214770647)) ;
#50932=CARTESIAN_POINT('Ctrl Pts',(28.9755781080381,587.552134138423,-47.7520520266294)) ;
#50933=CARTESIAN_POINT('Ctrl Pts',(29.0237816085301,587.575255016306,-47.7547547867105)) ;
#50934=CARTESIAN_POINT('Ctrl Pts',(29.1963957008045,587.649914106246,-47.7640861401261)) ;
#50935=CARTESIAN_POINT('Ctrl Pts',(29.3249122544347,587.691085679759,-47.7704390440422)) ;
#50936=CARTESIAN_POINT('Ctrl Pts',(29.521901707099,587.733447543895,-47.780329622509)) ;
#50937=CARTESIAN_POINT('Ctrl Pts',(29.5879097366807,587.744304487177,-47.7836642756877)) ;
#50938=CARTESIAN_POINT('Ctrl Pts',(29.7081549116701,587.758100000751,-47.7898716357544)) ;
#50939=CARTESIAN_POINT('Ctrl Pts',(29.7622030695182,587.762143729498,-47.7927092136559)) ;
#50940=CARTESIAN_POINT('Ctrl Pts',(29.8674117401597,587.765841961987,-47.7983577551711)) ;
#50941=CARTESIAN_POINT('Ctrl Pts',(29.9185241183404,587.765731371519,-47.8011589785321)) ;
#50942=CARTESIAN_POINT('Ctrl Pts',(30.0617085907539,587.760079130019,-47.8091822413788)) ;
#50943=CARTESIAN_POINT('Ctrl Pts',(30.1534808935024,587.750245395855,-47.8145343646433)) ;
#50944=CARTESIAN_POINT('Ctrl Pts',(30.359317180954,587.714061767701,-47.8269363661386)) ;
#50945=CARTESIAN_POINT('Ctrl Pts',(30.4724214579021,587.684066653035,-47.8340407963561)) ;
#50946=CARTESIAN_POINT('Ctrl Pts',(30.6247391686622,587.629423422938,-47.8436530868642)) ;
#50947=CARTESIAN_POINT('Ctrl Pts',(30.666607235695,587.612831446989,-47.8462980778568)) ;
#50948=CARTESIAN_POINT('Ctrl Pts',(30.7412348310008,587.580380508186,-47.8509781550086)) ;
#50949=CARTESIAN_POINT('Ctrl Pts',(30.7741830627879,587.565001414862,-47.8530317237531)) ;
#50950=CARTESIAN_POINT('Ctrl Pts',(30.8335104181901,587.53536725649,-47.8566827033609)) ;
#50951=CARTESIAN_POINT('Ctrl Pts',(30.8600163426123,587.521395047013,-47.858294053187)) ;
#50952=CARTESIAN_POINT('Ctrl Pts',(30.9386460594716,587.47772299346,-47.8630368487413)) ;
#50953=CARTESIAN_POINT('Ctrl Pts',(30.989787787867,587.446313630178,-47.8660737633124)) ;
#50954=CARTESIAN_POINT('Ctrl Pts',(31.1511088600168,587.337231335096,-47.8757313328263)) ;
#50955=CARTESIAN_POINT('Ctrl Pts',(31.2550393687273,587.250955542727,-47.882098111838)) ;
#50956=CARTESIAN_POINT('Ctrl Pts',(31.3969579715102,587.107396990695,-47.8920286314581)) ;
#50957=CARTESIAN_POINT('Ctrl Pts',(31.4417690113181,587.057391616715,-47.8953846192265)) ;
#50958=CARTESIAN_POINT('Ctrl Pts',(31.5178336423956,586.963654900244,-47.9015933280279)) ;
#50959=CARTESIAN_POINT('Ctrl Pts',(31.5499715471862,586.920720269273,-47.9044087387962)) ;
#50960=CARTESIAN_POINT('Ctrl Pts',(31.6098659187617,586.833814757294,-47.9100849141257)) ;
#50961=CARTESIAN_POINT('Ctrl Pts',(31.6377054130344,586.789949960652,-47.9129394017441)) ;
#50962=CARTESIAN_POINT('Ctrl Pts',(31.7563361671869,586.586368562414,-47.926166304809)) ;
#50963=CARTESIAN_POINT('Ctrl Pts',(31.8271070476719,586.41599171671,-47.9372812364368)) ;
#50964=CARTESIAN_POINT('Ctrl Pts',(31.8946776028362,586.161847301536,-47.9530245803131)) ;
#50965=CARTESIAN_POINT('Ctrl Pts',(31.9106083177976,586.084042191839,-47.9577222140946)) ;
#50966=CARTESIAN_POINT('Ctrl Pts',(31.9265403086592,585.974198569042,-47.9640213406026)) ;
#50967=CARTESIAN_POINT('Ctrl Pts',(31.9303579035701,585.942788656879,-47.9657847128987)) ;
#50968=CARTESIAN_POINT('Ctrl Pts',(31.9367236079293,585.877940180081,-47.9693303378259)) ;
#50969=CARTESIAN_POINT('Ctrl Pts',(31.9391817100796,585.844502811593,-47.9711079582763)) ;
#50970=CARTESIAN_POINT('Ctrl Pts',(31.9471323072716,585.682069113005,-47.9795619645583)) ;
#50971=CARTESIAN_POINT('Ctrl Pts',(31.9412774670893,585.552797949443,-47.9857492176068)) ;
#50972=CARTESIAN_POINT('Ctrl Pts',(31.9063792546025,585.304199292865,-47.9979042033426)) ;
#50973=CARTESIAN_POINT('Ctrl Pts',(31.8787237778798,585.185232675492,-48.0038451310871)) ;
#50974=CARTESIAN_POINT('Ctrl Pts',(31.824026800936,585.018689038426,-48.0128699415235)) ;
#50975=CARTESIAN_POINT('Ctrl Pts',(31.805392504124,584.968623134488,-48.0156770104237)) ;
#50976=CARTESIAN_POINT('Ctrl Pts',(31.7647433622415,584.871200380387,-48.0213587486375)) ;
#50977=CARTESIAN_POINT('Ctrl Pts',(31.7428317519569,584.823844107924,-48.0242282133877)) ;
#50978=CARTESIAN_POINT('Ctrl Pts',(31.6377074933674,584.617624340005,-48.0372337905549)) ;
#50979=CARTESIAN_POINT('Ctrl Pts',(31.5357205058415,584.469241835868,-48.0480686431251)) ;
#50980=CARTESIAN_POINT('Ctrl Pts',(31.3606108890533,584.274676360172,-48.0637589076327)) ;
#50981=CARTESIAN_POINT('Ctrl Pts',(31.3017641100319,584.216720889008,-48.0686546326443)) ;
#50982=CARTESIAN_POINT('Ctrl Pts',(31.2156033532213,584.141526958755,-48.0751505388989)) ;
#50983=CARTESIAN_POINT('Ctrl Pts',(31.1911346901922,584.121154563864,-48.0769265792578)) ;
#50984=CARTESIAN_POINT('Ctrl Pts',(31.1402183921068,584.080728232137,-48.080467117722)) ;
#50985=CARTESIAN_POINT('Ctrl Pts',(31.1137388779886,584.060730060345,-48.0822281910013)) ;
#50986=CARTESIAN_POINT('Ctrl Pts',(30.978719694028,583.963803844077,-48.0908771326382)) ;
#50987=CARTESIAN_POINT('Ctrl Pts',(30.8633639178683,583.896895993447,-48.0972385578789)) ;
#50988=CARTESIAN_POINT('Ctrl Pts',(30.6336529125506,583.791955335237,-48.109468931987)) ;
#50989=CARTESIAN_POINT('Ctrl Pts',(30.5208503590398,583.751881955797,-48.1153012344371)) ;
#50990=CARTESIAN_POINT('Ctrl Pts',(30.3536895456436,583.708452298691,-48.124196677322)) ;
#50991=CARTESIAN_POINT('Ctrl Pts',(30.3016679832874,583.697074192168,-48.1269959652828)) ;
#50992=CARTESIAN_POINT('Ctrl Pts',(30.1978439860137,583.678558937028,-48.1326742082429)) ;
#50993=CARTESIAN_POINT('Ctrl Pts',(30.146094564906,583.671353434077,-48.1355485533053)) ;
#50994=CARTESIAN_POINT('Ctrl Pts',(29.9183362257767,583.648448531857,-48.1484152304664)) ;
#50995=CARTESIAN_POINT('Ctrl Pts',(29.7410198324542,583.653520172812,-48.1590814486319)) ;
#50996=CARTESIAN_POINT('Ctrl Pts',(29.4833452460618,583.694398698308,-48.1747279541632)) ;
#50997=CARTESIAN_POINT('Ctrl Pts',(29.4009942358834,583.712712929357,-48.1797337826392)) ;
#50998=CARTESIAN_POINT('Ctrl Pts',(29.2893122274845,583.744869873336,-48.1863379078977)) ;
#50999=CARTESIAN_POINT('Ctrl Pts',(29.2588368531494,583.754419225053,-48.1881200510754)) ;
#51000=CARTESIAN_POINT('Ctrl Pts',(29.1973095361061,583.775285748045,-48.1916594170515)) ;
#51001=CARTESIAN_POINT('Ctrl Pts',(29.1662834416572,583.786649239736,-48.1934137471815)) ;
#51002=CARTESIAN_POINT('Ctrl Pts',(29.0102494313651,583.848104778917,-48.2021442611999)) ;
#51003=CARTESIAN_POINT('Ctrl Pts',(28.8900962194717,583.909655925334,-48.2085781117679)) ;
#51004=CARTESIAN_POINT('Ctrl Pts',(28.675545236477,584.047684154462,-48.2209340870237)) ;
#51005=CARTESIAN_POINT('Ctrl Pts',(28.5801994991868,584.121611589251,-48.2268168573551)) ;
#51006=CARTESIAN_POINT('Ctrl Pts',(28.4531719460388,584.239328606531,-48.2357514893828)) ;
#51007=CARTESIAN_POINT('Ctrl Pts',(28.4158607922054,584.276677212472,-48.2385311079599)) ;
#51008=CARTESIAN_POINT('Ctrl Pts',(28.3442567741649,584.354098782591,-48.2442168507004)) ;
#51009=CARTESIAN_POINT('Ctrl Pts',(28.3099865598374,584.394137846638,-48.2471206136923)) ;
#51010=CARTESIAN_POINT('Ctrl Pts',(28.1749867453748,584.56472294007,-48.2593677038929)) ;
#51011=CARTESIAN_POINT('Ctrl Pts',(28.0886231978602,584.705824474986,-48.2692774453331)) ;
#51012=CARTESIAN_POINT('Ctrl Pts',(27.9934242252772,584.913898527553,-48.2830221519237)) ;
#51013=CARTESIAN_POINT('Ctrl Pts',(27.9695268578066,584.973319331029,-48.2868490426797)) ;
#51014=CARTESIAN_POINT('Ctrl Pts',(27.9334539723609,585.076723707667,-48.2932466069319)) ;
#51015=CARTESIAN_POINT('Ctrl Pts',(27.9198964153185,585.120175665592,-48.2958584953778)) ;
#51016=CARTESIAN_POINT('Ctrl Pts',(27.9000910882341,585.191955481162,-48.3000097033398)) ;
#51017=CARTESIAN_POINT('Ctrl Pts',(27.8929810953536,585.220024496866,-48.3015911007769)) ;
#51018=CARTESIAN_POINT('Ctrl Pts',(27.881880517771,585.268094598002,-48.3042289210213)) ;
#51019=CARTESIAN_POINT('Ctrl Pts',(27.8775912202124,585.28801630178,-48.3053027255326)) ;
#51020=CARTESIAN_POINT('Ctrl Pts',(27.8735990519255,585.30799789136,-48.3063633758768)) ;
#51021=CARTESIAN_POINT('Origin',(29.8885276254155,585.710565160562,-51.0680854522906)) ;
#51022=CARTESIAN_POINT('',(27.87359904473,585.307997927374,-49.0033678628587)) ;
#51023=CARTESIAN_POINT('',(27.8735990520585,585.307997890694,-48.9453612460011)) ;
#51024=CARTESIAN_POINT('',(27.8735990520584,585.307997890694,-51.0680854522905)) ;
#51025=CARTESIAN_POINT('',(28.6368801712448,587.339287485482,-49.1271361537871)) ;
#51026=CARTESIAN_POINT('Ctrl Pts',(27.873599044712,585.307997927464,-49.0033678610064)) ;
#51027=CARTESIAN_POINT('Ctrl Pts',(27.8698044451442,585.326990648413,-49.0043292920081)) ;
#51028=CARTESIAN_POINT('Ctrl Pts',(27.8662773002645,585.346042440035,-49.0052965367617)) ;
#51029=CARTESIAN_POINT('Ctrl Pts',(27.8522738852341,585.428157689329,-49.0094833265671)) ;
#51030=CARTESIAN_POINT('Ctrl Pts',(27.8444753952256,585.491629795012,-49.0127661281195)) ;
#51031=CARTESIAN_POINT('Ctrl Pts',(27.8359270169899,585.604476743004,-49.0187470486518)) ;
#51032=CARTESIAN_POINT('Ctrl Pts',(27.8339739363669,585.653709544196,-49.0214042849436)) ;
#51033=CARTESIAN_POINT('Ctrl Pts',(27.8335495298772,585.768407778413,-49.0277249220421)) ;
#51034=CARTESIAN_POINT('Ctrl Pts',(27.8364342456864,585.833821556768,-49.0314290385932)) ;
#51035=CARTESIAN_POINT('Ctrl Pts',(27.8499665688143,585.980774838618,-49.0399727484017)) ;
#51036=CARTESIAN_POINT('Ctrl Pts',(27.8623957923818,586.062036905603,-49.0448547447766)) ;
#51037=CARTESIAN_POINT('Ctrl Pts',(27.9082682901971,586.275467394998,-49.0579623338322)) ;
#51038=CARTESIAN_POINT('Ctrl Pts',(27.9500484921029,586.405434989352,-49.0662576607064)) ;
#51039=CARTESIAN_POINT('Ctrl Pts',(28.0174950170872,586.560456219298,-49.0759010162996)) ;
#51040=CARTESIAN_POINT('Ctrl Pts',(28.03132982233,586.590277867984,-49.0777424831793)) ;
#51041=CARTESIAN_POINT('Ctrl Pts',(28.0601800189521,586.64874837403,-49.0813066865867)) ;
#51042=CARTESIAN_POINT('Ctrl Pts',(28.0751680862041,586.677400285444,-49.0830304273165)) ;
#51043=CARTESIAN_POINT('Ctrl Pts',(28.1336480025451,586.78304487914,-49.0893437095975)) ;
#51044=CARTESIAN_POINT('Ctrl Pts',(28.1814216529146,586.857564431637,-49.0937131246284)) ;
#51045=CARTESIAN_POINT('Ctrl Pts',(28.3174912346045,587.042384919887,-49.104909569831)) ;
#51046=CARTESIAN_POINT('Ctrl Pts',(28.4126026257719,587.147069027542,-49.1116446440223)) ;
#51047=CARTESIAN_POINT('Ctrl Pts',(28.5560453762575,587.275538057089,-49.1213964028017)) ;
#51048=CARTESIAN_POINT('Ctrl Pts',(28.5956789397844,587.308435868694,-49.1240512373501)) ;
#51049=CARTESIAN_POINT('Ctrl Pts',(28.6365041795376,587.339808805163,-49.1267657875976)) ;
#51050=CARTESIAN_POINT('',(31.9432775542228,585.710024266058,-49.3762357692215)) ;
#51051=CARTESIAN_POINT('Ctrl Pts',(31.9427342614473,585.709985596129,-49.3752948960846)) ;
#51052=CARTESIAN_POINT('Ctrl Pts',(31.9426172492493,585.780898218238,-49.3712207238047)) ;
#51053=CARTESIAN_POINT('Ctrl Pts',(31.9388560335549,585.851852550851,-49.3672016667734)) ;
#51054=CARTESIAN_POINT('Ctrl Pts',(31.9314771415032,585.922451909701,-49.3632671281545)) ;
#51055=CARTESIAN_POINT('Ctrl Pts',(31.9241001716764,585.993032877193,-49.3593336144954)) ;
#51056=CARTESIAN_POINT('Ctrl Pts',(31.9131074252591,586.063259034058,-49.3554846054318)) ;
#51057=CARTESIAN_POINT('Ctrl Pts',(31.8985598759689,586.132738183609,-49.3517248952043)) ;
#51058=CARTESIAN_POINT('Ctrl Pts',(31.8840111309949,586.202223043751,-49.347964875961)) ;
#51059=CARTESIAN_POINT('Ctrl Pts',(31.8659069048801,586.27096070311,-49.3442940977577)) ;
#51060=CARTESIAN_POINT('Ctrl Pts',(31.8443432717175,586.338563738127,-49.3406930811079)) ;
#51061=CARTESIAN_POINT('Ctrl Pts',(31.8227548532057,586.406244476415,-49.3370879254312)) ;
#51062=CARTESIAN_POINT('Ctrl Pts',(31.7976988646946,586.472787848852,-49.3335525062726)) ;
#51063=CARTESIAN_POINT('Ctrl Pts',(31.7693091276861,586.537811473414,-49.3300448494271)) ;
#51064=CARTESIAN_POINT('Ctrl Pts',(31.7409018983242,586.602875162322,-49.3265350313368)) ;
#51065=CARTESIAN_POINT('Ctrl Pts',(31.709156496649,586.666416994456,-49.3230526645967)) ;
#51066=CARTESIAN_POINT('Ctrl Pts',(31.6742483334829,586.728062954153,-49.3195371923347)) ;
#51067=CARTESIAN_POINT('Ctrl Pts',(31.64135561025,586.786149754111,-49.316224687589)) ;
#51068=CARTESIAN_POINT('Ctrl Pts',(31.605654388214,586.842553459408,-49.3128822981287)) ;
#51069=CARTESIAN_POINT('Ctrl Pts',(31.5673306236686,586.896971209509,-49.3094494968086)) ;
#51070=CARTESIAN_POINT('Ctrl Pts',(31.5649058173613,586.900414308203,-49.3092322979402)) ;
#51071=CARTESIAN_POINT('Ctrl Pts',(31.5624705110518,586.903849473833,-49.3090147371263)) ;
#51072=CARTESIAN_POINT('Ctrl Pts',(31.5600247511938,586.907276636694,-49.3087967990357)) ;
#51073=CARTESIAN_POINT('Ctrl Pts',(31.5337788156842,586.944054203026,-49.3064580620361)) ;
#51074=CARTESIAN_POINT('Ctrl Pts',(31.5063302027123,586.979908205151,-49.3040756442879)) ;
#51075=CARTESIAN_POINT('Ctrl Pts',(31.4777482332981,587.014748947238,-49.3016299549295)) ;
#51076=CARTESIAN_POINT('Ctrl Pts',(31.4777263603074,587.014775609894,-49.3016280833111)) ;
#51077=CARTESIAN_POINT('Ctrl Pts',(31.477704486653,587.014802271958,-49.3016262116556)) ;
#51078=CARTESIAN_POINT('Ctrl Pts',(31.4776826123349,587.014828933428,-49.3016243399631)) ;
#51079=CARTESIAN_POINT('Ctrl Pts',(31.436861728681,587.064583389718,-49.2981314702291)) ;
#51080=CARTESIAN_POINT('Ctrl Pts',(31.3935720803975,587.112452150401,-49.2945002447966)) ;
#51081=CARTESIAN_POINT('Ctrl Pts',(31.3480347240497,587.158205432452,-49.2907957449888)) ;
#51082=CARTESIAN_POINT('Ctrl Pts',(31.3434184878396,587.162843557593,-49.290420210537)) ;
#51083=CARTESIAN_POINT('Ctrl Pts',(31.3387791966602,587.167459934781,-49.2900439230894)) ;
#51084=CARTESIAN_POINT('Ctrl Pts',(31.3341171101784,587.172054319618,-49.2896669504441)) ;
#51085=CARTESIAN_POINT('Ctrl Pts',(31.2835431316144,587.221893875607,-49.285577578323)) ;
#51086=CARTESIAN_POINT('Ctrl Pts',(31.23028090373,587.26914702563,-49.281408189495)) ;
#51087=CARTESIAN_POINT('Ctrl Pts',(31.1746498895808,587.313549893559,-49.277233146996)) ;
#51088=CARTESIAN_POINT('Ctrl Pts',(31.1190876190499,587.357897892566,-49.2730632636251)) ;
#51089=CARTESIAN_POINT('Ctrl Pts',(31.0611626005585,587.399402981729,-49.2688880941617)) ;
#51090=CARTESIAN_POINT('Ctrl Pts',(31.0012105162553,587.437838534679,-49.2647623759951)) ;
#51091=CARTESIAN_POINT('Ctrl Pts',(30.9412984971703,587.476248401636,-49.2606394149936)) ;
#51092=CARTESIAN_POINT('Ctrl Pts',(30.8793621854795,587.511592996215,-49.2565660081323)) ;
#51093=CARTESIAN_POINT('Ctrl Pts',(30.815752194817,587.543678693284,-49.2525735976269)) ;
#51094=CARTESIAN_POINT('Ctrl Pts',(30.7521633355493,587.575753731407,-49.2485825134101)) ;
#51095=CARTESIAN_POINT('Ctrl Pts',(30.6869019273906,587.604572051931,-49.2446724121268)) ;
#51096=CARTESIAN_POINT('Ctrl Pts',(30.6203332569447,587.629971459751,-49.2408499953985)) ;
#51097=CARTESIAN_POINT('Ctrl Pts',(30.553764328658,587.655370965951,-49.2370275638647)) ;
#51098=CARTESIAN_POINT('Ctrl Pts',(30.4858881272273,587.677351423859,-49.2332927529147)) ;
#51099=CARTESIAN_POINT('Ctrl Pts',(30.4170848505969,587.695782599759,-49.229627736439)) ;
#51100=CARTESIAN_POINT('Ctrl Pts',(30.3482126673851,587.71423223451,-49.225959049444)) ;
#51101=CARTESIAN_POINT('Ctrl Pts',(30.2784115413041,587.729125234615,-49.2223601185614)) ;
#51102=CARTESIAN_POINT('Ctrl Pts',(30.2080778479719,587.7403656115,-49.2187902775781)) ;
#51103=CARTESIAN_POINT('Ctrl Pts',(30.1377062821471,587.751612040975,-49.2152185143472)) ;
#51104=CARTESIAN_POINT('Ctrl Pts',(30.0668015934413,587.759201521747,-49.2116755348893)) ;
#51105=CARTESIAN_POINT('Ctrl Pts',(29.9957758320383,587.76307726195,-49.2081016313498)) ;
#51106=CARTESIAN_POINT('Ctrl Pts',(29.9285127086579,587.76674768218,-49.2047170577813)) ;
#51107=CARTESIAN_POINT('Ctrl Pts',(29.86114066399,587.767087135098,-49.2013042591977)) ;
#51108=CARTESIAN_POINT('Ctrl Pts',(29.7940228864242,587.764086216671,-49.1978020133309)) ;
#51109=CARTESIAN_POINT('Ctrl Pts',(29.790146426521,587.763912895379,-49.1975997373295)) ;
#51110=CARTESIAN_POINT('Ctrl Pts',(29.7862708020056,587.763728438147,-49.1973971629529)) ;
#51111=CARTESIAN_POINT('Ctrl Pts',(29.782396078083,587.763532845537,-49.197194278406)) ;
#51112=CARTESIAN_POINT('Ctrl Pts',(29.7393732962058,587.761361093854,-49.1949415611081)) ;
#51113=CARTESIAN_POINT('Ctrl Pts',(29.6964635965521,587.757816517172,-49.1926503845548)) ;
#51114=CARTESIAN_POINT('Ctrl Pts',(29.6537643586418,587.752906705734,-49.1903039237657)) ;
#51115=CARTESIAN_POINT('Ctrl Pts',(29.6537316936418,587.752902949718,-49.1903021287186)) ;
#51116=CARTESIAN_POINT('Ctrl Pts',(29.6536990287645,587.752899192904,-49.1903003336392)) ;
#51117=CARTESIAN_POINT('Ctrl Pts',(29.6536663640099,587.752895435292,-49.1902985385274)) ;
#51118=CARTESIAN_POINT('Ctrl Pts',(29.5893679958149,587.745498828152,-49.1867649819548)) ;
#51119=CARTESIAN_POINT('Ctrl Pts',(29.5253262751425,587.734974334743,-49.1830973483189)) ;
#51120=CARTESIAN_POINT('Ctrl Pts',(29.4618575879369,587.721385123318,-49.1793605809766)) ;
#51121=CARTESIAN_POINT('Ctrl Pts',(29.4556601922994,587.720058205695,-49.1789957045841)) ;
#51122=CARTESIAN_POINT('Ctrl Pts',(29.4494682887654,587.718702096905,-49.178630169034)) ;
#51123=CARTESIAN_POINT('Ctrl Pts',(29.4432821898818,587.717316875284,-49.1782640347885)) ;
#51124=CARTESIAN_POINT('Ctrl Pts',(29.3742108042705,587.701850071642,-49.1741759333643)) ;
#51125=CARTESIAN_POINT('Ctrl Pts',(29.3058592650622,587.682749896166,-49.1700139311333)) ;
#51126=CARTESIAN_POINT('Ctrl Pts',(29.2386150934843,587.66014120432,-49.1658496212785)) ;
#51127=CARTESIAN_POINT('Ctrl Pts',(29.2350456187028,587.658941083128,-49.1656285701649)) ;
#51128=CARTESIAN_POINT('Ctrl Pts',(29.2314792738871,587.657731083287,-49.165407512549)) ;
#51129=CARTESIAN_POINT('Ctrl Pts',(29.2279161201886,587.656511226047,-49.1651864591392)) ;
#51130=CARTESIAN_POINT('Ctrl Pts',(29.1605148218425,587.633436172678,-49.161004970468)) ;
#51131=CARTESIAN_POINT('Ctrl Pts',(29.0942511943318,587.606831581313,-49.1568251938135)) ;
#51132=CARTESIAN_POINT('Ctrl Pts',(29.0294972717457,587.576859537621,-49.1526995732383)) ;
#51133=CARTESIAN_POINT('Ctrl Pts',(28.9647862388391,587.546907345874,-49.1485766852627)) ;
#51134=CARTESIAN_POINT('Ctrl Pts',(28.9015828172753,587.513592293906,-49.1445080396037)) ;
#51135=CARTESIAN_POINT('Ctrl Pts',(28.8402394930402,587.47710674899,-49.1405226886402)) ;
#51136=CARTESIAN_POINT('Ctrl Pts',(28.778912778203,587.440631082948,-49.1365384167554)) ;
#51137=CARTESIAN_POINT('Ctrl Pts',(28.7194451568417,587.400986656831,-49.1326374267466)) ;
#51138=CARTESIAN_POINT('Ctrl Pts',(28.6621707030406,587.35839521496,-49.1288240727973)) ;
#51139=CARTESIAN_POINT('Ctrl Pts',(28.6536921476701,587.352090241726,-49.1282595674994)) ;
#51140=CARTESIAN_POINT('Ctrl Pts',(28.6452616206402,587.34572074037,-49.1276969384294)) ;
#51141=CARTESIAN_POINT('Ctrl Pts',(28.6368801712448,587.339287485482,-49.1271361537871)) ;
#51142=CARTESIAN_POINT('',(30.4186978426039,583.72539083489,-49.522160171753)) ;
#51143=CARTESIAN_POINT('Ctrl Pts',(30.4186978426039,583.72539083489,-49.522160171753)) ;
#51144=CARTESIAN_POINT('Ctrl Pts',(30.4888501130091,583.74412603812,-49.5182232094813)) ;
#51145=CARTESIAN_POINT('Ctrl Pts',(30.558074738389,583.766601784023,-49.5142862472096)) ;
#51146=CARTESIAN_POINT('Ctrl Pts',(30.6259577141875,583.792703219057,-49.5103492849379)) ;
#51147=CARTESIAN_POINT('Ctrl Pts',(30.6937865685899,583.81878384407,-49.5064154615077)) ;
#51148=CARTESIAN_POINT('Ctrl Pts',(30.760275471702,583.848484245838,-49.5024816380774)) ;
#51149=CARTESIAN_POINT('Ctrl Pts',(30.8250269986058,583.881640206794,-49.4985478146471)) ;
#51150=CARTESIAN_POINT('Ctrl Pts',(30.8897595713106,583.91478646227,-49.4946151427336)) ;
#51151=CARTESIAN_POINT('Ctrl Pts',(30.9527553659939,583.95138606332,-49.4906824708202)) ;
#51152=CARTESIAN_POINT('Ctrl Pts',(31.0136393435251,583.991227734612,-49.4867497989067)) ;
#51153=CARTESIAN_POINT('Ctrl Pts',(31.0745166320784,584.031065028725,-49.4828175590536)) ;
#51154=CARTESIAN_POINT('Ctrl Pts',(31.1332821791065,584.074143433347,-49.4788853192006)) ;
#51155=CARTESIAN_POINT('Ctrl Pts',(31.1895891663767,584.120207833062,-49.4749530793475)) ;
#51156=CARTESIAN_POINT('Ctrl Pts',(31.2459058658637,584.166280178283,-49.4710201612346)) ;
#51157=CARTESIAN_POINT('Ctrl Pts',(31.2997628065398,584.215339250336,-49.4670872431217)) ;
#51158=CARTESIAN_POINT('Ctrl Pts',(31.3508466536646,584.267089971263,-49.4631543250089)) ;
#51159=CARTESIAN_POINT('Ctrl Pts',(31.4019537376977,584.318864232445,-49.4592196178989)) ;
#51160=CARTESIAN_POINT('Ctrl Pts',(31.4502848981567,584.37333224797,-49.4552849107888)) ;
#51161=CARTESIAN_POINT('Ctrl Pts',(31.4955650057395,584.430163496731,-49.4513502036788)) ;
#51162=CARTESIAN_POINT('Ctrl Pts',(31.5409123064666,584.487079079883,-49.4474096576837)) ;
#51163=CARTESIAN_POINT('Ctrl Pts',(31.5831992298913,584.54636453527,-49.4434691116887)) ;
#51164=CARTESIAN_POINT('Ctrl Pts',(31.6221924502075,584.607658166397,-49.4395285656936)) ;
#51165=CARTESIAN_POINT('Ctrl Pts',(31.6612182030292,584.669002935526,-49.4355847320544)) ;
#51166=CARTESIAN_POINT('Ctrl Pts',(31.6969445538274,584.732358816368,-49.4316408984151)) ;
#51167=CARTESIAN_POINT('Ctrl Pts',(31.7291841391883,584.7973394706,-49.4276970647759)) ;
#51168=CARTESIAN_POINT('Ctrl Pts',(31.7614851795532,584.862443990767,-49.4237457134124)) ;
#51169=CARTESIAN_POINT('Ctrl Pts',(31.7902860006525,584.929179046084,-49.4197943620489)) ;
#51170=CARTESIAN_POINT('Ctrl Pts',(31.8154475092004,584.997138693451,-49.4158430106855)) ;
#51171=CARTESIAN_POINT('Ctrl Pts',(31.8258590807965,585.025259691556,-49.4142079824222)) ;
#51172=CARTESIAN_POINT('Ctrl Pts',(31.8356481175698,585.053590198989,-49.4125729541589)) ;
#51173=CARTESIAN_POINT('Ctrl Pts',(31.8448073056395,585.082100861462,-49.4109379258956)) ;
#51174=CARTESIAN_POINT('Ctrl Pts',(31.8703011837991,585.161458043541,-49.4063869535808)) ;
#51175=CARTESIAN_POINT('Ctrl Pts',(31.8909902102017,585.242454756208,-49.4018359812659)) ;
#51176=CARTESIAN_POINT('Ctrl Pts',(31.9066925957177,585.324549985801,-49.3972850089511)) ;
#51177=CARTESIAN_POINT('Ctrl Pts',(31.9222261861017,585.405762720496,-49.392782957991)) ;
#51178=CARTESIAN_POINT('Ctrl Pts',(31.9328796837084,585.488050365867,-49.3882809070309)) ;
#51179=CARTESIAN_POINT('Ctrl Pts',(31.9385232994617,585.570867992043,-49.3837788560708)) ;
#51180=CARTESIAN_POINT('Ctrl Pts',(31.941675217269,585.617121025933,-49.3812644937877)) ;
#51181=CARTESIAN_POINT('Ctrl Pts',(31.9432653173924,585.663538997459,-49.3787501315046)) ;
#51182=CARTESIAN_POINT('Ctrl Pts',(31.9432775542228,585.710024266058,-49.3762357692215)) ;
#51183=CARTESIAN_POINT('',(29.3554857494733,583.724023010006,-49.520969598848)) ;
#51184=CARTESIAN_POINT('Origin',(29.8885276254156,585.710565160562,-49.522160171753)) ;
#51185=CARTESIAN_POINT('',(31.9432771921379,585.711899534809,-49.3167515585946)) ;
#51186=CARTESIAN_POINT('Ctrl Pts',(29.3561032364248,583.725994216376,-49.5197697712619)) ;
#51187=CARTESIAN_POINT('Ctrl Pts',(29.3727496069743,583.721528297083,-49.5188380786254)) ;
#51188=CARTESIAN_POINT('Ctrl Pts',(29.389452098046,583.717271838321,-49.5179182347525)) ;
#51189=CARTESIAN_POINT('Ctrl Pts',(29.42760619351,583.708058322594,-49.5158469303205)) ;
#51190=CARTESIAN_POINT('Ctrl Pts',(29.4490880857081,583.703234803234,-49.5147020929892)) ;
#51191=CARTESIAN_POINT('Ctrl Pts',(29.5663997223961,583.678867367023,-49.5085458593304)) ;
#51192=CARTESIAN_POINT('Ctrl Pts',(29.6634613133756,583.665837660712,-49.50379362785)) ;
#51193=CARTESIAN_POINT('Ctrl Pts',(29.8914659820262,583.651669118604,-49.4927219890668)) ;
#51194=CARTESIAN_POINT('Ctrl Pts',(30.0223150288558,583.656019056726,-49.4864219419482)) ;
#51195=CARTESIAN_POINT('Ctrl Pts',(30.2079227031544,583.680003598257,-49.476865979507)) ;
#51196=CARTESIAN_POINT('Ctrl Pts',(30.2636620249336,583.689558760685,-49.4739182958809)) ;
#51197=CARTESIAN_POINT('Ctrl Pts',(30.368021836059,583.711914837146,-49.4682127044214)) ;
#51198=CARTESIAN_POINT('Ctrl Pts',(30.41670492817,583.724225328291,-49.465472590941)) ;
#51199=CARTESIAN_POINT('Ctrl Pts',(30.5448306417442,583.761667801151,-49.458034393887)) ;
#51200=CARTESIAN_POINT('Ctrl Pts',(30.6232726258301,583.7898669098,-49.4532402606485)) ;
#51201=CARTESIAN_POINT('Ctrl Pts',(30.8144589531098,583.872025401809,-49.4409931195026)) ;
#51202=CARTESIAN_POINT('Ctrl Pts',(30.9244067011359,583.931652770115,-49.4334202284699)) ;
#51203=CARTESIAN_POINT('Ctrl Pts',(31.0665972759726,584.02644139404,-49.4232832711087)) ;
#51204=CARTESIAN_POINT('Ctrl Pts',(31.1040705280601,584.053285202713,-49.4205781844057)) ;
#51205=CARTESIAN_POINT('Ctrl Pts',(31.1698897288773,584.103869088047,-49.4158069079045)) ;
#51206=CARTESIAN_POINT('Ctrl Pts',(31.1985584653246,584.12715722885,-49.4137214875302)) ;
#51207=CARTESIAN_POINT('Ctrl Pts',(31.2492766783299,584.170677643862,-49.4100429487759)) ;
#51208=CARTESIAN_POINT('Ctrl Pts',(31.2715393300356,584.190640749755,-49.4084346002827)) ;
#51209=CARTESIAN_POINT('Ctrl Pts',(31.3366367885136,584.251629149287,-49.4037303262696)) ;
#51210=CARTESIAN_POINT('Ctrl Pts',(31.3781421201879,584.294032697368,-49.4007260188503)) ;
#51211=CARTESIAN_POINT('Ctrl Pts',(31.4872332340532,584.415591058406,-49.3926218442998)) ;
#51212=CARTESIAN_POINT('Ctrl Pts',(31.5507321885579,584.498172831176,-49.3876553770832)) ;
#51213=CARTESIAN_POINT('Ctrl Pts',(31.6648373497383,584.672488688262,-49.3775365661717)) ;
#51214=CARTESIAN_POINT('Ctrl Pts',(31.7152352371349,584.763984231751,-49.3723964178044)) ;
#51215=CARTESIAN_POINT('Ctrl Pts',(31.7802896740693,584.906820069323,-49.3642967745992)) ;
#51216=CARTESIAN_POINT('Ctrl Pts',(31.8002618798508,584.955554371325,-49.361522981914)) ;
#51217=CARTESIAN_POINT('Ctrl Pts',(31.8364526279581,585.054540627552,-49.3558401155416)) ;
#51218=CARTESIAN_POINT('Ctrl Pts',(31.8526499290609,585.10475755557,-49.3529329405142)) ;
#51219=CARTESIAN_POINT('Ctrl Pts',(31.9001636109969,585.274118188881,-49.3430319257071)) ;
#51220=CARTESIAN_POINT('Ctrl Pts',(31.9226980651836,585.395432614009,-49.3357653093595)) ;
#51221=CARTESIAN_POINT('Ctrl Pts',(31.9403021513818,585.582466556225,-49.324508207457)) ;
#51222=CARTESIAN_POINT('Ctrl Pts',(31.943319230883,585.64716575147,-49.3206092009813)) ;
#51223=CARTESIAN_POINT('Ctrl Pts',(31.9432771921379,585.711899534809,-49.3167515585946)) ;
#51224=CARTESIAN_POINT('Ctrl Pts',(31.9432771921379,585.711899534809,-49.3167515585946)) ;
#51225=CARTESIAN_POINT('Ctrl Pts',(31.9432348751065,585.777061840039,-49.3128683795542)) ;
#51226=CARTESIAN_POINT('Ctrl Pts',(31.9400934612341,585.842180325114,-49.3090321149406)) ;
#51227=CARTESIAN_POINT('Ctrl Pts',(31.9306699451326,585.940273858617,-49.3034191596782)) ;
#51228=CARTESIAN_POINT('Ctrl Pts',(31.9266694830996,585.973413788179,-49.3015520048186)) ;
#51229=CARTESIAN_POINT('Ctrl Pts',(31.9172136969372,586.03839582843,-49.2979677778171)) ;
#51230=CARTESIAN_POINT('Ctrl Pts',(31.91181152813,586.07023519843,-49.2962493140222)) ;
#51231=CARTESIAN_POINT('Ctrl Pts',(31.8748589370945,586.260689961285,-49.286127665874)) ;
#51232=CARTESIAN_POINT('Ctrl Pts',(31.8254194120802,586.415272833367,-49.2785375829958)) ;
#51233=CARTESIAN_POINT('Ctrl Pts',(31.7288202952011,586.627295713425,-49.2672078164776)) ;
#51234=CARTESIAN_POINT('Ctrl Pts',(31.6959363401496,586.690537026551,-49.2637043358643)) ;
#51235=CARTESIAN_POINT('Ctrl Pts',(31.6291816385339,586.804082274015,-49.257044942509)) ;
#51236=CARTESIAN_POINT('Ctrl Pts',(31.5962416654096,586.85484130385,-49.2539200585485)) ;
#51237=CARTESIAN_POINT('Ctrl Pts',(31.5322057216826,586.944581623722,-49.2480677964579)) ;
#51238=CARTESIAN_POINT('Ctrl Pts',(31.5018382578407,586.984025999526,-49.2453703059187)) ;
#51239=CARTESIAN_POINT('Ctrl Pts',(31.4244182089832,587.077368510806,-49.2386557729236)) ;
#51240=CARTESIAN_POINT('Ctrl Pts',(31.3759279939045,587.12998394573,-49.2345805764577)) ;
#51241=CARTESIAN_POINT('Ctrl Pts',(31.2220061019296,587.280435885778,-49.2220304549604)) ;
#51242=CARTESIAN_POINT('Ctrl Pts',(31.108958555868,587.369842396659,-49.213274993064)) ;
#51243=CARTESIAN_POINT('Ctrl Pts',(30.9298807886466,587.483200319502,-49.2006428123861)) ;
#51244=CARTESIAN_POINT('Ctrl Pts',(30.8704503577371,587.51679912355,-49.1966338336946)) ;
#51245=CARTESIAN_POINT('Ctrl Pts',(30.7818980334419,587.561196694896,-49.1910304785662)) ;
#51246=CARTESIAN_POINT('Ctrl Pts',(30.7540320136384,587.574391960404,-49.1893183707379)) ;
#51247=CARTESIAN_POINT('Ctrl Pts',(30.6938494436853,587.601248715634,-49.1857441530688)) ;
#51248=CARTESIAN_POINT('Ctrl Pts',(30.6614599368688,587.614719435174,-49.1838922022212)) ;
#51249=CARTESIAN_POINT('Ctrl Pts',(30.5010704301565,587.676657465136,-49.1749954499452)) ;
#51250=CARTESIAN_POINT('Ctrl Pts',(30.3687817933728,587.713086423931,-49.1684820778909)) ;
#51251=CARTESIAN_POINT('Ctrl Pts',(30.1208877559366,587.755347753783,-49.1562934538899)) ;
#51252=CARTESIAN_POINT('Ctrl Pts',(30.0065283230978,587.765120962132,-49.1506760898893)) ;
#51253=CARTESIAN_POINT('Ctrl Pts',(29.8391519457605,587.765400484348,-49.1420354531627)) ;
#51254=CARTESIAN_POINT('Ctrl Pts',(29.7863647142763,587.76345293798,-49.1392521210079)) ;
#51255=CARTESIAN_POINT('Ctrl Pts',(29.6805672758382,587.755458985498,-49.1335273754377)) ;
#51256=CARTESIAN_POINT('Ctrl Pts',(29.6276009230757,587.749377257029,-49.1305869222901)) ;
#51257=CARTESIAN_POINT('Ctrl Pts',(29.4523709481474,587.722316853398,-49.1205932892199)) ;
#51258=CARTESIAN_POINT('Ctrl Pts',(29.3317892717943,587.692335160207,-49.1132622141688)) ;
#51259=CARTESIAN_POINT('Ctrl Pts',(29.1027772765574,587.612832383946,-49.0987110132526)) ;
#51260=CARTESIAN_POINT('Ctrl Pts',(28.9944563572668,587.564389142153,-49.091532428306)) ;
#51261=CARTESIAN_POINT('Ctrl Pts',(28.8578944241586,587.488546846559,-49.0825276131734)) ;
#51262=CARTESIAN_POINT('Ctrl Pts',(28.8253896238524,587.469303816088,-49.0803892924135)) ;
#51263=CARTESIAN_POINT('Ctrl Pts',(28.7683979620093,587.433406537484,-49.0766745880042)) ;
#51264=CARTESIAN_POINT('Ctrl Pts',(28.7437085161875,587.417100282464,-49.0750797082498)) ;
#51265=CARTESIAN_POINT('Ctrl Pts',(28.6724653421315,587.367805219593,-49.0705010853089)) ;
#51266=CARTESIAN_POINT('Ctrl Pts',(28.6269205256296,587.333402382128,-49.0676013084715)) ;
#51267=CARTESIAN_POINT('Ctrl Pts',(28.4764516346427,587.20957518737,-49.0579018197985)) ;
#51268=CARTESIAN_POINT('Ctrl Pts',(28.3791168681472,587.111519152382,-49.051394557796)) ;
#51269=CARTESIAN_POINT('Ctrl Pts',(28.250033603472,586.952276155568,-49.0413120464771)) ;
#51270=CARTESIAN_POINT('Ctrl Pts',(28.2103249863393,586.898059918791,-49.0379547049008)) ;
#51271=CARTESIAN_POINT('Ctrl Pts',(28.1435333773355,586.796808043188,-49.0317195456947)) ;
#51272=CARTESIAN_POINT('Ctrl Pts',(28.1155222290976,586.750459228287,-49.0288778747164)) ;
#51273=CARTESIAN_POINT('Ctrl Pts',(28.0641614017278,586.657354613131,-49.0231607390919)) ;
#51274=CARTESIAN_POINT('Ctrl Pts',(28.0407002835535,586.610707256361,-49.0202922820085)) ;
#51275=CARTESIAN_POINT('Ctrl Pts',(27.942410589137,586.395202517148,-49.0069960877451)) ;
#51276=CARTESIAN_POINT('Ctrl Pts',(27.8887905528058,586.217642569628,-48.9958166242235)) ;
#51277=CARTESIAN_POINT('Ctrl Pts',(27.8470966723024,585.957190937153,-48.9800230846765)) ;
#51278=CARTESIAN_POINT('Ctrl Pts',(27.8391099652609,585.878356639662,-48.9753360542625)) ;
#51279=CARTESIAN_POINT('Ctrl Pts',(27.8343230697207,585.767554791414,-48.9690418959603)) ;
#51280=CARTESIAN_POINT('Ctrl Pts',(27.8336878743545,585.73582680545,-48.9672735116628)) ;
#51281=CARTESIAN_POINT('Ctrl Pts',(27.8338943420504,585.670270209594,-48.963707112722)) ;
#51282=CARTESIAN_POINT('Ctrl Pts',(27.8348360297956,585.636452145458,-48.9619142450768)) ;
#51283=CARTESIAN_POINT('Ctrl Pts',(27.8418201985542,585.503628712772,-48.9550041610073)) ;
#51284=CARTESIAN_POINT('Ctrl Pts',(27.8541891817581,585.405148119242,-48.9501645139598)) ;
#51285=CARTESIAN_POINT('Ctrl Pts',(27.8735990520585,585.307997890694,-48.9453612460011)) ;
#51286=CARTESIAN_POINT('Origin',(29.8885276254068,535.710565160562,-51.0680854522906)) ;
#51287=CARTESIAN_POINT('',(28.6364363648369,537.33975668942,-47.7296625859471)) ;
#51288=CARTESIAN_POINT('',(28.6364362717721,537.339756617897,-47.6715263025693)) ;
#51289=CARTESIAN_POINT('',(28.6364362890686,537.33975663119,-51.0680854522906)) ;
#51290=CARTESIAN_POINT('',(28.0059001157431,534.887332980459,-47.5221601717529)) ;
#51291=CARTESIAN_POINT('Ctrl Pts',(28.6364362717721,537.339756617897,-47.6715263025693)) ;
#51292=CARTESIAN_POINT('Ctrl Pts',(28.6229519010584,537.329393401282,-47.6705367994022)) ;
#51293=CARTESIAN_POINT('Ctrl Pts',(28.6095949668397,537.318861834874,-47.6695424325092)) ;
#51294=CARTESIAN_POINT('Ctrl Pts',(28.4906899310523,537.22268988732,-47.6605649924041)) ;
#51295=CARTESIAN_POINT('Ctrl Pts',(28.3937593383079,537.126946666423,-47.6523161876422)) ;
#51296=CARTESIAN_POINT('Ctrl Pts',(28.2733592557547,536.981786770602,-47.6412515673653)) ;
#51297=CARTESIAN_POINT('Ctrl Pts',(28.2412941831759,536.939953656133,-47.6382097796865)) ;
#51298=CARTESIAN_POINT('Ctrl Pts',(28.1936375284346,536.872561707023,-47.6335914716711)) ;
#51299=CARTESIAN_POINT('Ctrl Pts',(28.1769368227079,536.847818738453,-47.6319533520939)) ;
#51300=CARTESIAN_POINT('Ctrl Pts',(28.1385328243379,536.788157366576,-47.6281454212355)) ;
#51301=CARTESIAN_POINT('Ctrl Pts',(28.1173274645108,536.752936125062,-47.6260044508062)) ;
#51302=CARTESIAN_POINT('Ctrl Pts',(28.043699593253,536.621900176307,-47.6183401545964)) ;
#51303=CARTESIAN_POINT('Ctrl Pts',(27.9978773581579,536.522579550768,-47.6130954377196)) ;
#51304=CARTESIAN_POINT('Ctrl Pts',(27.914113775103,536.294922003483,-47.601417465512)) ;
#51305=CARTESIAN_POINT('Ctrl Pts',(27.8803609476191,536.165588216216,-47.5949920208164)) ;
#51306=CARTESIAN_POINT('Ctrl Pts',(27.8500194767232,535.975175062434,-47.5851524228382)) ;
#51307=CARTESIAN_POINT('Ctrl Pts',(27.8432162098397,535.916074775029,-47.5820513032532)) ;
#51308=CARTESIAN_POINT('Ctrl Pts',(27.8350054810978,535.800971259178,-47.5758826170011)) ;
#51309=CARTESIAN_POINT('Ctrl Pts',(27.8333057220121,535.745041214447,-47.5728266951823)) ;
#51310=CARTESIAN_POINT('Ctrl Pts',(27.8352084047887,535.562791639009,-47.5626630893591)) ;
#51311=CARTESIAN_POINT('Ctrl Pts',(27.8481740452597,535.436873093049,-47.5553003425646)) ;
#51312=CARTESIAN_POINT('Ctrl Pts',(27.8934226483909,535.20745811273,-47.5415298922178)) ;
#51313=CARTESIAN_POINT('Ctrl Pts',(27.9224812278494,535.103750171493,-47.5351707299196)) ;
#51314=CARTESIAN_POINT('Ctrl Pts',(27.9674385603888,534.981221504937,-47.5277695608863)) ;
#51315=CARTESIAN_POINT('Ctrl Pts',(27.9757135688146,534.95978701585,-47.5264795198703)) ;
#51316=CARTESIAN_POINT('Ctrl Pts',(27.9913001477852,534.921345339113,-47.5241793117858)) ;
#51317=CARTESIAN_POINT('Ctrl Pts',(27.9984852948278,534.904289734789,-47.5231636235137)) ;
#51318=CARTESIAN_POINT('Ctrl Pts',(28.0059001157432,534.887332980459,-47.522160171753)) ;
#51319=CARTESIAN_POINT('',(28.6659533919829,534.056441033381,-47.5234100306407)) ;
#51320=CARTESIAN_POINT('Origin',(29.8885276254069,535.710565160562,-47.522160171753)) ;
#51321=CARTESIAN_POINT('Ctrl Pts',(28.6670126483642,534.058324644366,-47.5246598895284)) ;
#51322=CARTESIAN_POINT('Ctrl Pts',(28.6536810751985,534.068180785848,-47.5255549008763)) ;
#51323=CARTESIAN_POINT('Ctrl Pts',(28.640468807915,534.07819827049,-47.5264390170894)) ;
#51324=CARTESIAN_POINT('Ctrl Pts',(28.6099842628224,534.101898048799,-47.5284758797812)) ;
#51325=CARTESIAN_POINT('Ctrl Pts',(28.5928077462511,534.115700567163,-47.5296212187846)) ;
#51326=CARTESIAN_POINT('Ctrl Pts',(28.4802750207493,534.209146697694,-47.5371339803449)) ;
#51327=CARTESIAN_POINT('Ctrl Pts',(28.3920809257021,534.297028599388,-47.5430782761334)) ;
#51328=CARTESIAN_POINT('Ctrl Pts',(28.2370086491919,534.482445296616,-47.5547981044329)) ;
#51329=CARTESIAN_POINT('Ctrl Pts',(28.1695245285968,534.578832731799,-47.5605465545282)) ;
#51330=CARTESIAN_POINT('Ctrl Pts',(28.0840728699006,534.72631397182,-47.5693391362522)) ;
#51331=CARTESIAN_POINT('Ctrl Pts',(28.0592849438008,534.773186954468,-47.5721304322513)) ;
#51332=CARTESIAN_POINT('Ctrl Pts',(28.0134445313532,534.868628663493,-47.5778373464681)) ;
#51333=CARTESIAN_POINT('Ctrl Pts',(27.9924011151873,534.917156561869,-47.5807504812757)) ;
#51334=CARTESIAN_POINT('Ctrl Pts',(27.9334882784982,535.068789752369,-47.5899032425551)) ;
#51335=CARTESIAN_POINT('Ctrl Pts',(27.9019958013547,535.174150679075,-47.5963435171337)) ;
#51336=CARTESIAN_POINT('Ctrl Pts',(27.8589907377098,535.375562679116,-47.6086396102651)) ;
#51337=CARTESIAN_POINT('Ctrl Pts',(27.8455367596986,535.47090865252,-47.6144504973346)) ;
#51338=CARTESIAN_POINT('Ctrl Pts',(27.8359039934508,535.608291488259,-47.6225776598932)) ;
#51339=CARTESIAN_POINT('Ctrl Pts',(27.834255557408,535.649817193532,-47.6250012461652)) ;
#51340=CARTESIAN_POINT('Ctrl Pts',(27.8335450457281,535.725856249888,-47.6293469310298)) ;
#51341=CARTESIAN_POINT('Ctrl Pts',(27.8340912333028,535.760351154407,-47.631283574115)) ;
#51342=CARTESIAN_POINT('Ctrl Pts',(27.8367782705162,535.825827155142,-47.6348727041961)) ;
#51343=CARTESIAN_POINT('Ctrl Pts',(27.8387532182284,535.8568036467,-47.6365319357389)) ;
#51344=CARTESIAN_POINT('Ctrl Pts',(27.8476334616252,535.959416044123,-47.6419314961922)) ;
#51345=CARTESIAN_POINT('Ctrl Pts',(27.8576001589336,536.0307388095,-47.6455294958112)) ;
#51346=CARTESIAN_POINT('Ctrl Pts',(27.9027819236631,536.263939819916,-47.6571878545444)) ;
#51347=CARTESIAN_POINT('Ctrl Pts',(27.953801714464,536.422075056185,-47.6649737327569)) ;
#51348=CARTESIAN_POINT('Ctrl Pts',(28.048524016192,536.6270894273,-47.6764039246535)) ;
#51349=CARTESIAN_POINT('Ctrl Pts',(28.0761957010942,536.680659016126,-47.6795203056941)) ;
#51350=CARTESIAN_POINT('Ctrl Pts',(28.1309358672665,536.776090513973,-47.6853633150728)) ;
#51351=CARTESIAN_POINT('Ctrl Pts',(28.1572495080626,536.818332529484,-47.6880608936032)) ;
#51352=CARTESIAN_POINT('Ctrl Pts',(28.2252830102685,536.919195210623,-47.6947972782927)) ;
#51353=CARTESIAN_POINT('Ctrl Pts',(28.2685956302042,536.976656720144,-47.6988948491933)) ;
#51354=CARTESIAN_POINT('Ctrl Pts',(28.4105620069439,537.145759982907,-47.7117623876639)) ;
#51355=CARTESIAN_POINT('Ctrl Pts',(28.5183981870897,537.249040178714,-47.7208335961535)) ;
#51356=CARTESIAN_POINT('Ctrl Pts',(28.6364363648367,537.33975668942,-47.7296625859469)) ;
#51357=CARTESIAN_POINT('Origin',(29.8885276254068,535.710565160562,-51.0680854522906)) ;
#51358=CARTESIAN_POINT('',(28.6364362890749,537.339756631195,-48.4293659750649)) ;
#51359=CARTESIAN_POINT('',(28.6364362059859,537.339756567338,-48.3712578505663)) ;
#51360=CARTESIAN_POINT('',(28.6364362890686,537.33975663119,-51.0680854522906)) ;
#51361=CARTESIAN_POINT('',(31.9432771143099,535.709988359856,-47.9195437309321)) ;
#51362=CARTESIAN_POINT('Ctrl Pts',(28.6364362059859,537.339756567338,-48.3712578505663)) ;
#51363=CARTESIAN_POINT('Ctrl Pts',(28.6109373565783,537.320159796562,-48.3696379689333)) ;
#51364=CARTESIAN_POINT('Ctrl Pts',(28.5858931562955,537.299960229751,-48.3679995024793)) ;
#51365=CARTESIAN_POINT('Ctrl Pts',(28.5209233590622,537.244989154561,-48.3636076747014)) ;
#51366=CARTESIAN_POINT('Ctrl Pts',(28.4818601041241,537.209259333955,-48.3608192591648)) ;
#51367=CARTESIAN_POINT('Ctrl Pts',(28.4064121405063,537.134698907347,-48.3550976484189)) ;
#51368=CARTESIAN_POINT('Ctrl Pts',(28.370069686407,537.095883888854,-48.3521660506704)) ;
#51369=CARTESIAN_POINT('Ctrl Pts',(28.2294668051104,536.933527814266,-48.3400650873756)) ;
#51370=CARTESIAN_POINT('Ctrl Pts',(28.1384583225618,536.799308462096,-48.3303582116747)) ;
#51371=CARTESIAN_POINT('Ctrl Pts',(28.0340965091599,536.597888948285,-48.3167281960818)) ;
#51372=CARTESIAN_POINT('Ctrl Pts',(28.0068447712792,536.538531741233,-48.3128227017384)) ;
#51373=CARTESIAN_POINT('Ctrl Pts',(27.9652482588921,536.435215982338,-48.3063124780048)) ;
#51374=CARTESIAN_POINT('Ctrl Pts',(27.9494749449593,536.391885701308,-48.3036649114146)) ;
#51375=CARTESIAN_POINT('Ctrl Pts',(27.9261319140714,536.32035984946,-48.2994690889924)) ;
#51376=CARTESIAN_POINT('Ctrl Pts',(27.9176826683432,536.292473133652,-48.297877310712)) ;
#51377=CARTESIAN_POINT('Ctrl Pts',(27.897985545229,536.222102142919,-48.2939698362875)) ;
#51378=CARTESIAN_POINT('Ctrl Pts',(27.8875022599321,536.179421104986,-48.2916936989802)) ;
#51379=CARTESIAN_POINT('Ctrl Pts',(27.8488082412559,535.99678238639,-48.2822248553158)) ;
#51380=CARTESIAN_POINT('Ctrl Pts',(27.8338529795646,535.854418611201,-48.2754888178683)) ;
#51381=CARTESIAN_POINT('Ctrl Pts',(27.8337277627725,535.616273478408,-48.2638635308259)) ;
#51382=CARTESIAN_POINT('Ctrl Pts',(27.8403176878507,535.521021106146,-48.2591232807637)) ;
#51383=CARTESIAN_POINT('Ctrl Pts',(27.8606540207356,535.375292854597,-48.2514929143581)) ;
#51384=CARTESIAN_POINT('Ctrl Pts',(27.8697462887423,535.324300818853,-48.2487516402753)) ;
#51385=CARTESIAN_POINT('Ctrl Pts',(27.8924007465118,535.220181739395,-48.2429801555364)) ;
#51386=CARTESIAN_POINT('Ctrl Pts',(27.9061824106991,535.167145387741,-48.2399446718402)) ;
#51387=CARTESIAN_POINT('Ctrl Pts',(27.9415050553485,535.050569173866,-48.2330478030471)) ;
#51388=CARTESIAN_POINT('Ctrl Pts',(27.9640711615652,534.987407076322,-48.2291571791792)) ;
#51389=CARTESIAN_POINT('Ctrl Pts',(28.0448067054993,534.792139840619,-48.2166811149391)) ;
#51390=CARTESIAN_POINT('Ctrl Pts',(28.1138158620912,534.66499969055,-48.2078571390363)) ;
#51391=CARTESIAN_POINT('Ctrl Pts',(28.2243861453056,534.504241605859,-48.196381660404)) ;
#51392=CARTESIAN_POINT('Ctrl Pts',(28.2547511106737,534.463425038424,-48.1934408918052)) ;
#51393=CARTESIAN_POINT('Ctrl Pts',(28.3050630369977,534.400791710184,-48.1889367908077)) ;
#51394=CARTESIAN_POINT('Ctrl Pts',(28.3240176395631,534.378208054442,-48.1873158913631)) ;
#51395=CARTESIAN_POINT('Ctrl Pts',(28.3697977513185,534.325987975007,-48.1835821376272)) ;
#51396=CARTESIAN_POINT('Ctrl Pts',(28.397013332639,534.29671228002,-48.181495871264)) ;
#51397=CARTESIAN_POINT('Ctrl Pts',(28.5028096550975,534.189365137898,-48.1737896786604)) ;
#51398=CARTESIAN_POINT('Ctrl Pts',(28.5868088374752,534.116891445342,-48.1684616328046)) ;
#51399=CARTESIAN_POINT('Ctrl Pts',(28.7789323167666,533.976503336049,-48.156943450731)) ;
#51400=CARTESIAN_POINT('Ctrl Pts',(28.8883571196168,533.911168768337,-48.1507570506228)) ;
#51401=CARTESIAN_POINT('Ctrl Pts',(29.0511683329638,533.833422846335,-48.1414566686948)) ;
#51402=CARTESIAN_POINT('Ctrl Pts',(29.1000976247429,533.812352502543,-48.1386537063286)) ;
#51403=CARTESIAN_POINT('Ctrl Pts',(29.1991013448848,533.774207278837,-48.1329360761211)) ;
#51404=CARTESIAN_POINT('Ctrl Pts',(29.2491263254306,533.757118031754,-48.1300246034284)) ;
#51405=CARTESIAN_POINT('Ctrl Pts',(29.41057820935,533.708830106848,-48.120540071454)) ;
#51406=CARTESIAN_POINT('Ctrl Pts',(29.5239917132856,533.685105683524,-48.1137327182557)) ;
#51407=CARTESIAN_POINT('Ctrl Pts',(29.7727717963409,533.654642022534,-48.0987142656839)) ;
#51408=CARTESIAN_POINT('Ctrl Pts',(29.9080539638011,533.651477732356,-48.0904915867883)) ;
#51409=CARTESIAN_POINT('Ctrl Pts',(30.0778754093109,533.664253544935,-48.0807259281393)) ;
#51410=CARTESIAN_POINT('Ctrl Pts',(30.1130065495387,533.667808845587,-48.0787376010803)) ;
#51411=CARTESIAN_POINT('Ctrl Pts',(30.1784829863121,533.676144896028,-48.0751135142922)) ;
#51412=CARTESIAN_POINT('Ctrl Pts',(30.2088443519621,533.680703792574,-48.0734680958025)) ;
#51413=CARTESIAN_POINT('Ctrl Pts',(30.3049223018832,533.697339775831,-48.0683440146239)) ;
#51414=CARTESIAN_POINT('Ctrl Pts',(30.3701623005118,533.711943004209,-48.0649864858338)) ;
#51415=CARTESIAN_POINT('Ctrl Pts',(30.5659881420948,533.765925033592,-48.0549772917546)) ;
#51416=CARTESIAN_POINT('Ctrl Pts',(30.6934660938249,533.815135456908,-48.0485353932678)) ;
#51417=CARTESIAN_POINT('Ctrl Pts',(30.8834635381441,533.911131694173,-48.0380034610122)) ;
#51418=CARTESIAN_POINT('Ctrl Pts',(30.9498039733512,533.949443590365,-48.0341342628143)) ;
#51419=CARTESIAN_POINT('Ctrl Pts',(31.0557736414362,534.018807172911,-48.0275105421192)) ;
#51420=CARTESIAN_POINT('Ctrl Pts',(31.0966778689256,534.047772108312,-48.0248356681508)) ;
#51421=CARTESIAN_POINT('Ctrl Pts',(31.1827523776767,534.113576633226,-48.0189228758712)) ;
#51422=CARTESIAN_POINT('Ctrl Pts',(31.2274954869947,534.150900404863,-48.015666532343)) ;
#51423=CARTESIAN_POINT('Ctrl Pts',(31.3199694784192,534.234955234246,-48.0085243131655)) ;
#51424=CARTESIAN_POINT('Ctrl Pts',(31.3671293792817,534.282214335788,-48.0046196854311)) ;
#51425=CARTESIAN_POINT('Ctrl Pts',(31.5042084026115,534.433657704003,-47.9924851855872)) ;
#51426=CARTESIAN_POINT('Ctrl Pts',(31.5860366787711,534.544641150565,-47.9840709416786)) ;
#51427=CARTESIAN_POINT('Ctrl Pts',(31.6811007971023,534.705044609478,-47.9731237842977)) ;
#51428=CARTESIAN_POINT('Ctrl Pts',(31.704530820794,534.748004361622,-47.9703015186387)) ;
#51429=CARTESIAN_POINT('Ctrl Pts',(31.7395079098674,534.81796896631,-47.9659248578064)) ;
#51430=CARTESIAN_POINT('Ctrl Pts',(31.7520469900934,534.844452099457,-47.9643183313891)) ;
#51431=CARTESIAN_POINT('Ctrl Pts',(31.7812462894337,534.909695373233,-47.9604830276036)) ;
#51432=CARTESIAN_POINT('Ctrl Pts',(31.7972869857427,534.948715727084,-47.9582877085315)) ;
#51433=CARTESIAN_POINT('Ctrl Pts',(31.8319311008321,535.0409702687,-47.9532642090832)) ;
#51434=CARTESIAN_POINT('Ctrl Pts',(31.8495675686885,535.094531569758,-47.9504733186191)) ;
#51435=CARTESIAN_POINT('Ctrl Pts',(31.905219379795,535.290314283257,-47.9405093302048)) ;
#51436=CARTESIAN_POINT('Ctrl Pts',(31.9301326190769,535.435783171807,-47.9335159171135)) ;
#51437=CARTESIAN_POINT('Ctrl Pts',(31.9419369878692,535.625057469517,-47.9239369811701)) ;
#51438=CARTESIAN_POINT('Ctrl Pts',(31.9432655974392,535.667518055835,-47.9217603139583)) ;
#51439=CARTESIAN_POINT('Ctrl Pts',(31.9432775441096,535.709987153938,-47.919544539831)) ;
#51440=CARTESIAN_POINT('Ctrl Pts',(31.9432775444593,535.709988398555,-47.9195444748946)) ;
#51441=CARTESIAN_POINT('Ctrl Pts',(31.9432897614835,535.753512294332,-47.9172736671991)) ;
#51442=CARTESIAN_POINT('Ctrl Pts',(31.9419190958385,535.79702374984,-47.9149628739012)) ;
#51443=CARTESIAN_POINT('Ctrl Pts',(31.9358760518337,535.892426708692,-47.9097903438074)) ;
#51444=CARTESIAN_POINT('Ctrl Pts',(31.930610071471,535.944248248271,-47.9069113174683)) ;
#51445=CARTESIAN_POINT('Ctrl Pts',(31.9006628291596,536.157882650572,-47.894734617352)) ;
#51446=CARTESIAN_POINT('Ctrl Pts',(31.858664665141,536.316638422322,-47.8848850330862)) ;
#51447=CARTESIAN_POINT('Ctrl Pts',(31.7641216900513,536.554795412575,-47.8694839341399)) ;
#51448=CARTESIAN_POINT('Ctrl Pts',(31.7241586760957,536.638487194049,-47.8639549100924)) ;
#51449=CARTESIAN_POINT('Ctrl Pts',(31.6627136730293,536.747541295564,-47.8568315313557)) ;
#51450=CARTESIAN_POINT('Ctrl Pts',(31.6460742161577,536.775499891421,-47.855013526813)) ;
#51451=CARTESIAN_POINT('Ctrl Pts',(31.6109596809507,536.831434589283,-47.8514118218475)) ;
#51452=CARTESIAN_POINT('Ctrl Pts',(31.5924501733249,536.859377025864,-47.8496305838173)) ;
#51453=CARTESIAN_POINT('Ctrl Pts',(31.4990206132572,536.99319105263,-47.8411255546595)) ;
#51454=CARTESIAN_POINT('Ctrl Pts',(31.4148682444253,537.092270037291,-47.8348933711343)) ;
#51455=CARTESIAN_POINT('Ctrl Pts',(31.2359450420417,537.26647824529,-47.8227593885476)) ;
#51456=CARTESIAN_POINT('Ctrl Pts',(31.1427982617474,537.342496847014,-47.8168876740319)) ;
#51457=CARTESIAN_POINT('Ctrl Pts',(30.9991748428906,537.44011428871,-47.8079246422935)) ;
#51458=CARTESIAN_POINT('Ctrl Pts',(30.9536300446027,537.468528062422,-47.8050970577741)) ;
#51459=CARTESIAN_POINT('Ctrl Pts',(30.8605190212433,537.521669230653,-47.7993132744161)) ;
#51460=CARTESIAN_POINT('Ctrl Pts',(30.8129937074386,537.546382942972,-47.7963596086639)) ;
#51461=CARTESIAN_POINT('Ctrl Pts',(30.6626442170341,537.617246945069,-47.7869931032003)) ;
#51462=CARTESIAN_POINT('Ctrl Pts',(30.5569627822929,537.656812971335,-47.7803653748098)) ;
#51463=CARTESIAN_POINT('Ctrl Pts',(30.3562777350725,537.713665690896,-47.7678730689376)) ;
#51464=CARTESIAN_POINT('Ctrl Pts',(30.2622527716955,537.733318666073,-47.7620602555263)) ;
#51465=CARTESIAN_POINT('Ctrl Pts',(30.1107729669971,537.754054344038,-47.7530165131444)) ;
#51466=CARTESIAN_POINT('Ctrl Pts',(30.05404613902,537.759429651115,-47.7497018429617)) ;
#51467=CARTESIAN_POINT('Ctrl Pts',(29.9677666229353,537.763997759885,-47.744839498185)) ;
#51468=CARTESIAN_POINT('Ctrl Pts',(29.9383351986624,537.764922437003,-47.7432125918351)) ;
#51469=CARTESIAN_POINT('Ctrl Pts',(29.8744250774901,537.765555839649,-47.7397629580682)) ;
#51470=CARTESIAN_POINT('Ctrl Pts',(29.839953758065,537.765030169449,-47.7379531173712)) ;
#51471=CARTESIAN_POINT('Ctrl Pts',(29.6927721689412,537.759078744344,-47.7303812126777)) ;
#51472=CARTESIAN_POINT('Ctrl Pts',(29.5805894497075,537.74524140175,-47.724993027963)) ;
#51473=CARTESIAN_POINT('Ctrl Pts',(29.3347550937227,537.694108620168,-47.7130131154768)) ;
#51474=CARTESIAN_POINT('Ctrl Pts',(29.2026079582314,537.652373390694,-47.7064367229642)) ;
#51475=CARTESIAN_POINT('Ctrl Pts',(29.0246296991013,537.575709820794,-47.6965920527537)) ;
#51476=CARTESIAN_POINT('Ctrl Pts',(28.9745204955043,537.551672004371,-47.6937062239928)) ;
#51477=CARTESIAN_POINT('Ctrl Pts',(28.8814101810037,537.502267568968,-47.6880896084753)) ;
#51478=CARTESIAN_POINT('Ctrl Pts',(28.8382389188391,537.477306815434,-47.6853753235415)) ;
#51479=CARTESIAN_POINT('Ctrl Pts',(28.7410910438642,537.416318150144,-47.6789977661128)) ;
#51480=CARTESIAN_POINT('Ctrl Pts',(28.6878377483695,537.379260473703,-47.6752982193288)) ;
#51481=CARTESIAN_POINT('Ctrl Pts',(28.6364362717721,537.339756617897,-47.6715263025693)) ;
#51482=CARTESIAN_POINT('Ctrl Pts',(28.6364363648367,537.33975668942,-47.7296625859469)) ;
#51483=CARTESIAN_POINT('Ctrl Pts',(28.6660459719102,537.362512718769,-47.7318773178551)) ;
#51484=CARTESIAN_POINT('Ctrl Pts',(28.6962636054984,537.384452512989,-47.734071696501)) ;
#51485=CARTESIAN_POINT('Ctrl Pts',(28.7490501031617,537.420623168944,-47.7377734537237)) ;
#51486=CARTESIAN_POINT('Ctrl Pts',(28.7713202615108,537.435255059537,-47.7392968165599)) ;
#51487=CARTESIAN_POINT('Ctrl Pts',(28.8165336432896,537.463717658096,-47.7423038814074)) ;
#51488=CARTESIAN_POINT('Ctrl Pts',(28.8394763173039,537.477541783534,-47.7437870181451)) ;
#51489=CARTESIAN_POINT('Ctrl Pts',(28.8925447807788,537.508119992424,-47.747109858126)) ;
#51490=CARTESIAN_POINT('Ctrl Pts',(28.9228347712996,537.52457255355,-47.7489307975608)) ;
#51491=CARTESIAN_POINT('Ctrl Pts',(29.0795026035766,537.604632314948,-47.7580411470102)) ;
#51492=CARTESIAN_POINT('Ctrl Pts',(29.2118042502731,537.65583276028,-47.7647513513814)) ;
#51493=CARTESIAN_POINT('Ctrl Pts',(29.4230576751126,537.713396723879,-47.7753602418018)) ;
#51494=CARTESIAN_POINT('Ctrl Pts',(29.4988744684411,537.72951686742,-47.7791437532152)) ;
#51495=CARTESIAN_POINT('Ctrl Pts',(29.6380035302706,537.750968418156,-47.7862229273434)) ;
#51496=CARTESIAN_POINT('Ctrl Pts',(29.700998013372,537.757719131493,-47.7894772513634)) ;
#51497=CARTESIAN_POINT('Ctrl Pts',(29.8133813905988,537.764531640296,-47.7954297810772)) ;
#51498=CARTESIAN_POINT('Ctrl Pts',(29.8626506906498,537.765742781107,-47.7980888454819)) ;
#51499=CARTESIAN_POINT('Ctrl Pts',(29.978040418492,537.764429421712,-47.8044504349252)) ;
#51500=CARTESIAN_POINT('Ctrl Pts',(30.0440867152625,537.760484893908,-47.8081956368863)) ;
#51501=CARTESIAN_POINT('Ctrl Pts',(30.2561079644868,537.737516726513,-47.8205492276318)) ;
#51502=CARTESIAN_POINT('Ctrl Pts',(30.4002582688995,537.706002848547,-47.8294934326989)) ;
#51503=CARTESIAN_POINT('Ctrl Pts',(30.6097949661098,537.635979283451,-47.8426982223909)) ;
#51504=CARTESIAN_POINT('Ctrl Pts',(30.6784982833515,537.608826028134,-47.8470542292525)) ;
#51505=CARTESIAN_POINT('Ctrl Pts',(30.7739258916887,537.565029800985,-47.8530060354114)) ;
#51506=CARTESIAN_POINT('Ctrl Pts',(30.8019589495922,537.551383673851,-47.8547414012516)) ;
#51507=CARTESIAN_POINT('Ctrl Pts',(30.8597879536473,537.521586582734,-47.8582773697266)) ;
#51508=CARTESIAN_POINT('Ctrl Pts',(30.8895160489951,537.505326339535,-47.860071504798)) ;
#51509=CARTESIAN_POINT('Ctrl Pts',(31.0443915833832,537.41556867621,-47.8693635898957)) ;
#51510=CARTESIAN_POINT('Ctrl Pts',(31.161904253365,537.329694517413,-47.8762430399588)) ;
#51511=CARTESIAN_POINT('Ctrl Pts',(31.3506788637338,537.158377277678,-47.88861378739)) ;
#51512=CARTESIAN_POINT('Ctrl Pts',(31.4259151389213,537.078221051206,-47.89401157208)) ;
#51513=CARTESIAN_POINT('Ctrl Pts',(31.5270596417343,536.951513786517,-47.9023868249005)) ;
#51514=CARTESIAN_POINT('Ctrl Pts',(31.5581549586403,536.909349780766,-47.9051488721096)) ;
#51515=CARTESIAN_POINT('Ctrl Pts',(31.6174540091543,536.822153538575,-47.9108405047916)) ;
#51516=CARTESIAN_POINT('Ctrl Pts',(31.6455896826167,536.77712380655,-47.9137696934752)) ;
#51517=CARTESIAN_POINT('Ctrl Pts',(31.732414537059,536.625388029269,-47.9236245451744)) ;
#51518=CARTESIAN_POINT('Ctrl Pts',(31.7833610427512,536.514566987941,-47.9308155449626)) ;
#51519=CARTESIAN_POINT('Ctrl Pts',(31.8617261896303,536.294517151395,-47.9448317156167)) ;
#51520=CARTESIAN_POINT('Ctrl Pts',(31.8905889544197,536.186238106078,-47.9516112696373)) ;
#51521=CARTESIAN_POINT('Ctrl Pts',(31.9179322861602,536.035006209979,-47.9605385585402)) ;
#51522=CARTESIAN_POINT('Ctrl Pts',(31.9241136350263,535.993647084515,-47.962924360334)) ;
#51523=CARTESIAN_POINT('Ctrl Pts',(31.9324460946066,535.92326133233,-47.966858419421)) ;
#51524=CARTESIAN_POINT('Ctrl Pts',(31.9352500514238,535.89433081867,-47.9684373779893)) ;
#51525=CARTESIAN_POINT('Ctrl Pts',(31.9410632027104,535.817378948874,-47.9725442344738)) ;
#51526=CARTESIAN_POINT('Ctrl Pts',(31.9430014798801,535.7692963048,-47.975018867384)) ;
#51527=CARTESIAN_POINT('Ctrl Pts',(31.943980337516,535.579936201775,-47.984555301875)) ;
#51528=CARTESIAN_POINT('Ctrl Pts',(31.9301437139032,535.438979707353,-47.9912197198367)) ;
#51529=CARTESIAN_POINT('Ctrl Pts',(31.8838428720012,535.211613933217,-48.0025773169541)) ;
#51530=CARTESIAN_POINT('Ctrl Pts',(31.8598608655246,535.123983324473,-48.0071050777366)) ;
#51531=CARTESIAN_POINT('Ctrl Pts',(31.8134105482822,534.989839354403,-48.014478168151)) ;
#51532=CARTESIAN_POINT('Ctrl Pts',(31.7948523605926,534.942095689224,-48.0171929570401)) ;
#51533=CARTESIAN_POINT('Ctrl Pts',(31.7527450622742,534.844710425386,-48.0229461371169)) ;
#51534=CARTESIAN_POINT('Ctrl Pts',(31.7289499489372,534.795220458472,-48.0259915044107)) ;
#51535=CARTESIAN_POINT('Ctrl Pts',(31.6290810709249,534.607187704454,-48.0380596045783)) ;
#51536=CARTESIAN_POINT('Ctrl Pts',(31.539115539315,534.476663386456,-48.0475755529853)) ;
#51537=CARTESIAN_POINT('Ctrl Pts',(31.3936804647077,534.310396722979,-48.0608417533435)) ;
#51538=CARTESIAN_POINT('Ctrl Pts',(31.3500983344297,534.264961995106,-48.0646012090386)) ;
#51539=CARTESIAN_POINT('Ctrl Pts',(31.2718645101486,534.190563627827,-48.0709042393895)) ;
#51540=CARTESIAN_POINT('Ctrl Pts',(31.2382170198493,534.160608793194,-48.0734876321035)) ;
#51541=CARTESIAN_POINT('Ctrl Pts',(31.181369745335,534.113256602909,-48.0776103992252)) ;
#51542=CARTESIAN_POINT('Ctrl Pts',(31.1587417426899,534.095203995221,-48.0791904427315)) ;
#51543=CARTESIAN_POINT('Ctrl Pts',(31.1006465377737,534.050831799082,-48.0830971593247)) ;
#51544=CARTESIAN_POINT('Ctrl Pts',(31.0646999927773,534.025167222701,-48.0853831688788)) ;
#51545=CARTESIAN_POINT('Ctrl Pts',(30.9151257349926,533.925494760977,-48.0944941962105)) ;
#51546=CARTESIAN_POINT('Ctrl Pts',(30.7951276440468,533.861656871508,-48.1009140460509)) ;
#51547=CARTESIAN_POINT('Ctrl Pts',(30.5773987270047,533.772159928521,-48.1123812269167)) ;
#51548=CARTESIAN_POINT('Ctrl Pts',(30.4824549290364,533.740995184651,-48.1173244356803)) ;
#51549=CARTESIAN_POINT('Ctrl Pts',(30.3353562124117,533.704318336775,-48.1251747936067)) ;
#51550=CARTESIAN_POINT('Ctrl Pts',(30.2846301301824,533.693690285201,-48.1279135276775)) ;
#51551=CARTESIAN_POINT('Ctrl Pts',(30.180547010276,533.675960998018,-48.1336238953026)) ;
#51552=CARTESIAN_POINT('Ctrl Pts',(30.1272045696466,533.669016248177,-48.1365982345536)) ;
#51553=CARTESIAN_POINT('Ctrl Pts',(29.9051259251516,533.648925918834,-48.149198132912)) ;
#51554=CARTESIAN_POINT('Ctrl Pts',(29.735380185855,533.654559287559,-48.1594168093959)) ;
#51555=CARTESIAN_POINT('Ctrl Pts',(29.4845561586807,533.694135330239,-48.1746470997079)) ;
#51556=CARTESIAN_POINT('Ctrl Pts',(29.4017199246338,533.712515392963,-48.1796832363303)) ;
#51557=CARTESIAN_POINT('Ctrl Pts',(29.2895396983399,533.744800099161,-48.1863171665115)) ;
#51558=CARTESIAN_POINT('Ctrl Pts',(29.2590370330932,533.754354349092,-48.1881010093543)) ;
#51559=CARTESIAN_POINT('Ctrl Pts',(29.1975154126042,533.775212832741,-48.1916402352516)) ;
#51560=CARTESIAN_POINT('Ctrl Pts',(29.1665213127764,533.786560567338,-48.1933928627051)) ;
#51561=CARTESIAN_POINT('Ctrl Pts',(29.0101605586639,533.848119372036,-48.202142122044)) ;
#51562=CARTESIAN_POINT('Ctrl Pts',(28.8896773064733,533.909859961679,-48.2085926857946)) ;
#51563=CARTESIAN_POINT('Ctrl Pts',(28.6750745216497,534.04804561447,-48.2209552361665)) ;
#51564=CARTESIAN_POINT('Ctrl Pts',(28.579943276341,534.121841425235,-48.2268267184197)) ;
#51565=CARTESIAN_POINT('Ctrl Pts',(28.4531105372464,534.239388859163,-48.2357482155519)) ;
#51566=CARTESIAN_POINT('Ctrl Pts',(28.4158075464454,534.276732247989,-48.2385273902011)) ;
#51567=CARTESIAN_POINT('Ctrl Pts',(28.3442113023573,534.35415048482,-48.2442128033654)) ;
#51568=CARTESIAN_POINT('Ctrl Pts',(28.309941324366,534.394192021872,-48.2471167087464)) ;
#51569=CARTESIAN_POINT('Ctrl Pts',(28.174983697265,534.564736134942,-48.2593607093954)) ;
#51570=CARTESIAN_POINT('Ctrl Pts',(28.0886506241526,534.705785183858,-48.2692666928378)) ;
#51571=CARTESIAN_POINT('Ctrl Pts',(27.9934576786508,534.9138173918,-48.283009016606)) ;
#51572=CARTESIAN_POINT('Ctrl Pts',(27.9695507903834,534.973255351297,-48.2868371165224)) ;
#51573=CARTESIAN_POINT('Ctrl Pts',(27.933466461241,535.076684624439,-48.2932363467774)) ;
#51574=CARTESIAN_POINT('Ctrl Pts',(27.919905782499,535.120143827584,-48.2958487176514)) ;
#51575=CARTESIAN_POINT('Ctrl Pts',(27.9000978580295,535.191929603653,-48.3000003258659)) ;
#51576=CARTESIAN_POINT('Ctrl Pts',(27.8929878337704,535.219997167993,-48.3015816682146)) ;
#51577=CARTESIAN_POINT('Ctrl Pts',(27.8766337334246,535.29081255544,-48.3054676855118)) ;
#51578=CARTESIAN_POINT('Ctrl Pts',(27.8681568358877,535.3337207632,-48.3077330754487)) ;
#51579=CARTESIAN_POINT('Ctrl Pts',(27.839073549619,535.51042548027,-48.3168174950013)) ;
#51580=CARTESIAN_POINT('Ctrl Pts',(27.8303406821866,535.645835563483,-48.3232280107875)) ;
#51581=CARTESIAN_POINT('Ctrl Pts',(27.8384461539867,535.881720685387,-48.3347206892156)) ;
#51582=CARTESIAN_POINT('Ctrl Pts',(27.8492888562128,535.98191502232,-48.3397026946008)) ;
#51583=CARTESIAN_POINT('Ctrl Pts',(27.87677739035,536.13193167462,-48.3475983376188)) ;
#51584=CARTESIAN_POINT('Ctrl Pts',(27.888055826285,536.182582829214,-48.350339811795)) ;
#51585=CARTESIAN_POINT('Ctrl Pts',(27.9148894365981,536.284704012378,-48.3560492903768)) ;
#51586=CARTESIAN_POINT('Ctrl Pts',(27.9305719722151,536.336098541244,-48.3590196961411)) ;
#51587=CARTESIAN_POINT('Ctrl Pts',(28.0041409314059,536.547180239176,-48.3716475431238)) ;
#51588=CARTESIAN_POINT('Ctrl Pts',(28.0796920896114,536.699976212486,-48.3819036165961)) ;
#51589=CARTESIAN_POINT('Ctrl Pts',(28.2196062326397,536.912155696837,-48.3971448334858)) ;
#51590=CARTESIAN_POINT('Ctrl Pts',(28.2703602318251,536.979681034504,-48.402157057251)) ;
#51591=CARTESIAN_POINT('Ctrl Pts',(28.3458550789782,537.068202567596,-48.408767890696)) ;
#51592=CARTESIAN_POINT('Ctrl Pts',(28.3671485886185,537.092022388839,-48.4105507195528)) ;
#51593=CARTESIAN_POINT('Ctrl Pts',(28.4115793806403,537.139450430223,-48.4140910037266)) ;
#51594=CARTESIAN_POINT('Ctrl Pts',(28.434747921837,537.163016221716,-48.4158455698408)) ;
#51595=CARTESIAN_POINT('Ctrl Pts',(28.5148079957574,537.240612940701,-48.4216497193311)) ;
#51596=CARTESIAN_POINT('Ctrl Pts',(28.5742250409781,537.291945084075,-48.4255364649937)) ;
#51597=CARTESIAN_POINT('Ctrl Pts',(28.6364362890811,537.3397566312,-48.4293659750649)) ;
#51598=CARTESIAN_POINT('Origin',(29.8885276254068,535.710565160562,-51.0680854522906)) ;
#51599=CARTESIAN_POINT('',(28.6368808924516,537.339275726356,-49.1271194481244)) ;
#51600=CARTESIAN_POINT('',(28.6364362889498,537.339756631099,-49.0682055192064)) ;
#51601=CARTESIAN_POINT('',(28.6364362890686,537.33975663119,-51.0680854522906)) ;
#51602=CARTESIAN_POINT('',(31.943277537214,535.709963140231,-49.3762357707893)) ;
#51603=CARTESIAN_POINT('Ctrl Pts',(31.9427353807384,535.709924613476,-49.3752968619707)) ;
#51604=CARTESIAN_POINT('Ctrl Pts',(31.9426199546863,535.780830487742,-49.3712221291559)) ;
#51605=CARTESIAN_POINT('Ctrl Pts',(31.9388610049111,535.851778410132,-49.3672024739762)) ;
#51606=CARTESIAN_POINT('Ctrl Pts',(31.9314849812218,535.922371758857,-49.3632673200693)) ;
#51607=CARTESIAN_POINT('Ctrl Pts',(31.9241108995947,535.992946520782,-49.3593332022646)) ;
#51608=CARTESIAN_POINT('Ctrl Pts',(31.913121663627,536.063166873767,-49.3554835715093)) ;
#51609=CARTESIAN_POINT('Ctrl Pts',(31.8985781724063,536.132640674243,-49.3517232456352)) ;
#51610=CARTESIAN_POINT('Ctrl Pts',(31.8840335242281,536.202120001468,-49.3479626206213)) ;
#51611=CARTESIAN_POINT('Ctrl Pts',(31.865933961411,536.270852586537,-49.3442912423131)) ;
#51612=CARTESIAN_POINT('Ctrl Pts',(31.8443754859495,536.338451052282,-49.3406896571612)) ;
#51613=CARTESIAN_POINT('Ctrl Pts',(31.8227923040914,536.406126987072,-49.3370839445287)) ;
#51614=CARTESIAN_POINT('Ctrl Pts',(31.7977420713674,536.472666069719,-49.3335479997593)) ;
#51615=CARTESIAN_POINT('Ctrl Pts',(31.7693585376145,536.537685961532,-49.3300398756539)) ;
#51616=CARTESIAN_POINT('Ctrl Pts',(31.7409575727637,536.602745783825,-49.3265295971143)) ;
#51617=CARTESIAN_POINT('Ctrl Pts',(31.7092188973427,536.666284313147,-49.3230468284672)) ;
#51618=CARTESIAN_POINT('Ctrl Pts',(31.6743178484239,536.727927574273,-49.3195310381818)) ;
#51619=CARTESIAN_POINT('Ctrl Pts',(31.6414276231321,536.78601925945,-49.3162178101228)) ;
#51620=CARTESIAN_POINT('Ctrl Pts',(31.605728525571,536.842427954752,-49.3128747645005)) ;
#51621=CARTESIAN_POINT('Ctrl Pts',(31.5674065174128,536.896850717022,-49.3094413669133)) ;
#51622=CARTESIAN_POINT('Ctrl Pts',(31.5649871231534,536.900286604778,-49.3092246052452)) ;
#51623=CARTESIAN_POINT('Ctrl Pts',(31.5625572732845,536.903714594207,-49.3090074834512)) ;
#51624=CARTESIAN_POINT('Ctrl Pts',(31.5601170139572,536.907134616038,-49.3087899862986)) ;
#51625=CARTESIAN_POINT('Ctrl Pts',(31.5338502905483,536.943947411504,-49.3064488672681)) ;
#51626=CARTESIAN_POINT('Ctrl Pts',(31.5063786491928,536.97983508785,-49.3040640238)) ;
#51627=CARTESIAN_POINT('Ctrl Pts',(31.4777715977333,537.014707694267,-49.3016158100282)) ;
#51628=CARTESIAN_POINT('Ctrl Pts',(31.4777498830234,537.014734164962,-49.3016139516664)) ;
#51629=CARTESIAN_POINT('Ctrl Pts',(31.4777281676594,537.014760635073,-49.301612093268)) ;
#51630=CARTESIAN_POINT('Ctrl Pts',(31.4777064516412,537.014787104599,-49.3016102348332)) ;
#51631=CARTESIAN_POINT('Ctrl Pts',(31.4368869866815,537.064541709808,-49.2981169463691)) ;
#51632=CARTESIAN_POINT('Ctrl Pts',(31.3935987794868,537.112410718029,-49.294485333284)) ;
#51633=CARTESIAN_POINT('Ctrl Pts',(31.3480628704188,537.158164346995,-49.2907804710927)) ;
#51634=CARTESIAN_POINT('Ctrl Pts',(31.3434468252196,537.162802462795,-49.2904049035092)) ;
#51635=CARTESIAN_POINT('Ctrl Pts',(31.3388077255577,537.167418832085,-49.290028583204)) ;
#51636=CARTESIAN_POINT('Ctrl Pts',(31.3341458310762,537.172013210475,-49.2896515779672)) ;
#51637=CARTESIAN_POINT('Ctrl Pts',(31.2835734989649,537.221853126567,-49.2855618170084)) ;
#51638=CARTESIAN_POINT('Ctrl Pts',(31.2303129280193,537.269106762271,-49.2813920692415)) ;
#51639=CARTESIAN_POINT('Ctrl Pts',(31.1746835629705,537.313510240679,-49.2772166934141)) ;
#51640=CARTESIAN_POINT('Ctrl Pts',(31.1191229434999,537.357858846219,-49.2730464774268)) ;
#51641=CARTESIAN_POINT('Ctrl Pts',(31.0611995686604,537.399364666718,-49.2688710009134)) ;
#51642=CARTESIAN_POINT('Ctrl Pts',(31.0012491055257,537.437801073993,-49.2647450006894)) ;
#51643=CARTESIAN_POINT('Ctrl Pts',(30.9413387091166,537.476211793044,-49.2606217579973)) ;
#51644=CARTESIAN_POINT('Ctrl Pts',(30.8794039979015,537.511557362762,-49.2565480944349)) ;
#51645=CARTESIAN_POINT('Ctrl Pts',(30.815795572546,537.543644156167,-49.2525554549385)) ;
#51646=CARTESIAN_POINT('Ctrl Pts',(30.7522082799242,537.575720289322,-49.2485641419233)) ;
#51647=CARTESIAN_POINT('Ctrl Pts',(30.686948403443,537.604539826175,-49.2446538395684)) ;
#51648=CARTESIAN_POINT('Ctrl Pts',(30.6203812176618,537.629940570116,-49.2408312549402)) ;
#51649=CARTESIAN_POINT('Ctrl Pts',(30.5538137750593,537.655341412055,-49.2370086555642)) ;
#51650=CARTESIAN_POINT('Ctrl Pts',(30.4859390124216,537.677323325623,-49.2332737099885)) ;
#51651=CARTESIAN_POINT('Ctrl Pts',(30.4171371153688,537.695756075853,-49.2296085996251)) ;
#51652=CARTESIAN_POINT('Ctrl Pts',(30.3482663065826,537.71420728826,-49.2259398183002)) ;
#51653=CARTESIAN_POINT('Ctrl Pts',(30.2784664955002,537.729101984314,-49.222340833987)) ;
#51654=CARTESIAN_POINT('Ctrl Pts',(30.2081340439748,537.740344173802,-49.2187709892463)) ;
#51655=CARTESIAN_POINT('Ctrl Pts',(30.1377637201469,537.751592416934,-49.2151992222317)) ;
#51656=CARTESIAN_POINT('Ctrl Pts',(30.0668602002263,537.759183828206,-49.2116562888183)) ;
#51657=CARTESIAN_POINT('Ctrl Pts',(29.9958355179518,537.763061612476,-49.2080824899406)) ;
#51658=CARTESIAN_POINT('Ctrl Pts',(29.9285703348079,537.766734136743,-49.204697860424)) ;
#51659=CARTESIAN_POINT('Ctrl Pts',(29.8611961404133,537.76707549024,-49.2012850560164)) ;
#51660=CARTESIAN_POINT('Ctrl Pts',(29.7940761550714,537.764076262402,-49.1977828519104)) ;
#51661=CARTESIAN_POINT('Ctrl Pts',(29.7902028026375,537.763903183305,-49.1975807471166)) ;
#51662=CARTESIAN_POINT('Ctrl Pts',(29.7863302840043,537.763718986147,-49.1973783446039)) ;
#51663=CARTESIAN_POINT('Ctrl Pts',(29.7824586642199,537.763523671486,-49.1971756326062)) ;
#51664=CARTESIAN_POINT('Ctrl Pts',(29.7394170961748,537.761352319517,-49.1949220429648)) ;
#51665=CARTESIAN_POINT('Ctrl Pts',(29.6964886714984,537.757806947959,-49.1926299836999)) ;
#51666=CARTESIAN_POINT('Ctrl Pts',(29.6537708961817,537.752895156457,-49.1902826080212)) ;
#51667=CARTESIAN_POINT('Ctrl Pts',(29.6537386176986,537.752891445,-49.1902808342929)) ;
#51668=CARTESIAN_POINT('Ctrl Pts',(29.6537063393353,537.752887732763,-49.1902790605331)) ;
#51669=CARTESIAN_POINT('Ctrl Pts',(29.6536740610918,537.752884019747,-49.1902772867416)) ;
#51670=CARTESIAN_POINT('Ctrl Pts',(29.5893740015573,537.745487483915,-49.1867437953227)) ;
#51671=CARTESIAN_POINT('Ctrl Pts',(29.5253306330089,537.734962903227,-49.1830762567584)) ;
#51672=CARTESIAN_POINT('Ctrl Pts',(29.4618603629612,537.72137346018,-49.1793396131153)) ;
#51673=CARTESIAN_POINT('Ctrl Pts',(29.4556644772076,537.720046876309,-49.1789748467908)) ;
#51674=CARTESIAN_POINT('Ctrl Pts',(29.449474081227,537.718691115574,-49.1786094219356)) ;
#51675=CARTESIAN_POINT('Ctrl Pts',(29.4432894873336,537.717306256261,-49.178243398962)) ;
#51676=CARTESIAN_POINT('Ctrl Pts',(29.3742159037184,537.701839243031,-49.1741554153508)) ;
#51677=CARTESIAN_POINT('Ctrl Pts',(29.3058622453113,537.682738637951,-49.1699935618367)) ;
#51678=CARTESIAN_POINT('Ctrl Pts',(29.2386160666126,537.660129319953,-49.1658294303658)) ;
#51679=CARTESIAN_POINT('Ctrl Pts',(29.23504794841,537.658929657449,-49.1656084793231)) ;
#51680=CARTESIAN_POINT('Ctrl Pts',(29.2314829579231,537.65772012384,-49.165387521867)) ;
#51681=CARTESIAN_POINT('Ctrl Pts',(29.2279211562329,537.656500740354,-49.1651665686925)) ;
#51682=CARTESIAN_POINT('Ctrl Pts',(29.1605197194827,537.633425845665,-49.1609853809922)) ;
#51683=CARTESIAN_POINT('Ctrl Pts',(29.0942559948543,537.606821413716,-49.1568059334518)) ;
#51684=CARTESIAN_POINT('Ctrl Pts',(29.0295020143273,537.576849542796,-49.1526806630055)) ;
#51685=CARTESIAN_POINT('Ctrl Pts',(28.9647908786836,537.546897502956,-49.1485581220707)) ;
#51686=CARTESIAN_POINT('Ctrl Pts',(28.9015873956338,537.51358261161,-49.1444898445045)) ;
#51687=CARTESIAN_POINT('Ctrl Pts',(28.8402440473705,537.477097248407,-49.1405048762514)) ;
#51688=CARTESIAN_POINT('Ctrl Pts',(28.7789172502295,537.440621729364,-49.1365209831874)) ;
#51689=CARTESIAN_POINT('Ctrl Pts',(28.7194495875471,537.400977465339,-49.1326203867606)) ;
#51690=CARTESIAN_POINT('Ctrl Pts',(28.6621751277739,537.358386212482,-49.1288074354721)) ;
#51691=CARTESIAN_POINT('Ctrl Pts',(28.6536953228304,537.352080338661,-49.1282429066522)) ;
#51692=CARTESIAN_POINT('Ctrl Pts',(28.6452635611451,537.345709918296,-49.1276802548137)) ;
#51693=CARTESIAN_POINT('Ctrl Pts',(28.6368808924516,537.339275726356,-49.1271194481244)) ;
#51694=CARTESIAN_POINT('',(30.4186978425951,533.72539083489,-49.522160171753)) ;
#51695=CARTESIAN_POINT('Ctrl Pts',(30.4186978425951,533.72539083489,-49.522160171753)) ;
#51696=CARTESIAN_POINT('Ctrl Pts',(30.4888567936994,533.744127822299,-49.5182228345589)) ;
#51697=CARTESIAN_POINT('Ctrl Pts',(30.558087616928,533.766605982304,-49.5142854973648)) ;
#51698=CARTESIAN_POINT('Ctrl Pts',(30.6259762638657,533.792710351632,-49.5103481601707)) ;
#51699=CARTESIAN_POINT('Ctrl Pts',(30.6938110350337,533.818794004787,-49.506413947609)) ;
#51700=CARTESIAN_POINT('Ctrl Pts',(30.7603053193206,533.848497980627,-49.5024797350474)) ;
#51701=CARTESIAN_POINT('Ctrl Pts',(30.8250616606322,533.881657955873,-49.4985455224858)) ;
#51702=CARTESIAN_POINT('Ctrl Pts',(30.8897993492147,533.91480837956,-49.4946124431537)) ;
#51703=CARTESIAN_POINT('Ctrl Pts',(30.9527996772528,533.951412621011,-49.4906793638217)) ;
#51704=CARTESIAN_POINT('Ctrl Pts',(31.013687583735,533.991259303341,-49.4867462844896)) ;
#51705=CARTESIAN_POINT('Ctrl Pts',(31.074568968254,534.031101717522,-49.4828136264465)) ;
#51706=CARTESIAN_POINT('Ctrl Pts',(31.1333379955336,534.074185630533,-49.4788809684033)) ;
#51707=CARTESIAN_POINT('Ctrl Pts',(31.1896478347493,534.120255831111,-49.4749483103601)) ;
#51708=CARTESIAN_POINT('Ctrl Pts',(31.2459675257825,534.166334092006,-49.4710149642697)) ;
#51709=CARTESIAN_POINT('Ctrl Pts',(31.2998268175,534.215399387038,-49.4670816181793)) ;
#51710=CARTESIAN_POINT('Ctrl Pts',(31.3509123698971,534.267156548428,-49.463148272089)) ;
#51711=CARTESIAN_POINT('Ctrl Pts',(31.4020212719486,534.318937366444,-49.4592131281855)) ;
#51712=CARTESIAN_POINT('Ctrl Pts',(31.4503535920648,534.373412168299,-49.4552779842821)) ;
#51713=CARTESIAN_POINT('Ctrl Pts',(31.4956342011548,534.430250349007,-49.4513428403787)) ;
#51714=CARTESIAN_POINT('Ctrl Pts',(31.5409821077165,534.487173004415,-49.44740184794)) ;
#51715=CARTESIAN_POINT('Ctrl Pts',(31.5832689630283,534.546465688977,-49.4434608555014)) ;
#51716=CARTESIAN_POINT('Ctrl Pts',(31.6222614450573,534.607766627239,-49.4395198630628)) ;
#51717=CARTESIAN_POINT('Ctrl Pts',(31.6612865134216,534.669118795194,-49.4355755771047)) ;
#51718=CARTESIAN_POINT('Ctrl Pts',(31.6970114993853,534.732482158629,-49.4316312911465)) ;
#51719=CARTESIAN_POINT('Ctrl Pts',(31.7292490458786,534.797470305294,-49.4276870051883)) ;
#51720=CARTESIAN_POINT('Ctrl Pts',(31.7615480685897,534.862582382776,-49.4237351975727)) ;
#51721=CARTESIAN_POINT('Ctrl Pts',(31.7903461900897,534.929325007906,-49.419783389957)) ;
#51722=CARTESIAN_POINT('Ctrl Pts',(31.8155043249335,534.997292167956,-49.4158315823414)) ;
#51723=CARTESIAN_POINT('Ctrl Pts',(31.8258890467887,535.025347508973,-49.4142003635262)) ;
#51724=CARTESIAN_POINT('Ctrl Pts',(31.8356541601606,535.053611326253,-49.4125691447109)) ;
#51725=CARTESIAN_POINT('Ctrl Pts',(31.8447924034538,535.082054475949,-49.4109379258957)) ;
#51726=CARTESIAN_POINT('Ctrl Pts',(31.8702884146574,535.161411836006,-49.4063867696335)) ;
#51727=CARTESIAN_POINT('Ctrl Pts',(31.8909796284462,535.242409214064,-49.4018356133713)) ;
#51728=CARTESIAN_POINT('Ctrl Pts',(31.906684111172,535.324505629577,-49.3972844571091)) ;
#51729=CARTESIAN_POINT('Ctrl Pts',(31.9222193282413,535.405717195592,-49.3927823540036)) ;
#51730=CARTESIAN_POINT('Ctrl Pts',(31.932874645567,535.488004119788,-49.3882802508982)) ;
#51731=CARTESIAN_POINT('Ctrl Pts',(31.9385201320457,535.570821519473,-49.3837781477928)) ;
#51732=CARTESIAN_POINT('Ctrl Pts',(31.9416727614126,535.617069538546,-49.381264022125)) ;
#51733=CARTESIAN_POINT('Ctrl Pts',(31.9432639189038,535.663482614069,-49.3787498964571)) ;
#51734=CARTESIAN_POINT('Ctrl Pts',(31.9432775372141,535.709963140231,-49.3762357707893)) ;
#51735=CARTESIAN_POINT('',(29.3554672321407,533.72404407569,-49.5209785487821)) ;
#51736=CARTESIAN_POINT('Origin',(29.8885276254068,535.710565160562,-49.522160171753)) ;
#51737=CARTESIAN_POINT('',(31.9432771819323,535.711915145219,-49.3167693044577)) ;
#51738=CARTESIAN_POINT('Ctrl Pts',(29.3560800705629,533.726000431499,-49.5197877449898)) ;
#51739=CARTESIAN_POINT('Ctrl Pts',(29.3727232359274,533.721535163839,-49.5188564377852)) ;
#51740=CARTESIAN_POINT('Ctrl Pts',(29.3894225027156,533.717279276791,-49.5179369715456)) ;
#51741=CARTESIAN_POINT('Ctrl Pts',(29.4275700894734,533.708066669072,-49.5158664643182)) ;
#51742=CARTESIAN_POINT('Ctrl Pts',(29.4490486950172,533.703243462867,-49.5147220435414)) ;
#51743=CARTESIAN_POINT('Ctrl Pts',(29.5664110730149,533.678862888878,-49.5085644277625)) ;
#51744=CARTESIAN_POINT('Ctrl Pts',(29.6635282606455,533.665827630833,-49.5038106332384)) ;
#51745=CARTESIAN_POINT('Ctrl Pts',(29.8915725628636,533.651670337441,-49.4927393155173)) ;
#51746=CARTESIAN_POINT('Ctrl Pts',(30.0224045088476,533.65602595308,-49.4864409899781)) ;
#51747=CARTESIAN_POINT('Ctrl Pts',(30.2079858419884,533.680013778618,-49.4768874456396)) ;
#51748=CARTESIAN_POINT('Ctrl Pts',(30.2637160955301,533.689569047045,-49.4739405330125)) ;
#51749=CARTESIAN_POINT('Ctrl Pts',(30.3680315882367,533.711918078274,-49.4682378815688)) ;
#51750=CARTESIAN_POINT('Ctrl Pts',(30.4166798891431,533.724219577228,-49.4655000002555)) ;
#51751=CARTESIAN_POINT('Ctrl Pts',(30.5445911424325,533.761595219636,-49.4580750887874)) ;
#51752=CARTESIAN_POINT('Ctrl Pts',(30.6228598065772,533.789717209359,-49.4532925867747)) ;
#51753=CARTESIAN_POINT('Ctrl Pts',(30.8140677135829,533.871815859139,-49.4410475906918)) ;
#51754=CARTESIAN_POINT('Ctrl Pts',(30.9241891067755,533.931513110172,-49.4334636245622)) ;
#51755=CARTESIAN_POINT('Ctrl Pts',(31.0665555861296,534.026411614519,-49.4233144062885)) ;
#51756=CARTESIAN_POINT('Ctrl Pts',(31.1040477223569,534.053267848236,-49.4206079819085)) ;
#51757=CARTESIAN_POINT('Ctrl Pts',(31.1698936576313,534.103871969374,-49.4158347599524)) ;
#51758=CARTESIAN_POINT('Ctrl Pts',(31.1985707888151,534.127167169066,-49.4137487080267)) ;
#51759=CARTESIAN_POINT('Ctrl Pts',(31.2493004256202,534.170698534935,-49.4100692849863)) ;
#51760=CARTESIAN_POINT('Ctrl Pts',(31.2715663529941,534.190665243779,-49.4084606671827)) ;
#51761=CARTESIAN_POINT('Ctrl Pts',(31.3366761739484,534.251667683194,-49.4037553528811)) ;
#51762=CARTESIAN_POINT('Ctrl Pts',(31.3781898803372,534.294082346143,-49.4007502827554)) ;
#51763=CARTESIAN_POINT('Ctrl Pts',(31.4873264227819,534.415701166193,-49.3926420604992)) ;
#51764=CARTESIAN_POINT('Ctrl Pts',(31.55085602518,534.498337347723,-49.387672378011)) ;
#51765=CARTESIAN_POINT('Ctrl Pts',(31.6648889251331,534.672592225477,-49.3775567511667)) ;
#51766=CARTESIAN_POINT('Ctrl Pts',(31.7152113557656,534.763954895763,-49.37242335646)) ;
#51767=CARTESIAN_POINT('Ctrl Pts',(31.7802066507066,534.906626139092,-49.3643321820162)) ;
#51768=CARTESIAN_POINT('Ctrl Pts',(31.8001756990715,534.955337738357,-49.3615594048482)) ;
#51769=CARTESIAN_POINT('Ctrl Pts',(31.8363684585771,535.054291381281,-49.3558778863244)) ;
#51770=CARTESIAN_POINT('Ctrl Pts',(31.8525698956854,535.104498811128,-49.3529710065729)) ;
#51771=CARTESIAN_POINT('Ctrl Pts',(31.9000570651526,535.273676769314,-49.3430798085291)) ;
#51772=CARTESIAN_POINT('Ctrl Pts',(31.922591208741,535.39481190557,-49.335823589588)) ;
#51773=CARTESIAN_POINT('Ctrl Pts',(31.9402776177387,535.581936393661,-49.3245597660857)) ;
#51774=CARTESIAN_POINT('Ctrl Pts',(31.9433198919006,535.64690826683,-49.320643686283)) ;
#51775=CARTESIAN_POINT('Ctrl Pts',(31.9432771819323,535.711915145219,-49.3167693044577)) ;
#51776=CARTESIAN_POINT('Ctrl Pts',(31.9432771821887,535.711914754875,-49.316769327722)) ;
#51777=CARTESIAN_POINT('Ctrl Pts',(31.9432442412748,535.762067106419,-49.3137802691297)) ;
#51778=CARTESIAN_POINT('Ctrl Pts',(31.941375124574,535.81220422679,-49.3108186377364)) ;
#51779=CARTESIAN_POINT('Ctrl Pts',(31.935239464843,535.895105881199,-49.3060138397542)) ;
#51780=CARTESIAN_POINT('Ctrl Pts',(31.9320147090053,535.927925272046,-49.3041359273484)) ;
#51781=CARTESIAN_POINT('Ctrl Pts',(31.9244399497136,535.989697261163,-49.3006647157832)) ;
#51782=CARTESIAN_POINT('Ctrl Pts',(31.9202587559306,536.018660315781,-49.2990652834471)) ;
#51783=CARTESIAN_POINT('Ctrl Pts',(31.908350508511,536.09029170372,-49.295181798816)) ;
#51784=CARTESIAN_POINT('Ctrl Pts',(31.8998895435613,536.132821597177,-49.2929352499796)) ;
#51785=CARTESIAN_POINT('Ctrl Pts',(31.8569359724237,536.317915483408,-49.2832956882657)) ;
#51786=CARTESIAN_POINT('Ctrl Pts',(31.8085816250829,536.456826069626,-49.2763964087115)) ;
#51787=CARTESIAN_POINT('Ctrl Pts',(31.7057618926767,536.674120685695,-49.2646638002179)) ;
#51788=CARTESIAN_POINT('Ctrl Pts',(31.659934744771,536.755980875926,-49.2600041806642)) ;
#51789=CARTESIAN_POINT('Ctrl Pts',(31.5805394180119,536.87750203505,-49.2524774593003)) ;
#51790=CARTESIAN_POINT('Ctrl Pts',(31.5507872934754,536.919505907853,-49.2497534889718)) ;
#51791=CARTESIAN_POINT('Ctrl Pts',(31.4863647494126,537.003577295079,-49.2440172155548)) ;
#51792=CARTESIAN_POINT('Ctrl Pts',(31.45153460719,537.045470484097,-49.2409995908442)) ;
#51793=CARTESIAN_POINT('Ctrl Pts',(31.3064081366201,537.206550656237,-49.2287249406726)) ;
#51794=CARTESIAN_POINT('Ctrl Pts',(31.1838318185616,537.313852215177,-49.2189349912047)) ;
#51795=CARTESIAN_POINT('Ctrl Pts',(30.9992486535197,537.440325784766,-49.2055003678904)) ;
#51796=CARTESIAN_POINT('Ctrl Pts',(30.9470260259433,537.472766870433,-49.2018322810649)) ;
#51797=CARTESIAN_POINT('Ctrl Pts',(30.8546840726854,537.524542022241,-49.1956566208903)) ;
#51798=CARTESIAN_POINT('Ctrl Pts',(30.8152451609863,537.545003912148,-49.1931110486386)) ;
#51799=CARTESIAN_POINT('Ctrl Pts',(30.7489496785119,537.576715299247,-49.1890192263442)) ;
#51800=CARTESIAN_POINT('Ctrl Pts',(30.7224665776565,537.588699467579,-49.1874343691132)) ;
#51801=CARTESIAN_POINT('Ctrl Pts',(30.6541063944406,537.617902503545,-49.1834660876428)) ;
#51802=CARTESIAN_POINT('Ctrl Pts',(30.6119000927807,537.634306166757,-49.1811267062722)) ;
#51803=CARTESIAN_POINT('Ctrl Pts',(30.4405285772705,537.694471602745,-49.1719380640321)) ;
#51804=CARTESIAN_POINT('Ctrl Pts',(30.3076890610578,537.72672458864,-49.1654883249192)) ;
#51805=CARTESIAN_POINT('Ctrl Pts',(30.0753224501381,537.75916413168,-49.154053407005)) ;
#51806=CARTESIAN_POINT('Ctrl Pts',(29.9771775838908,537.765750941677,-49.1491818034942)) ;
#51807=CARTESIAN_POINT('Ctrl Pts',(29.8269908818347,537.765050517608,-49.1414011947215)) ;
#51808=CARTESIAN_POINT('Ctrl Pts',(29.7750682356347,537.762837843774,-49.138653428477)) ;
#51809=CARTESIAN_POINT('Ctrl Pts',(29.6690509062983,537.754284405276,-49.1328974098437)) ;
#51810=CARTESIAN_POINT('Ctrl Pts',(29.6150131225046,537.74775621618,-49.1298852279418)) ;
#51811=CARTESIAN_POINT('Ctrl Pts',(29.398899056158,537.712894370113,-49.1175034461975)) ;
#51812=CARTESIAN_POINT('Ctrl Pts',(29.2402503322034,537.667291745539,-49.1075843390555)) ;
#51813=CARTESIAN_POINT('Ctrl Pts',(29.0328830950625,537.579669339908,-49.0940780794124)) ;
#51814=CARTESIAN_POINT('Ctrl Pts',(28.9780709480623,537.553591837422,-49.0904601762015)) ;
#51815=CARTESIAN_POINT('Ctrl Pts',(28.8855561250087,537.504440720834,-49.0843545219273)) ;
#51816=CARTESIAN_POINT('Ctrl Pts',(28.8472941897546,537.482506148734,-49.081829938437)) ;
#51817=CARTESIAN_POINT('Ctrl Pts',(28.7849406839166,537.444042639508,-49.0777535852956)) ;
#51818=CARTESIAN_POINT('Ctrl Pts',(28.7604467942342,537.428203695349,-49.076164555607)) ;
#51819=CARTESIAN_POINT('Ctrl Pts',(28.7022966236552,537.388820082287,-49.072418156034)) ;
#51820=CARTESIAN_POINT('Ctrl Pts',(28.6689956370738,537.364779643092,-49.0702908162921)) ;
#51821=CARTESIAN_POINT('Ctrl Pts',(28.6364362889498,537.339756631099,-49.0682055192064)) ;
#51822=CARTESIAN_POINT('Origin',(179.888527625407,535.710565160536,-51.0680854522974)) ;
#51823=CARTESIAN_POINT('',(178.636454084242,537.33977030723,-47.7297172548539)) ;
#51824=CARTESIAN_POINT('',(178.636454031283,537.33977026653,-47.6715235483075)) ;
#51825=CARTESIAN_POINT('',(178.636454050035,537.339770280941,-51.0680854522974)) ;
#51826=CARTESIAN_POINT('',(178.005900115743,534.887332980433,-47.5221601717597)) ;
#51827=CARTESIAN_POINT('Ctrl Pts',(178.636454031283,537.33977026653,-47.6715235483074)) ;
#51828=CARTESIAN_POINT('Ctrl Pts',(178.622241244291,537.328847482636,-47.6704814600419)) ;
#51829=CARTESIAN_POINT('Ctrl Pts',(178.608170085452,537.317737714185,-47.6694339709133)) ;
#51830=CARTESIAN_POINT('Ctrl Pts',(178.487795454974,537.220111933605,-47.6603392051397)) ;
#51831=CARTESIAN_POINT('Ctrl Pts',(178.390257733755,537.123352082591,-47.6520244043183)) ;
#51832=CARTESIAN_POINT('Ctrl Pts',(178.270766695043,536.978408908741,-47.6410250446098)) ;
#51833=CARTESIAN_POINT('Ctrl Pts',(178.239914709743,536.938023679574,-47.6380976511002)) ;
#51834=CARTESIAN_POINT('Ctrl Pts',(178.193334887254,536.872121366306,-47.6335859562082)) ;
#51835=CARTESIAN_POINT('Ctrl Pts',(178.176614522369,536.847334760524,-47.6319467323779)) ;
#51836=CARTESIAN_POINT('Ctrl Pts',(178.137892637096,536.787139091179,-47.6281088021966)) ;
#51837=CARTESIAN_POINT('Ctrl Pts',(178.116416799119,536.751410008282,-47.6259405168292)) ;
#51838=CARTESIAN_POINT('Ctrl Pts',(178.042631843038,536.619741986076,-47.6182538607249)) ;
#51839=CARTESIAN_POINT('Ctrl Pts',(177.996904655671,536.5203182312,-47.6130098299662)) ;
#51840=CARTESIAN_POINT('Ctrl Pts',(177.913976207121,536.29407751075,-47.6014095683289)) ;
#51841=CARTESIAN_POINT('Ctrl Pts',(177.880648984741,536.166371915471,-47.5950602972033)) ;
#51842=CARTESIAN_POINT('Ctrl Pts',(177.850344127141,535.977660837293,-47.585308473829)) ;
#51843=CARTESIAN_POINT('Ctrl Pts',(177.843470324144,535.91858396682,-47.5822086935008)) ;
#51844=CARTESIAN_POINT('Ctrl Pts',(177.835129018986,535.803648919444,-47.5760493617157)) ;
#51845=CARTESIAN_POINT('Ctrl Pts',(177.833358928503,535.747864828306,-47.5730017673884)) ;
#51846=CARTESIAN_POINT('Ctrl Pts',(177.834390525618,535.63319364148,-47.5666077983981)) ;
#51847=CARTESIAN_POINT('Ctrl Pts',(177.837451587011,535.574359951797,-47.5632571137478)) ;
#51848=CARTESIAN_POINT('Ctrl Pts',(177.860528500515,535.332069906454,-47.5491992978391)) ;
#51849=CARTESIAN_POINT('Ctrl Pts',(177.902678893347,535.151601443863,-47.538034543782)) ;
#51850=CARTESIAN_POINT('Ctrl Pts',(177.980123617115,534.948275115569,-47.5257870782419)) ;
#51851=CARTESIAN_POINT('Ctrl Pts',(177.99264445056,534.917647004273,-47.523954068162)) ;
#51852=CARTESIAN_POINT('Ctrl Pts',(178.005900115743,534.887332980433,-47.5221601717592)) ;
#51853=CARTESIAN_POINT('',(178.665833051125,534.0564728875,-47.5234367538311)) ;
#51854=CARTESIAN_POINT('Origin',(179.888527625407,535.710565160536,-47.5221601717598)) ;
#51855=CARTESIAN_POINT('Ctrl Pts',(178.66691495143,534.058396876953,-47.5247133359024)) ;
#51856=CARTESIAN_POINT('Ctrl Pts',(178.653554632771,534.068275492082,-47.5256108747939)) ;
#51857=CARTESIAN_POINT('Ctrl Pts',(178.640314154938,534.078316154102,-47.5264974635798)) ;
#51858=CARTESIAN_POINT('Ctrl Pts',(178.609741628923,534.10208984521,-47.5285415549366)) ;
#51859=CARTESIAN_POINT('Ctrl Pts',(178.592506376018,534.115944372768,-47.529691568149)) ;
#51860=CARTESIAN_POINT('Ctrl Pts',(178.480887460634,534.208674458136,-47.5371483885131)) ;
#51861=CARTESIAN_POINT('Ctrl Pts',(178.393517563906,534.295617517028,-47.543040828045)) ;
#51862=CARTESIAN_POINT('Ctrl Pts',(178.238400994016,534.480493399766,-47.554746511401)) ;
#51863=CARTESIAN_POINT('Ctrl Pts',(178.17033202049,534.577518430838,-47.5605359409273)) ;
#51864=CARTESIAN_POINT('Ctrl Pts',(178.0843676294,534.725769974689,-47.569377909882)) ;
#51865=CARTESIAN_POINT('Ctrl Pts',(178.059533375984,534.772698322752,-47.5721734120944)) ;
#51866=CARTESIAN_POINT('Ctrl Pts',(178.013598200371,534.868280411217,-47.5778903672997)) ;
#51867=CARTESIAN_POINT('Ctrl Pts',(177.992508280832,534.91689403092,-47.58080939126)) ;
#51868=CARTESIAN_POINT('Ctrl Pts',(177.933132345828,535.069678090164,-47.5900337950995)) ;
#51869=CARTESIAN_POINT('Ctrl Pts',(177.901389966094,535.176163280757,-47.5965450728088)) ;
#51870=CARTESIAN_POINT('Ctrl Pts',(177.85863217262,535.377973848484,-47.6088662704022)) ;
#51871=CARTESIAN_POINT('Ctrl Pts',(177.845384512702,535.472533506183,-47.6146279962836)) ;
#51872=CARTESIAN_POINT('Ctrl Pts',(177.83587297935,535.608974478693,-47.6226983222894)) ;
#51873=CARTESIAN_POINT('Ctrl Pts',(177.834242565512,535.650357026585,-47.6251131677995)) ;
#51874=CARTESIAN_POINT('Ctrl Pts',(177.833548742366,535.726175030821,-47.6294456249277)) ;
#51875=CARTESIAN_POINT('Ctrl Pts',(177.834098391708,535.760592294423,-47.631377639716)) ;
#51876=CARTESIAN_POINT('Ctrl Pts',(177.836788018584,535.8260042097,-47.634962833962)) ;
#51877=CARTESIAN_POINT('Ctrl Pts',(177.838766611096,535.856994141036,-47.6366225394175)) ;
#51878=CARTESIAN_POINT('Ctrl Pts',(177.847683417546,535.959909738471,-47.6420371816208)) ;
#51879=CARTESIAN_POINT('Ctrl Pts',(177.857712919098,536.031518797643,-47.6456483375471)) ;
#51880=CARTESIAN_POINT('Ctrl Pts',(177.90335162002,536.266417695381,-47.657388391457)) ;
#51881=CARTESIAN_POINT('Ctrl Pts',(177.955078554029,536.425877429872,-47.6652397567559)) ;
#51882=CARTESIAN_POINT('Ctrl Pts',(178.050738467198,536.631487382625,-47.6767287643819)) ;
#51883=CARTESIAN_POINT('Ctrl Pts',(178.078288131683,536.684525530326,-47.6798209461223)) ;
#51884=CARTESIAN_POINT('Ctrl Pts',(178.132999386801,536.779492003157,-47.6856461779284)) ;
#51885=CARTESIAN_POINT('Ctrl Pts',(178.159454084318,536.821775344459,-47.6883518928744)) ;
#51886=CARTESIAN_POINT('Ctrl Pts',(178.228469563014,536.923644446014,-47.695170288032)) ;
#51887=CARTESIAN_POINT('Ctrl Pts',(178.272724187717,536.981994100583,-47.6993455034216)) ;
#51888=CARTESIAN_POINT('Ctrl Pts',(178.414445354432,537.149474191995,-47.7121467206265)) ;
#51889=CARTESIAN_POINT('Ctrl Pts',(178.520532853448,537.250682750497,-47.7210498099191)) ;
#51890=CARTESIAN_POINT('Ctrl Pts',(178.636454084242,537.33977030723,-47.7297172548539)) ;
#51891=CARTESIAN_POINT('Origin',(179.888527625407,535.710565160536,-51.0680854522974)) ;
#51892=CARTESIAN_POINT('',(178.636454050042,537.339770280947,-48.4293891818575)) ;
#51893=CARTESIAN_POINT('',(178.636454050035,537.339770280941,-48.3712393117967)) ;
#51894=CARTESIAN_POINT('',(178.636454050035,537.339770280941,-51.0680854522974)) ;
#51895=CARTESIAN_POINT('',(181.943277552311,535.710017082759,-47.9194801829612)) ;
#51896=CARTESIAN_POINT('Ctrl Pts',(178.636454050035,537.339770280941,-48.3712393117967)) ;
#51897=CARTESIAN_POINT('Ctrl Pts',(178.61681784653,537.324679503714,-48.3699919406657)) ;
#51898=CARTESIAN_POINT('Ctrl Pts',(178.597447145434,537.309228100014,-48.3687333142884)) ;
#51899=CARTESIAN_POINT('Ctrl Pts',(178.53619493261,537.258527921646,-48.3646541659042)) ;
#51900=CARTESIAN_POINT('Ctrl Pts',(178.495451670995,537.221965527656,-48.3617871416412)) ;
#51901=CARTESIAN_POINT('Ctrl Pts',(178.419091441373,537.147727686935,-48.3560701383734)) ;
#51902=CARTESIAN_POINT('Ctrl Pts',(178.383344862517,537.110244761674,-48.3532296844346)) ;
#51903=CARTESIAN_POINT('Ctrl Pts',(178.285708819313,536.999796288613,-48.3449692570823)) ;
#51904=CARTESIAN_POINT('Ctrl Pts',(178.2274514836,536.923811742882,-48.3394070274034)) ;
#51905=CARTESIAN_POINT('Ctrl Pts',(178.099180161897,536.729866740007,-48.3255872806016)) ;
#51906=CARTESIAN_POINT('Ctrl Pts',(178.035261483984,536.608420374485,-48.3172233934903)) ;
#51907=CARTESIAN_POINT('Ctrl Pts',(177.96633307106,536.438134095399,-48.3064756171413)) ;
#51908=CARTESIAN_POINT('Ctrl Pts',(177.950257036136,536.394155862429,-48.3037846453818)) ;
#51909=CARTESIAN_POINT('Ctrl Pts',(177.926626139136,536.32194923244,-48.2995449213575)) ;
#51910=CARTESIAN_POINT('Ctrl Pts',(177.918147228565,536.29404547518,-48.2979504864009)) ;
#51911=CARTESIAN_POINT('Ctrl Pts',(177.898542956795,536.224217629692,-48.2940696480827)) ;
#51912=CARTESIAN_POINT('Ctrl Pts',(177.88814575171,536.182105970463,-48.2918209449869)) ;
#51913=CARTESIAN_POINT('Ctrl Pts',(177.866756075967,536.081946641437,-48.2866210903349)) ;
#51914=CARTESIAN_POINT('Ctrl Pts',(177.85691814294,536.023691392238,-48.2837120782991)) ;
#51915=CARTESIAN_POINT('Ctrl Pts',(177.828580044645,535.796683649006,-48.2725614363835)) ;
#51916=CARTESIAN_POINT('Ctrl Pts',(177.828502451848,535.626333647324,-48.2645239715233)) ;
#51917=CARTESIAN_POINT('Ctrl Pts',(177.85601137451,535.404309255045,-48.2530204633537)) ;
#51918=CARTESIAN_POINT('Ctrl Pts',(177.864763379831,535.350992423478,-48.250184514104)) ;
#51919=CARTESIAN_POINT('Ctrl Pts',(177.886104562335,535.246846390212,-48.2444671461068)) ;
#51920=CARTESIAN_POINT('Ctrl Pts',(177.898556008103,535.196030932204,-48.24159216538)) ;
#51921=CARTESIAN_POINT('Ctrl Pts',(177.941407423834,535.046146656137,-48.2328388124249)) ;
#51922=CARTESIAN_POINT('Ctrl Pts',(177.977371222526,534.948852930602,-48.2267844777629)) ;
#51923=CARTESIAN_POINT('Ctrl Pts',(178.076475489919,534.732548601796,-48.2125910509409)) ;
#51924=CARTESIAN_POINT('Ctrl Pts',(178.144284352135,534.616186123,-48.2043923758195)) ;
#51925=CARTESIAN_POINT('Ctrl Pts',(178.247791903485,534.472913818179,-48.1941182136836)) ;
#51926=CARTESIAN_POINT('Ctrl Pts',(178.273675922731,534.439325978522,-48.1916974722371)) ;
#51927=CARTESIAN_POINT('Ctrl Pts',(178.319142746753,534.383958966747,-48.1877195471781)) ;
#51928=CARTESIAN_POINT('Ctrl Pts',(178.338181747529,534.361758022489,-48.1861303511333)) ;
#51929=CARTESIAN_POINT('Ctrl Pts',(178.389902506627,534.303990534366,-48.1820036036833)) ;
#51930=CARTESIAN_POINT('Ctrl Pts',(178.42337409428,534.269157775859,-48.1795195938335)) ;
#51931=CARTESIAN_POINT('Ctrl Pts',(178.508728658754,534.186381007479,-48.1735325044469)) ;
#51932=CARTESIAN_POINT('Ctrl Pts',(178.561915306547,534.139870008612,-48.1700918698385)) ;
#51933=CARTESIAN_POINT('Ctrl Pts',(178.733413332153,534.004835267902,-48.1595104238687)) ;
#51934=CARTESIAN_POINT('Ctrl Pts',(178.858932391316,533.926263119798,-48.1524274739569)) ;
#51935=CARTESIAN_POINT('Ctrl Pts',(179.040596208193,533.838146157368,-48.1420539146653)) ;
#51936=CARTESIAN_POINT('Ctrl Pts',(179.090322079901,533.816414217006,-48.1392077861016)) ;
#51937=CARTESIAN_POINT('Ctrl Pts',(179.18933198082,533.777734954425,-48.1334948978683)) ;
#51938=CARTESIAN_POINT('Ctrl Pts',(179.238515931001,533.760644328828,-48.1306357841272)) ;
#51939=CARTESIAN_POINT('Ctrl Pts',(179.383738495676,533.716287018275,-48.1221158578994)) ;
#51940=CARTESIAN_POINT('Ctrl Pts',(179.481169690976,533.694129539853,-48.1162953426907)) ;
#51941=CARTESIAN_POINT('Ctrl Pts',(179.714214922398,533.658713979496,-48.102252649518)) ;
#51942=CARTESIAN_POINT('Ctrl Pts',(179.850308016329,533.651677714594,-48.093947686279)) ;
#51943=CARTESIAN_POINT('Ctrl Pts',(180.030456657865,533.660241816041,-48.0834283459741)) ;
#51944=CARTESIAN_POINT('Ctrl Pts',(180.074738376255,533.663788227966,-48.0808835460415)) ;
#51945=CARTESIAN_POINT('Ctrl Pts',(180.147774755263,533.672027840135,-48.0767916304269)) ;
#51946=CARTESIAN_POINT('Ctrl Pts',(180.176601900043,533.675901331577,-48.0752059894901)) ;
#51947=CARTESIAN_POINT('Ctrl Pts',(180.250162087207,533.68738058732,-48.0712321752011)) ;
#51948=CARTESIAN_POINT('Ctrl Pts',(180.294741366709,533.695857664443,-48.0688883242128)) ;
#51949=CARTESIAN_POINT('Ctrl Pts',(180.401053808762,533.719746552248,-48.06337697629)) ;
#51950=CARTESIAN_POINT('Ctrl Pts',(180.462423730457,533.736562651236,-48.0602593885099)) ;
#51951=CARTESIAN_POINT('Ctrl Pts',(180.67122633419,533.804340257326,-48.0495907810143)) ;
#51952=CARTESIAN_POINT('Ctrl Pts',(180.813562497029,533.869201881747,-48.0421664624997)) ;
#51953=CARTESIAN_POINT('Ctrl Pts',(180.994395316116,533.977911858992,-48.0313605436958)) ;
#51954=CARTESIAN_POINT('Ctrl Pts',(181.040434135106,534.008172298556,-48.028479989484)) ;
#51955=CARTESIAN_POINT('Ctrl Pts',(181.126766735997,534.070023736512,-48.0227868124446)) ;
#51956=CARTESIAN_POINT('Ctrl Pts',(181.167204890963,534.101342975496,-48.0199861807067)) ;
#51957=CARTESIAN_POINT('Ctrl Pts',(181.274979489639,534.19144309082,-48.0121268326259)) ;
#51958=CARTESIAN_POINT('Ctrl Pts',(181.339709689749,534.253153739325,-48.0069492620272)) ;
#51959=CARTESIAN_POINT('Ctrl Pts',(181.51000038868,534.438127290328,-47.9920464639506)) ;
#51960=CARTESIAN_POINT('Ctrl Pts',(181.605285557693,534.569945891328,-47.9820652095229)) ;
#51961=CARTESIAN_POINT('Ctrl Pts',(181.702850138356,534.745308503317,-47.9704548150123)) ;
#51962=CARTESIAN_POINT('Ctrl Pts',(181.720658563074,534.779553215839,-47.9682616028805)) ;
#51963=CARTESIAN_POINT('Ctrl Pts',(181.750455348452,534.841021728951,-47.9644807979488)) ;
#51964=CARTESIAN_POINT('Ctrl Pts',(181.762834472073,534.868036512242,-47.9628730883071)) ;
#51965=CARTESIAN_POINT('Ctrl Pts',(181.796020306939,534.944812569609,-47.958437123859)) ;
#51966=CARTESIAN_POINT('Ctrl Pts',(181.815460302174,534.995137516539,-47.9556805832737)) ;
#51967=CARTESIAN_POINT('Ctrl Pts',(181.860682373304,535.127481722694,-47.9486790861811)) ;
#51968=CARTESIAN_POINT('Ctrl Pts',(181.883339355026,535.210457074341,-47.9445258986763)) ;
#51969=CARTESIAN_POINT('Ctrl Pts',(181.919415715015,535.384978693358,-47.9358756317244)) ;
#51970=CARTESIAN_POINT('Ctrl Pts',(181.93198670496,535.476499536271,-47.9313838294082)) ;
#51971=CARTESIAN_POINT('Ctrl Pts',(181.941626372663,535.61563888671,-47.924358540693)) ;
#51972=CARTESIAN_POINT('Ctrl Pts',(181.943264963639,535.662822005758,-47.9219435873794)) ;
#51973=CARTESIAN_POINT('Ctrl Pts',(181.943277552311,535.710017082759,-47.9194801829612)) ;
#51974=CARTESIAN_POINT('Ctrl Pts',(181.943277552624,535.710018258454,-47.9194801215943)) ;
#51975=CARTESIAN_POINT('Ctrl Pts',(181.943289182331,535.753711894313,-47.9171994784251)) ;
#51976=CARTESIAN_POINT('Ctrl Pts',(181.941907122319,535.797392922001,-47.9148785468896)) ;
#51977=CARTESIAN_POINT('Ctrl Pts',(181.935807836813,535.893285140802,-47.9096765599099)) ;
#51978=CARTESIAN_POINT('Ctrl Pts',(181.930483325185,535.945424826066,-47.9067778059617)) ;
#51979=CARTESIAN_POINT('Ctrl Pts',(181.899871429793,536.162643392762,-47.894386332717)) ;
#51980=CARTESIAN_POINT('Ctrl Pts',(181.856505277595,536.324507726671,-47.8843162387126)) ;
#51981=CARTESIAN_POINT('Ctrl Pts',(181.760655183561,536.562096114654,-47.868923340987)) ;
#51982=CARTESIAN_POINT('Ctrl Pts',(181.721894328725,536.642625116597,-47.8636035240152)) ;
#51983=CARTESIAN_POINT('Ctrl Pts',(181.662105794812,536.748575747719,-47.8566824597145)) ;
#51984=CARTESIAN_POINT('Ctrl Pts',(181.64553099857,536.776391143384,-47.8548737936266)) ;
#51985=CARTESIAN_POINT('Ctrl Pts',(181.61040251692,536.832294406511,-47.8512741825207)) ;
#51986=CARTESIAN_POINT('Ctrl Pts',(181.591802550929,536.860340992242,-47.8494863364649)) ;
#51987=CARTESIAN_POINT('Ctrl Pts',(181.499101817306,536.9929326575,-47.8410586031852)) ;
#51988=CARTESIAN_POINT('Ctrl Pts',(181.416012823482,537.090859172478,-47.8348961676524)) ;
#51989=CARTESIAN_POINT('Ctrl Pts',(181.237719945758,537.265022725074,-47.8227870929446)) ;
#51990=CARTESIAN_POINT('Ctrl Pts',(181.143801406468,537.341804745452,-47.8168668400908)) ;
#51991=CARTESIAN_POINT('Ctrl Pts',(180.999193941225,537.440105869839,-47.8078436098311)) ;
#51992=CARTESIAN_POINT('Ctrl Pts',(180.953543430938,537.468584318471,-47.8050099607897)) ;
#51993=CARTESIAN_POINT('Ctrl Pts',(180.860275747129,537.521801245292,-47.7992175498136)) ;
#51994=CARTESIAN_POINT('Ctrl Pts',(180.812702534486,537.546530994621,-47.796261516008)) ;
#51995=CARTESIAN_POINT('Ctrl Pts',(180.661918162597,537.617566219307,-47.786870025466)) ;
#51996=CARTESIAN_POINT('Ctrl Pts',(180.555825367047,537.657227384585,-47.7802179886134)) ;
#51997=CARTESIAN_POINT('Ctrl Pts',(180.355248261042,537.713878343011,-47.7677376528832)) ;
#51998=CARTESIAN_POINT('Ctrl Pts',(180.261781089591,537.733378562018,-47.7619624973742)) ;
#51999=CARTESIAN_POINT('Ctrl Pts',(180.111044672498,537.754019928219,-47.7529668189346)) ;
#52000=CARTESIAN_POINT('Ctrl Pts',(180.054492459894,537.759388708774,-47.7496635970557)) ;
#52001=CARTESIAN_POINT('Ctrl Pts',(179.968382870824,537.763973965642,-47.744812096897)) ;
#52002=CARTESIAN_POINT('Ctrl Pts',(179.938946271435,537.764907607887,-47.7431853149115)) ;
#52003=CARTESIAN_POINT('Ctrl Pts',(179.87501806743,537.765560039696,-47.739735646073)) ;
#52004=CARTESIAN_POINT('Ctrl Pts',(179.840533702508,537.765044015645,-47.7379257465054)) ;
#52005=CARTESIAN_POINT('Ctrl Pts',(179.693200965336,537.759127210237,-47.7303492195271)) ;
#52006=CARTESIAN_POINT('Ctrl Pts',(179.580879348399,537.745292849729,-47.7249582791518)) ;
#52007=CARTESIAN_POINT('Ctrl Pts',(179.334288381766,537.694022409274,-47.7129510924467)) ;
#52008=CARTESIAN_POINT('Ctrl Pts',(179.201550247138,537.652044534648,-47.7063503629113)) ;
#52009=CARTESIAN_POINT('Ctrl Pts',(179.022973899834,537.574944681291,-47.6964728773845)) ;
#52010=CARTESIAN_POINT('Ctrl Pts',(178.972805295937,537.550822227816,-47.6935832826104)) ;
#52011=CARTESIAN_POINT('Ctrl Pts',(178.879618558127,537.501260740286,-47.6879606784832)) ;
#52012=CARTESIAN_POINT('Ctrl Pts',(178.836428328765,537.47623064679,-47.6852442933513)) ;
#52013=CARTESIAN_POINT('Ctrl Pts',(178.739916262091,537.415499816828,-47.6789059786744)) ;
#52014=CARTESIAN_POINT('Ctrl Pts',(178.687279541144,537.378830590225,-47.6752500987332)) ;
#52015=CARTESIAN_POINT('Ctrl Pts',(178.636454031283,537.33977026653,-47.6715235483074)) ;
#52016=CARTESIAN_POINT('Ctrl Pts',(178.636454084242,537.33977030723,-47.7297172548539)) ;
#52017=CARTESIAN_POINT('Ctrl Pts',(178.685687477448,537.37760705793,-47.7333984418258)) ;
#52018=CARTESIAN_POINT('Ctrl Pts',(178.736606611229,537.413190289609,-47.7370242250661)) ;
#52019=CARTESIAN_POINT('Ctrl Pts',(178.81115013104,537.46040467576,-47.7419998958145)) ;
#52020=CARTESIAN_POINT('Ctrl Pts',(178.833494913938,537.473967190394,-47.7434510381069)) ;
#52021=CARTESIAN_POINT('Ctrl Pts',(178.884590621336,537.503661479162,-47.7466683557087)) ;
#52022=CARTESIAN_POINT('Ctrl Pts',(178.913483882856,537.519535555978,-47.7484173758533)) ;
#52023=CARTESIAN_POINT('Ctrl Pts',(179.062251292068,537.59666827089,-47.7571337599225)) ;
#52024=CARTESIAN_POINT('Ctrl Pts',(179.187567416033,537.646741921251,-47.7635554209541)) ;
#52025=CARTESIAN_POINT('Ctrl Pts',(179.396521964938,537.707262613412,-47.774072988367)) ;
#52026=CARTESIAN_POINT('Ctrl Pts',(179.477470882733,537.725484920213,-47.7781011992131)) ;
#52027=CARTESIAN_POINT('Ctrl Pts',(179.624237138341,537.749309043585,-47.7855481689957)) ;
#52028=CARTESIAN_POINT('Ctrl Pts',(179.689642272061,537.756724871013,-47.788915922458)) ;
#52029=CARTESIAN_POINT('Ctrl Pts',(179.804441588076,537.76418477248,-47.7949809709441)) ;
#52030=CARTESIAN_POINT('Ctrl Pts',(179.853692118013,537.76561014154,-47.7976317136049)) ;
#52031=CARTESIAN_POINT('Ctrl Pts',(179.966529828995,537.764818463141,-47.8038352455562)) ;
#52032=CARTESIAN_POINT('Ctrl Pts',(180.030055466799,537.76142097971,-47.8074232914933)) ;
#52033=CARTESIAN_POINT('Ctrl Pts',(180.240322480307,537.740359586022,-47.819617383276)) ;
#52034=CARTESIAN_POINT('Ctrl Pts',(180.385300255133,537.709823286097,-47.8285802680629)) ;
#52035=CARTESIAN_POINT('Ctrl Pts',(180.59961835303,537.639914291865,-47.8420724700505)) ;
#52036=CARTESIAN_POINT('Ctrl Pts',(180.672087200866,537.611637101074,-47.8466703459523)) ;
#52037=CARTESIAN_POINT('Ctrl Pts',(180.771414483415,537.566231969079,-47.8528671189628)) ;
#52038=CARTESIAN_POINT('Ctrl Pts',(180.799742361165,537.55248714087,-47.8546214501462)) ;
#52039=CARTESIAN_POINT('Ctrl Pts',(180.857528093276,537.522789460561,-47.8581560180192)) ;
#52040=CARTESIAN_POINT('Ctrl Pts',(180.886933737727,537.506756782897,-47.8599313551668)) ;
#52041=CARTESIAN_POINT('Ctrl Pts',(181.02800350684,537.425306566577,-47.8683969585011)) ;
#52042=CARTESIAN_POINT('Ctrl Pts',(181.133720115245,537.350152378984,-47.8745943726628)) ;
#52043=CARTESIAN_POINT('Ctrl Pts',(181.319259516789,537.189889052216,-47.8864586667367)) ;
#52044=CARTESIAN_POINT('Ctrl Pts',(181.400293523093,537.106972648024,-47.8920931915066)) ;
#52045=CARTESIAN_POINT('Ctrl Pts',(181.508904298271,536.975240139511,-47.9008373333092)) ;
#52046=CARTESIAN_POINT('Ctrl Pts',(181.542175965983,536.931413138843,-47.9037142096324)) ;
#52047=CARTESIAN_POINT('Ctrl Pts',(181.602880850663,536.844408458367,-47.9094002714266)) ;
#52048=CARTESIAN_POINT('Ctrl Pts',(181.630539202881,536.801437566428,-47.912197582475)) ;
#52049=CARTESIAN_POINT('Ctrl Pts',(181.70221812751,536.680385981463,-47.9200649155108)) ;
#52050=CARTESIAN_POINT('Ctrl Pts',(181.742773293613,536.600394060534,-47.92525409321)) ;
#52051=CARTESIAN_POINT('Ctrl Pts',(181.825000726815,536.407981178919,-47.937645641096)) ;
#52052=CARTESIAN_POINT('Ctrl Pts',(181.862320735848,536.294051458501,-47.9449225581174)) ;
#52053=CARTESIAN_POINT('Ctrl Pts',(181.899846458246,536.133248562576,-47.9547314664799)) ;
#52054=CARTESIAN_POINT('Ctrl Pts',(181.908707131037,536.08863911412,-47.9574030989414)) ;
#52055=CARTESIAN_POINT('Ctrl Pts',(181.922017294556,536.007646758512,-47.9621243266189)) ;
#52056=CARTESIAN_POINT('Ctrl Pts',(181.92698775211,535.971368515585,-47.9641927971265)) ;
#52057=CARTESIAN_POINT('Ctrl Pts',(181.934265639859,535.905128903429,-47.9678620142713)) ;
#52058=CARTESIAN_POINT('Ctrl Pts',(181.936890223218,535.875215636876,-47.969477156334)) ;
#52059=CARTESIAN_POINT('Ctrl Pts',(181.942795410697,535.785322881013,-47.9742283013494)) ;
#52060=CARTESIAN_POINT('Ctrl Pts',(181.944103114246,535.725242506601,-47.9772698330283)) ;
#52061=CARTESIAN_POINT('Ctrl Pts',(181.939807372805,535.530777245452,-47.9869191182631)) ;
#52062=CARTESIAN_POINT('Ctrl Pts',(181.923654142591,535.396981089927,-47.9932757005685)) ;
#52063=CARTESIAN_POINT('Ctrl Pts',(181.880006417125,535.200153733712,-48.0031982680774)) ;
#52064=CARTESIAN_POINT('Ctrl Pts',(181.862262496659,535.135345816245,-48.0065581455773)) ;
#52065=CARTESIAN_POINT('Ctrl Pts',(181.824716310563,535.020607722103,-48.0127700932045)) ;
#52066=CARTESIAN_POINT('Ctrl Pts',(181.806070139393,534.970363904315,-48.0155846515336)) ;
#52067=CARTESIAN_POINT('Ctrl Pts',(181.765484718173,534.872867392984,-48.0212662086155)) ;
#52068=CARTESIAN_POINT('Ctrl Pts',(181.743669947075,534.825606549667,-48.0241272649742)) ;
#52069=CARTESIAN_POINT('Ctrl Pts',(181.637263841788,534.616349464793,-48.037310963502)) ;
#52070=CARTESIAN_POINT('Ctrl Pts',(181.533094672285,534.46526905478,-48.0483661238227)) ;
#52071=CARTESIAN_POINT('Ctrl Pts',(181.356431001054,534.27053028914,-48.0641163596042)) ;
#52072=CARTESIAN_POINT('Ctrl Pts',(181.299055818234,534.214285394287,-48.0688725918868)) ;
#52073=CARTESIAN_POINT('Ctrl Pts',(181.214643608276,534.140718643376,-48.0752298539368)) ;
#52074=CARTESIAN_POINT('Ctrl Pts',(181.190274298195,534.120452697429,-48.0769969582583)) ;
#52075=CARTESIAN_POINT('Ctrl Pts',(181.139306206774,534.080024295535,-48.0805382092355)) ;
#52076=CARTESIAN_POINT('Ctrl Pts',(181.11266591736,534.059930040175,-48.0823082034492)) ;
#52077=CARTESIAN_POINT('Ctrl Pts',(180.953855587551,533.946103305297,-48.0924699359517)) ;
#52078=CARTESIAN_POINT('Ctrl Pts',(180.81144783541,533.867610934047,-48.1000769692788)) ;
#52079=CARTESIAN_POINT('Ctrl Pts',(180.570904824445,533.769979519519,-48.1127366084379)) ;
#52080=CARTESIAN_POINT('Ctrl Pts',(180.478037008903,533.739781721875,-48.1175760540537)) ;
#52081=CARTESIAN_POINT('Ctrl Pts',(180.333230600594,533.703849705101,-48.1253071526701)) ;
#52082=CARTESIAN_POINT('Ctrl Pts',(180.282630468146,533.693302172839,-48.1280403114051)) ;
#52083=CARTESIAN_POINT('Ctrl Pts',(180.178433531459,533.675652461824,-48.1337593693304)) ;
#52084=CARTESIAN_POINT('Ctrl Pts',(180.124846742387,533.668735682704,-48.1367489086414)) ;
#52085=CARTESIAN_POINT('Ctrl Pts',(179.904910132251,533.649120960526,-48.1492346210964)) ;
#52086=CARTESIAN_POINT('Ctrl Pts',(179.737601533126,533.654592126093,-48.159301603949)) ;
#52087=CARTESIAN_POINT('Ctrl Pts',(179.487761388751,533.693439602165,-48.1744722269792)) ;
#52088=CARTESIAN_POINT('Ctrl Pts',(179.403601174043,533.712001199492,-48.1795913309669)) ;
#52089=CARTESIAN_POINT('Ctrl Pts',(179.290062045862,533.744639780057,-48.1863067908646)) ;
#52090=CARTESIAN_POINT('Ctrl Pts',(179.259484878687,533.754209058198,-48.1880953221101)) ;
#52091=CARTESIAN_POINT('Ctrl Pts',(179.197961285549,533.77505501519,-48.1916352548595)) ;
#52092=CARTESIAN_POINT('Ctrl Pts',(179.167037319044,533.786368339009,-48.1933842396946)) ;
#52093=CARTESIAN_POINT('Ctrl Pts',(179.009921108121,533.848169089616,-48.2021772461662)) ;
#52094=CARTESIAN_POINT('Ctrl Pts',(178.888678795771,533.910348738732,-48.2086665715154)) ;
#52095=CARTESIAN_POINT('Ctrl Pts',(178.673966415221,534.048896898901,-48.2210444597538)) ;
#52096=CARTESIAN_POINT('Ctrl Pts',(178.57933642824,534.122385320502,-48.226889775387)) ;
#52097=CARTESIAN_POINT('Ctrl Pts',(178.452950738439,534.239545158775,-48.2357814647762)) ;
#52098=CARTESIAN_POINT('Ctrl Pts',(178.415658974168,534.276885243045,-48.2385603147672)) ;
#52099=CARTESIAN_POINT('Ctrl Pts',(178.344055460991,534.354326682618,-48.2442473141203)) ;
#52100=CARTESIAN_POINT('Ctrl Pts',(178.309769405397,534.394396923196,-48.2471532337662)) ;
#52101=CARTESIAN_POINT('Ctrl Pts',(178.175002471345,534.564751096159,-48.2593832535293)) ;
#52102=CARTESIAN_POINT('Ctrl Pts',(178.088817253075,534.705535772939,-48.2692705151715)) ;
#52103=CARTESIAN_POINT('Ctrl Pts',(177.993640978736,534.913372349241,-48.2830021825533)) ;
#52104=CARTESIAN_POINT('Ctrl Pts',(177.969679022503,534.972911745534,-48.2868374235868)) ;
#52105=CARTESIAN_POINT('Ctrl Pts',(177.933527588759,535.076492484416,-48.2932467352559)) ;
#52106=CARTESIAN_POINT('Ctrl Pts',(177.919948078301,535.119998914121,-48.2958621955047)) ;
#52107=CARTESIAN_POINT('Ctrl Pts',(177.90012185313,535.191837338889,-48.3000171060359)) ;
#52108=CARTESIAN_POINT('Ctrl Pts',(177.893009336659,535.219909412402,-48.3015988068127)) ;
#52109=CARTESIAN_POINT('Ctrl Pts',(177.876657549292,535.290701370407,-48.3054837502227)) ;
#52110=CARTESIAN_POINT('Ctrl Pts',(177.868183479543,535.333581232832,-48.3077478081702)) ;
#52111=CARTESIAN_POINT('Ctrl Pts',(177.83909292664,535.510238707624,-48.3168304746283)) ;
#52112=CARTESIAN_POINT('Ctrl Pts',(177.830348255772,535.645630785443,-48.3232403425754)) ;
#52113=CARTESIAN_POINT('Ctrl Pts',(177.838429805884,535.88156067798,-48.3347349174434)) ;
#52114=CARTESIAN_POINT('Ctrl Pts',(177.849272749966,535.981816591309,-48.339719750075)) ;
#52115=CARTESIAN_POINT('Ctrl Pts',(177.876771223467,536.131903443152,-48.3476189791927)) ;
#52116=CARTESIAN_POINT('Ctrl Pts',(177.888051210792,536.182564349684,-48.3503609527888)) ;
#52117=CARTESIAN_POINT('Ctrl Pts',(177.914888722308,536.284702240533,-48.3560713388705)) ;
#52118=CARTESIAN_POINT('Ctrl Pts',(177.930573436248,536.336103750902,-48.3590421460671)) ;
#52119=CARTESIAN_POINT('Ctrl Pts',(178.004141518487,536.547178733051,-48.37166963816)) ;
#52120=CARTESIAN_POINT('Ctrl Pts',(178.079685826321,536.69996237271,-48.3819248012611)) ;
#52121=CARTESIAN_POINT('Ctrl Pts',(178.219595310628,536.912141291437,-48.3971658400929)) ;
#52122=CARTESIAN_POINT('Ctrl Pts',(178.270355455873,536.97967566915,-48.4021787262244)) ;
#52123=CARTESIAN_POINT('Ctrl Pts',(178.345859865158,537.068208090769,-48.4087903721179)) ;
#52124=CARTESIAN_POINT('Ctrl Pts',(178.367155882681,537.092030505018,-48.4105733956411)) ;
#52125=CARTESIAN_POINT('Ctrl Pts',(178.411595647049,537.139467452332,-48.4141143447367)) ;
#52126=CARTESIAN_POINT('Ctrl Pts',(178.434770842369,537.163039368276,-48.415869368546)) ;
#52127=CARTESIAN_POINT('Ctrl Pts',(178.514834388777,537.240636309498,-48.4216735689377)) ;
#52128=CARTESIAN_POINT('Ctrl Pts',(178.574247376926,537.29196332856,-48.4255599821672)) ;
#52129=CARTESIAN_POINT('Ctrl Pts',(178.636454050048,537.339770280952,-48.4293891818575)) ;
#52130=CARTESIAN_POINT('Origin',(179.888527625407,535.710565160536,-51.0680854522974)) ;
#52131=CARTESIAN_POINT('',(178.636879422838,537.339310206396,-49.1271677662019)) ;
#52132=CARTESIAN_POINT('',(178.63645405003,537.339770280938,-49.068197094383)) ;
#52133=CARTESIAN_POINT('',(178.636454050035,537.339770280941,-51.0680854522974)) ;
#52134=CARTESIAN_POINT('',(181.943277580094,535.710133636274,-49.3762357667005)) ;
#52135=CARTESIAN_POINT('Ctrl Pts',(181.942732094631,535.710094699042,-49.3752911028376)) ;
#52136=CARTESIAN_POINT('Ctrl Pts',(181.942612236032,535.781018676224,-49.3712179668236)) ;
#52137=CARTESIAN_POINT('Ctrl Pts',(181.938847034173,535.851983770071,-49.3672000176889)) ;
#52138=CARTESIAN_POINT('Ctrl Pts',(181.931463151663,535.922593192326,-49.3632666223797)) ;
#52139=CARTESIAN_POINT('Ctrl Pts',(181.924081156149,535.993184569906,-49.3593342322741)) ;
#52140=CARTESIAN_POINT('Ctrl Pts',(181.913082344595,536.063420436168,-49.3554863828943)) ;
#52141=CARTESIAN_POINT('Ctrl Pts',(181.898527821528,536.132908506928,-49.3517278271686)) ;
#52142=CARTESIAN_POINT('Ctrl Pts',(181.883972033896,536.202402615143,-49.3479689448817)) ;
#52143=CARTESIAN_POINT('Ctrl Pts',(181.865859822924,536.271148727557,-49.3442992991325)) ;
#52144=CARTESIAN_POINT('Ctrl Pts',(181.844287389052,536.33875934524,-49.340699365354)) ;
#52145=CARTESIAN_POINT('Ctrl Pts',(181.822690028396,536.406448086481,-49.3370952718792)) ;
#52146=CARTESIAN_POINT('Ctrl Pts',(181.797624237622,536.472998575918,-49.3335608658333)) ;
#52147=CARTESIAN_POINT('Ctrl Pts',(181.769223963578,536.538028362011,-49.3300541262992)) ;
#52148=CARTESIAN_POINT('Ctrl Pts',(181.740806087874,536.603098451665,-49.3265452133903)) ;
#52149=CARTESIAN_POINT('Ctrl Pts',(181.709049279655,536.666645717014,-49.3230636557219)) ;
#52150=CARTESIAN_POINT('Ctrl Pts',(181.674129078134,536.72829607859,-49.3195488526866)) ;
#52151=CARTESIAN_POINT('Ctrl Pts',(181.641232218846,536.786374302125,-49.3162377039577)) ;
#52152=CARTESIAN_POINT('Ctrl Pts',(181.605527529697,536.842769255252,-49.3128965589948)) ;
#52153=CARTESIAN_POINT('Ctrl Pts',(181.567200958708,536.897178224159,-49.309464902831)) ;
#52154=CARTESIAN_POINT('Ctrl Pts',(181.564766879856,536.900633678617,-49.3092469620792)) ;
#52155=CARTESIAN_POINT('Ctrl Pts',(181.562322224758,536.904081140274,-49.3090286562612)) ;
#52156=CARTESIAN_POINT('Ctrl Pts',(181.559867040392,536.907520538678,-49.3088099698756)) ;
#52157=CARTESIAN_POINT('Ctrl Pts',(181.533655540383,536.944239488394,-49.3064752783248)) ;
#52158=CARTESIAN_POINT('Ctrl Pts',(181.506245088415,536.980037446018,-49.3040969780512)) ;
#52159=CARTESIAN_POINT('Ctrl Pts',(181.477704697016,537.01482513965,-49.3016555691048)) ;
#52160=CARTESIAN_POINT('Ctrl Pts',(181.477682537963,537.014852149172,-49.3016536735699)) ;
#52161=CARTESIAN_POINT('Ctrl Pts',(181.47766037823,537.014879158086,-49.3016517779969)) ;
#52162=CARTESIAN_POINT('Ctrl Pts',(181.477638217815,537.014906166391,-49.3016498823858)) ;
#52163=CARTESIAN_POINT('Ctrl Pts',(181.436814508576,537.064660614799,-49.2981578054215)) ;
#52164=CARTESIAN_POINT('Ctrl Pts',(181.393521978287,537.112529155155,-49.2945273176486)) ;
#52165=CARTESIAN_POINT('Ctrl Pts',(181.347981718345,537.158282002969,-49.2908235105092)) ;
#52166=CARTESIAN_POINT('Ctrl Pts',(181.343365148449,537.162920123616,-49.2904480430753)) ;
#52167=CARTESIAN_POINT('Ctrl Pts',(181.338725522968,537.167536493735,-49.2900718221704)) ;
#52168=CARTESIAN_POINT('Ctrl Pts',(181.334063101611,537.172130868916,-49.2896949156048)) ;
#52169=CARTESIAN_POINT('Ctrl Pts',(181.283485863795,537.221969952159,-49.2856062905021)) ;
#52170=CARTESIAN_POINT('Ctrl Pts',(181.230220348857,537.269222364421,-49.2814375954658)) ;
#52171=CARTESIAN_POINT('Ctrl Pts',(181.174586059164,537.31362423241,-49.2772632006393)) ;
#52172=CARTESIAN_POINT('Ctrl Pts',(181.11902049435,537.357971250897,-49.2730939624307)) ;
#52173=CARTESIAN_POINT('Ctrl Pts',(181.061092190998,537.399475095859,-49.2689193920925)) ;
#52174=CARTESIAN_POINT('Ctrl Pts',(181.001136864184,537.43790914616,-49.264794227375)) ;
#52175=CARTESIAN_POINT('Ctrl Pts',(180.941221589826,537.476317521041,-49.2606718184257)) ;
#52176=CARTESIAN_POINT('Ctrl Pts',(180.879282064005,537.51166036401,-49.2565989179649)) ;
#52177=CARTESIAN_POINT('Ctrl Pts',(180.815668928836,537.543744055674,-49.2526069624869)) ;
#52178=CARTESIAN_POINT('Ctrl Pts',(180.7520769123,537.57581709602,-49.24861633228)) ;
#52179=CARTESIAN_POINT('Ctrl Pts',(180.686812415575,537.604633163758,-49.2447066336286)) ;
#52180=CARTESIAN_POINT('Ctrl Pts',(180.620240751481,537.630030069174,-49.2408845573474)) ;
#52181=CARTESIAN_POINT('Ctrl Pts',(180.553668817217,537.65542707766,-49.2370624655548)) ;
#52182=CARTESIAN_POINT('Ctrl Pts',(180.485789704087,537.677404786938,-49.2333279321044)) ;
#52183=CARTESIAN_POINT('Ctrl Pts',(180.416983636269,537.695832968407,-49.2296631161707)) ;
#52184=CARTESIAN_POINT('Ctrl Pts',(180.348108656542,537.714279606405,-49.2259946297836)) ;
#52185=CARTESIAN_POINT('Ctrl Pts',(180.278304854469,537.729169363093,-49.2223958222781)) ;
#52186=CARTESIAN_POINT('Ctrl Pts',(180.207968634237,537.74040625583,-49.2188260103383)) ;
#52187=CARTESIAN_POINT('Ctrl Pts',(180.137594532266,537.751649200542,-49.2152542757663)) ;
#52188=CARTESIAN_POINT('Ctrl Pts',(180.066687456419,537.759234954533,-49.2117112303463)) ;
#52189=CARTESIAN_POINT('Ctrl Pts',(179.995659490086,537.763106735024,-49.2081371490813)) ;
#52190=CARTESIAN_POINT('Ctrl Pts',(179.928400267569,537.766773078845,-49.2047527085643)) ;
#52191=CARTESIAN_POINT('Ctrl Pts',(179.861032305697,537.767108839787,-49.201339947582)) ;
#52192=CARTESIAN_POINT('Ctrl Pts',(179.793918731335,537.764104628672,-49.1978376486995)) ;
#52193=CARTESIAN_POINT('Ctrl Pts',(179.790036214827,537.763930835227,-49.1976350409058)) ;
#52194=CARTESIAN_POINT('Ctrl Pts',(179.786154536828,537.763745870956,-49.1974321334632)) ;
#52195=CARTESIAN_POINT('Ctrl Pts',(179.782273762848,537.763549736425,-49.1972289145198)) ;
#52196=CARTESIAN_POINT('Ctrl Pts',(179.739287724431,537.76137721967,-49.1949779260948)) ;
#52197=CARTESIAN_POINT('Ctrl Pts',(179.696414650976,537.757834212928,-49.1926884999008)) ;
#52198=CARTESIAN_POINT('Ctrl Pts',(179.653751674576,537.752928288526,-49.1903438535763)) ;
#52199=CARTESIAN_POINT('Ctrl Pts',(179.653718285716,537.752924449056,-49.1903420186113)) ;
#52200=CARTESIAN_POINT('Ctrl Pts',(179.653684896984,537.752920608751,-49.1903401836125)) ;
#52201=CARTESIAN_POINT('Ctrl Pts',(179.65365150838,537.752916767612,-49.1903383485799)) ;
#52202=CARTESIAN_POINT('Ctrl Pts',(179.589356052093,537.745519998755,-49.1868046799592)) ;
#52203=CARTESIAN_POINT('Ctrl Pts',(179.525317171513,537.734995616538,-49.1831368770369)) ;
#52204=CARTESIAN_POINT('Ctrl Pts',(179.461851214523,537.721406764875,-49.1793998856796)) ;
#52205=CARTESIAN_POINT('Ctrl Pts',(179.455650975345,537.720079216462,-49.1790348042829)) ;
#52206=CARTESIAN_POINT('Ctrl Pts',(179.449456232737,537.718722449947,-49.1786690625444)) ;
#52207=CARTESIAN_POINT('Ctrl Pts',(179.443267299683,537.717336543757,-49.1783027210199)) ;
#52208=CARTESIAN_POINT('Ctrl Pts',(179.374199730459,537.701870037523,-49.1742144042798)) ;
#52209=CARTESIAN_POINT('Ctrl Pts',(179.305851875357,537.682770540929,-49.1700521274263)) ;
#52210=CARTESIAN_POINT('Ctrl Pts',(179.238611196729,537.660162868676,-49.1658874860574)) ;
#52211=CARTESIAN_POINT('Ctrl Pts',(179.23503962159,537.658962033083,-49.165666275774)) ;
#52212=CARTESIAN_POINT('Ctrl Pts',(179.231471179888,537.657751307145,-49.1654450588195)) ;
#52213=CARTESIAN_POINT('Ctrl Pts',(179.227905932883,537.656530712147,-49.1652238459231)) ;
#52214=CARTESIAN_POINT('Ctrl Pts',(179.160504656848,537.633455267364,-49.1610417986558)) ;
#52215=CARTESIAN_POINT('Ctrl Pts',(179.094240989185,537.606850259365,-49.1568614088824)) ;
#52216=CARTESIAN_POINT('Ctrl Pts',(179.029486970148,537.576877752761,-49.1527351337744)) ;
#52217=CARTESIAN_POINT('Ctrl Pts',(178.964775922315,537.546925136113,-49.1486115968904)) ;
#52218=CARTESIAN_POINT('Ctrl Pts',(178.901572425724,537.513609621424,-49.1445422608489)) ;
#52219=CARTESIAN_POINT('Ctrl Pts',(178.840228975474,537.477123555206,-49.1405561895766)) ;
#52220=CARTESIAN_POINT('Ctrl Pts',(178.778902241526,537.440647431568,-49.1365712045225)) ;
#52221=CARTESIAN_POINT('Ctrl Pts',(178.719434543581,537.401002500273,-49.1326694711559)) ;
#52222=CARTESIAN_POINT('Ctrl Pts',(178.662159968225,537.358410485806,-49.1288553535565)) ;
#52223=CARTESIAN_POINT('Ctrl Pts',(178.653684781395,537.352107946191,-49.1282909607339)) ;
#52224=CARTESIAN_POINT('Ctrl Pts',(178.645257583569,537.345740928522,-49.1277284421922)) ;
#52225=CARTESIAN_POINT('Ctrl Pts',(178.636879422838,537.339310206396,-49.1271677662019)) ;
#52226=CARTESIAN_POINT('',(180.418697842595,533.725390834864,-49.5221601717598)) ;
#52227=CARTESIAN_POINT('Ctrl Pts',(180.418697842595,533.725390834864,-49.5221601717598)) ;
#52228=CARTESIAN_POINT('Ctrl Pts',(180.488838649278,533.744122976537,-49.518223852835)) ;
#52229=CARTESIAN_POINT('Ctrl Pts',(180.558052648722,533.766594582606,-49.5142875339101)) ;
#52230=CARTESIAN_POINT('Ctrl Pts',(180.625925910679,533.792690990686,-49.5103512149853)) ;
#52231=CARTESIAN_POINT('Ctrl Pts',(180.693744619936,533.818766423945,-49.5064180598516)) ;
#52232=CARTESIAN_POINT('Ctrl Pts',(180.760224305597,533.848460701642,-49.5024849047179)) ;
#52233=CARTESIAN_POINT('Ctrl Pts',(180.824967594848,533.88160979035,-49.4985517495843)) ;
#52234=CARTESIAN_POINT('Ctrl Pts',(180.889691398045,533.914748902039,-49.4946197782285)) ;
#52235=CARTESIAN_POINT('Ctrl Pts',(180.952679430811,533.951340554724,-49.4906878068727)) ;
#52236=CARTESIAN_POINT('Ctrl Pts',(181.013556689828,533.99117364994,-49.4867558355169)) ;
#52237=CARTESIAN_POINT('Ctrl Pts',(181.074426964584,534.031002175228,-49.4828243152641)) ;
#52238=CARTESIAN_POINT('Ctrl Pts',(181.133186561213,534.07407115205,-49.4788927950113)) ;
#52239=CARTESIAN_POINT('Ctrl Pts',(181.189488680937,534.120125631823,-49.4749612747585)) ;
#52240=CARTESIAN_POINT('Ctrl Pts',(181.24580026511,534.166187853405,-49.4710290936129)) ;
#52241=CARTESIAN_POINT('Ctrl Pts',(181.299653194963,534.215236283368,-49.4670969124672)) ;
#52242=CARTESIAN_POINT('Ctrl Pts',(181.350734142247,534.266975999933,-49.4631647313215)) ;
#52243=CARTESIAN_POINT('Ctrl Pts',(181.401838125353,534.318739049403,-49.4592307768919)) ;
#52244=CARTESIAN_POINT('Ctrl Pts',(181.450167318291,534.373195469547,-49.4552968224622)) ;
#52245=CARTESIAN_POINT('Ctrl Pts',(181.495446588511,534.430014884867,-49.4513628680326)) ;
#52246=CARTESIAN_POINT('Ctrl Pts',(181.540792862541,534.486918380989,-49.4474230921767)) ;
#52247=CARTESIAN_POINT('Ctrl Pts',(181.583079917915,534.546191490856,-49.4434833163208)) ;
#52248=CARTESIAN_POINT('Ctrl Pts',(181.622074419214,534.607472654813,-49.4395435404648)) ;
#52249=CARTESIAN_POINT('Ctrl Pts',(181.661101355421,534.668804791314,-49.4356004875759)) ;
#52250=CARTESIAN_POINT('Ctrl Pts',(181.696830057013,534.732147907397,-49.431657434687)) ;
#52251=CARTESIAN_POINT('Ctrl Pts',(181.72907314629,534.79711579245,-49.4277143817981)) ;
#52252=CARTESIAN_POINT('Ctrl Pts',(181.76137764778,534.862207419418,-49.423763818723)) ;
#52253=CARTESIAN_POINT('Ctrl Pts',(181.790183098063,534.928929571959,-49.419813255648)) ;
#52254=CARTESIAN_POINT('Ctrl Pts',(181.815350386823,534.99687642685,-49.4158626925729)) ;
#52255=CARTESIAN_POINT('Ctrl Pts',(181.825808223044,535.025110579802,-49.4142211036828)) ;
#52256=CARTESIAN_POINT('Ctrl Pts',(181.835638465713,535.053556030198,-49.4125795147927)) ;
#52257=CARTESIAN_POINT('Ctrl Pts',(181.844833710026,535.082183058801,-49.4109379259025)) ;
#52258=CARTESIAN_POINT('Ctrl Pts',(181.870323447816,535.161538802694,-49.4063873485671)) ;
#52259=CARTESIAN_POINT('Ctrl Pts',(181.891008381187,535.242533191184,-49.4018367712316)) ;
#52260=CARTESIAN_POINT('Ctrl Pts',(181.906706975086,535.32462517164,-49.3972861938962)) ;
#52261=CARTESIAN_POINT('Ctrl Pts',(181.922237610317,535.405838853072,-49.3927843030172)) ;
#52262=CARTESIAN_POINT('Ctrl Pts',(181.932887947934,535.488126649793,-49.3882824121382)) ;
#52263=CARTESIAN_POINT('Ctrl Pts',(181.938528448063,535.570943566185,-49.3837805212593)) ;
#52264=CARTESIAN_POINT('Ctrl Pts',(181.941679434335,535.617208074757,-49.381265603073)) ;
#52265=CARTESIAN_POINT('Ctrl Pts',(181.943267815266,535.663637337958,-49.3787506848868)) ;
#52266=CARTESIAN_POINT('Ctrl Pts',(181.943277580094,535.710133636274,-49.3762357667005)) ;
#52267=CARTESIAN_POINT('',(179.355529476285,533.723981678234,-49.5209531416429)) ;
#52268=CARTESIAN_POINT('Origin',(179.888527625407,535.710565160536,-49.5221601717598)) ;
#52269=CARTESIAN_POINT('Ctrl Pts',(179.35615550176,533.725980195244,-49.5197367207334)) ;
#52270=CARTESIAN_POINT('Ctrl Pts',(179.386645754433,533.717801074244,-49.5180294859388)) ;
#52271=CARTESIAN_POINT('Ctrl Pts',(179.417322303353,533.710325199925,-49.5163621213256)) ;
#52272=CARTESIAN_POINT('Ctrl Pts',(179.622903662318,533.665217608102,-49.5054480379446)) ;
#52273=CARTESIAN_POINT('Ctrl Pts',(179.801923802628,533.649856959711,-49.4971291703748)) ;
#52274=CARTESIAN_POINT('Ctrl Pts',(180.047717573492,533.660892458951,-49.485012096855)) ;
#52275=CARTESIAN_POINT('Ctrl Pts',(180.114555802346,533.667183176172,-49.4816539730302)) ;
#52276=CARTESIAN_POINT('Ctrl Pts',(180.23424793227,533.684393154191,-49.4754314008979)) ;
#52277=CARTESIAN_POINT('Ctrl Pts',(180.287207316818,533.694145231136,-49.472603422141)) ;
#52278=CARTESIAN_POINT('Ctrl Pts',(180.390698302709,533.717438814379,-49.4668972475788)) ;
#52279=CARTESIAN_POINT('Ctrl Pts',(180.441216797588,533.730852555527,-49.4640251044105)) ;
#52280=CARTESIAN_POINT('Ctrl Pts',(180.65792497081,533.797334656294,-49.4513013214398)) ;
#52281=CARTESIAN_POINT('Ctrl Pts',(180.81746876098,533.869513342516,-49.4408032426431)) ;
#52282=CARTESIAN_POINT('Ctrl Pts',(181.037110801698,534.004769463289,-49.4253764557488)) ;
#52283=CARTESIAN_POINT('Ctrl Pts',(181.105540710678,534.052897009306,-49.4204246101205)) ;
#52284=CARTESIAN_POINT('Ctrl Pts',(181.195790796679,534.124980360512,-49.4138717576755)) ;
#52285=CARTESIAN_POINT('Ctrl Pts',(181.220262775655,534.145477956014,-49.41209288984)) ;
#52286=CARTESIAN_POINT('Ctrl Pts',(181.269176698201,534.188426483131,-49.4085509733121)) ;
#52287=CARTESIAN_POINT('Ctrl Pts',(181.293572257131,534.210915908282,-49.4067913841307)) ;
#52288=CARTESIAN_POINT('Ctrl Pts',(181.413278697187,534.326756018982,-49.3981294082487)) ;
#52289=CARTESIAN_POINT('Ctrl Pts',(181.499892092085,534.428650202827,-49.3917554730396)) ;
#52290=CARTESIAN_POINT('Ctrl Pts',(181.623697003062,534.606858943087,-49.3812561991762)) ;
#52291=CARTESIAN_POINT('Ctrl Pts',(181.667140637198,534.678327334671,-49.3771939039362)) ;
#52292=CARTESIAN_POINT('Ctrl Pts',(181.736988274943,534.810801955952,-49.369689875594)) ;
#52293=CARTESIAN_POINT('Ctrl Pts',(181.76501496088,534.870818336318,-49.3662998245454)) ;
#52294=CARTESIAN_POINT('Ctrl Pts',(181.808861072802,534.977918947993,-49.3601970782553)) ;
#52295=CARTESIAN_POINT('Ctrl Pts',(181.825962549433,535.024419149913,-49.3575312027147)) ;
#52296=CARTESIAN_POINT('Ctrl Pts',(181.86132212056,535.132468189636,-49.3512810088282)) ;
#52297=CARTESIAN_POINT('Ctrl Pts',(181.878408942312,535.194343014748,-49.3476608654176)) ;
#52298=CARTESIAN_POINT('Ctrl Pts',(181.924965648381,535.400010234328,-49.3354964877004)) ;
#52299=CARTESIAN_POINT('Ctrl Pts',(181.941935976674,535.546157336872,-49.326610785419)) ;
#52300=CARTESIAN_POINT('Ctrl Pts',(181.943858047043,535.768996053101,-49.3133059277999)) ;
#52301=CARTESIAN_POINT('Ctrl Pts',(181.940280670191,535.845133634881,-49.308812340963)) ;
#52302=CARTESIAN_POINT('Ctrl Pts',(181.929263808215,535.952190298597,-49.3027147707102)) ;
#52303=CARTESIAN_POINT('Ctrl Pts',(181.925325785789,535.983402940241,-49.3009641218704)) ;
#52304=CARTESIAN_POINT('Ctrl Pts',(181.915727075197,536.047577823389,-49.2974378479214)) ;
#52305=CARTESIAN_POINT('Ctrl Pts',(181.909975421435,536.080516829146,-49.2956673991572)) ;
#52306=CARTESIAN_POINT('Ctrl Pts',(181.895615113128,536.15236137623,-49.2918641429117)) ;
#52307=CARTESIAN_POINT('Ctrl Pts',(181.886673590913,536.191186753956,-49.2898467372816)) ;
#52308=CARTESIAN_POINT('Ctrl Pts',(181.854447986343,536.314591035259,-49.2834880027757)) ;
#52309=CARTESIAN_POINT('Ctrl Pts',(181.82687567018,536.397950309466,-49.2792712225611)) ;
#52310=CARTESIAN_POINT('Ctrl Pts',(181.747185681869,536.595486203075,-49.2689783750769)) ;
#52311=CARTESIAN_POINT('Ctrl Pts',(181.689785794362,536.707139456508,-49.26288796729)) ;
#52312=CARTESIAN_POINT('Ctrl Pts',(181.594309382983,536.857336006462,-49.2537261138182)) ;
#52313=CARTESIAN_POINT('Ctrl Pts',(181.564339655096,536.900703029251,-49.250956476311)) ;
#52314=CARTESIAN_POINT('Ctrl Pts',(181.501853638212,536.984075525302,-49.2453503902744)) ;
#52315=CARTESIAN_POINT('Ctrl Pts',(181.469433382929,537.024104568198,-49.2425189484251)) ;
#52316=CARTESIAN_POINT('Ctrl Pts',(181.368551378238,537.1395120866,-49.2339115252726)) ;
#52317=CARTESIAN_POINT('Ctrl Pts',(181.29596259545,537.211059055025,-49.2279652371632)) ;
#52318=CARTESIAN_POINT('Ctrl Pts',(181.115758623106,537.364053576331,-49.2138677783475)) ;
#52319=CARTESIAN_POINT('Ctrl Pts',(181.004824180477,537.440883735331,-49.2056485411836)) ;
#52320=CARTESIAN_POINT('Ctrl Pts',(180.849733588312,537.527132198193,-49.1953182933574)) ;
#52321=CARTESIAN_POINT('Ctrl Pts',(180.811650056526,537.546778170894,-49.1928681465783)) ;
#52322=CARTESIAN_POINT('Ctrl Pts',(180.74705806749,537.577580865455,-49.1888888216884)) ;
#52323=CARTESIAN_POINT('Ctrl Pts',(180.720884240904,537.589395861228,-49.1873250373415)) ;
#52324=CARTESIAN_POINT('Ctrl Pts',(180.65272788296,537.6184578222,-49.1833730240811)) ;
#52325=CARTESIAN_POINT('Ctrl Pts',(180.610407892758,537.634869168835,-49.1810299284733)) ;
#52326=CARTESIAN_POINT('Ctrl Pts',(180.507305367133,537.67097063546,-49.1755073434259)) ;
#52327=CARTESIAN_POINT('Ctrl Pts',(180.446080180925,537.689254498746,-49.1723782979835)) ;
#52328=CARTESIAN_POINT('Ctrl Pts',(180.223772643284,537.744502436524,-49.1612495035639)) ;
#52329=CARTESIAN_POINT('Ctrl Pts',(180.059239454266,537.764864176168,-49.1533859499329)) ;
#52330=CARTESIAN_POINT('Ctrl Pts',(179.841632287978,537.765448490495,-49.1421589582639)) ;
#52331=CARTESIAN_POINT('Ctrl Pts',(179.789237030738,537.763583764509,-49.1393986005986)) ;
#52332=CARTESIAN_POINT('Ctrl Pts',(179.684831578572,537.755861986112,-49.1337552721455)) ;
#52333=CARTESIAN_POINT('Ctrl Pts',(179.632859975274,537.750017176451,-49.1308747110985)) ;
#52334=CARTESIAN_POINT('Ctrl Pts',(179.468617674125,537.725169679011,-49.1215274928822)) ;
#52335=CARTESIAN_POINT('Ctrl Pts',(179.357688670585,537.698820597104,-49.1148350393141)) ;
#52336=CARTESIAN_POINT('Ctrl Pts',(179.115814682438,537.619676163128,-49.0995968615698)) ;
#52337=CARTESIAN_POINT('Ctrl Pts',(178.98694741049,537.562306659906,-49.091019789403)) ;
#52338=CARTESIAN_POINT('Ctrl Pts',(178.836039648971,537.475608581037,-49.0810857387213)) ;
#52339=CARTESIAN_POINT('Ctrl Pts',(178.80753618604,537.458297124332,-49.0792162124116)) ;
#52340=CARTESIAN_POINT('Ctrl Pts',(178.757341218784,537.426113339013,-49.0759540762785)) ;
#52341=CARTESIAN_POINT('Ctrl Pts',(178.735491174142,537.411504682479,-49.0745453838288)) ;
#52342=CARTESIAN_POINT('Ctrl Pts',(178.687662906414,537.378182055663,-49.0714736136423)) ;
#52343=CARTESIAN_POINT('Ctrl Pts',(178.66183693877,537.359277489613,-49.0698228176136)) ;
#52344=CARTESIAN_POINT('Ctrl Pts',(178.63645405003,537.339770280938,-49.0681970943831)) ;
#52345=CARTESIAN_POINT('Origin',(29.8885276254157,585.710565160562,-48.522160171753)) ;
#52346=CARTESIAN_POINT('',(31.4521967054837,586.286174104269,-47.6539767957637)) ;
#52347=CARTESIAN_POINT('',(31.4519519036773,586.286117526679,-47.522160171753)) ;
#52348=CARTESIAN_POINT('',(31.4519519036773,586.286117526679,-48.5221601717531)) ;
#52349=CARTESIAN_POINT('',(29.9644663285049,587.375713641869,-47.5221677112006)) ;
#52350=CARTESIAN_POINT('Origin',(29.8885276254157,585.710565160562,-47.522160171753)) ;
#52351=CARTESIAN_POINT('Ctrl Pts',(29.9644663292412,587.375713658016,-47.5221677113392)) ;
#52352=CARTESIAN_POINT('Ctrl Pts',(30.0172117431049,587.373277266171,-47.5257729693611)) ;
#52353=CARTESIAN_POINT('Ctrl Pts',(30.0699288534817,587.368272470247,-47.5294752834428)) ;
#52354=CARTESIAN_POINT('Ctrl Pts',(30.1223497103767,587.360732154157,-47.5332205362781)) ;
#52355=CARTESIAN_POINT('Ctrl Pts',(30.1822042172788,587.352122567664,-47.537496892579)) ;
#52356=CARTESIAN_POINT('Ctrl Pts',(30.2416737256479,587.340207082712,-47.5418286678001)) ;
#52357=CARTESIAN_POINT('Ctrl Pts',(30.3003811691045,587.325072957424,-47.5461497278178)) ;
#52358=CARTESIAN_POINT('Ctrl Pts',(30.3590287596007,587.309954261563,-47.5504663824616)) ;
#52359=CARTESIAN_POINT('Ctrl Pts',(30.4169159760224,587.291623764065,-47.5547720457429)) ;
#52360=CARTESIAN_POINT('Ctrl Pts',(30.4736830094216,587.270203172543,-47.559021543743)) ;
#52361=CARTESIAN_POINT('Ctrl Pts',(30.5304137076198,587.248796291821,-47.5632683217425)) ;
#52362=CARTESIAN_POINT('Ctrl Pts',(30.5860257065395,587.224303361531,-47.5674588881871)) ;
#52363=CARTESIAN_POINT('Ctrl Pts',(30.640174533252,587.196877873331,-47.5715719488526)) ;
#52364=CARTESIAN_POINT('Ctrl Pts',(30.6943092455541,587.169459533846,-47.5756839374094)) ;
#52365=CARTESIAN_POINT('Ctrl Pts',(30.7469814967011,587.139110137708,-47.5797184700438)) ;
#52366=CARTESIAN_POINT('Ctrl Pts',(30.7978617422621,587.106014648331,-47.5836788440787)) ;
#52367=CARTESIAN_POINT('Ctrl Pts',(30.8487848475891,587.072891280453,-47.5876425541962)) ;
#52368=CARTESIAN_POINT('Ctrl Pts',(30.8979127734843,587.037017070334,-47.5915321047031)) ;
#52369=CARTESIAN_POINT('Ctrl Pts',(30.9449313656306,586.998610227493,-47.5953744366989)) ;
#52370=CARTESIAN_POINT('Ctrl Pts',(30.9919676158759,586.960188960745,-47.5992182117043)) ;
#52371=CARTESIAN_POINT('Ctrl Pts',(31.0368926718298,586.919232960551,-47.6030150058583)) ;
#52372=CARTESIAN_POINT('Ctrl Pts',(31.0794114305104,586.875995869049,-47.6068124945089)) ;
#52373=CARTESIAN_POINT('Ctrl Pts',(31.1220109466605,586.832676655721,-47.6106171958718)) ;
#52374=CARTESIAN_POINT('Ctrl Pts',(31.1621945398082,586.787067423539,-47.6144230682816)) ;
#52375=CARTESIAN_POINT('Ctrl Pts',(31.1996904671793,586.739462053043,-47.6182932968595)) ;
#52376=CARTESIAN_POINT('Ctrl Pts',(31.2333844159271,586.696683729475,-47.6217710954496)) ;
#52377=CARTESIAN_POINT('Ctrl Pts',(31.2649083917971,586.652293270558,-47.6253014502317)) ;
#52378=CARTESIAN_POINT('Ctrl Pts',(31.2940874544249,586.606534862519,-47.6289347067773)) ;
#52379=CARTESIAN_POINT('Ctrl Pts',(31.2967009856576,586.602436340572,-47.6292601329083)) ;
#52380=CARTESIAN_POINT('Ctrl Pts',(31.2992957374993,586.598326833112,-47.6295863845744)) ;
#52381=CARTESIAN_POINT('Ctrl Pts',(31.3018716034924,586.594206508618,-47.6299134979525)) ;
#52382=CARTESIAN_POINT('Ctrl Pts',(31.3018890076405,586.59417866915,-47.6299157081333)) ;
#52383=CARTESIAN_POINT('Ctrl Pts',(31.3019064109265,586.594150829189,-47.6299179183535)) ;
#52384=CARTESIAN_POINT('Ctrl Pts',(31.3019238133503,586.594122988734,-47.629920128613)) ;
#52385=CARTESIAN_POINT('Ctrl Pts',(31.331784986765,586.546350984788,-47.6337127579626)) ;
#52386=CARTESIAN_POINT('Ctrl Pts',(31.3592023676582,586.496958448299,-47.6376306020833)) ;
#52387=CARTESIAN_POINT('Ctrl Pts',(31.3840375644497,586.44622538852,-47.6416083928178)) ;
#52388=CARTESIAN_POINT('Ctrl Pts',(31.3866785765017,586.440830358899,-47.6420313970467)) ;
#52389=CARTESIAN_POINT('Ctrl Pts',(31.3892903905504,586.43542021845,-47.6424550791829)) ;
#52390=CARTESIAN_POINT('Ctrl Pts',(31.391872843012,586.429995338376,-47.642879360737)) ;
#52391=CARTESIAN_POINT('Ctrl Pts',(31.4142029661715,586.383087121489,-47.6465480669371)) ;
#52392=CARTESIAN_POINT('Ctrl Pts',(31.4343386697815,586.335072588071,-47.6502614936775)) ;
#52393=CARTESIAN_POINT('Ctrl Pts',(31.4521967054837,586.286174104269,-47.6539767957637)) ;
#52394=CARTESIAN_POINT('Origin',(29.8885276254157,585.710565160562,-48.522160171753)) ;
#52395=CARTESIAN_POINT('',(31.4519519011282,586.286117533603,-48.355726152802)) ;
#52396=CARTESIAN_POINT('',(31.4519307013587,586.286106548708,-48.1612775350459)) ;
#52397=CARTESIAN_POINT('',(31.4519519036773,586.286117526679,-48.5221601717531)) ;
#52398=CARTESIAN_POINT('',(31.5236569526671,585.391334705933,-47.522160171753)) ;
#52399=CARTESIAN_POINT('Ctrl Pts',(31.4519307013587,586.286106548708,-48.1612775350459)) ;
#52400=CARTESIAN_POINT('Ctrl Pts',(31.4307799415804,586.343123822471,-48.1569517643851)) ;
#52401=CARTESIAN_POINT('Ctrl Pts',(31.4064967643115,586.399036969702,-48.1526486462426)) ;
#52402=CARTESIAN_POINT('Ctrl Pts',(31.3792408298284,586.453499502786,-48.1484091084437)) ;
#52403=CARTESIAN_POINT('Ctrl Pts',(31.3519986288077,586.507934593803,-48.144171706823)) ;
#52404=CARTESIAN_POINT('Ctrl Pts',(31.3217867261071,586.560920578791,-48.1399979131416)) ;
#52405=CARTESIAN_POINT('Ctrl Pts',(31.2887947141343,586.612128861891,-48.1359042980891)) ;
#52406=CARTESIAN_POINT('Ctrl Pts',(31.2558070590083,586.663330382545,-48.1318112236296)) ;
#52407=CARTESIAN_POINT('Ctrl Pts',(31.2200399857983,586.712754605879,-48.1277982748074)) ;
#52408=CARTESIAN_POINT('Ctrl Pts',(31.1817130950373,586.760090581968,-48.1238572931125)) ;
#52409=CARTESIAN_POINT('Ctrl Pts',(31.1433492593098,586.807472187274,-48.1199125125329)) ;
#52410=CARTESIAN_POINT('Ctrl Pts',(31.1024205399601,586.852761339475,-48.11603968801)) ;
#52411=CARTESIAN_POINT('Ctrl Pts',(31.059178620734,586.895665555711,-48.1122072045106)) ;
#52412=CARTESIAN_POINT('Ctrl Pts',(31.0159161277447,586.938590185037,-48.1083728975813)) ;
#52413=CARTESIAN_POINT('Ctrl Pts',(30.9703380380091,586.979127289515,-48.1045786603127)) ;
#52414=CARTESIAN_POINT('Ctrl Pts',(30.9227303036629,587.017007018988,-48.1007727915254)) ;
#52415=CARTESIAN_POINT('Ctrl Pts',(30.8750327440127,587.054958219163,-48.0969597419024)) ;
#52416=CARTESIAN_POINT('Ctrl Pts',(30.825297653982,587.090241462823,-48.0931344909291)) ;
#52417=CARTESIAN_POINT('Ctrl Pts',(30.7738498578355,587.12261490586,-48.0892311392184)) ;
#52418=CARTESIAN_POINT('Ctrl Pts',(30.7324088206022,587.148691611934,-48.0860870017491)) ;
#52419=CARTESIAN_POINT('Ctrl Pts',(30.6898572447864,587.172880722555,-48.0828917299347)) ;
#52420=CARTESIAN_POINT('Ctrl Pts',(30.6463835469031,587.195074223284,-48.0796086475328)) ;
#52421=CARTESIAN_POINT('Ctrl Pts',(30.6463569495885,587.195087801322,-48.079606638935)) ;
#52422=CARTESIAN_POINT('Ctrl Pts',(30.6463303519284,587.195101378614,-48.0796046303043)) ;
#52423=CARTESIAN_POINT('Ctrl Pts',(30.6463037539227,587.19511495516,-48.0796026216407)) ;
#52424=CARTESIAN_POINT('Ctrl Pts',(30.5969598112004,587.22030181766,-48.0758762001295)) ;
#52425=CARTESIAN_POINT('Ctrl Pts',(30.5462426003204,587.243005533324,-48.0720268035916)) ;
#52426=CARTESIAN_POINT('Ctrl Pts',(30.4944371047044,587.263110400219,-48.0681175601719)) ;
#52427=CARTESIAN_POINT('Ctrl Pts',(30.4895940946485,587.264989893338,-48.0677521065657)) ;
#52428=CARTESIAN_POINT('Ctrl Pts',(30.48474161048,587.266846682069,-48.0673861299368)) ;
#52429=CARTESIAN_POINT('Ctrl Pts',(30.4798799075965,587.268680677295,-48.0670196818603)) ;
#52430=CARTESIAN_POINT('Ctrl Pts',(30.4223039395851,587.290400237913,-48.0626799261751)) ;
#52431=CARTESIAN_POINT('Ctrl Pts',(30.3634290732152,587.308922130295,-48.0582747193363)) ;
#52432=CARTESIAN_POINT('Ctrl Pts',(30.3036482873888,587.324138482308,-48.0538756019817)) ;
#52433=CARTESIAN_POINT('Ctrl Pts',(30.2447665225575,587.339126001264,-48.0495426413161)) ;
#52434=CARTESIAN_POINT('Ctrl Pts',(30.1850058966653,587.350907103944,-48.045215873412)) ;
#52435=CARTESIAN_POINT('Ctrl Pts',(30.1247435266456,587.359417808461,-48.040943152075)) ;
#52436=CARTESIAN_POINT('Ctrl Pts',(30.0645180032693,587.367923309218,-48.036673043238)) ;
#52437=CARTESIAN_POINT('Ctrl Pts',(30.0037913375607,587.373162539151,-48.0324570503659)) ;
#52438=CARTESIAN_POINT('Ctrl Pts',(29.9429416361881,587.375106883817,-48.0283191850485)) ;
#52439=CARTESIAN_POINT('Ctrl Pts',(29.8821064426302,587.377050764912,-48.024182306283)) ;
#52440=CARTESIAN_POINT('Ctrl Pts',(29.8211482924624,587.375701301232,-48.0201235209901)) ;
#52441=CARTESIAN_POINT('Ctrl Pts',(29.7604466594093,587.371064453128,-48.0161420673551)) ;
#52442=CARTESIAN_POINT('Ctrl Pts',(29.6980479193189,587.366297967202,-48.0120492995323)) ;
#52443=CARTESIAN_POINT('Ctrl Pts',(29.6359203077301,587.358057352657,-48.0080382404948)) ;
#52444=CARTESIAN_POINT('Ctrl Pts',(29.5744771200985,587.346388751218,-48.0040817200879)) ;
#52445=CARTESIAN_POINT('Ctrl Pts',(29.514627676142,587.335022815711,-48.0002278258568)) ;
#52446=CARTESIAN_POINT('Ctrl Pts',(29.4554277481429,587.320404294539,-47.9964253109212)) ;
#52447=CARTESIAN_POINT('Ctrl Pts',(29.3972588143385,587.302615983661,-47.9926275534585)) ;
#52448=CARTESIAN_POINT('Ctrl Pts',(29.3367663910192,587.284117139666,-47.9886780990492)) ;
#52449=CARTESIAN_POINT('Ctrl Pts',(29.2773893147356,587.262189397615,-47.9847333742759)) ;
#52450=CARTESIAN_POINT('Ctrl Pts',(29.2195525913832,587.236977680796,-47.980722871614)) ;
#52451=CARTESIAN_POINT('Ctrl Pts',(29.1694833278862,587.215151892275,-47.9772509786211)) ;
#52452=CARTESIAN_POINT('Ctrl Pts',(29.1205675372531,587.190864738412,-47.9737291323648)) ;
#52453=CARTESIAN_POINT('Ctrl Pts',(29.0730774892506,587.164249422843,-47.9701065357073)) ;
#52454=CARTESIAN_POINT('Ctrl Pts',(29.0657368158185,587.160135416897,-47.9695465805134)) ;
#52455=CARTESIAN_POINT('Ctrl Pts',(29.0584301072712,587.155965801168,-47.9689842181129)) ;
#52456=CARTESIAN_POINT('Ctrl Pts',(29.0511582586619,587.15174108262,-47.9684192609029)) ;
#52457=CARTESIAN_POINT('Ctrl Pts',(29.051131846989,587.151725738257,-47.9684172089536)) ;
#52458=CARTESIAN_POINT('Ctrl Pts',(29.0511054357758,587.151710393167,-47.96841515697)) ;
#52459=CARTESIAN_POINT('Ctrl Pts',(29.0510790250225,587.15169504735,-47.9684131049522)) ;
#52460=CARTESIAN_POINT('Ctrl Pts',(29.0030794916229,587.123805193757,-47.9646837187795)) ;
#52461=CARTESIAN_POINT('Ctrl Pts',(28.9564309626375,587.093407305578,-47.9608314366137)) ;
#52462=CARTESIAN_POINT('Ctrl Pts',(28.9113857090435,587.060679387765,-47.9569193612993)) ;
#52463=CARTESIAN_POINT('Ctrl Pts',(28.9071765430953,587.057621191258,-47.9565538050445)) ;
#52464=CARTESIAN_POINT('Ctrl Pts',(28.9029813896465,587.054542684994,-47.9561877266996)) ;
#52465=CARTESIAN_POINT('Ctrl Pts',(28.8988004622044,587.051444036078,-47.9558211777507)) ;
#52466=CARTESIAN_POINT('Ctrl Pts',(28.8493826163757,587.01481853694,-47.9514886319951)) ;
#52467=CARTESIAN_POINT('Ctrl Pts',(28.8019497425696,586.975373500213,-47.9470909996863)) ;
#52468=CARTESIAN_POINT('Ctrl Pts',(28.7568040004953,586.933380274201,-47.9426992373383)) ;
#52469=CARTESIAN_POINT('Ctrl Pts',(28.7122319909216,586.89192071709,-47.9383632874918)) ;
#52470=CARTESIAN_POINT('Ctrl Pts',(28.6698889901391,586.84797757195,-47.9340333518222)) ;
#52471=CARTESIAN_POINT('Ctrl Pts',(28.6300337605279,586.801834383049,-47.9297571682477)) ;
#52472=CARTESIAN_POINT('Ctrl Pts',(28.5902028650029,586.755719367423,-47.925483595548)) ;
#52473=CARTESIAN_POINT('Ctrl Pts',(28.5528565856751,586.707407050929,-47.9212638443896)) ;
#52474=CARTESIAN_POINT('Ctrl Pts',(28.5182244800743,586.657200914689,-47.9171217491355)) ;
#52475=CARTESIAN_POINT('Ctrl Pts',(28.4836007390349,586.607006904549,-47.9129806543059)) ;
#52476=CARTESIAN_POINT('Ctrl Pts',(28.4516898961422,586.554919985649,-47.9089171797078)) ;
#52477=CARTESIAN_POINT('Ctrl Pts',(28.4226932061505,586.501263517939,-47.9049303377222)) ;
#52478=CARTESIAN_POINT('Ctrl Pts',(28.3930074424623,586.446331964673,-47.9008487529248)) ;
#52479=CARTESIAN_POINT('Ctrl Pts',(28.3663762908088,586.389755253745,-47.8968474592338)) ;
#52480=CARTESIAN_POINT('Ctrl Pts',(28.3429834443105,586.331902521544,-47.8928994043826)) ;
#52481=CARTESIAN_POINT('Ctrl Pts',(28.320104812319,586.27532149068,-47.8890381344841)) ;
#52482=CARTESIAN_POINT('Ctrl Pts',(28.300323889067,586.217519948497,-47.8852274348512)) ;
#52483=CARTESIAN_POINT('Ctrl Pts',(28.2837785816813,586.158864668577,-47.8814205514702)) ;
#52484=CARTESIAN_POINT('Ctrl Pts',(28.2666754719051,586.098231906186,-47.8774853242271)) ;
#52485=CARTESIAN_POINT('Ctrl Pts',(28.2530306485098,586.036686735904,-47.8735537450999)) ;
#52486=CARTESIAN_POINT('Ctrl Pts',(28.2429516138147,585.974658674776,-47.8695565520771)) ;
#52487=CARTESIAN_POINT('Ctrl Pts',(28.2341794744453,585.920673465528,-47.8660776540136)) ;
#52488=CARTESIAN_POINT('Ctrl Pts',(28.2281080884414,585.866321616251,-47.862548405409)) ;
#52489=CARTESIAN_POINT('Ctrl Pts',(28.2247736387295,585.811904521213,-47.8589182141461)) ;
#52490=CARTESIAN_POINT('Ctrl Pts',(28.2242788682371,585.803830033596,-47.8583795610927)) ;
#52491=CARTESIAN_POINT('Ctrl Pts',(28.223844294058,585.795754040162,-47.8578386855792)) ;
#52492=CARTESIAN_POINT('Ctrl Pts',(28.2234699704405,585.787677451147,-47.857295422325)) ;
#52493=CARTESIAN_POINT('Ctrl Pts',(28.2234684541509,585.787644734943,-47.857293221704)) ;
#52494=CARTESIAN_POINT('Ctrl Pts',(28.2234669388499,585.787612018729,-47.8572910210438)) ;
#52495=CARTESIAN_POINT('Ctrl Pts',(28.2234654245374,585.787579302505,-47.8572888203444)) ;
#52496=CARTESIAN_POINT('Ctrl Pts',(28.2208975126388,585.732100408197,-47.8535569602791)) ;
#52497=CARTESIAN_POINT('Ctrl Pts',(28.2211715555489,585.6763966939,-47.8497027637132)) ;
#52498=CARTESIAN_POINT('Ctrl Pts',(28.2242746982778,585.62077759501,-47.8457897027703)) ;
#52499=CARTESIAN_POINT('Ctrl Pts',(28.224556744825,585.615722340975,-47.8454340422595)) ;
#52500=CARTESIAN_POINT('Ctrl Pts',(28.2248621419837,585.610667814763,-47.8450778954639)) ;
#52501=CARTESIAN_POINT('Ctrl Pts',(28.2251908671879,585.605614265628,-47.8447213100422)) ;
#52502=CARTESIAN_POINT('Ctrl Pts',(28.2291850993401,585.544210247373,-47.8403885575222)) ;
#52503=CARTESIAN_POINT('Ctrl Pts',(28.2366266261737,585.482945411913,-47.8359917090826)) ;
#52504=CARTESIAN_POINT('Ctrl Pts',(28.2474511325718,585.422221922197,-47.8316017875513)) ;
#52505=CARTESIAN_POINT('Ctrl Pts',(28.2581147419081,585.3624010354,-47.827277118462)) ;
#52506=CARTESIAN_POINT('Ctrl Pts',(28.2720610984026,585.303105348989,-47.8229594508306)) ;
#52507=CARTESIAN_POINT('Ctrl Pts',(28.2891925640849,585.244704728804,-47.818695940337)) ;
#52508=CARTESIAN_POINT('Ctrl Pts',(28.3063140801705,585.186338026478,-47.8144349060011)) ;
#52509=CARTESIAN_POINT('Ctrl Pts',(28.3266168980108,585.128865287691,-47.8102280971683)) ;
#52510=CARTESIAN_POINT('Ctrl Pts',(28.3499707951118,585.072642760978,-47.8060986683029)) ;
#52511=CARTESIAN_POINT('Ctrl Pts',(28.3733198454859,585.01643190235,-47.8019700964341)) ;
#52512=CARTESIAN_POINT('Ctrl Pts',(28.3997187320752,584.961470768536,-47.7979188721716)) ;
#52513=CARTESIAN_POINT('Ctrl Pts',(28.4290051501343,584.908102651446,-47.7939432696954)) ;
#52514=CARTESIAN_POINT('Ctrl Pts',(28.4590986110284,584.853263874598,-47.7898581119473)) ;
#52515=CARTESIAN_POINT('Ctrl Pts',(28.4922412383819,584.800107328767,-47.7858527879754)) ;
#52516=CARTESIAN_POINT('Ctrl Pts',(28.5282203181192,584.748990154992,-47.7818990589373)) ;
#52517=CARTESIAN_POINT('Ctrl Pts',(28.563282523068,584.699175628429,-47.7780460849631)) ;
#52518=CARTESIAN_POINT('Ctrl Pts',(28.6010385236517,584.651298038033,-47.7742417386034)) ;
#52519=CARTESIAN_POINT('Ctrl Pts',(28.6412549150907,584.605670911219,-47.7704383928721)) ;
#52520=CARTESIAN_POINT('Ctrl Pts',(28.683048791265,584.558254064007,-47.7664858612089)) ;
#52521=CARTESIAN_POINT('Ctrl Pts',(28.7275004729346,584.513268348445,-47.7625339815812)) ;
#52522=CARTESIAN_POINT('Ctrl Pts',(28.7743022676147,584.471040595246,-47.7585114229537)) ;
#52523=CARTESIAN_POINT('Ctrl Pts',(28.8146927457334,584.434597566655,-47.7550399093646)) ;
#52524=CARTESIAN_POINT('Ctrl Pts',(28.8568341583957,584.400207859665,-47.7515150920462)) ;
#52525=CARTESIAN_POINT('Ctrl Pts',(28.9004946041224,584.368062445012,-47.7478863622271)) ;
#52526=CARTESIAN_POINT('Ctrl Pts',(28.9073968524377,584.362980599638,-47.7473126989522)) ;
#52527=CARTESIAN_POINT('Ctrl Pts',(28.9143370917191,584.357954741647,-47.7467364386732)) ;
#52528=CARTESIAN_POINT('Ctrl Pts',(28.9213144393905,584.352985510748,-47.7461573814348)) ;
#52529=CARTESIAN_POINT('Ctrl Pts',(28.9213428665735,584.352965265055,-47.7461550222338)) ;
#52530=CARTESIAN_POINT('Ctrl Pts',(28.9213712943725,584.352945020302,-47.7461526629863)) ;
#52531=CARTESIAN_POINT('Ctrl Pts',(28.9213997227874,584.352924776489,-47.7461503036923)) ;
#52532=CARTESIAN_POINT('Ctrl Pts',(28.966188167755,584.321031021641,-47.7424332794709)) ;
#52533=CARTESIAN_POINT('Ctrl Pts',(29.012678507572,584.291357561665,-47.7385907161729)) ;
#52534=CARTESIAN_POINT('Ctrl Pts',(29.0606107579876,584.264058947249,-47.7346854302868)) ;
#52535=CARTESIAN_POINT('Ctrl Pts',(29.0652818423194,584.261398647994,-47.7343048531272)) ;
#52536=CARTESIAN_POINT('Ctrl Pts',(29.0699665795344,584.258760899231,-47.7339236803004)) ;
#52537=CARTESIAN_POINT('Ctrl Pts',(29.0746647027699,584.256145841362,-47.733541969942)) ;
#52538=CARTESIAN_POINT('Ctrl Pts',(29.1284270591468,584.226220770002,-47.7291739175751)) ;
#52539=CARTESIAN_POINT('Ctrl Pts',(29.183948470999,584.199267172114,-47.7247361715027)) ;
#52540=CARTESIAN_POINT('Ctrl Pts',(29.2408544318338,584.175450784657,-47.7203020289527)) ;
#52541=CARTESIAN_POINT('Ctrl Pts',(29.29669672858,584.152079563851,-47.7159507676707)) ;
#52542=CARTESIAN_POINT('Ctrl Pts',(29.3538722052045,584.131728897117,-47.7116032602347)) ;
#52543=CARTESIAN_POINT('Ctrl Pts',(29.4120195720763,584.114516711758,-47.7073085328236)) ;
#52544=CARTESIAN_POINT('Ctrl Pts',(29.4701302786454,584.097315378204,-47.7030165131192)) ;
#52545=CARTESIAN_POINT('Ctrl Pts',(29.5292116364245,584.083248435898,-47.6987773495737)) ;
#52546=CARTESIAN_POINT('Ctrl Pts',(29.5888962456398,584.072398855542,-47.6946164046111)) ;
#52547=CARTESIAN_POINT('Ctrl Pts',(29.648565919294,584.0615519902,-47.6904565008893)) ;
#52548=CARTESIAN_POINT('Ctrl Pts',(29.7088385196163,584.053920903689,-47.686374787176)) ;
#52549=CARTESIAN_POINT('Ctrl Pts',(29.7693403765114,584.049554530518,-47.6823719266044)) ;
#52550=CARTESIAN_POINT('Ctrl Pts',(29.8319369391989,584.045036984016,-47.6782304782992)) ;
#52551=CARTESIAN_POINT('Ctrl Pts',(29.8947788908135,584.044014527707,-47.6741734692833)) ;
#52552=CARTESIAN_POINT('Ctrl Pts',(29.9574456165983,584.046501475673,-47.6701746338271)) ;
#52553=CARTESIAN_POINT('Ctrl Pts',(30.0180948327723,584.048908358159,-47.666304537967)) ;
#52554=CARTESIAN_POINT('Ctrl Pts',(30.078579797218,584.054602405714,-47.662488549878)) ;
#52555=CARTESIAN_POINT('Ctrl Pts',(30.1385141518014,584.063556938655,-47.6586810573511)) ;
#52556=CARTESIAN_POINT('Ctrl Pts',(30.2014391007573,584.072958283379,-47.6546835792007)) ;
#52557=CARTESIAN_POINT('Ctrl Pts',(30.2637569006503,584.085954563593,-47.6506950903516)) ;
#52558=CARTESIAN_POINT('Ctrl Pts',(30.3250171285409,584.102461888914,-47.6466435972635)) ;
#52559=CARTESIAN_POINT('Ctrl Pts',(30.3778105795844,584.116687736601,-47.6431520610848)) ;
#52560=CARTESIAN_POINT('Ctrl Pts',(30.4298195954929,584.133521283782,-47.6396130697671)) ;
#52561=CARTESIAN_POINT('Ctrl Pts',(30.4807536481331,584.15286909452,-47.6359748345754)) ;
#52562=CARTESIAN_POINT('Ctrl Pts',(30.4889046723152,584.155965342806,-47.6353926043878)) ;
#52563=CARTESIAN_POINT('Ctrl Pts',(30.4970282706236,584.159125949638,-47.6348078325743)) ;
#52564=CARTESIAN_POINT('Ctrl Pts',(30.5051233723068,584.162350499438,-47.6342203068854)) ;
#52565=CARTESIAN_POINT('Ctrl Pts',(30.5051408025854,584.162357442501,-47.6342190418319)) ;
#52566=CARTESIAN_POINT('Ctrl Pts',(30.5051582327318,584.16236438586,-47.6342177767657)) ;
#52567=CARTESIAN_POINT('Ctrl Pts',(30.5051756627462,584.162371329516,-47.6342165116867)) ;
#52568=CARTESIAN_POINT('Ctrl Pts',(30.5573892114869,584.183171823977,-47.630426826679)) ;
#52569=CARTESIAN_POINT('Ctrl Pts',(30.6085975773506,584.206713047159,-47.626512651755)) ;
#52570=CARTESIAN_POINT('Ctrl Pts',(30.6585215269897,584.2328521311,-47.6225363273908)) ;
#52571=CARTESIAN_POINT('Ctrl Pts',(30.6635495891892,584.235484714076,-47.6221358541436)) ;
#52572=CARTESIAN_POINT('Ctrl Pts',(30.6685646018945,584.238143610051,-47.6217347504899)) ;
#52573=CARTESIAN_POINT('Ctrl Pts',(30.6735662663411,584.240828647163,-47.6213330801159)) ;
#52574=CARTESIAN_POINT('Ctrl Pts',(30.7281138703226,584.27011136747,-47.6169525070642)) ;
#52575=CARTESIAN_POINT('Ctrl Pts',(30.7810772240688,584.302508244197,-47.6125051654418)) ;
#52576=CARTESIAN_POINT('Ctrl Pts',(30.832118315781,584.337794643179,-47.60806028493)) ;
#52577=CARTESIAN_POINT('Ctrl Pts',(30.8830961268198,584.373037294134,-47.6036209151749)) ;
#52578=CARTESIAN_POINT('Ctrl Pts',(30.9321567446921,584.411162079793,-47.5991843410106)) ;
#52579=CARTESIAN_POINT('Ctrl Pts',(30.9789917031901,584.451918727176,-47.5947989528455)) ;
#52580=CARTESIAN_POINT('Ctrl Pts',(31.0257833074872,584.49263764693,-47.5904176241481)) ;
#52581=CARTESIAN_POINT('Ctrl Pts',(31.070353511841,584.535983515777,-47.5860875232072)) ;
#52582=CARTESIAN_POINT('Ctrl Pts',(31.112419599329,584.581682212606,-47.5818328533529)) ;
#52583=CARTESIAN_POINT('Ctrl Pts',(31.1544599489697,584.627352949001,-47.5775807866892)) ;
#52584=CARTESIAN_POINT('Ctrl Pts',(31.1939992242414,584.675373687706,-47.5734040517902)) ;
#52585=CARTESIAN_POINT('Ctrl Pts',(31.2307792211875,584.725446151378,-47.5693018382)) ;
#52586=CARTESIAN_POINT('Ctrl Pts',(31.2675624397705,584.775523001001,-47.5651992652882)) ;
#52587=CARTESIAN_POINT('Ctrl Pts',(31.3015857225035,584.827652045966,-47.5611710924071)) ;
#52588=CARTESIAN_POINT('Ctrl Pts',(31.332616267389,584.881509006654,-47.5571925755217)) ;
#52589=CARTESIAN_POINT('Ctrl Pts',(31.3636455912645,584.935363848142,-47.5532142151856)) ;
#52590=CARTESIAN_POINT('Ctrl Pts',(31.3916820678538,584.990946608284,-47.5492852144427)) ;
#52591=CARTESIAN_POINT('Ctrl Pts',(31.416522243606,585.047905215767,-47.5453600602187)) ;
#52592=CARTESIAN_POINT('Ctrl Pts',(31.4413870439082,585.104920287427,-47.5414310149129)) ;
#52593=CARTESIAN_POINT('Ctrl Pts',(31.4630486289947,585.163314038115,-47.5375053197114)) ;
#52594=CARTESIAN_POINT('Ctrl Pts',(31.4813391707566,585.222703536039,-47.5335224252991)) ;
#52595=CARTESIAN_POINT('Ctrl Pts',(31.4984177883923,585.278157909114,-47.529803435909)) ;
#52596=CARTESIAN_POINT('Ctrl Pts',(31.5125570804919,585.334480084893,-47.5260339239252)) ;
#52597=CARTESIAN_POINT('Ctrl Pts',(31.523656952667,585.391334705933,-47.522160171753)) ;
#52598=CARTESIAN_POINT('Origin',(29.8885276254157,585.710565160562,-47.522160171753)) ;
#52599=CARTESIAN_POINT('Ctrl Pts',(31.4519518985791,586.286117540527,-48.355726152802)) ;
#52600=CARTESIAN_POINT('Ctrl Pts',(31.4434820923154,586.30912483085,-48.3540957748191)) ;
#52601=CARTESIAN_POINT('Ctrl Pts',(31.4345047739506,586.331944217182,-48.3524484063256)) ;
#52602=CARTESIAN_POINT('Ctrl Pts',(31.3977455599149,586.419647652667,-48.3459926605691)) ;
#52603=CARTESIAN_POINT('Ctrl Pts',(31.3663605758364,586.482927804222,-48.3410625763967)) ;
#52604=CARTESIAN_POINT('Ctrl Pts',(31.2785534651235,586.63490332075,-48.328535319917)) ;
#52605=CARTESIAN_POINT('Ctrl Pts',(31.2175745308427,586.720616863932,-48.3208259901791)) ;
#52606=CARTESIAN_POINT('Ctrl Pts',(31.1122495956988,586.842470426917,-48.3091819134654)) ;
#52607=CARTESIAN_POINT('Ctrl Pts',(31.0734280608116,586.883048528962,-48.3051714342576)) ;
#52608=CARTESIAN_POINT('Ctrl Pts',(31.0107179042492,586.942293027323,-48.2991977981767)) ;
#52609=CARTESIAN_POINT('Ctrl Pts',(30.9882475352005,586.962396315996,-48.2971492841245)) ;
#52610=CARTESIAN_POINT('Ctrl Pts',(30.9328771429415,587.009290909575,-48.2923306471091)) ;
#52611=CARTESIAN_POINT('Ctrl Pts',(30.8994771595535,587.035456204803,-48.2896004631163)) ;
#52612=CARTESIAN_POINT('Ctrl Pts',(30.815785738447,587.096009165938,-48.2830759481163)) ;
#52613=CARTESIAN_POINT('Ctrl Pts',(30.7645373235593,587.128969438512,-48.2793399671403)) ;
#52614=CARTESIAN_POINT('Ctrl Pts',(30.6050431270322,587.219598301561,-48.268127635221)) ;
#52615=CARTESIAN_POINT('Ctrl Pts',(30.4921467594447,587.26819662629,-48.2607012196546)) ;
#52616=CARTESIAN_POINT('Ctrl Pts',(30.3256890081963,587.319011110516,-48.2495284044689)) ;
#52617=CARTESIAN_POINT('Ctrl Pts',(30.2757654955829,587.33175432779,-48.2461559803733)) ;
#52618=CARTESIAN_POINT('Ctrl Pts',(30.1687055260016,587.353854555756,-48.2388306597564)) ;
#52619=CARTESIAN_POINT('Ctrl Pts',(30.1115115655679,587.362587079098,-48.2348619921694)) ;
#52620=CARTESIAN_POINT('Ctrl Pts',(29.9858394415985,587.375130120162,-48.2260048679559)) ;
#52621=CARTESIAN_POINT('Ctrl Pts',(29.9173459661159,587.377722585799,-48.2210890939331)) ;
#52622=CARTESIAN_POINT('Ctrl Pts',(29.7352369839165,587.373389001206,-48.2078743745191)) ;
#52623=CARTESIAN_POINT('Ctrl Pts',(29.6221505526748,587.35905760391,-48.1995036984888)) ;
#52624=CARTESIAN_POINT('Ctrl Pts',(29.4802874975646,587.326088693546,-48.1893377525639)) ;
#52625=CARTESIAN_POINT('Ctrl Pts',(29.4493846048396,587.317963778217,-48.1871464048208)) ;
#52626=CARTESIAN_POINT('Ctrl Pts',(29.3834550593428,587.298585781513,-48.1825469955573)) ;
#52627=CARTESIAN_POINT('Ctrl Pts',(29.3485297743631,587.287051967299,-48.1801540135514)) ;
#52628=CARTESIAN_POINT('Ctrl Pts',(29.2153641266709,587.238129118544,-48.1710955704189)) ;
#52629=CARTESIAN_POINT('Ctrl Pts',(29.1203571942751,587.192631114113,-48.1647620970404)) ;
#52630=CARTESIAN_POINT('Ctrl Pts',(28.9502432465714,587.090382174046,-48.1526245190228)) ;
#52631=CARTESIAN_POINT('Ctrl Pts',(28.8744171500099,587.035649869731,-48.1468612904288)) ;
#52632=CARTESIAN_POINT('Ctrl Pts',(28.7653265369692,586.942034221644,-48.1376049626789)) ;
#52633=CARTESIAN_POINT('Ctrl Pts',(28.7285879982721,586.907492844215,-48.1342947388423)) ;
#52634=CARTESIAN_POINT('Ctrl Pts',(28.6520689312175,586.828714286352,-48.1269183641127)) ;
#52635=CARTESIAN_POINT('Ctrl Pts',(28.6129790806541,586.783906639688,-48.1228277465482)) ;
#52636=CARTESIAN_POINT('Ctrl Pts',(28.5318026543341,586.680144856249,-48.1135611775892)) ;
#52637=CARTESIAN_POINT('Ctrl Pts',(28.4909969376601,586.620341792121,-48.108350738309)) ;
#52638=CARTESIAN_POINT('Ctrl Pts',(28.398980177153,586.464614810847,-48.0952056364894)) ;
#52639=CARTESIAN_POINT('Ctrl Pts',(28.3530159852892,586.365965819127,-48.0872350874343)) ;
#52640=CARTESIAN_POINT('Ctrl Pts',(28.3066817501423,586.234284057102,-48.0775251205083)) ;
#52641=CARTESIAN_POINT('Ctrl Pts',(28.2972052233884,586.204742757341,-48.075405885814)) ;
#52642=CARTESIAN_POINT('Ctrl Pts',(28.2777097233127,586.137573634432,-48.0707402797996)) ;
#52643=CARTESIAN_POINT('Ctrl Pts',(28.26817368348,586.099826346297,-48.0682187418209)) ;
#52644=CARTESIAN_POINT('Ctrl Pts',(28.2488926753565,586.010420568848,-48.0624052876878)) ;
#52645=CARTESIAN_POINT('Ctrl Pts',(28.2402520817229,585.958566265076,-48.0591552791752)) ;
#52646=CARTESIAN_POINT('Ctrl Pts',(28.2180236567539,585.770763684508,-48.0475533311717)) ;
#52647=CARTESIAN_POINT('Ctrl Pts',(28.2187086349124,585.633694396307,-48.0393524164731)) ;
#52648=CARTESIAN_POINT('Ctrl Pts',(28.2427019025735,585.44696022208,-48.0272773716683)) ;
#52649=CARTESIAN_POINT('Ctrl Pts',(28.2516753408951,585.396012303652,-48.0238945161476)) ;
#52650=CARTESIAN_POINT('Ctrl Pts',(28.275567948487,585.289605813336,-48.0165927403749)) ;
#52651=CARTESIAN_POINT('Ctrl Pts',(28.2910137821265,585.23433642384,-48.012660232188)) ;
#52652=CARTESIAN_POINT('Ctrl Pts',(28.3307370662613,585.116103024297,-48.0039221943929)) ;
#52653=CARTESIAN_POINT('Ctrl Pts',(28.3560510063055,585.053594533359,-47.9990913492981)) ;
#52654=CARTESIAN_POINT('Ctrl Pts',(28.4356104065225,584.886948200739,-47.9857054012247)) ;
#52655=CARTESIAN_POINT('Ctrl Pts',(28.4971821595587,584.786728527473,-47.9770612025327)) ;
#52656=CARTESIAN_POINT('Ctrl Pts',(28.5880558327149,584.668774692363,-47.9666824044219)) ;
#52657=CARTESIAN_POINT('Ctrl Pts',(28.6080493415936,584.644295841396,-47.9645182147761)) ;
#52658=CARTESIAN_POINT('Ctrl Pts',(28.6533595746993,584.591935417487,-47.9598898545011)) ;
#52659=CARTESIAN_POINT('Ctrl Pts',(28.6789483862941,584.564314205919,-47.957444546878)) ;
#52660=CARTESIAN_POINT('Ctrl Pts',(28.7404506589192,584.502282894467,-47.9518769547255)) ;
#52661=CARTESIAN_POINT('Ctrl Pts',(28.7770125723721,584.468566065907,-47.9487913869087)) ;
#52662=CARTESIAN_POINT('Ctrl Pts',(28.9300296203272,584.339634161256,-47.936488708907)) ;
#52663=CARTESIAN_POINT('Ctrl Pts',(29.0576059344332,584.25876059873,-47.9274946523805)) ;
#52664=CARTESIAN_POINT('Ctrl Pts',(29.2401925518158,584.175063157958,-47.9145226693446)) ;
#52665=CARTESIAN_POINT('Ctrl Pts',(29.2870135986645,584.156124838573,-47.9111964579189)) ;
#52666=CARTESIAN_POINT('Ctrl Pts',(29.3930438224229,584.118745574372,-47.9036212642135)) ;
#52667=CARTESIAN_POINT('Ctrl Pts',(29.4525652720331,584.101425986229,-47.8993394303105)) ;
#52668=CARTESIAN_POINT('Ctrl Pts',(29.6704561507284,584.051001330273,-47.8835425147065)) ;
#52669=CARTESIAN_POINT('Ctrl Pts',(29.8324466201678,584.037678042522,-47.871471761408)) ;
#52670=CARTESIAN_POINT('Ctrl Pts',(30.0297368999949,584.050169926224,-47.857532286556)) ;
#52671=CARTESIAN_POINT('Ctrl Pts',(30.0655909462358,584.053609670541,-47.8550353021252)) ;
#52672=CARTESIAN_POINT('Ctrl Pts',(30.1333240279881,584.0623319556,-47.8504214657627)) ;
#52673=CARTESIAN_POINT('Ctrl Pts',(30.165214136751,584.067384476811,-47.8482954856133)) ;
#52674=CARTESIAN_POINT('Ctrl Pts',(30.235039137753,584.080537890546,-47.8437040606502)) ;
#52675=CARTESIAN_POINT('Ctrl Pts',(30.2728800108991,584.08904339965,-47.8412572218737)) ;
#52676=CARTESIAN_POINT('Ctrl Pts',(30.400986006455,584.122575253693,-47.833010927125)) ;
#52677=CARTESIAN_POINT('Ctrl Pts',(30.4894222289005,584.153885137202,-47.8273739750085)) ;
#52678=CARTESIAN_POINT('Ctrl Pts',(30.6495351696288,584.226261624706,-47.8165814671852)) ;
#52679=CARTESIAN_POINT('Ctrl Pts',(30.7217000115368,584.265535491428,-47.811468224425)) ;
#52680=CARTESIAN_POINT('Ctrl Pts',(30.8327702045291,584.337077130835,-47.8029241742964)) ;
#52681=CARTESIAN_POINT('Ctrl Pts',(30.8736191757821,584.366073755343,-47.799620470658)) ;
#52682=CARTESIAN_POINT('Ctrl Pts',(30.9624623585322,584.43536345828,-47.7920193414021)) ;
#52683=CARTESIAN_POINT('Ctrl Pts',(31.0096117297751,584.476610613006,-47.7876853302185)) ;
#52684=CARTESIAN_POINT('Ctrl Pts',(31.1407662981794,584.605080633558,-47.7746958260141)) ;
#52685=CARTESIAN_POINT('Ctrl Pts',(31.217720517408,584.6989139922,-47.7657921836445)) ;
#52686=CARTESIAN_POINT('Ctrl Pts',(31.3145920495733,584.847392708989,-47.7529620027299)) ;
#52687=CARTESIAN_POINT('Ctrl Pts',(31.3429517098784,584.896084763225,-47.748933560168)) ;
#52688=CARTESIAN_POINT('Ctrl Pts',(31.3826562844653,584.972968817756,-47.7429361312224)) ;
#52689=CARTESIAN_POINT('Ctrl Pts',(31.3957877698077,585.000187637959,-47.7408811769365)) ;
#52690=CARTESIAN_POINT('Ctrl Pts',(31.4256401872173,585.066626463372,-47.7360395404856)) ;
#52691=CARTESIAN_POINT('Ctrl Pts',(31.4416100700602,585.106158218874,-47.7332930325006)) ;
#52692=CARTESIAN_POINT('Ctrl Pts',(31.4767960265537,585.203897847987,-47.7267233752158)) ;
#52693=CARTESIAN_POINT('Ctrl Pts',(31.4943513299144,585.26263715905,-47.722958663885)) ;
#52694=CARTESIAN_POINT('Ctrl Pts',(31.5368042679642,585.439739969753,-47.7118059565235)) ;
#52695=CARTESIAN_POINT('Ctrl Pts',(31.5521019910453,585.559969909567,-47.7044627376934)) ;
#52696=CARTESIAN_POINT('Ctrl Pts',(31.5551863622036,585.732531768951,-47.6933701959639)) ;
#52697=CARTESIAN_POINT('Ctrl Pts',(31.5536999385663,585.78428131776,-47.6899780448717)) ;
#52698=CARTESIAN_POINT('Ctrl Pts',(31.5454131947141,585.894143126491,-47.6825877391369)) ;
#52699=CARTESIAN_POINT('Ctrl Pts',(31.5379559238235,585.952133936346,-47.6785727010562)) ;
#52700=CARTESIAN_POINT('Ctrl Pts',(31.5102876804173,586.103773434535,-47.6677499481555)) ;
#52701=CARTESIAN_POINT('Ctrl Pts',(31.4850246340391,586.196272217906,-47.6608060977828)) ;
#52702=CARTESIAN_POINT('Ctrl Pts',(31.4519662334624,586.286078599909,-47.653833696077)) ;
#52703=CARTESIAN_POINT('Origin',(29.8885276254157,585.710565160562,-48.522160171753)) ;
#52704=CARTESIAN_POINT('',(31.4519519036772,586.286117526679,-49.0537704297649)) ;
#52705=CARTESIAN_POINT('',(31.4519519037552,586.286117526467,-48.8631174034081)) ;
#52706=CARTESIAN_POINT('',(31.4519519036773,586.286117526679,-48.5221601717531)) ;
#52707=CARTESIAN_POINT('',(31.5549951295688,585.711651406811,-49.0928293408672)) ;
#52708=CARTESIAN_POINT('Ctrl Pts',(31.5545272840244,585.711631704242,-49.0925609297511)) ;
#52709=CARTESIAN_POINT('Ctrl Pts',(31.5544977221009,585.757809048348,-49.0892228343914)) ;
#52710=CARTESIAN_POINT('Ctrl Pts',(31.5525482815855,585.803968862486,-49.0859127753278)) ;
#52711=CARTESIAN_POINT('Ctrl Pts',(31.5460913158,585.880852396666,-49.080499904251)) ;
#52712=CARTESIAN_POINT('Ctrl Pts',(31.5426392122963,585.911638093734,-49.0783597445402)) ;
#52713=CARTESIAN_POINT('Ctrl Pts',(31.5338748303722,585.974031563823,-49.0741012708764)) ;
#52714=CARTESIAN_POINT('Ctrl Pts',(31.5285053045551,586.005616576846,-49.0719902830301)) ;
#52715=CARTESIAN_POINT('Ctrl Pts',(31.5052725851344,586.121878570276,-49.0643251078782)) ;
#52716=CARTESIAN_POINT('Ctrl Pts',(31.481757603648,586.20515364275,-49.0590354631716)) ;
#52717=CARTESIAN_POINT('Ctrl Pts',(31.4519519036772,586.286117526679,-49.0537704297648)) ;
#52718=CARTESIAN_POINT('',(28.6194567455633,586.789923813611,-49.5221601717529)) ;
#52719=CARTESIAN_POINT('Ctrl Pts',(31.5549951295688,585.711651406811,-49.0928293408672)) ;
#52720=CARTESIAN_POINT('Ctrl Pts',(31.5549004634924,585.651788058804,-49.0970785373116)) ;
#52721=CARTESIAN_POINT('Ctrl Pts',(31.5515533777371,585.591824499677,-49.1013669242796)) ;
#52722=CARTESIAN_POINT('Ctrl Pts',(31.5449787198106,585.532138025659,-49.1056345435034)) ;
#52723=CARTESIAN_POINT('Ctrl Pts',(31.5384111864713,585.472516230519,-49.1098975381481)) ;
#52724=CARTESIAN_POINT('Ctrl Pts',(31.5286233097781,585.413170884277,-49.1141395515163)) ;
#52725=CARTESIAN_POINT('Ctrl Pts',(31.5156767976258,585.354469497454,-49.1183211131778)) ;
#52726=CARTESIAN_POINT('Ctrl Pts',(31.5027392387105,585.295808705922,-49.1224997830556)) ;
#52727=CARTESIAN_POINT('Ctrl Pts',(31.486647481512,585.237791002754,-49.1266179865489)) ;
#52728=CARTESIAN_POINT('Ctrl Pts',(31.4674977847107,585.180774747157,-49.1306592310771)) ;
#52729=CARTESIAN_POINT('Ctrl Pts',(31.4483537584412,585.123775374985,-49.1346992789281)) ;
#52730=CARTESIAN_POINT('Ctrl Pts',(31.426153560656,585.06777695046,-49.1386624357151)) ;
#52731=CARTESIAN_POINT('Ctrl Pts',(31.4010278693363,585.013128286434,-49.1425556647614)) ;
#52732=CARTESIAN_POINT('Ctrl Pts',(31.3758819407826,584.958435606193,-49.1464520295697)) ;
#52733=CARTESIAN_POINT('Ctrl Pts',(31.3478056647439,584.905095035362,-49.1502784917524)) ;
#52734=CARTESIAN_POINT('Ctrl Pts',(31.3169659821272,584.853444993432,-49.1540643342011)) ;
#52735=CARTESIAN_POINT('Ctrl Pts',(31.2861148200487,584.801775725796,-49.1578515858547)) ;
#52736=CARTESIAN_POINT('Ctrl Pts',(31.2524979705717,584.751798528007,-49.1615984774341)) ;
#52737=CARTESIAN_POINT('Ctrl Pts',(31.216321245005,584.70383758609,-49.1653534658704)) ;
#52738=CARTESIAN_POINT('Ctrl Pts',(31.1800774948503,584.655787786977,-49.1691154111705)) ;
#52739=CARTESIAN_POINT('Ctrl Pts',(31.1412640853418,584.609762194078,-49.1728859737232)) ;
#52740=CARTESIAN_POINT('Ctrl Pts',(31.1001307191771,584.566066556702,-49.1767272898374)) ;
#52741=CARTESIAN_POINT('Ctrl Pts',(31.0641200442947,584.527812712244,-49.1800902138723)) ;
#52742=CARTESIAN_POINT('Ctrl Pts',(31.0263318317532,584.491344652427,-49.1835078935255)) ;
#52743=CARTESIAN_POINT('Ctrl Pts',(30.9869628963889,584.456849398685,-49.1870249440584)) ;
#52744=CARTESIAN_POINT('Ctrl Pts',(30.9869382635993,584.456827815314,-49.1870271446453)) ;
#52745=CARTESIAN_POINT('Ctrl Pts',(30.9869136301907,584.456806232714,-49.1870293452712)) ;
#52746=CARTESIAN_POINT('Ctrl Pts',(30.9868889961631,584.456784650885,-49.187031545936)) ;
#52747=CARTESIAN_POINT('Ctrl Pts',(30.9451149164525,584.420186451609,-49.1907634060781)) ;
#52748=CARTESIAN_POINT('Ctrl Pts',(30.9013931355104,584.385670009117,-49.1946176026786)) ;
#52749=CARTESIAN_POINT('Ctrl Pts',(30.8559735946312,584.3534182028,-49.1985306636151)) ;
#52750=CARTESIAN_POINT('Ctrl Pts',(30.851845386038,584.350486817291,-49.1988863240086)) ;
#52751=CARTESIAN_POINT('Ctrl Pts',(30.8477031876204,584.347574141802,-49.1992424706862)) ;
#52752=CARTESIAN_POINT('Ctrl Pts',(30.8435472083229,584.3446803141,-49.1995990559895)) ;
#52753=CARTESIAN_POINT('Ctrl Pts',(30.793049249511,584.309518350659,-49.2039318085532)) ;
#52754=CARTESIAN_POINT('Ctrl Pts',(30.740510754993,584.277138369889,-49.2083286569907)) ;
#52755=CARTESIAN_POINT('Ctrl Pts',(30.6862862482676,584.247740832729,-49.2127185784724)) ;
#52756=CARTESIAN_POINT('Ctrl Pts',(30.6328677448689,584.218780266124,-49.2170432473307)) ;
#52757=CARTESIAN_POINT('Ctrl Pts',(30.5778131003371,584.192713711564,-49.2213609146856)) ;
#52758=CARTESIAN_POINT('Ctrl Pts',(30.521472363694,584.169695440192,-49.2256244248628)) ;
#52759=CARTESIAN_POINT('Ctrl Pts',(30.4651643485759,584.146690537352,-49.2298854588822)) ;
#52760=CARTESIAN_POINT('Ctrl Pts',(30.4075717531272,584.126730253415,-49.2340922673582)) ;
#52761=CARTESIAN_POINT('Ctrl Pts',(30.349054296051,584.109934893663,-49.23822169583)) ;
#52762=CARTESIAN_POINT('Ctrl Pts',(30.2905489833374,584.093143019519,-49.2423502673049)) ;
#52763=CARTESIAN_POINT('Ctrl Pts',(30.231119203068,584.079514793908,-49.2464014911362)) ;
#52764=CARTESIAN_POINT('Ctrl Pts',(30.1711345470063,584.069137360875,-49.250377093143)) ;
#52765=CARTESIAN_POINT('Ctrl Pts',(30.1094968953937,584.0584739572,-49.2544622507071)) ;
#52766=CARTESIAN_POINT('Ctrl Pts',(30.0472733406778,584.051243342123,-49.2584675744432)) ;
#52767=CARTESIAN_POINT('Ctrl Pts',(29.9848757320995,584.04750188289,-49.2624213031963)) ;
#52768=CARTESIAN_POINT('Ctrl Pts',(29.9240682407258,584.043855769598,-49.2662742766118)) ;
#52769=CARTESIAN_POINT('Ctrl Pts',(29.8630955529396,584.043523410377,-49.2700786223735)) ;
#52770=CARTESIAN_POINT('Ctrl Pts',(29.8023483198256,584.046517803162,-49.2738819674629)) ;
#52771=CARTESIAN_POINT('Ctrl Pts',(29.7392182745368,584.049629651102,-49.2778344988859)) ;
#52772=CARTESIAN_POINT('Ctrl Pts',(29.6763318499431,584.056335241496,-49.281786378225)) ;
#52773=CARTESIAN_POINT('Ctrl Pts',(29.6141364158333,584.066597786271,-49.2858089365303)) ;
#52774=CARTESIAN_POINT('Ctrl Pts',(29.5604610580425,584.075454477611,-49.2892804495018)) ;
#52775=CARTESIAN_POINT('Ctrl Pts',(29.5072993619206,584.086960329732,-49.292805266168)) ;
#52776=CARTESIAN_POINT('Ctrl Pts',(29.4549452226018,584.101053103059,-49.2964339952949)) ;
#52777=CARTESIAN_POINT('Ctrl Pts',(29.4466685882797,584.103281021098,-49.2970076588949)) ;
#52778=CARTESIAN_POINT('Ctrl Pts',(29.4384120397071,584.105573549329,-49.2975839195019)) ;
#52779=CARTESIAN_POINT('Ctrl Pts',(29.4301766273081,584.107930396578,-49.2981629770717)) ;
#52780=CARTESIAN_POINT('Ctrl Pts',(29.4301430748617,584.107939998767,-49.298165336249)) ;
#52781=CARTESIAN_POINT('Ctrl Pts',(29.4301095227661,584.107949602025,-49.2981676954727)) ;
#52782=CARTESIAN_POINT('Ctrl Pts',(29.4300759710213,584.107959206349,-49.2981700547429)) ;
#52783=CARTESIAN_POINT('Ctrl Pts',(29.377215290868,584.123090793065,-49.3018870783155)) ;
#52784=CARTESIAN_POINT('Ctrl Pts',(29.3250293931448,584.140937305961,-49.3057296409284)) ;
#52785=CARTESIAN_POINT('Ctrl Pts',(29.2738012079945,584.161391841912,-49.3096349260873)) ;
#52786=CARTESIAN_POINT('Ctrl Pts',(29.2688089330185,584.16338517171,-49.3100155028599)) ;
#52787=CARTESIAN_POINT('Ctrl Pts',(29.2638257762798,584.165403235723,-49.3103966752985)) ;
#52788=CARTESIAN_POINT('Ctrl Pts',(29.2588520139343,584.167445912848,-49.3107783852673)) ;
#52789=CARTESIAN_POINT('Ctrl Pts',(29.201935368766,584.190821040376,-49.3151464369237)) ;
#52790=CARTESIAN_POINT('Ctrl Pts',(29.1462451621245,584.217424136405,-49.3195841822428)) ;
#52791=CARTESIAN_POINT('Ctrl Pts',(29.0921444734093,584.247065735209,-49.3240183239897)) ;
#52792=CARTESIAN_POINT('Ctrl Pts',(29.0390550187489,584.276153282025,-49.328369584072)) ;
#52793=CARTESIAN_POINT('Ctrl Pts',(28.9874959042153,584.308166435024,-49.3327170902622)) ;
#52794=CARTESIAN_POINT('Ctrl Pts',(28.9377845894302,584.342896253063,-49.3370118163971)) ;
#52795=CARTESIAN_POINT('Ctrl Pts',(28.8881046161158,584.377604175009,-49.341303834838)) ;
#52796=CARTESIAN_POINT('Ctrl Pts',(28.840270017296,584.415025243138,-49.3455429970899)) ;
#52797=CARTESIAN_POINT('Ctrl Pts',(28.7945747320282,584.45492394412,-49.3497039407454)) ;
#52798=CARTESIAN_POINT('Ctrl Pts',(28.7488908814825,584.49481266091,-49.3538638431724)) ;
#52799=CARTESIAN_POINT('Ctrl Pts',(28.7053453092586,584.537177769595,-49.3579455555769)) ;
#52800=CARTESIAN_POINT('Ctrl Pts',(28.66420925332,584.581757633295,-49.361948414843)) ;
#52801=CARTESIAN_POINT('Ctrl Pts',(28.6216489710894,584.627880955952,-49.3660898624418)) ;
#52802=CARTESIAN_POINT('Ctrl Pts',(28.5816682634495,584.676375284731,-49.3701468707268)) ;
#52803=CARTESIAN_POINT('Ctrl Pts',(28.5445405706483,584.726920694313,-49.3741457054608)) ;
#52804=CARTESIAN_POINT('Ctrl Pts',(28.5086081821852,584.775838824018,-49.3780158000512)) ;
#52805=CARTESIAN_POINT('Ctrl Pts',(28.4753482118881,584.826678049973,-49.3818317868948)) ;
#52806=CARTESIAN_POINT('Ctrl Pts',(28.4449806910114,584.87911967072,-49.3856392782212)) ;
#52807=CARTESIAN_POINT('Ctrl Pts',(28.4130978897292,584.934178026652,-49.3896367559816)) ;
#52808=CARTESIAN_POINT('Ctrl Pts',(28.3844042744588,584.9910031002,-49.393625244486)) ;
#52809=CARTESIAN_POINT('Ctrl Pts',(28.3591150911948,585.049190431488,-49.3976767373463)) ;
#52810=CARTESIAN_POINT('Ctrl Pts',(28.3373211325259,585.099335676587,-49.4011682723248)) ;
#52811=CARTESIAN_POINT('Ctrl Pts',(28.3180550420476,585.150493499069,-49.4047072625028)) ;
#52812=CARTESIAN_POINT('Ctrl Pts',(28.3014249098296,585.202378498608,-49.4083454966198)) ;
#52813=CARTESIAN_POINT('Ctrl Pts',(28.2987635686985,585.210681720828,-49.4089277278356)) ;
#52814=CARTESIAN_POINT('Ctrl Pts',(28.2961696451147,585.219003627598,-49.4095125006894)) ;
#52815=CARTESIAN_POINT('Ctrl Pts',(28.2936434817717,585.227343122656,-49.4101000274321)) ;
#52816=CARTESIAN_POINT('Ctrl Pts',(28.2936380424176,585.22736107932,-49.4101012924991)) ;
#52817=CARTESIAN_POINT('Ctrl Pts',(28.2936326033777,585.227379036065,-49.4101025575789)) ;
#52818=CARTESIAN_POINT('Ctrl Pts',(28.2936271646519,585.227396992892,-49.4101038226715)) ;
#52819=CARTESIAN_POINT('Ctrl Pts',(28.277335033442,585.281188082002,-49.4138935070696)) ;
#52820=CARTESIAN_POINT('Ctrl Pts',(28.2638124112331,585.335902103654,-49.4178076815085)) ;
#52821=CARTESIAN_POINT('Ctrl Pts',(28.2531216984605,585.391231667786,-49.4217840055249)) ;
#52822=CARTESIAN_POINT('Ctrl Pts',(28.2520449872732,585.396804164396,-49.4221844795292)) ;
#52823=CARTESIAN_POINT('Ctrl Pts',(28.2509969847544,585.402382864411,-49.4225855839438)) ;
#52824=CARTESIAN_POINT('Ctrl Pts',(28.249977742813,585.40796742709,-49.4229872550822)) ;
#52825=CARTESIAN_POINT('Ctrl Pts',(28.2388620219692,585.468871945688,-49.4273678285887)) ;
#52826=CARTESIAN_POINT('Ctrl Pts',(28.2311688113756,585.53047949232,-49.4318151708419)) ;
#52827=CARTESIAN_POINT('Ctrl Pts',(28.2269332318505,585.592385741501,-49.4362600521213)) ;
#52828=CARTESIAN_POINT('Ctrl Pts',(28.2227029035984,585.65421523929,-49.4406994226351)) ;
#52829=CARTESIAN_POINT('Ctrl Pts',(28.2219212701929,585.716342796566,-49.4451359976939)) ;
#52830=CARTESIAN_POINT('Ctrl Pts',(28.2245849858367,585.778371201992,-49.4495213868474)) ;
#52831=CARTESIAN_POINT('Ctrl Pts',(28.2272462357256,585.840342188806,-49.4539027165228)) ;
#52832=CARTESIAN_POINT('Ctrl Pts',(28.2333463380861,585.902214290954,-49.458232818535)) ;
#52833=CARTESIAN_POINT('Ctrl Pts',(28.242847247488,585.963595559647,-49.4624874895138)) ;
#52834=CARTESIAN_POINT('Ctrl Pts',(28.252342343799,586.024939272474,-49.4667395572903)) ;
#52835=CARTESIAN_POINT('Ctrl Pts',(28.2652341409681,586.085792768793,-49.4709162933552)) ;
#52836=CARTESIAN_POINT('Ctrl Pts',(28.2814504238792,586.145768203664,-49.4750185081275)) ;
#52837=CARTESIAN_POINT('Ctrl Pts',(28.2976681271212,586.205748891586,-49.4791210821994)) ;
#52838=CARTESIAN_POINT('Ctrl Pts',(28.3172110937834,586.264851297271,-49.4831492562576)) ;
#52839=CARTESIAN_POINT('Ctrl Pts',(28.3399709414953,586.322691223682,-49.4871277743043)) ;
#52840=CARTESIAN_POINT('Ctrl Pts',(28.3627298935716,586.380528874002,-49.4911061357901)) ;
#52841=CARTESIAN_POINT('Ctrl Pts',(28.3887057972037,586.437103961319,-49.4950351376672)) ;
#52842=CARTESIAN_POINT('Ctrl Pts',(28.417750243145,586.492037906295,-49.4989602929812)) ;
#52843=CARTESIAN_POINT('Ctrl Pts',(28.4468234812195,586.547026307999,-49.5028893393523)) ;
#52844=CARTESIAN_POINT('Ctrl Pts',(28.4789717865111,586.600369927032,-49.5068150355747)) ;
#52845=CARTESIAN_POINT('Ctrl Pts',(28.5140004099809,586.651698795954,-49.5107979309393)) ;
#52846=CARTESIAN_POINT('Ctrl Pts',(28.5467080078033,586.699626571443,-49.5145169163532)) ;
#52847=CARTESIAN_POINT('Ctrl Pts',(28.5819267144592,586.745797359943,-49.5182864241681)) ;
#52848=CARTESIAN_POINT('Ctrl Pts',(28.6194567455635,586.789923813611,-49.5221601717529)) ;
#52849=CARTESIAN_POINT('',(31.1430459483832,586.808139740278,-49.5221526322664)) ;
#52850=CARTESIAN_POINT('Origin',(29.8885276254156,585.710565160562,-49.522160171753)) ;
#52851=CARTESIAN_POINT('',(31.5540518914521,585.711428744506,-48.8998571438181)) ;
#52852=CARTESIAN_POINT('Ctrl Pts',(31.1430459605378,586.808139750912,-49.5221526321279)) ;
#52853=CARTESIAN_POINT('Ctrl Pts',(31.1082549275998,586.847858648898,-49.5185473794)) ;
#52854=CARTESIAN_POINT('Ctrl Pts',(31.0714734883611,586.885954048843,-49.5148450709363)) ;
#52855=CARTESIAN_POINT('Ctrl Pts',(31.0328944158098,586.922236962595,-49.5110998238165)) ;
#52856=CARTESIAN_POINT('Ctrl Pts',(30.9888444934954,586.963665110718,-49.5068234679126)) ;
#52857=CARTESIAN_POINT('Ctrl Pts',(30.9424499583342,587.002731060734,-49.5024916930553)) ;
#52858=CARTESIAN_POINT('Ctrl Pts',(30.8940141285388,587.039194414828,-49.4981706333717)) ;
#52859=CARTESIAN_POINT('Ctrl Pts',(30.8456276796615,587.075620594089,-49.493853979061)) ;
#52860=CARTESIAN_POINT('Ctrl Pts',(30.7952042286405,587.109449763238,-49.4895483160835)) ;
#52861=CARTESIAN_POINT('Ctrl Pts',(30.743063267547,587.140476495768,-49.485298818357)) ;
#52862=CARTESIAN_POINT('Ctrl Pts',(30.6909556806126,587.171483368843,-49.4810520406306)) ;
#52863=CARTESIAN_POINT('Ctrl Pts',(30.6371328205902,587.199691487015,-49.4768614744286)) ;
#52864=CARTESIAN_POINT('Ctrl Pts',(30.5819294674629,587.224927230988,-49.4727484139713)) ;
#52865=CARTESIAN_POINT('Ctrl Pts',(30.5267405036143,587.250156397024,-49.4686364256223)) ;
#52866=CARTESIAN_POINT('Ctrl Pts',(30.4701717770591,587.272414680804,-49.4646018931605)) ;
#52867=CARTESIAN_POINT('Ctrl Pts',(30.4125733656241,587.291559756921,-49.4606415192554)) ;
#52868=CARTESIAN_POINT('Ctrl Pts',(30.3549264352746,587.310720960189,-49.4566778092681)) ;
#52869=CARTESIAN_POINT('Ctrl Pts',(30.2962480859876,587.326763513427,-49.4527882588481)) ;
#52870=CARTESIAN_POINT('Ctrl Pts',(30.2369047928652,587.339577852312,-49.448945926886)) ;
#52871=CARTESIAN_POINT('Ctrl Pts',(30.1775392130304,587.352397003695,-49.4451021519142)) ;
#52872=CARTESIAN_POINT('Ctrl Pts',(30.1175082069774,587.361985176315,-49.4413053577402)) ;
#52873=CARTESIAN_POINT('Ctrl Pts',(30.057194073834,587.368269792658,-49.4375078690049)) ;
#52874=CARTESIAN_POINT('Ctrl Pts',(29.996765383819,587.374566345606,-49.4337031675583)) ;
#52875=CARTESIAN_POINT('Ctrl Pts',(29.9360525884205,587.377546250347,-49.4298972949997)) ;
#52876=CARTESIAN_POINT('Ctrl Pts',(29.8754548815714,587.377180281353,-49.4260270661981)) ;
#52877=CARTESIAN_POINT('Ctrl Pts',(29.8210016094304,587.376851420572,-49.4225492675629)) ;
#52878=CARTESIAN_POINT('Ctrl Pts',(29.7666408751731,587.373820856864,-49.4190189126796)) ;
#52879=CARTESIAN_POINT('Ctrl Pts',(29.7126726647831,587.368104063971,-49.4153856559798)) ;
#52880=CARTESIAN_POINT('Ctrl Pts',(29.7078388194358,587.367592020075,-49.4150602310515)) ;
#52881=CARTESIAN_POINT('Ctrl Pts',(29.7030080940045,587.367058444666,-49.4147339805939)) ;
#52882=CARTESIAN_POINT('Ctrl Pts',(29.6981806865841,587.366503359557,-49.4144068684306)) ;
#52883=CARTESIAN_POINT('Ctrl Pts',(29.6981480689928,587.366499608985,-49.4144046582151)) ;
#52884=CARTESIAN_POINT('Ctrl Pts',(29.698115451553,587.366495857431,-49.4144024479602)) ;
#52885=CARTESIAN_POINT('Ctrl Pts',(29.6980828342647,587.366492104895,-49.414400237666)) ;
#52886=CARTESIAN_POINT('Ctrl Pts',(29.6429112083997,587.360144749872,-49.4106615600452)) ;
#52887=CARTESIAN_POINT('Ctrl Pts',(29.58797454581,587.350956557579,-49.4068004115545)) ;
#52888=CARTESIAN_POINT('Ctrl Pts',(29.533575462541,587.338989812433,-49.4028798514077)) ;
#52889=CARTESIAN_POINT('Ctrl Pts',(29.5285116112468,587.337875863185,-49.4025148979493)) ;
#52890=CARTESIAN_POINT('Ctrl Pts',(29.5234524442729,587.336737863875,-49.4021494296769)) ;
#52891=CARTESIAN_POINT('Ctrl Pts',(29.5183982213193,587.335575881509,-49.4017834974551)) ;
#52892=CARTESIAN_POINT('Ctrl Pts',(29.4584472249493,587.321792951626,-49.3974429684558)) ;
#52893=CARTESIAN_POINT('Ctrl Pts',(29.3991873543754,587.304631710942,-49.3930378230853)) ;
#52894=CARTESIAN_POINT('Ctrl Pts',(29.3410040316313,587.284219960435,-49.3886388765359)) ;
#52895=CARTESIAN_POINT('Ctrl Pts',(29.2835610543231,587.264067936352,-49.3842959037578)) ;
#52896=CARTESIAN_POINT('Ctrl Pts',(29.2271671710291,587.240747966385,-49.3799592650711)) ;
#52897=CARTESIAN_POINT('Ctrl Pts',(29.1721729220915,587.21441638561,-49.3756765623397)) ;
#52898=CARTESIAN_POINT('Ctrl Pts',(29.1172118889562,587.188100708764,-49.3713964463043)) ;
#52899=CARTESIAN_POINT('Ctrl Pts',(29.0636487152697,587.15877715734,-49.3671703361583)) ;
#52900=CARTESIAN_POINT('Ctrl Pts',(29.0118151758906,587.126632032098,-49.3630219371472)) ;
#52901=CARTESIAN_POINT('Ctrl Pts',(28.9599938148718,587.094494459397,-49.358874512808)) ;
#52902=CARTESIAN_POINT('Ctrl Pts',(28.9099013067565,587.059536620886,-49.3548047650706)) ;
#52903=CARTESIAN_POINT('Ctrl Pts',(28.8618514567854,587.02197437252,-49.3508115819677)) ;
#52904=CARTESIAN_POINT('Ctrl Pts',(28.8126592671132,586.983519117254,-49.3467234647164)) ;
#52905=CARTESIAN_POINT('Ctrl Pts',(28.7656082490994,586.942333905959,-49.3427155690382)) ;
#52906=CARTESIAN_POINT('Ctrl Pts',(28.7210144421838,586.898683596496,-49.3387607110024)) ;
#52907=CARTESIAN_POINT('Ctrl Pts',(28.6774006108051,586.85599252865,-49.3348927633337)) ;
#52908=CARTESIAN_POINT('Ctrl Pts',(28.6361373799858,586.810943459451,-49.3310751940078)) ;
#52909=CARTESIAN_POINT('Ctrl Pts',(28.5974978886643,586.763817419732,-49.3272611266717)) ;
#52910=CARTESIAN_POINT('Ctrl Pts',(28.5575560895066,586.715103041019,-49.3233185097712)) ;
#52911=CARTESIAN_POINT('Ctrl Pts',(28.5204185737604,586.66416887415,-49.3193792044937)) ;
#52912=CARTESIAN_POINT('Ctrl Pts',(28.4863557060612,586.611365641621,-49.315373822326)) ;
#52913=CARTESIAN_POINT('Ctrl Pts',(28.4567183675625,586.565422731291,-49.3118888289846)) ;
#52914=CARTESIAN_POINT('Ctrl Pts',(28.4294080495839,586.518064194444,-49.3083531635697)) ;
#52915=CARTESIAN_POINT('Ctrl Pts',(28.4045783576044,586.469551626168,-49.3047162086791)) ;
#52916=CARTESIAN_POINT('Ctrl Pts',(28.4008846903444,586.462334892055,-49.3041751749354)) ;
#52917=CARTESIAN_POINT('Ctrl Pts',(28.3972458323923,586.455092581239,-49.3036318996998)) ;
#52918=CARTESIAN_POINT('Ctrl Pts',(28.3936622003196,586.447825511975,-49.3030862163398)) ;
#52919=CARTESIAN_POINT('Ctrl Pts',(28.3936486456252,586.447798025084,-49.3030841523525)) ;
#52920=CARTESIAN_POINT('Ctrl Pts',(28.3936350917208,586.447770537839,-49.3030820883307)) ;
#52921=CARTESIAN_POINT('Ctrl Pts',(28.3936215386065,586.44774305024,-49.3030800242744)) ;
#52922=CARTESIAN_POINT('Ctrl Pts',(28.369105706428,586.398021535994,-49.2993464132927)) ;
#52923=CARTESIAN_POINT('Ctrl Pts',(28.3470946232122,586.346959372583,-49.2954902524912)) ;
#52924=CARTESIAN_POINT('Ctrl Pts',(28.3277003414553,586.294843528449,-49.2915747618002)) ;
#52925=CARTESIAN_POINT('Ctrl Pts',(28.3259022254139,586.29001167458,-49.291211742086)) ;
#52926=CARTESIAN_POINT('Ctrl Pts',(28.3241265948477,586.28517079955,-49.2908482123818)) ;
#52927=CARTESIAN_POINT('Ctrl Pts',(28.3223735335455,586.280321154001,-49.290484223071)) ;
#52928=CARTESIAN_POINT('Ctrl Pts',(28.301455594047,586.222454043439,-49.2861410170623)) ;
#52929=CARTESIAN_POINT('Ctrl Pts',(28.2837519466565,586.163332258295,-49.2817330394404)) ;
#52930=CARTESIAN_POINT('Ctrl Pts',(28.269365237472,586.103349954343,-49.27733166919)) ;
#52931=CARTESIAN_POINT('Ctrl Pts',(28.2551945664532,586.044268375271,-49.272996392161)) ;
#52932=CARTESIAN_POINT('Ctrl Pts',(28.2442415172068,585.984351936258,-49.2686678082078)) ;
#52933=CARTESIAN_POINT('Ctrl Pts',(28.2365651414893,585.923978458449,-49.2643935745064)) ;
#52934=CARTESIAN_POINT('Ctrl Pts',(28.2288935295783,585.863642447223,-49.2601219933097)) ;
#52935=CARTESIAN_POINT('Ctrl Pts',(28.2244943989448,585.80284995105,-49.2559048289096)) ;
#52936=CARTESIAN_POINT('Ctrl Pts',(28.2233914542907,585.74197937957,-49.2517658773966)) ;
#52937=CARTESIAN_POINT('Ctrl Pts',(28.2222887826853,585.681123877412,-49.2476279505364)) ;
#52938=CARTESIAN_POINT('Ctrl Pts',(28.2244806974172,585.620190359768,-49.2435681999355)) ;
#52939=CARTESIAN_POINT('Ctrl Pts',(28.2299563119541,585.559558208652,-49.2395856489644)) ;
#52940=CARTESIAN_POINT('Ctrl Pts',(28.2355849365913,585.497231757936,-49.2354918099325)) ;
#52941=CARTESIAN_POINT('Ctrl Pts',(28.2446837012938,585.435223824145,-49.2314795365644)) ;
#52942=CARTESIAN_POINT('Ctrl Pts',(28.2572010712248,585.373947134114,-49.2275214453289)) ;
#52943=CARTESIAN_POINT('Ctrl Pts',(28.2693936536096,585.314260387171,-49.2236660544807)) ;
#52944=CARTESIAN_POINT('Ctrl Pts',(28.2848298640616,585.255267569577,-49.219861702331)) ;
#52945=CARTESIAN_POINT('Ctrl Pts',(28.3034218749836,585.197349148697,-49.2160616096605)) ;
#52946=CARTESIAN_POINT('Ctrl Pts',(28.3227567704007,585.137116470525,-49.2121096759688)) ;
#52947=CARTESIAN_POINT('Ctrl Pts',(28.3455055208302,585.078046121607,-49.2081619304247)) ;
#52948=CARTESIAN_POINT('Ctrl Pts',(28.371517494248,585.020561337141,-49.2041477630991)) ;
#52949=CARTESIAN_POINT('Ctrl Pts',(28.3940194411683,584.970833484969,-49.200675263007)) ;
#52950=CARTESIAN_POINT('Ctrl Pts',(28.4189635994826,584.922291233137,-49.1971523990756)) ;
#52951=CARTESIAN_POINT('Ctrl Pts',(28.4462133426358,584.875204601401,-49.1935285002376)) ;
#52952=CARTESIAN_POINT('Ctrl Pts',(28.4504490032766,584.867885523506,-49.1929652066465)) ;
#52953=CARTESIAN_POINT('Ctrl Pts',(28.4547403539537,584.860601513723,-49.1923994719366)) ;
#52954=CARTESIAN_POINT('Ctrl Pts',(28.4590868675054,584.85335347353,-49.1918311058089)) ;
#52955=CARTESIAN_POINT('Ctrl Pts',(28.4591022226987,584.853327867936,-49.1918290979073)) ;
#52956=CARTESIAN_POINT('Ctrl Pts',(28.4591175785805,584.853302262792,-49.1918270899728)) ;
#52957=CARTESIAN_POINT('Ctrl Pts',(28.4591329351506,584.853276658097,-49.1918250820054)) ;
#52958=CARTESIAN_POINT('Ctrl Pts',(28.4876439124845,584.805739031774,-49.1880970938573)) ;
#52959=CARTESIAN_POINT('Ctrl Pts',(28.5186379375329,584.759581449879,-49.1842460094343)) ;
#52960=CARTESIAN_POINT('Ctrl Pts',(28.5519343532963,584.715053248464,-49.1803349721041)) ;
#52961=CARTESIAN_POINT('Ctrl Pts',(28.5550479549378,584.710889344397,-49.1799692446835)) ;
#52962=CARTESIAN_POINT('Ctrl Pts',(28.5581816542848,584.706739701188,-49.1796029930094)) ;
#52963=CARTESIAN_POINT('Ctrl Pts',(28.5613352815921,584.702604530114,-49.1792362687144)) ;
#52964=CARTESIAN_POINT('Ctrl Pts',(28.5986481131138,584.653678348742,-49.1748972899763)) ;
#52965=CARTESIAN_POINT('Ctrl Pts',(28.6387561539551,584.606775674653,-49.1704928166311)) ;
#52966=CARTESIAN_POINT('Ctrl Pts',(28.681383484678,584.562195913215,-49.1660942438563)) ;
#52967=CARTESIAN_POINT('Ctrl Pts',(28.7233976927919,584.518257356825,-49.1617589371686)) ;
#52968=CARTESIAN_POINT('Ctrl Pts',(28.7678589922592,584.476575000279,-49.157429649602)) ;
#52969=CARTESIAN_POINT('Ctrl Pts',(28.8144811521911,584.437403214667,-49.153154203207)) ;
#52970=CARTESIAN_POINT('Ctrl Pts',(28.8610746801217,584.398255485569,-49.148881382486)) ;
#52971=CARTESIAN_POINT('Ctrl Pts',(28.909826357949,584.361615128034,-49.1446624721032)) ;
#52972=CARTESIAN_POINT('Ctrl Pts',(28.9604303812696,584.327707055385,-49.1405214176195)) ;
#52973=CARTESIAN_POINT('Ctrl Pts',(29.0110221426583,584.293807199048,-49.1363813665605)) ;
#52974=CARTESIAN_POINT('Ctrl Pts',(29.0634653525719,584.262638340035,-49.1323191363699)) ;
#52975=CARTESIAN_POINT('Ctrl Pts',(29.1174347103728,584.234396814664,-49.12833387015)) ;
#52976=CARTESIAN_POINT('Ctrl Pts',(29.1728496356943,584.205398840941,-49.1242418587021)) ;
#52977=CARTESIAN_POINT('Ctrl Pts',(29.2298736888144,584.179487448832,-49.1202309763558)) ;
#52978=CARTESIAN_POINT('Ctrl Pts',(29.2881328095016,584.156842272946,-49.1162740363857)) ;
#52979=CARTESIAN_POINT('Ctrl Pts',(29.3449446176583,584.134759663856,-49.112415397398)) ;
#52980=CARTESIAN_POINT('Ctrl Pts',(29.4029308467287,584.115783191148,-49.1086076904091)) ;
#52981=CARTESIAN_POINT('Ctrl Pts',(29.4617236953144,584.100045151821,-49.1048042023169)) ;
#52982=CARTESIAN_POINT('Ctrl Pts',(29.5227632148621,584.083705709487,-49.1008553702507)) ;
#52983=CARTESIAN_POINT('Ctrl Pts',(29.5846723184021,584.070857799057,-49.0969106653445)) ;
#52984=CARTESIAN_POINT('Ctrl Pts',(29.6470154064052,584.061603646524,-49.0928998653571)) ;
#52985=CARTESIAN_POINT('Ctrl Pts',(29.7010540955114,584.053582191577,-49.0894233232011)) ;
#52986=CARTESIAN_POINT('Ctrl Pts',(29.7554197479734,584.048260564658,-49.0858964661079)) ;
#52987=CARTESIAN_POINT('Ctrl Pts',(29.809810853575,584.045670322028,-49.0822685563521)) ;
#52988=CARTESIAN_POINT('Ctrl Pts',(29.8181398865501,584.045273672318,-49.0817130063288)) ;
#52989=CARTESIAN_POINT('Ctrl Pts',(29.8264695910836,584.044941006331,-49.0811550866721)) ;
#52990=CARTESIAN_POINT('Ctrl Pts',(29.8347989676782,584.044672368068,-49.0805946151893)) ;
#52991=CARTESIAN_POINT('Ctrl Pts',(29.8348284924448,584.044671415838,-49.0805926285113)) ;
#52992=CARTESIAN_POINT('Ctrl Pts',(29.8348580172073,584.044670464412,-49.0805906418011)) ;
#52993=CARTESIAN_POINT('Ctrl Pts',(29.8348875419656,584.044669513791,-49.0805886550589)) ;
#52994=CARTESIAN_POINT('Ctrl Pts',(29.8903175165627,584.042884811547,-49.0768587322658)) ;
#52995=CARTESIAN_POINT('Ctrl Pts',(29.9459321440122,584.043937425318,-49.0730059557604)) ;
#52996=CARTESIAN_POINT('Ctrl Pts',(30.0014236513393,584.04781044237,-49.0690934740472)) ;
#52997=CARTESIAN_POINT('Ctrl Pts',(30.0065959059976,584.0481714387,-49.0687287992936)) ;
#52998=CARTESIAN_POINT('Ctrl Pts',(30.0117670612265,584.048556915355,-49.0683636058366)) ;
#52999=CARTESIAN_POINT('Ctrl Pts',(30.0169368498329,584.048966844287,-49.067997944812)) ;
#53000=CARTESIAN_POINT('Ctrl Pts',(30.0782730130214,584.053830383164,-49.0636596157266)) ;
#53001=CARTESIAN_POINT('Ctrl Pts',(30.1394218342725,584.062139185518,-49.0592561361515)) ;
#53002=CARTESIAN_POINT('Ctrl Pts',(30.1999823563176,584.07382344307,-49.0548587678238)) ;
#53003=CARTESIAN_POINT('Ctrl Pts',(30.2596856714703,584.085342315222,-49.0505236422628)) ;
#53004=CARTESIAN_POINT('Ctrl Pts',(30.3188174004899,584.100141355125,-49.0461947433676)) ;
#53005=CARTESIAN_POINT('Ctrl Pts',(30.3770085797434,584.118117662475,-49.0419198022215)) ;
#53006=CARTESIAN_POINT('Ctrl Pts',(30.4351642463517,584.136082999327,-49.0376474699668)) ;
#53007=CARTESIAN_POINT('Ctrl Pts',(30.4923805778851,584.157221615747,-49.0334291645333)) ;
#53008=CARTESIAN_POINT('Ctrl Pts',(30.548302767096,584.181398204428,-49.0292887349009)) ;
#53009=CARTESIAN_POINT('Ctrl Pts',(30.6042116002257,584.205569018935,-49.025149294141)) ;
#53010=CARTESIAN_POINT('Ctrl Pts',(30.6588268789108,584.232776375357,-49.0210876943239)) ;
#53011=CARTESIAN_POINT('Ctrl Pts',(30.7118072538956,584.262853095794,-49.0171029811632)) ;
#53012=CARTESIAN_POINT('Ctrl Pts',(30.7661843114642,584.293722706647,-49.0130132219459)) ;
#53013=CARTESIAN_POINT('Ctrl Pts',(30.8188389230425,584.32761524715,-49.0090044413065)) ;
#53014=CARTESIAN_POINT('Ctrl Pts',(30.8694177914357,584.364313765642,-49.0050493917579)) ;
#53015=CARTESIAN_POINT('Ctrl Pts',(30.9187607530955,584.400115547067,-49.0011909847899)) ;
#53016=CARTESIAN_POINT('Ctrl Pts',(30.9661279918959,584.438587919974,-48.9973833526409)) ;
#53017=CARTESIAN_POINT('Ctrl Pts',(31.0112089557346,584.479493276818,-48.9935797119252)) ;
#53018=CARTESIAN_POINT('Ctrl Pts',(31.0579836525257,584.521935485249,-48.9896331649567)) ;
#53019=CARTESIAN_POINT('Ctrl Pts',(31.102296402178,584.566997512617,-48.9856904925102)) ;
#53020=CARTESIAN_POINT('Ctrl Pts',(31.143825788243,584.614369021137,-48.9816815573379)) ;
#53021=CARTESIAN_POINT('Ctrl Pts',(31.1798354338611,584.655444302904,-48.978205456472)) ;
#53022=CARTESIAN_POINT('Ctrl Pts',(31.2137531507878,584.698256546786,-48.9746788816414)) ;
#53023=CARTESIAN_POINT('Ctrl Pts',(31.2453891710365,584.742569517941,-48.9710511387411)) ;
#53024=CARTESIAN_POINT('Ctrl Pts',(31.2502212057411,584.74933780968,-48.970497043142)) ;
#53025=CARTESIAN_POINT('Ctrl Pts',(31.2550001060564,584.756141138826,-48.9699405873914)) ;
#53026=CARTESIAN_POINT('Ctrl Pts',(31.2597252983142,584.762978695664,-48.9693815908545)) ;
#53027=CARTESIAN_POINT('Ctrl Pts',(31.2597422102587,584.763003167976,-48.9693795901489)) ;
#53028=CARTESIAN_POINT('Ctrl Pts',(31.2597591215152,584.763027640727,-48.9693775894108)) ;
#53029=CARTESIAN_POINT('Ctrl Pts',(31.2597760320838,584.763052113917,-48.9693755886401)) ;
#53030=CARTESIAN_POINT('Ctrl Pts',(31.291512138973,584.808981010507,-48.9656207372716)) ;
#53031=CARTESIAN_POINT('Ctrl Pts',(31.3209299268057,584.856619987665,-48.9617415914158)) ;
#53032=CARTESIAN_POINT('Ctrl Pts',(31.3478772797298,584.905699548094,-48.957802345134)) ;
#53033=CARTESIAN_POINT('Ctrl Pts',(31.3505714667192,584.910606505505,-48.9574085006584)) ;
#53034=CARTESIAN_POINT('Ctrl Pts',(31.3532409612405,584.915527819945,-48.9570140554231)) ;
#53035=CARTESIAN_POINT('Ctrl Pts',(31.3558856132298,584.920463193576,-48.956619073583)) ;
#53036=CARTESIAN_POINT('Ctrl Pts',(31.3849334868214,584.974671501491,-48.9522807399917)) ;
#53037=CARTESIAN_POINT('Ctrl Pts',(31.410984647693,585.030581948043,-48.9478783028844)) ;
#53038=CARTESIAN_POINT('Ctrl Pts',(31.4338829509442,585.08782613794,-48.9434824085856)) ;
#53039=CARTESIAN_POINT('Ctrl Pts',(31.4567460818547,585.144982399393,-48.9390932664854)) ;
#53040=CARTESIAN_POINT('Ctrl Pts',(31.4764664101212,585.203468299925,-48.9347109833581)) ;
#53041=CARTESIAN_POINT('Ctrl Pts',(31.49292594124,585.262910672511,-48.9303843986088)) ;
#53042=CARTESIAN_POINT('Ctrl Pts',(31.5093706759025,585.322299608796,-48.9260617032851)) ;
#53043=CARTESIAN_POINT('Ctrl Pts',(31.522560610632,585.382643343148,-48.9217947462704)) ;
#53044=CARTESIAN_POINT('Ctrl Pts',(31.5324116742823,585.443562888578,-48.9176072870562)) ;
#53045=CARTESIAN_POINT('Ctrl Pts',(31.5422576410633,585.504450914674,-48.9134219944033)) ;
#53046=CARTESIAN_POINT('Ctrl Pts',(31.5487681465865,585.565914190783,-48.9093161225875)) ;
#53047=CARTESIAN_POINT('Ctrl Pts',(31.5518921895599,585.627566870626,-48.9052874063687)) ;
#53048=CARTESIAN_POINT('Ctrl Pts',(31.5533073133279,585.655494198564,-48.9034624852251)) ;
#53049=CARTESIAN_POINT('Ctrl Pts',(31.5540280230629,585.683460285665,-48.9016530418679)) ;
#53050=CARTESIAN_POINT('Ctrl Pts',(31.5540518914521,585.711428744506,-48.8998571438181)) ;
#53051=CARTESIAN_POINT('Ctrl Pts',(31.5545274105876,585.711411214421,-48.8995834207373)) ;
#53052=CARTESIAN_POINT('Ctrl Pts',(31.5544903932093,585.784303671105,-48.8949620477403)) ;
#53053=CARTESIAN_POINT('Ctrl Pts',(31.5496696402885,585.857118891942,-48.8904723599722)) ;
#53054=CARTESIAN_POINT('Ctrl Pts',(31.5263027539008,586.033479051458,-48.8795927983639)) ;
#53055=CARTESIAN_POINT('Ctrl Pts',(31.5027036142072,586.13602033832,-48.8732665485696)) ;
#53056=CARTESIAN_POINT('Ctrl Pts',(31.4639986027888,586.25256609756,-48.8654275397895)) ;
#53057=CARTESIAN_POINT('Ctrl Pts',(31.4581092953798,586.269391653842,-48.8642790344837)) ;
#53058=CARTESIAN_POINT('Ctrl Pts',(31.451951903833,586.286117526255,-48.8631174034081)) ;
#53059=CARTESIAN_POINT('Origin',(29.8885276254069,535.710565160562,-48.522160171753)) ;
#53060=CARTESIAN_POINT('',(31.4521854151178,536.286177671927,-47.6539925072191)) ;
#53061=CARTESIAN_POINT('',(31.4519498093679,536.286123215583,-47.522160171753)) ;
#53062=CARTESIAN_POINT('',(31.4519498093678,536.286123215583,-48.5221601717531)) ;
#53063=CARTESIAN_POINT('',(29.9642548136477,537.375716565857,-47.5221676802302)) ;
#53064=CARTESIAN_POINT('Origin',(29.8885276254069,535.710565160562,-47.522160171753)) ;
#53065=CARTESIAN_POINT('Ctrl Pts',(29.9642548143816,537.375716581994,-47.5221676803692)) ;
#53066=CARTESIAN_POINT('Ctrl Pts',(30.0170574073778,537.373284149692,-47.5257769798607)) ;
#53067=CARTESIAN_POINT('Ctrl Pts',(30.0698319721191,537.368277725697,-47.5294835831224)) ;
#53068=CARTESIAN_POINT('Ctrl Pts',(30.1223097046126,537.360730277946,-47.5332331994959)) ;
#53069=CARTESIAN_POINT('Ctrl Pts',(30.1821635812742,537.352121979048,-47.5375098529502)) ;
#53070=CARTESIAN_POINT('Ctrl Pts',(30.2416325433276,537.340207859062,-47.5418418996151)) ;
#53071=CARTESIAN_POINT('Ctrl Pts',(30.3003395339928,537.32507516245,-47.5461632085829)) ;
#53072=CARTESIAN_POINT('Ctrl Pts',(30.3589866688338,537.309957894666,-47.5504801116784)) ;
#53073=CARTESIAN_POINT('Ctrl Pts',(30.416873522907,537.291628889203,-47.5547860009387)) ;
#53074=CARTESIAN_POINT('Ctrl Pts',(30.4736402945146,537.27020984188,-47.5590357020397)) ;
#53075=CARTESIAN_POINT('Ctrl Pts',(30.5303707287166,537.248804505264,-47.5632826828325)) ;
#53076=CARTESIAN_POINT('Ctrl Pts',(30.5859825640855,537.224313171479,-47.5674734291859)) ;
#53077=CARTESIAN_POINT('Ctrl Pts',(30.6401313340043,537.196889321788,-47.5715866433701)) ;
#53078=CARTESIAN_POINT('Ctrl Pts',(30.6942659880685,537.169472621124,-47.5756987852949)) ;
#53079=CARTESIAN_POINT('Ctrl Pts',(30.746938287709,537.139124906016,-47.5797334448799)) ;
#53080=CARTESIAN_POINT('Ctrl Pts',(30.7978186947913,537.106031130019,-47.5836939134857)) ;
#53081=CARTESIAN_POINT('Ctrl Pts',(30.8487419661031,537.07290947415,-47.5876577185906)) ;
#53082=CARTESIAN_POINT('Ctrl Pts',(30.8978701708745,537.037037008071,-47.5915473315807)) ;
#53083=CARTESIAN_POINT('Ctrl Pts',(30.9448891615152,536.998631930822,-47.5953896858911)) ;
#53084=CARTESIAN_POINT('Ctrl Pts',(30.9919258102846,536.960212430426,-47.5992334832097)) ;
#53085=CARTESIAN_POINT('Ctrl Pts',(31.0368513845029,536.919258218283,-47.6030302593924)) ;
#53086=CARTESIAN_POINT('Ctrl Pts',(31.0793707884461,536.876022923814,-47.6068276814917)) ;
#53087=CARTESIAN_POINT('Ctrl Pts',(31.1219709625019,536.832705499323,-47.6106323171967)) ;
#53088=CARTESIAN_POINT('Ctrl Pts',(31.1621553398343,536.787098063884,-47.6144380750506)) ;
#53089=CARTESIAN_POINT('Ctrl Pts',(31.1996521844407,536.73949448145,-47.6183081328949)) ;
#53090=CARTESIAN_POINT('Ctrl Pts',(31.2333481056982,536.696716306856,-47.6217858965775)) ;
#53091=CARTESIAN_POINT('Ctrl Pts',(31.2648740144835,536.652325877933,-47.6253161745565)) ;
#53092=CARTESIAN_POINT('Ctrl Pts',(31.2940549538489,536.606567395771,-47.6289493146419)) ;
#53093=CARTESIAN_POINT('Ctrl Pts',(31.2966758844579,536.602457527853,-47.6292756306641)) ;
#53094=CARTESIAN_POINT('Ctrl Pts',(31.2992779311643,536.598336612712,-47.6296027764757)) ;
#53095=CARTESIAN_POINT('Ctrl Pts',(31.3018609866169,536.594204820238,-47.6299307885563)) ;
#53096=CARTESIAN_POINT('Ctrl Pts',(31.3018781850347,536.594177310068,-47.629932972516)) ;
#53097=CARTESIAN_POINT('Ctrl Pts',(31.3018953826107,536.594149799416,-47.629935156514)) ;
#53098=CARTESIAN_POINT('Ctrl Pts',(31.3019125793448,536.594122288282,-47.6299373405505)) ;
#53099=CARTESIAN_POINT('Ctrl Pts',(31.3317744651969,536.546349592843,-47.6337298889883)) ;
#53100=CARTESIAN_POINT('Ctrl Pts',(31.359192467101,536.496956319906,-47.6376476228927)) ;
#53101=CARTESIAN_POINT('Ctrl Pts',(31.384028189051,536.446222500673,-47.6416252768862)) ;
#53102=CARTESIAN_POINT('Ctrl Pts',(31.3866683921264,536.440829156931,-47.6420481280651)) ;
#53103=CARTESIAN_POINT('Ctrl Pts',(31.3892794152376,536.435420711993,-47.6424716564076)) ;
#53104=CARTESIAN_POINT('Ctrl Pts',(31.3918610949582,536.429997536727,-47.6428957835048)) ;
#53105=CARTESIAN_POINT('Ctrl Pts',(31.4141913480305,536.383089752166,-47.646564273186)) ;
#53106=CARTESIAN_POINT('Ctrl Pts',(31.434327202609,536.335075674395,-47.6502774611457)) ;
#53107=CARTESIAN_POINT('Ctrl Pts',(31.4521854151178,536.286177671927,-47.6539925072191)) ;
#53108=CARTESIAN_POINT('Origin',(29.8885276254069,535.710565160562,-48.522160171753)) ;
#53109=CARTESIAN_POINT('',(31.4519498068212,536.2861232225,-48.3557322092704)) ;
#53110=CARTESIAN_POINT('',(31.4519274540278,536.286111640514,-48.1612746756653)) ;
#53111=CARTESIAN_POINT('',(31.4519498093678,536.286123215583,-48.5221601717531)) ;
#53112=CARTESIAN_POINT('',(31.5236569526584,535.391334705934,-47.522160171753)) ;
#53113=CARTESIAN_POINT('Ctrl Pts',(31.4519274540278,536.286111640514,-48.1612746756653)) ;
#53114=CARTESIAN_POINT('Ctrl Pts',(31.4307763993745,536.343129105232,-48.1569488744972)) ;
#53115=CARTESIAN_POINT('Ctrl Pts',(31.4064929013936,536.399042410981,-48.1526457224962)) ;
#53116=CARTESIAN_POINT('Ctrl Pts',(31.3792366254787,536.453505067295,-48.1484061457518)) ;
#53117=CARTESIAN_POINT('Ctrl Pts',(31.3519940803956,536.507940287082,-48.1441687047693)) ;
#53118=CARTESIAN_POINT('Ctrl Pts',(31.3217818123083,536.560926365304,-48.1399948666501)) ;
#53119=CARTESIAN_POINT('Ctrl Pts',(31.2887894185131,536.612134703357,-48.1359011995699)) ;
#53120=CARTESIAN_POINT('Ctrl Pts',(31.2558013785795,536.66333628367,-48.1318080727131)) ;
#53121=CARTESIAN_POINT('Ctrl Pts',(31.220033903596,536.712760528073,-48.1277950639092)) ;
#53122=CARTESIAN_POINT('Ctrl Pts',(31.1817065990466,536.760096483813,-48.1238540114814)) ;
#53123=CARTESIAN_POINT('Ctrl Pts',(31.1433423463772,536.807478072153,-48.1199091598175)) ;
#53124=CARTESIAN_POINT('Ctrl Pts',(31.1024131976471,536.85276716559,-48.1160362534294)) ;
#53125=CARTESIAN_POINT('Ctrl Pts',(31.0591708420407,536.895671278289,-48.1122036736627)) ;
#53126=CARTESIAN_POINT('Ctrl Pts',(31.0159079097594,536.938595806712,-48.1083692701806)) ;
#53127=CARTESIAN_POINT('Ctrl Pts',(30.9703293733988,536.979132765155,-48.1045749219151)) ;
#53128=CARTESIAN_POINT('Ctrl Pts',(30.9227211915417,537.017012300491,-48.1007689239922)) ;
#53129=CARTESIAN_POINT('Ctrl Pts',(30.8750231851506,537.054963304879,-48.0969557451189)) ;
#53130=CARTESIAN_POINT('Ctrl Pts',(30.825287647601,537.090246304601,-48.0931303466352)) ;
#53131=CARTESIAN_POINT('Ctrl Pts',(30.7738394110681,537.122619453151,-48.089226826036)) ;
#53132=CARTESIAN_POINT('Ctrl Pts',(30.7324041251834,537.148692079844,-48.0860830158126)) ;
#53133=CARTESIAN_POINT('Ctrl Pts',(30.6898586330363,537.172877634962,-48.0828880724602)) ;
#53134=CARTESIAN_POINT('Ctrl Pts',(30.6463912714896,537.195068149825,-48.0796053349554)) ;
#53135=CARTESIAN_POINT('Ctrl Pts',(30.6463647388652,537.195081694991,-48.0796033311613)) ;
#53136=CARTESIAN_POINT('Ctrl Pts',(30.6463382058969,537.195095239413,-48.0796013273345)) ;
#53137=CARTESIAN_POINT('Ctrl Pts',(30.6463116725847,537.195108783094,-48.079599323475)) ;
#53138=CARTESIAN_POINT('Ctrl Pts',(30.5969681857448,537.220295703685,-48.0758727847674)) ;
#53139=CARTESIAN_POINT('Ctrl Pts',(30.5462514251147,537.242999512425,-48.0720232603926)) ;
#53140=CARTESIAN_POINT('Ctrl Pts',(30.4944463678682,537.263104505909,-48.0681138788279)) ;
#53141=CARTESIAN_POINT('Ctrl Pts',(30.4896029522929,537.264984184145,-48.0677483786129)) ;
#53142=CARTESIAN_POINT('Ctrl Pts',(30.4847500607543,537.266841154097,-48.0673823551886)) ;
#53143=CARTESIAN_POINT('Ctrl Pts',(30.4798879487158,537.268675326625,-48.0670158601448)) ;
#53144=CARTESIAN_POINT('Ctrl Pts',(30.4223124608371,537.290394977941,-48.0626759496729)) ;
#53145=CARTESIAN_POINT('Ctrl Pts',(30.3634380633247,537.308917002742,-48.0582705761492)) ;
#53146=CARTESIAN_POINT('Ctrl Pts',(30.3036577270648,537.324133525588,-48.0538712807422)) ;
#53147=CARTESIAN_POINT('Ctrl Pts',(30.2447759697572,537.339121323607,-48.0495381126691)) ;
#53148=CARTESIAN_POINT('Ctrl Pts',(30.1850153196505,537.350902695154,-48.045211126453)) ;
#53149=CARTESIAN_POINT('Ctrl Pts',(30.1247528952844,537.359413652336,-48.0409381775236)) ;
#53150=CARTESIAN_POINT('Ctrl Pts',(30.0645273363901,537.367919402949,-48.036667842566)) ;
#53151=CARTESIAN_POINT('Ctrl Pts',(30.003800605354,537.373158868586,-48.0324516142783)) ;
#53152=CARTESIAN_POINT('Ctrl Pts',(29.9429508114481,537.375103428451,-48.0283135052074)) ;
#53153=CARTESIAN_POINT('Ctrl Pts',(29.8821155448548,537.377047524072,-48.0241763840708)) ;
#53154=CARTESIAN_POINT('Ctrl Pts',(29.8211572945153,537.37569825651,-48.0201173480267)) ;
#53155=CARTESIAN_POINT('Ctrl Pts',(29.7604555381149,537.371061579568,-48.0161356354981)) ;
#53156=CARTESIAN_POINT('Ctrl Pts',(29.6980574154047,537.366295326432,-48.0120426503574)) ;
#53157=CARTESIAN_POINT('Ctrl Pts',(29.6359303902143,537.358055001222,-48.0080313634024)) ;
#53158=CARTESIAN_POINT('Ctrl Pts',(29.574487749723,537.346386736832,-48.0040746050507)) ;
#53159=CARTESIAN_POINT('Ctrl Pts',(29.5146381758799,537.335021003758,-48.0002204363617)) ;
#53160=CARTESIAN_POINT('Ctrl Pts',(29.4554380951338,537.320402658138,-47.9964176386363)) ;
#53161=CARTESIAN_POINT('Ctrl Pts',(29.3972689929696,537.302614489539,-47.9926195892224)) ;
#53162=CARTESIAN_POINT('Ctrl Pts',(29.336777386634,537.284116096882,-47.9886698959756)) ;
#53163=CARTESIAN_POINT('Ctrl Pts',(29.2774010738504,537.262188882748,-47.9847249222463)) ;
#53164=CARTESIAN_POINT('Ctrl Pts',(29.2195650502174,537.236977757016,-47.9807141626381)) ;
#53165=CARTESIAN_POINT('Ctrl Pts',(29.1694956145773,537.215152141111,-47.9772419932625)) ;
#53166=CARTESIAN_POINT('Ctrl Pts',(29.1205796400799,537.190865130713,-47.9737198631058)) ;
#53167=CARTESIAN_POINT('Ctrl Pts',(29.0730894036172,537.164249925727,-47.970096974239)) ;
#53168=CARTESIAN_POINT('Ctrl Pts',(29.0657493701776,537.160136311874,-47.9695370249229)) ;
#53169=CARTESIAN_POINT('Ctrl Pts',(29.0584432953211,537.155967097591,-47.9689746686405)) ;
#53170=CARTESIAN_POINT('Ctrl Pts',(29.0511720738838,537.15174278969,-47.9684097178374)) ;
#53171=CARTESIAN_POINT('Ctrl Pts',(29.0511458435209,537.15172755083,-47.9684076798215)) ;
#53172=CARTESIAN_POINT('Ctrl Pts',(29.0511196136116,537.151712311252,-47.9684056417719)) ;
#53173=CARTESIAN_POINT('Ctrl Pts',(29.0510933841558,537.151697070958,-47.9684036036885)) ;
#53174=CARTESIAN_POINT('Ctrl Pts',(29.0030948273822,537.123808115142,-47.9646740157731)) ;
#53175=CARTESIAN_POINT('Ctrl Pts',(28.9564471739132,537.093411201235,-47.9608215272907)) ;
#53176=CARTESIAN_POINT('Ctrl Pts',(28.911402686255,537.060684312441,-47.9569092390924)) ;
#53177=CARTESIAN_POINT('Ctrl Pts',(28.907192685099,537.057625553272,-47.9565435841878)) ;
#53178=CARTESIAN_POINT('Ctrl Pts',(28.9029967015222,537.054546476073,-47.9561774069107)) ;
#53179=CARTESIAN_POINT('Ctrl Pts',(28.8988149491624,537.051447248039,-47.955810758779)) ;
#53180=CARTESIAN_POINT('Ctrl Pts',(28.8493969261517,537.014821998832,-47.9514778800595)) ;
#53181=CARTESIAN_POINT('Ctrl Pts',(28.8019638330814,536.975377158774,-47.9470799052921)) ;
#53182=CARTESIAN_POINT('Ctrl Pts',(28.7568178425373,536.933384066512,-47.9426877957958)) ;
#53183=CARTESIAN_POINT('Ctrl Pts',(28.7122458337714,536.891924870382,-47.938351527157)) ;
#53184=CARTESIAN_POINT('Ctrl Pts',(28.6699027807026,536.847982052344,-47.9340212680818)) ;
#53185=CARTESIAN_POINT('Ctrl Pts',(28.6300474554127,536.801839145611,-47.9297447615701)) ;
#53186=CARTESIAN_POINT('Ctrl Pts',(28.5902164977647,536.755724450761,-47.9254708697248)) ;
#53187=CARTESIAN_POINT('Ctrl Pts',(28.5528701088114,536.707412413854,-47.9212507998254)) ;
#53188=CARTESIAN_POINT('Ctrl Pts',(28.5182378571019,536.657206506776,-47.9171083924019)) ;
#53189=CARTESIAN_POINT('Ctrl Pts',(28.4836139993599,536.60701276832,-47.9129669889915)) ;
#53190=CARTESIAN_POINT('Ctrl Pts',(28.4517029987154,536.554926073915,-47.9089032122735)) ;
#53191=CARTESIAN_POINT('Ctrl Pts',(28.4227061221089,536.501269776009,-47.9049160816052)) ;
#53192=CARTESIAN_POINT('Ctrl Pts',(28.3930198148266,536.446337744229,-47.9008341527891)) ;
#53193=CARTESIAN_POINT('Ctrl Pts',(28.3663881619663,536.38976045835,-47.8968325311477)) ;
#53194=CARTESIAN_POINT('Ctrl Pts',(28.34299487761,536.331907062595,-47.8928841713042)) ;
#53195=CARTESIAN_POINT('Ctrl Pts',(28.3201161371515,536.275326173569,-47.8890226570883)) ;
#53196=CARTESIAN_POINT('Ctrl Pts',(28.3003350793831,536.217524722683,-47.8852117336552)) ;
#53197=CARTESIAN_POINT('Ctrl Pts',(28.2837896250148,536.158869478422,-47.8814046545605)) ;
#53198=CARTESIAN_POINT('Ctrl Pts',(28.2666860086315,536.098235495554,-47.8774691433968)) ;
#53199=CARTESIAN_POINT('Ctrl Pts',(28.253040808891,536.036689007455,-47.8735373106197)) ;
#53200=CARTESIAN_POINT('Ctrl Pts',(28.242961550844,535.974659553968,-47.8695398976371)) ;
#53201=CARTESIAN_POINT('Ctrl Pts',(28.2341891644994,535.920672809289,-47.86606078728)) ;
#53202=CARTESIAN_POINT('Ctrl Pts',(28.2281176798626,535.866319363877,-47.8625313512965)) ;
#53203=CARTESIAN_POINT('Ctrl Pts',(28.2247832934975,535.811900633933,-47.8589009975942)) ;
#53204=CARTESIAN_POINT('Ctrl Pts',(28.2242885317416,535.803825892907,-47.858362319716)) ;
#53205=CARTESIAN_POINT('Ctrl Pts',(28.2238539700256,535.795749645206,-47.8578214199208)) ;
#53206=CARTESIAN_POINT('Ctrl Pts',(28.2234796626412,535.787672801144,-47.8572781329275)) ;
#53207=CARTESIAN_POINT('Ctrl Pts',(28.2234781642949,535.787640469671,-47.8572759581586)) ;
#53208=CARTESIAN_POINT('Ctrl Pts',(28.2234766669142,535.787608138189,-47.8572737833515)) ;
#53209=CARTESIAN_POINT('Ctrl Pts',(28.2234751704988,535.787575806697,-47.8572716085062)) ;
#53210=CARTESIAN_POINT('Ctrl Pts',(28.2209073996856,535.732096649492,-47.853539687112)) ;
#53211=CARTESIAN_POINT('Ctrl Pts',(28.2211816101443,535.676392651554,-47.8496854610932)) ;
#53212=CARTESIAN_POINT('Ctrl Pts',(28.2242849530107,535.620773255338,-47.8457724017947)) ;
#53213=CARTESIAN_POINT('Ctrl Pts',(28.2245669508371,535.615719173494,-47.8454168258032)) ;
#53214=CARTESIAN_POINT('Ctrl Pts',(28.2248722884664,535.610665819014,-47.8450607640144)) ;
#53215=CARTESIAN_POINT('Ctrl Pts',(28.2252009433535,535.60561344098,-47.8447042640523)) ;
#53216=CARTESIAN_POINT('Ctrl Pts',(28.22919531299,535.544208404265,-47.8403714740051)) ;
#53217=CARTESIAN_POINT('Ctrl Pts',(28.2366370952629,535.482942529108,-47.8359746228171)) ;
#53218=CARTESIAN_POINT('Ctrl Pts',(28.2474619790141,535.422218004487,-47.8315847343143)) ;
#53219=CARTESIAN_POINT('Ctrl Pts',(28.258125627529,535.362397963767,-47.8272602326301)) ;
#53220=CARTESIAN_POINT('Ctrl Pts',(28.2720719365899,535.303103095364,-47.8229427665659)) ;
#53221=CARTESIAN_POINT('Ctrl Pts',(28.289203276634,535.244703256875,-47.8186794877983)) ;
#53222=CARTESIAN_POINT('Ctrl Pts',(28.3063246657586,535.186337340548,-47.8144186854011)) ;
#53223=CARTESIAN_POINT('Ctrl Pts',(28.3266272780083,535.128865351449,-47.8102121386028)) ;
#53224=CARTESIAN_POINT('Ctrl Pts',(28.3499808983447,535.072643531161,-47.806083000012)) ;
#53225=CARTESIAN_POINT('Ctrl Pts',(28.3733296704721,535.016433382518,-47.8019547186299)) ;
#53226=CARTESIAN_POINT('Ctrl Pts',(28.3997282072346,534.961472915357,-47.7979038130668)) ;
#53227=CARTESIAN_POINT('Ctrl Pts',(28.4290142106474,534.90810541461,-47.7939285579771)) ;
#53228=CARTESIAN_POINT('Ctrl Pts',(28.4591088753211,534.85326430103,-47.7898435359537)) ;
#53229=CARTESIAN_POINT('Ctrl Pts',(28.4922529685829,534.800105547781,-47.785838386868)) ;
#53230=CARTESIAN_POINT('Ctrl Pts',(28.5282337480971,534.748986344858,-47.7818848696984)) ;
#53231=CARTESIAN_POINT('Ctrl Pts',(28.5632957111165,534.699172537969,-47.7780323107858)) ;
#53232=CARTESIAN_POINT('Ctrl Pts',(28.6010513997611,534.651295626704,-47.7742284091018)) ;
#53233=CARTESIAN_POINT('Ctrl Pts',(28.6412674151399,534.605669127893,-47.7704255416625)) ;
#53234=CARTESIAN_POINT('Ctrl Pts',(28.6830642520887,534.558249130826,-47.7664731901229)) ;
#53235=CARTESIAN_POINT('Ctrl Pts',(28.7275192520828,534.513260600536,-47.7625215272401)) ;
#53236=CARTESIAN_POINT('Ctrl Pts',(28.7743246561547,534.471030431014,-47.7584992110668)) ;
#53237=CARTESIAN_POINT('Ctrl Pts',(28.8147152696772,534.434588005401,-47.7550281627714)) ;
#53238=CARTESIAN_POINT('Ctrl Pts',(28.8568567763365,534.40019889432,-47.7515038375611)) ;
#53239=CARTESIAN_POINT('Ctrl Pts',(28.900517275209,534.368054060937,-47.7478756307004)) ;
#53240=CARTESIAN_POINT('Ctrl Pts',(28.9074234764699,534.362969403305,-47.7473017223062)) ;
#53241=CARTESIAN_POINT('Ctrl Pts',(28.9143677111017,534.3579407967,-47.7467252147108)) ;
#53242=CARTESIAN_POINT('Ctrl Pts',(28.9213490950115,534.352968881888,-47.7461459076316)) ;
#53243=CARTESIAN_POINT('Ctrl Pts',(28.9213773075326,534.352948789847,-47.7461435665896)) ;
#53244=CARTESIAN_POINT('Ctrl Pts',(28.9214055206604,534.352928698732,-47.7461412255018)) ;
#53245=CARTESIAN_POINT('Ctrl Pts',(28.9214337343949,534.352908608542,-47.7461388843683)) ;
#53246=CARTESIAN_POINT('Ctrl Pts',(28.9662228141892,534.321015591944,-47.7424223535122)) ;
#53247=CARTESIAN_POINT('Ctrl Pts',(29.0127137470464,534.291342910262,-47.7385803120396)) ;
#53248=CARTESIAN_POINT('Ctrl Pts',(29.0606465209006,534.264045111964,-47.7346755810524)) ;
#53249=CARTESIAN_POINT('Ctrl Pts',(29.0653146261795,534.261386617867,-47.7342953048057)) ;
#53250=CARTESIAN_POINT('Ctrl Pts',(29.0699963659741,534.258750645376,-47.7339144339779)) ;
#53251=CARTESIAN_POINT('Ctrl Pts',(29.0746914739163,534.256137334618,-47.7335330265961)) ;
#53252=CARTESIAN_POINT('Ctrl Pts',(29.1284554251062,534.226212162759,-47.7291655087216)) ;
#53253=CARTESIAN_POINT('Ctrl Pts',(29.18397844417,534.199258635353,-47.7247283308864)) ;
#53254=CARTESIAN_POINT('Ctrl Pts',(29.2408859625142,534.175442489054,-47.7202947956306)) ;
#53255=CARTESIAN_POINT('Ctrl Pts',(29.2967255816198,534.152073265151,-47.7159444579744)) ;
#53256=CARTESIAN_POINT('Ctrl Pts',(29.3538981316818,534.131724304163,-47.7115979109087)) ;
#53257=CARTESIAN_POINT('Ctrl Pts',(29.4120423473608,534.114513494693,-47.7073041677962)) ;
#53258=CARTESIAN_POINT('Ctrl Pts',(29.4701500258677,534.097313500303,-47.7030131228236)) ;
#53259=CARTESIAN_POINT('Ctrl Pts',(29.5292281351195,534.083247580819,-47.6987749580719)) ;
#53260=CARTESIAN_POINT('Ctrl Pts',(29.5889093029062,534.072398666365,-47.694615023098)) ;
#53261=CARTESIAN_POINT('Ctrl Pts',(29.6485756671699,534.061552442913,-47.6904561199688)) ;
#53262=CARTESIAN_POINT('Ctrl Pts',(29.7088447677984,534.053921655637,-47.6863754183603)) ;
#53263=CARTESIAN_POINT('Ctrl Pts',(29.7693429677503,534.049555196414,-47.6823735688117)) ;
#53264=CARTESIAN_POINT('Ctrl Pts',(29.8319435161226,534.045037000136,-47.6782326526117)) ;
#53265=CARTESIAN_POINT('Ctrl Pts',(29.8947893459226,534.044014349964,-47.6741761960406)) ;
#53266=CARTESIAN_POINT('Ctrl Pts',(29.957459733137,534.046501514119,-47.6701779083722)) ;
#53267=CARTESIAN_POINT('Ctrl Pts',(30.0181053442043,534.04890832213,-47.6663087987392)) ;
#53268=CARTESIAN_POINT('Ctrl Pts',(30.0785865391467,534.054601903472,-47.6624937791813)) ;
#53269=CARTESIAN_POINT('Ctrl Pts',(30.1385170065825,534.063555529739,-47.6586872219254)) ;
#53270=CARTESIAN_POINT('Ctrl Pts',(30.2014488234682,534.072957558337,-47.6546900302724)) ;
#53271=CARTESIAN_POINT('Ctrl Pts',(30.2637731501992,534.085955289501,-47.6507017947997)) ;
#53272=CARTESIAN_POINT('Ctrl Pts',(30.3250393960605,534.102464729901,-47.6466504651268)) ;
#53273=CARTESIAN_POINT('Ctrl Pts',(30.3778260115243,534.11668916082,-47.6431598647391)) ;
#53274=CARTESIAN_POINT('Ctrl Pts',(30.4298281741923,534.133520596369,-47.6396217634346)) ;
#53275=CARTESIAN_POINT('Ctrl Pts',(30.4807554477069,534.152865574823,-47.635984368866)) ;
#53276=CARTESIAN_POINT('Ctrl Pts',(30.4889186970596,534.155966425741,-47.6354013225569)) ;
#53277=CARTESIAN_POINT('Ctrl Pts',(30.4970544327808,534.15913182708,-47.6348157250445)) ;
#53278=CARTESIAN_POINT('Ctrl Pts',(30.5051615792712,534.162361361118,-47.6342273630226)) ;
#53279=CARTESIAN_POINT('Ctrl Pts',(30.5051791544077,534.162368362287,-47.6342260875377)) ;
#53280=CARTESIAN_POINT('Ctrl Pts',(30.5051967294098,534.162375363757,-47.6342248120398)) ;
#53281=CARTESIAN_POINT('Ctrl Pts',(30.5052143042776,534.162382365529,-47.6342235365289)) ;
#53282=CARTESIAN_POINT('Ctrl Pts',(30.5574247027775,534.183182822828,-47.6304343227569)) ;
#53283=CARTESIAN_POINT('Ctrl Pts',(30.608629897713,534.20672373114,-47.6265205232274)) ;
#53284=CARTESIAN_POINT('Ctrl Pts',(30.658550718741,534.232862233993,-47.6225444679815)) ;
#53285=CARTESIAN_POINT('Ctrl Pts',(30.6635861589343,534.23549878654,-47.622143409105)) ;
#53286=CARTESIAN_POINT('Ctrl Pts',(30.6686085101118,534.238161729959,-47.6217417168101)) ;
#53287=CARTESIAN_POINT('Ctrl Pts',(30.673617472207,534.2408508916,-47.621339455065)) ;
#53288=CARTESIAN_POINT('Ctrl Pts',(30.7281687379782,534.270137831401,-47.6169585300456)) ;
#53289=CARTESIAN_POINT('Ctrl Pts',(30.7811353217736,534.30253943713,-47.6125107004893)) ;
#53290=CARTESIAN_POINT('Ctrl Pts',(30.8321791594224,534.337831003257,-47.6080652262423)) ;
#53291=CARTESIAN_POINT('Ctrl Pts',(30.8831596432466,534.373078766727,-47.6036252695624)) ;
#53292=CARTESIAN_POINT('Ctrl Pts',(30.9322224567569,534.411209093894,-47.599188003276)) ;
#53293=CARTESIAN_POINT('Ctrl Pts',(30.9790590951107,534.451971645344,-47.5948018504151)) ;
#53294=CARTESIAN_POINT('Ctrl Pts',(31.0258522993938,534.492696395543,-47.5904197650637)) ;
#53295=CARTESIAN_POINT('Ctrl Pts',(31.0704235967529,534.536048447987,-47.5860888350347)) ;
#53296=CARTESIAN_POINT('Ctrl Pts',(31.1124902383189,534.581753621128,-47.5818332950153)) ;
#53297=CARTESIAN_POINT('Ctrl Pts',(31.1545310584144,534.627430739385,-47.577580367144)) ;
#53298=CARTESIAN_POINT('Ctrl Pts',(31.1940702760404,534.675458143157,-47.57340272979)) ;
#53299=CARTESIAN_POINT('Ctrl Pts',(31.2308496570034,534.725537499311,-47.5692996009665)) ;
#53300=CARTESIAN_POINT('Ctrl Pts',(31.2676321070151,534.775621034328,-47.5651961297582)) ;
#53301=CARTESIAN_POINT('Ctrl Pts',(31.3016540857673,534.827756975292,-47.5611670452076)) ;
#53302=CARTESIAN_POINT('Ctrl Pts',(31.3326827611293,534.881620991051,-47.5571876285342)) ;
#53303=CARTESIAN_POINT('Ctrl Pts',(31.3637101458964,534.93548276641,-47.5532083773791)) ;
#53304=CARTESIAN_POINT('Ctrl Pts',(31.3917441313433,534.991072611886,-47.549278497494)) ;
#53305=CARTESIAN_POINT('Ctrl Pts',(31.4165812310452,535.048038404901,-47.545352497709)) ;
#53306=CARTESIAN_POINT('Ctrl Pts',(31.4414428254077,535.105060378299,-47.5414226260537)) ;
#53307=CARTESIAN_POINT('Ctrl Pts',(31.4631006511519,535.163461117163,-47.5374961381248)) ;
#53308=CARTESIAN_POINT('Ctrl Pts',(31.4813868456706,535.22285764003,-47.5335125036937)) ;
#53309=CARTESIAN_POINT('Ctrl Pts',(31.4984440040268,535.27826205429,-47.5297966139138)) ;
#53310=CARTESIAN_POINT('Ctrl Pts',(31.5125673198299,535.33453253182,-47.5260303504884)) ;
#53311=CARTESIAN_POINT('Ctrl Pts',(31.5236569526584,535.391334705934,-47.522160171753)) ;
#53312=CARTESIAN_POINT('Origin',(29.8885276254069,535.710565160562,-47.522160171753)) ;
#53313=CARTESIAN_POINT('Ctrl Pts',(31.4519498042747,536.286123229417,-48.3557322092704)) ;
#53314=CARTESIAN_POINT('Ctrl Pts',(31.4435375980647,536.308973799105,-48.3541129334884)) ;
#53315=CARTESIAN_POINT('Ctrl Pts',(31.4346247554841,536.331639052111,-48.3524768959164)) ;
#53316=CARTESIAN_POINT('Ctrl Pts',(31.3980363936659,536.419007631093,-48.3460474798456)) ;
#53317=CARTESIAN_POINT('Ctrl Pts',(31.3667745744052,536.482116170551,-48.3411329619198)) ;
#53318=CARTESIAN_POINT('Ctrl Pts',(31.2795416155593,536.633332059891,-48.3286756769509)) ;
#53319=CARTESIAN_POINT('Ctrl Pts',(31.2191064536547,536.718521459963,-48.3210228426008)) ;
#53320=CARTESIAN_POINT('Ctrl Pts',(31.1140768495141,536.840524596727,-48.3093794549558)) ;
#53321=CARTESIAN_POINT('Ctrl Pts',(31.0748574789422,536.881633916768,-48.3053192228784)) ;
#53322=CARTESIAN_POINT('Ctrl Pts',(31.0116610518251,536.941435006098,-48.2992914617993)) ;
#53323=CARTESIAN_POINT('Ctrl Pts',(30.9891472863017,536.961607208327,-48.2972363119432)) ;
#53324=CARTESIAN_POINT('Ctrl Pts',(30.9341002736848,537.008291419052,-48.2924405283549)) ;
#53325=CARTESIAN_POINT('Ctrl Pts',(30.9010916999685,537.034207987955,-48.2897378805944)) ;
#53326=CARTESIAN_POINT('Ctrl Pts',(30.8187997554234,537.093936790622,-48.28331051432)) ;
#53327=CARTESIAN_POINT('Ctrl Pts',(30.768607921265,537.12639810772,-48.279641766959)) ;
#53328=CARTESIAN_POINT('Ctrl Pts',(30.6079765977659,537.218435592228,-48.2683224233389)) ;
#53329=CARTESIAN_POINT('Ctrl Pts',(30.49249755534,537.26828679375,-48.2607328450771)) ;
#53330=CARTESIAN_POINT('Ctrl Pts',(30.3233801460445,537.319632298555,-48.2493791966046)) ;
#53331=CARTESIAN_POINT('Ctrl Pts',(30.2735774770622,537.332270874295,-48.2460138389042)) ;
#53332=CARTESIAN_POINT('Ctrl Pts',(30.1662553931302,537.354283897131,-48.2386681198289)) ;
#53333=CARTESIAN_POINT('Ctrl Pts',(30.1086692273945,537.362981636789,-48.234670290237)) ;
#53334=CARTESIAN_POINT('Ctrl Pts',(29.9816941536233,537.375404675195,-48.2257163471331)) ;
#53335=CARTESIAN_POINT('Ctrl Pts',(29.9122886418477,537.377839663216,-48.2207312683048)) ;
#53336=CARTESIAN_POINT('Ctrl Pts',(29.7256897867378,537.372731736576,-48.2071828687329)) ;
#53337=CARTESIAN_POINT('Ctrl Pts',(29.6090995680451,537.357148793933,-48.1985461025743)) ;
#53338=CARTESIAN_POINT('Ctrl Pts',(29.465816766739,537.322328208713,-48.1883170822733)) ;
#53339=CARTESIAN_POINT('Ctrl Pts',(29.4367215658954,537.314415671059,-48.186263453143)) ;
#53340=CARTESIAN_POINT('Ctrl Pts',(29.3690785968729,537.294032412185,-48.181561139837)) ;
#53341=CARTESIAN_POINT('Ctrl Pts',(29.3307406787046,537.280937800884,-48.1789454749204)) ;
#53342=CARTESIAN_POINT('Ctrl Pts',(29.2404289822054,537.246365458977,-48.1728177249305)) ;
#53343=CARTESIAN_POINT('Ctrl Pts',(29.1889900644198,537.223629098726,-48.1693545796757)) ;
#53344=CARTESIAN_POINT('Ctrl Pts',(29.0184835421417,537.137705722292,-48.1576654452413)) ;
#53345=CARTESIAN_POINT('Ctrl Pts',(28.905982853372,537.062714884904,-48.1495440974203)) ;
#53346=CARTESIAN_POINT('Ctrl Pts',(28.7654839429592,536.942177865081,-48.1376246569897)) ;
#53347=CARTESIAN_POINT('Ctrl Pts',(28.7287393246251,536.907639573054,-48.1343144477807)) ;
#53348=CARTESIAN_POINT('Ctrl Pts',(28.6522413966884,536.828902485285,-48.1269414072774)) ;
#53349=CARTESIAN_POINT('Ctrl Pts',(28.6131748790197,536.784136694127,-48.1228542724197)) ;
#53350=CARTESIAN_POINT('Ctrl Pts',(28.5320725015873,536.680514248351,-48.1135992380317)) ;
#53351=CARTESIAN_POINT('Ctrl Pts',(28.4913098596715,536.620813678713,-48.108397049967)) ;
#53352=CARTESIAN_POINT('Ctrl Pts',(28.3991304209052,536.464955397473,-48.0952380751858)) ;
#53353=CARTESIAN_POINT('Ctrl Pts',(28.353023778856,536.366034576115,-48.0872442426966)) ;
#53354=CARTESIAN_POINT('Ctrl Pts',(28.3066145792634,536.234079826741,-48.0775153206307)) ;
#53355=CARTESIAN_POINT('Ctrl Pts',(28.2971483976233,536.204558351429,-48.0753977671491)) ;
#53356=CARTESIAN_POINT('Ctrl Pts',(28.2776526871594,536.137362750658,-48.0707307657612)) ;
#53357=CARTESIAN_POINT('Ctrl Pts',(28.2681104947567,536.099567977191,-48.0682063745697)) ;
#53358=CARTESIAN_POINT('Ctrl Pts',(28.2488134287677,536.010005988046,-48.0623835007591)) ;
#53359=CARTESIAN_POINT('Ctrl Pts',(28.2401698091122,535.958041923795,-48.0591271252558)) ;
#53360=CARTESIAN_POINT('Ctrl Pts',(28.2180401003055,535.770457042348,-48.0475397746605)) ;
#53361=CARTESIAN_POINT('Ctrl Pts',(28.2187345711917,535.633727927844,-48.0393577355581)) ;
#53362=CARTESIAN_POINT('Ctrl Pts',(28.2426459436233,535.447306795531,-48.0273042054568)) ;
#53363=CARTESIAN_POINT('Ctrl Pts',(28.2516115785173,535.396341737346,-48.0239206118743)) ;
#53364=CARTESIAN_POINT('Ctrl Pts',(28.2754750864591,535.289969296684,-48.0166220183331)) ;
#53365=CARTESIAN_POINT('Ctrl Pts',(28.2908927234949,535.234749339229,-48.0126936576772)) ;
#53366=CARTESIAN_POINT('Ctrl Pts',(28.3305243776014,535.116674810865,-48.0039690553726)) ;
#53367=CARTESIAN_POINT('Ctrl Pts',(28.3557662184974,535.054272026154,-47.9991477148186)) ;
#53368=CARTESIAN_POINT('Ctrl Pts',(28.4353701154607,534.887311186294,-47.9857406464015)) ;
#53369=CARTESIAN_POINT('Ctrl Pts',(28.4971543769131,534.786715967458,-47.9770636544323)) ;
#53370=CARTESIAN_POINT('Ctrl Pts',(28.5882917440669,534.668481620317,-47.9666595873728)) ;
#53371=CARTESIAN_POINT('Ctrl Pts',(28.6082622562069,534.644041522845,-47.9644987882644)) ;
#53372=CARTESIAN_POINT('Ctrl Pts',(28.6536053052531,534.591661424027,-47.9598685952331)) ;
#53373=CARTESIAN_POINT('Ctrl Pts',(28.6792559040783,534.563987127291,-47.9574184549172)) ;
#53374=CARTESIAN_POINT('Ctrl Pts',(28.7409596624373,534.501792156922,-47.9518353684137)) ;
#53375=CARTESIAN_POINT('Ctrl Pts',(28.7776682006956,534.467972525959,-47.9487394549282)) ;
#53376=CARTESIAN_POINT('Ctrl Pts',(28.9305656981363,534.339307778057,-47.9364546280536)) ;
#53377=CARTESIAN_POINT('Ctrl Pts',(29.057784187646,534.258704192475,-47.9274846601584)) ;
#53378=CARTESIAN_POINT('Ctrl Pts',(29.2399660973278,534.175158470707,-47.9145414001103)) ;
#53379=CARTESIAN_POINT('Ctrl Pts',(29.2867935212821,534.156209699931,-47.9112147795177)) ;
#53380=CARTESIAN_POINT('Ctrl Pts',(29.3927751972407,534.11883138921,-47.9036431981116)) ;
#53381=CARTESIAN_POINT('Ctrl Pts',(29.4522396252813,534.101516399241,-47.8993656143163)) ;
#53382=CARTESIAN_POINT('Ctrl Pts',(29.66974165479,534.051127598483,-47.8835975082911)) ;
#53383=CARTESIAN_POINT('Ctrl Pts',(29.8313899202287,534.037745769076,-47.8715536681794)) ;
#53384=CARTESIAN_POINT('Ctrl Pts',(30.0285574105528,534.050065737868,-47.8576182398169)) ;
#53385=CARTESIAN_POINT('Ctrl Pts',(30.0646107414035,534.05350090764,-47.8551065105941)) ;
#53386=CARTESIAN_POINT('Ctrl Pts',(30.1324093343848,534.062199020259,-47.8504868905879)) ;
#53387=CARTESIAN_POINT('Ctrl Pts',(30.1641679603495,534.067211327545,-47.8483689220744)) ;
#53388=CARTESIAN_POINT('Ctrl Pts',(30.2335954821385,534.080238250613,-47.8438022911596)) ;
#53389=CARTESIAN_POINT('Ctrl Pts',(30.2711731263722,534.088646382792,-47.8413717662144)) ;
#53390=CARTESIAN_POINT('Ctrl Pts',(30.3973734928361,534.121515201023,-47.8332472451969)) ;
#53391=CARTESIAN_POINT('Ctrl Pts',(30.4842523194431,534.152002534313,-47.8277112406882)) ;
#53392=CARTESIAN_POINT('Ctrl Pts',(30.645469916295,534.224038501226,-47.8168750338328)) ;
#53393=CARTESIAN_POINT('Ctrl Pts',(30.7200094252909,534.264412170001,-47.8116064339739)) ;
#53394=CARTESIAN_POINT('Ctrl Pts',(30.833231439325,534.337394745914,-47.8028941814984)) ;
#53395=CARTESIAN_POINT('Ctrl Pts',(30.8740615324785,534.366398397338,-47.7995909204402)) ;
#53396=CARTESIAN_POINT('Ctrl Pts',(30.9629568464386,534.435774865285,-47.7919828115356)) ;
#53397=CARTESIAN_POINT('Ctrl Pts',(31.0101687469789,534.477111538993,-47.787640975437)) ;
#53398=CARTESIAN_POINT('Ctrl Pts',(31.1379081208986,534.60236466765,-47.7749820022143)) ;
#53399=CARTESIAN_POINT('Ctrl Pts',(31.2121359025443,534.692176375442,-47.7664459392426)) ;
#53400=CARTESIAN_POINT('Ctrl Pts',(31.3087781660287,534.837714150281,-47.753782702513)) ;
#53401=CARTESIAN_POINT('Ctrl Pts',(31.3385622549675,534.888141037319,-47.7495846721178)) ;
#53402=CARTESIAN_POINT('Ctrl Pts',(31.3796701118715,534.966944804672,-47.7434086604974)) ;
#53403=CARTESIAN_POINT('Ctrl Pts',(31.3929709952149,534.994235706057,-47.7413374390977)) ;
#53404=CARTESIAN_POINT('Ctrl Pts',(31.4221282223764,535.058461507149,-47.7366349899464)) ;
#53405=CARTESIAN_POINT('Ctrl Pts',(31.4374083891385,535.095635077976,-47.7340347120364)) ;
#53406=CARTESIAN_POINT('Ctrl Pts',(31.4704882920144,535.185195183456,-47.7279713655755)) ;
#53407=CARTESIAN_POINT('Ctrl Pts',(31.487053207048,535.237987156671,-47.7245549000931)) ;
#53408=CARTESIAN_POINT('Ctrl Pts',(31.5352891797283,535.423588236114,-47.7127863493649)) ;
#53409=CARTESIAN_POINT('Ctrl Pts',(31.5532545328925,535.559370104463,-47.7045493541162)) ;
#53410=CARTESIAN_POINT('Ctrl Pts',(31.5549141180346,535.746853850405,-47.6924529456395)) ;
#53411=CARTESIAN_POINT('Ctrl Pts',(31.5530204561047,535.797877709024,-47.6890942462937)) ;
#53412=CARTESIAN_POINT('Ctrl Pts',(31.5437271359293,535.909551101256,-47.6815511577299)) ;
#53413=CARTESIAN_POINT('Ctrl Pts',(31.535328088606,535.970040391314,-47.6773389707263)) ;
#53414=CARTESIAN_POINT('Ctrl Pts',(31.5066058944178,536.117095652395,-47.6667710894643)) ;
#53415=CARTESIAN_POINT('Ctrl Pts',(31.4826388185315,536.20275469549,-47.6603239369838)) ;
#53416=CARTESIAN_POINT('Ctrl Pts',(31.451963599978,536.286085753953,-47.6538547791721)) ;
#53417=CARTESIAN_POINT('Origin',(29.8885276254069,535.710565160562,-48.522160171753)) ;
#53418=CARTESIAN_POINT('',(31.4519498093678,536.286123215583,-49.053781357604)) ;
#53419=CARTESIAN_POINT('',(31.451949809446,536.28612321537,-48.8631108318347)) ;
#53420=CARTESIAN_POINT('',(31.4519498093678,536.286123215583,-48.5221601717531)) ;
#53421=CARTESIAN_POINT('',(31.5549889082353,535.711664315652,-49.0928401252964)) ;
#53422=CARTESIAN_POINT('Ctrl Pts',(31.5545272755358,535.711644868924,-49.0925752748111)) ;
#53423=CARTESIAN_POINT('Ctrl Pts',(31.55449757292,535.757476270547,-49.0892618616175)) ;
#53424=CARTESIAN_POINT('Ctrl Pts',(31.5525766500511,535.803290525822,-49.0859760681493)) ;
#53425=CARTESIAN_POINT('Ctrl Pts',(31.5462160716639,535.879588900661,-49.0806023568414)) ;
#53426=CARTESIAN_POINT('Ctrl Pts',(31.542816820287,535.910133684156,-49.0784777929953)) ;
#53427=CARTESIAN_POINT('Ctrl Pts',(31.5341919410292,535.97200840949,-49.0742513050239)) ;
#53428=CARTESIAN_POINT('Ctrl Pts',(31.5289119118011,536.003316152231,-49.0721567469035)) ;
#53429=CARTESIAN_POINT('Ctrl Pts',(31.5057653726932,536.120103714187,-49.0644503423696)) ;
#53430=CARTESIAN_POINT('Ctrl Pts',(31.4820903240614,536.204250763452,-49.0591060070419)) ;
#53431=CARTESIAN_POINT('Ctrl Pts',(31.4519498093678,536.286123215583,-49.053781357604)) ;
#53432=CARTESIAN_POINT('',(28.6194567455546,536.789923813611,-49.5221601717529)) ;
#53433=CARTESIAN_POINT('Ctrl Pts',(31.5549889082353,535.711664315652,-49.0928401252965)) ;
#53434=CARTESIAN_POINT('Ctrl Pts',(31.5548945150024,535.651801552434,-49.0970896085957)) ;
#53435=CARTESIAN_POINT('Ctrl Pts',(31.5515477486577,535.591838508281,-49.1013782898962)) ;
#53436=CARTESIAN_POINT('Ctrl Pts',(31.5449734388419,535.532152475187,-49.1056462076814)) ;
#53437=CARTESIAN_POINT('Ctrl Pts',(31.5384062586401,535.472531169551,-49.1099094970558)) ;
#53438=CARTESIAN_POINT('Ctrl Pts',(31.5286187690042,535.413186238494,-49.1141518093791)) ;
#53439=CARTESIAN_POINT('Ctrl Pts',(31.5156726607986,535.354485191027,-49.1183336692113)) ;
#53440=CARTESIAN_POINT('Ctrl Pts',(31.5027355157954,535.295824785069,-49.1225126337444)) ;
#53441=CARTESIAN_POINT('Ctrl Pts',(31.4866441943593,535.237807390759,-49.1266311311775)) ;
#53442=CARTESIAN_POINT('Ctrl Pts',(31.4674949390496,535.180791368193,-49.1306726625041)) ;
#53443=CARTESIAN_POINT('Ctrl Pts',(31.448351369271,535.123792274033,-49.1347129938754)) ;
#53444=CARTESIAN_POINT('Ctrl Pts',(31.4261516385317,535.067794050184,-49.1386764271401)) ;
#53445=CARTESIAN_POINT('Ctrl Pts',(31.4010264095637,535.013145512418,-49.1425699181009)) ;
#53446=CARTESIAN_POINT('Ctrl Pts',(31.3758809737919,534.958453023916,-49.1464665403767)) ;
#53447=CARTESIAN_POINT('Ctrl Pts',(31.3478051928575,534.905112567087,-49.1502932455774)) ;
#53448=CARTESIAN_POINT('Ctrl Pts',(31.3169659928077,534.853462565541,-49.1540793082628)) ;
#53449=CARTESIAN_POINT('Ctrl Pts',(31.2861153343653,534.801793373291,-49.1578667776706)) ;
#53450=CARTESIAN_POINT('Ctrl Pts',(31.2524989797646,534.751816174951,-49.1616138642146)) ;
#53451=CARTESIAN_POINT('Ctrl Pts',(31.2163227255207,534.703855161998,-49.1653690162118)) ;
#53452=CARTESIAN_POINT('Ctrl Pts',(31.1800794842795,534.655805340396,-49.1691311215645)) ;
#53453=CARTESIAN_POINT('Ctrl Pts',(31.1412665653164,534.609779650157,-49.1729018125606)) ;
#53454=CARTESIAN_POINT('Ctrl Pts',(31.1001336553491,534.566083846947,-49.1767432173366)) ;
#53455=CARTESIAN_POINT('Ctrl Pts',(31.0641191958142,534.527825412574,-49.1801066097387)) ;
#53456=CARTESIAN_POINT('Ctrl Pts',(31.0263267587359,534.491353125802,-49.183524739968)) ;
#53457=CARTESIAN_POINT('Ctrl Pts',(30.9869532174238,534.45685407754,-49.1870422345052)) ;
#53458=CARTESIAN_POINT('Ctrl Pts',(30.9869288742596,534.45683274809,-49.1870444092384)) ;
#53459=CARTESIAN_POINT('Ctrl Pts',(30.9869045304909,534.456811419392,-49.1870465840096)) ;
#53460=CARTESIAN_POINT('Ctrl Pts',(30.9868801861176,534.456790091447,-49.1870487588188)) ;
#53461=CARTESIAN_POINT('Ctrl Pts',(30.9451058127731,534.420191838465,-49.1907806803159)) ;
#53462=CARTESIAN_POINT('Ctrl Pts',(30.9013837054678,534.385675350033,-49.1946349063943)) ;
#53463=CARTESIAN_POINT('Ctrl Pts',(30.8559638071929,534.353423514733,-49.1985479657098)) ;
#53464=CARTESIAN_POINT('Ctrl Pts',(30.851836545535,534.350492822056,-49.1989035415761)) ;
#53465=CARTESIAN_POINT('Ctrl Pts',(30.8476953004339,534.347580830664,-49.199259603239)) ;
#53466=CARTESIAN_POINT('Ctrl Pts',(30.8435402806864,534.344687678229,-49.1996161030745)) ;
#53467=CARTESIAN_POINT('Ctrl Pts',(30.7930414398575,534.309525187273,-49.2039488931799)) ;
#53468=CARTESIAN_POINT('Ctrl Pts',(30.7405019731692,534.277144757969,-49.2083457443779)) ;
#53469=CARTESIAN_POINT('Ctrl Pts',(30.6862764220024,534.247746870581,-49.212735632841)) ;
#53470=CARTESIAN_POINT('Ctrl Pts',(30.6328585556239,534.218786862126,-49.2170601343038)) ;
#53471=CARTESIAN_POINT('Ctrl Pts',(30.5778045801627,534.192720780501,-49.2213776000998)) ;
#53472=CARTESIAN_POINT('Ctrl Pts',(30.5214645329549,534.169702898285,-49.2256408785573)) ;
#53473=CARTESIAN_POINT('Ctrl Pts',(30.4651572114663,534.146698386252,-49.2299016806438)) ;
#53474=CARTESIAN_POINT('Ctrl Pts',(30.4075653302754,534.126738409008,-49.2341082270902)) ;
#53475=CARTESIAN_POINT('Ctrl Pts',(30.3490485980044,534.109943273336,-49.2382373652898)) ;
#53476=CARTESIAN_POINT('Ctrl Pts',(30.2905440138085,534.093151624335,-49.2423656462802)) ;
#53477=CARTESIAN_POINT('Ctrl Pts',(30.2311149728027,534.079523540889,-49.2464165514128)) ;
#53478=CARTESIAN_POINT('Ctrl Pts',(30.1711310570779,534.069146167981,-49.2503918060323)) ;
#53479=CARTESIAN_POINT('Ctrl Pts',(30.1094908279039,534.058482248553,-49.2544768278722)) ;
#53480=CARTESIAN_POINT('Ctrl Pts',(30.0472646332882,534.051251403299,-49.2584819767203)) ;
#53481=CARTESIAN_POINT('Ctrl Pts',(29.9848643783669,534.047510007894,-49.2624354936015)) ;
#53482=CARTESIAN_POINT('Ctrl Pts',(29.924057600434,534.043864154206,-49.26628805195)) ;
#53483=CARTESIAN_POINT('Ctrl Pts',(29.8630856380362,534.043531974582,-49.2700919530291)) ;
#53484=CARTESIAN_POINT('Ctrl Pts',(29.8023391303135,534.046526464964,-49.2738948198168)) ;
#53485=CARTESIAN_POINT('Ctrl Pts',(29.7392047762322,534.04963866389,-49.2778471711089)) ;
#53486=CARTESIAN_POINT('Ctrl Pts',(29.6763140819269,534.056345093778,-49.2817988336936)) ;
#53487=CARTESIAN_POINT('Ctrl Pts',(29.6141145081114,534.06660895403,-49.2858211495323)) ;
#53488=CARTESIAN_POINT('Ctrl Pts',(29.560439537276,534.075466127253,-49.2892921971954)) ;
#53489=CARTESIAN_POINT('Ctrl Pts',(29.5072782483975,534.086972424484,-49.2928165217358)) ;
#53490=CARTESIAN_POINT('Ctrl Pts',(29.454924530345,534.101065601861,-49.2964447278837)) ;
#53491=CARTESIAN_POINT('Ctrl Pts',(29.4466432325861,534.103294857062,-49.2970186366061)) ;
#53492=CARTESIAN_POINT('Ctrl Pts',(29.4383820438979,534.105588795292,-49.2975951445327)) ;
#53493=CARTESIAN_POINT('Ctrl Pts',(29.430142016476,534.107947124849,-49.2981744519464)) ;
#53494=CARTESIAN_POINT('Ctrl Pts',(29.4301087180222,534.107956655002,-49.298176792963)) ;
#53495=CARTESIAN_POINT('Ctrl Pts',(29.4300754199139,534.107966186208,-49.2981791340253)) ;
#53496=CARTESIAN_POINT('Ctrl Pts',(29.4300421221512,534.107975718464,-49.2981814751334)) ;
#53497=CARTESIAN_POINT('Ctrl Pts',(29.3771816235799,534.12310826182,-49.3018980053008)) ;
#53498=CARTESIAN_POINT('Ctrl Pts',(29.324995964791,534.140955723634,-49.3057400460438)) ;
#53499=CARTESIAN_POINT('Ctrl Pts',(29.2737680915368,534.161411177651,-49.309644776254)) ;
#53500=CARTESIAN_POINT('Ctrl Pts',(29.2687790857812,534.163403303643,-49.3100250520737)) ;
#53501=CARTESIAN_POINT('Ctrl Pts',(29.2637991871285,534.165420131474,-49.3104059224729)) ;
#53502=CARTESIAN_POINT('Ctrl Pts',(29.2588286712114,534.167461540257,-49.3107873294248)) ;
#53503=CARTESIAN_POINT('Ctrl Pts',(29.2019109528873,534.190837852099,-49.3151548465633)) ;
#53504=CARTESIAN_POINT('Ctrl Pts',(29.1462197990437,534.217442248767,-49.3195920236138)) ;
#53505=CARTESIAN_POINT('Ctrl Pts',(29.0921183275704,534.247085215786,-49.3240255580288)) ;
#53506=CARTESIAN_POINT('Ctrl Pts',(29.0390321042312,534.276171913888,-49.3283758943825)) ;
#53507=CARTESIAN_POINT('Ctrl Pts',(28.9874761485506,534.308183841957,-49.3327224400922)) ;
#53508=CARTESIAN_POINT('Ctrl Pts',(28.9377678747413,534.342912053716,-49.3370161818138)) ;
#53509=CARTESIAN_POINT('Ctrl Pts',(28.8880908369075,534.377618442757,-49.3413072254089)) ;
#53510=CARTESIAN_POINT('Ctrl Pts',(28.8402590636623,534.415037608316,-49.3455453887482)) ;
#53511=CARTESIAN_POINT('Ctrl Pts',(28.7945664451433,534.454934033315,-49.3497053222925)) ;
#53512=CARTESIAN_POINT('Ctrl Pts',(28.748885160238,534.49482056239,-49.3538642240053)) ;
#53513=CARTESIAN_POINT('Ctrl Pts',(28.7053420043622,534.537183120873,-49.3579449241799)) ;
#53514=CARTESIAN_POINT('Ctrl Pts',(28.6642081615329,534.58176007115,-49.3619467722947)) ;
#53515=CARTESIAN_POINT('Ctrl Pts',(28.6216448854951,534.627886105312,-49.3660876877613)) ;
#53516=CARTESIAN_POINT('Ctrl Pts',(28.5816616075933,534.676383345868,-49.3701441435676)) ;
#53517=CARTESIAN_POINT('Ctrl Pts',(28.5445318003552,534.726931753464,-49.3741424304751)) ;
#53518=CARTESIAN_POINT('Ctrl Pts',(28.5086016017281,534.775847017514,-49.3780115387049)) ;
#53519=CARTESIAN_POINT('Ctrl Pts',(28.4753436174409,534.82668300498,-49.3818265568833)) ;
#53520=CARTESIAN_POINT('Ctrl Pts',(28.4449778114948,534.879121020584,-49.3856331128046)) ;
#53521=CARTESIAN_POINT('Ctrl Pts',(28.413091261842,534.934185173704,-49.3896303040733)) ;
#53522=CARTESIAN_POINT('Ctrl Pts',(28.384394710758,534.9910162561,-49.3936185392059)) ;
#53523=CARTESIAN_POINT('Ctrl Pts',(28.3591034283671,535.049209612495,-49.3976698686656)) ;
#53524=CARTESIAN_POINT('Ctrl Pts',(28.3373126243316,535.099348629005,-49.4011604677176)) ;
#53525=CARTESIAN_POINT('Ctrl Pts',(28.3180491561457,535.150499775786,-49.4046985677495)) ;
#53526=CARTESIAN_POINT('Ctrl Pts',(28.3014210364866,535.202377708198,-49.4083359611142)) ;
#53527=CARTESIAN_POINT('Ctrl Pts',(28.2987556707882,535.210693360502,-49.4089190086087)) ;
#53528=CARTESIAN_POINT('Ctrl Pts',(28.2961579274069,535.219027748387,-49.4095046073204)) ;
#53529=CARTESIAN_POINT('Ctrl Pts',(28.2936281503815,535.227379770461,-49.4100929705568)) ;
#53530=CARTESIAN_POINT('Ctrl Pts',(28.2936226661343,535.227397876623,-49.4100942460564)) ;
#53531=CARTESIAN_POINT('Ctrl Pts',(28.2936171822064,535.227415982868,-49.4100955215689)) ;
#53532=CARTESIAN_POINT('Ctrl Pts',(28.293611698598,535.227434089197,-49.4100967970944)) ;
#53533=CARTESIAN_POINT('Ctrl Pts',(28.2773215026631,535.281222691997,-49.4138860101986)) ;
#53534=CARTESIAN_POINT('Ctrl Pts',(28.2638006114948,535.335934037994,-49.4177998091959)) ;
#53535=CARTESIAN_POINT('Ctrl Pts',(28.2531113952247,535.391260793551,-49.4217758640599)) ;
#53536=CARTESIAN_POINT('Ctrl Pts',(28.2520331872799,535.396841534542,-49.4221769237666)) ;
#53537=CARTESIAN_POINT('Ctrl Pts',(28.2509837735385,535.402428496592,-49.4225786168961)) ;
#53538=CARTESIAN_POINT('Ctrl Pts',(28.2499632061062,535.408021337453,-49.4229808794796)) ;
#53539=CARTESIAN_POINT('Ctrl Pts',(28.2388485012066,535.468931350599,-49.4273618049979)) ;
#53540=CARTESIAN_POINT('Ctrl Pts',(28.231156974193,535.530544371899,-49.4318096352455)) ;
#53541=CARTESIAN_POINT('Ctrl Pts',(28.2269237227364,535.592455990411,-49.4362551103338)) ;
#53542=CARTESIAN_POINT('Ctrl Pts',(28.2226957254514,535.654290766273,-49.4406950678456)) ;
#53543=CARTESIAN_POINT('Ctrl Pts',(28.2219170560046,535.716423496026,-49.4451323351127)) ;
#53544=CARTESIAN_POINT('Ctrl Pts',(28.2245843407441,535.778456896699,-49.4495184890573)) ;
#53545=CARTESIAN_POINT('Ctrl Pts',(28.2272491519643,535.840432770401,-49.453900575481)) ;
#53546=CARTESIAN_POINT('Ctrl Pts',(28.2333534079484,535.902309583222,-49.4582315066852)) ;
#53547=CARTESIAN_POINT('Ctrl Pts',(28.242859035928,535.963695323706,-49.4624870479383)) ;
#53548=CARTESIAN_POINT('Ctrl Pts',(28.2523588291084,536.025043384042,-49.4667399770305)) ;
#53549=CARTESIAN_POINT('Ctrl Pts',(28.2652558739135,536.085900991523,-49.470917615664)) ;
#53550=CARTESIAN_POINT('Ctrl Pts',(28.2814779304573,536.145880242774,-49.4750207457855)) ;
#53551=CARTESIAN_POINT('Ctrl Pts',(28.2977013405527,536.205864498632,-49.479124218268)) ;
#53552=CARTESIAN_POINT('Ctrl Pts',(28.3172505126246,536.264970184918,-49.4831533041118)) ;
#53553=CARTESIAN_POINT('Ctrl Pts',(28.3400170427953,536.322813048898,-49.4871327220622)) ;
#53554=CARTESIAN_POINT('Ctrl Pts',(28.3627826259513,536.3806535068,-49.4911119744816)) ;
#53555=CARTESIAN_POINT('Ctrl Pts',(28.3887656233382,536.437231064484,-49.4950418556151)) ;
#53556=CARTESIAN_POINT('Ctrl Pts',(28.4178176061229,536.49216708494,-49.4989678566015)) ;
#53557=CARTESIAN_POINT('Ctrl Pts',(28.4468982401289,536.547157283593,-49.5028977294311)) ;
#53558=CARTESIAN_POINT('Ctrl Pts',(28.4790543540341,536.600502320741,-49.5068242184869)) ;
#53559=CARTESIAN_POINT('Ctrl Pts',(28.5140911814731,536.651832170997,-49.5108078539714)) ;
#53560=CARTESIAN_POINT('Ctrl Pts',(28.5467730958851,536.699712013306,-49.514523739326)) ;
#53561=CARTESIAN_POINT('Ctrl Pts',(28.5819613399247,536.745838071324,-49.5182899981151)) ;
#53562=CARTESIAN_POINT('Ctrl Pts',(28.6194567455546,536.789923813611,-49.5221601717528)) ;
#53563=CARTESIAN_POINT('',(31.1431801000586,536.807976208783,-49.5221526632306)) ;
#53564=CARTESIAN_POINT('Origin',(29.8885276254068,535.710565160562,-49.522160171753)) ;
#53565=CARTESIAN_POINT('',(31.5540494077382,535.71142659878,-48.8998528498641)) ;
#53566=CARTESIAN_POINT('Ctrl Pts',(31.1431801122076,536.807976219409,-49.5221526630917)) ;
#53567=CARTESIAN_POINT('Ctrl Pts',(31.1083565274205,536.847742286154,-49.5185433692491)) ;
#53568=CARTESIAN_POINT('Ctrl Pts',(31.0715379965842,536.885881586539,-49.5148367719832)) ;
#53569=CARTESIAN_POINT('Ctrl Pts',(31.0329178907796,536.922204517176,-49.5110871617097)) ;
#53570=CARTESIAN_POINT('Ctrl Pts',(30.9888693681021,536.963632975243,-49.5068105086626)) ;
#53571=CARTESIAN_POINT('Ctrl Pts',(30.9424762407452,537.002699349067,-49.5024784623692)) ;
#53572=CARTESIAN_POINT('Ctrl Pts',(30.894041810257,537.03916323982,-49.4981571537409)) ;
#53573=CARTESIAN_POINT('Ctrl Pts',(30.8456567620084,537.075589953124,-49.4938402509847)) ;
#53574=CARTESIAN_POINT('Ctrl Pts',(30.7952347034472,537.109419769151,-49.4895343620322)) ;
#53575=CARTESIAN_POINT('Ctrl Pts',(30.7430951129014,537.140447259709,-49.4852846612071)) ;
#53576=CARTESIAN_POINT('Ctrl Pts',(30.6909888978209,537.171454889028,-49.4810376806901)) ;
#53577=CARTESIAN_POINT('Ctrl Pts',(30.6371673879947,537.199663874653,-49.4768469345805)) ;
#53578=CARTESIAN_POINT('Ctrl Pts',(30.581965351342,537.224900595741,-49.4727337206037)) ;
#53579=CARTESIAN_POINT('Ctrl Pts',(30.5267777051169,537.250130737957,-49.4686215788865)) ;
#53580=CARTESIAN_POINT('Ctrl Pts',(30.4702102626389,537.272390107686,-49.4645869194723)) ;
#53581=CARTESIAN_POINT('Ctrl Pts',(30.4126130901018,537.291536378296,-49.4606264509924)) ;
#53582=CARTESIAN_POINT('Ctrl Pts',(30.3549673948026,537.310698778691,-49.4566626460141)) ;
#53583=CARTESIAN_POINT('Ctrl Pts',(30.2962902352208,537.326742637295,-49.4527730331063)) ;
#53584=CARTESIAN_POINT('Ctrl Pts',(30.2369480740712,537.33955838851,-49.4489306788226)) ;
#53585=CARTESIAN_POINT('Ctrl Pts',(30.1775836267898,537.35237895272,-49.4450868815308)) ;
#53586=CARTESIAN_POINT('Ctrl Pts',(30.1175536955959,537.361968645317,-49.4412901053197)) ;
#53587=CARTESIAN_POINT('Ctrl Pts',(30.0572405651505,537.368254886535,-49.4374926831251)) ;
#53588=CARTESIAN_POINT('Ctrl Pts',(29.9968128635493,537.374553069131,-49.4336880473262)) ;
#53589=CARTESIAN_POINT('Ctrl Pts',(29.9361009840112,537.377534707185,-49.4298822893108)) ;
#53590=CARTESIAN_POINT('Ctrl Pts',(29.8755041032753,537.377170570117,-49.4260122312284)) ;
#53591=CARTESIAN_POINT('Ctrl Pts',(29.8210497178999,537.376843344359,-49.422534467494)) ;
#53592=CARTESIAN_POINT('Ctrl Pts',(29.7666878020697,537.373814310548,-49.4190041894054)) ;
#53593=CARTESIAN_POINT('Ctrl Pts',(29.7127183637283,537.368098938728,-49.4153710491561)) ;
#53594=CARTESIAN_POINT('Ctrl Pts',(29.707871034377,537.367585605804,-49.4150447343397)) ;
#53595=CARTESIAN_POINT('Ctrl Pts',(29.7030268418567,537.367050621183,-49.4147175897395)) ;
#53596=CARTESIAN_POINT('Ctrl Pts',(29.6981859859229,537.366494006858,-49.4143895788765)) ;
#53597=CARTESIAN_POINT('Ctrl Pts',(29.698153754034,537.366490300751,-49.4143873948805)) ;
#53598=CARTESIAN_POINT('Ctrl Pts',(29.6981215222931,537.366486593685,-49.4143852108462)) ;
#53599=CARTESIAN_POINT('Ctrl Pts',(29.6980892907001,537.36648288566,-49.4143830267734)) ;
#53600=CARTESIAN_POINT('Ctrl Pts',(29.6429162247681,537.360135600715,-49.4106443970974)) ;
#53601=CARTESIAN_POINT('Ctrl Pts',(29.5879781605852,537.350947335582,-49.4067833237044)) ;
#53602=CARTESIAN_POINT('Ctrl Pts',(29.5335777348821,537.338980388243,-49.4028628644713)) ;
#53603=CARTESIAN_POINT('Ctrl Pts',(29.5285151673266,537.337866730059,-49.4024980219272)) ;
#53604=CARTESIAN_POINT('Ctrl Pts',(29.5234572819973,537.336729034071,-49.4021326650789)) ;
#53605=CARTESIAN_POINT('Ctrl Pts',(29.5184043383932,537.335567367242,-49.4017668447478)) ;
#53606=CARTESIAN_POINT('Ctrl Pts',(29.4584525440487,537.321784507932,-49.3974264865378)) ;
#53607=CARTESIAN_POINT('Ctrl Pts',(29.3991919237932,537.304623258597,-49.3930215428258)) ;
#53608=CARTESIAN_POINT('Ctrl Pts',(29.3410079109624,537.284211436378,-49.3886228235456)) ;
#53609=CARTESIAN_POINT('Ctrl Pts',(29.283564807459,537.264059536236,-49.3842801171112)) ;
#53610=CARTESIAN_POINT('Ctrl Pts',(29.2271708358056,537.240739690067,-49.3799437695657)) ;
#53611=CARTESIAN_POINT('Ctrl Pts',(29.1721765345475,537.214408245045,-49.3756613760682)) ;
#53612=CARTESIAN_POINT('Ctrl Pts',(29.1172154023898,537.188092681492,-49.3713815654409)) ;
#53613=CARTESIAN_POINT('Ctrl Pts',(29.0636521680889,537.158769250228,-49.3671557788563)) ;
#53614=CARTESIAN_POINT('Ctrl Pts',(29.0118186029896,537.126624263931,-49.3630077155754)) ;
#53615=CARTESIAN_POINT('Ctrl Pts',(28.9599971726063,537.094486803072,-49.3588606233943)) ;
#53616=CARTESIAN_POINT('Ctrl Pts',(28.9099046329241,537.059529090471,-49.3547912200999)) ;
#53617=CARTESIAN_POINT('Ctrl Pts',(28.8618547835675,537.021966993312,-49.3507983884807)) ;
#53618=CARTESIAN_POINT('Ctrl Pts',(28.8126618845849,536.983511337865,-49.3467105720748)) ;
#53619=CARTESIAN_POINT('Ctrl Pts',(28.7656102528472,536.942325674075,-49.3427029869773)) ;
#53620=CARTESIAN_POINT('Ctrl Pts',(28.7210159321545,536.898674881616,-49.3387484432116)) ;
#53621=CARTESIAN_POINT('Ctrl Pts',(28.6774021379088,536.855983869591,-49.3348808507591)) ;
#53622=CARTESIAN_POINT('Ctrl Pts',(28.6361389815893,536.810934885481,-49.3310636388541)) ;
#53623=CARTESIAN_POINT('Ctrl Pts',(28.5974995922091,536.763808969429,-49.3272499272855)) ;
#53624=CARTESIAN_POINT('Ctrl Pts',(28.5575571652059,536.715093824286,-49.3233076057742)) ;
#53625=CARTESIAN_POINT('Ctrl Pts',(28.5204191540007,536.664158850631,-49.319368594247)) ;
#53626=CARTESIAN_POINT('Ctrl Pts',(28.4863559239369,536.611354798058,-49.315363497479)) ;
#53627=CARTESIAN_POINT('Ctrl Pts',(28.4567192744058,536.565412730996,-49.3118788705359)) ;
#53628=CARTESIAN_POINT('Ctrl Pts',(28.4294095880391,536.518055123191,-49.3083435685584)) ;
#53629=CARTESIAN_POINT('Ctrl Pts',(28.4045804526383,536.469543561243,-49.3047069758659)) ;
#53630=CARTESIAN_POINT('Ctrl Pts',(28.400885802758,536.462324895202,-49.3041658399569)) ;
#53631=CARTESIAN_POINT('Ctrl Pts',(28.3972459921483,536.455080639415,-49.303622461235)) ;
#53632=CARTESIAN_POINT('Ctrl Pts',(28.3936614376786,536.447811612819,-49.3030766729295)) ;
#53633=CARTESIAN_POINT('Ctrl Pts',(28.3936479789086,536.447784320122,-49.3030746236821)) ;
#53634=CARTESIAN_POINT('Ctrl Pts',(28.3936345209176,536.447757027077,-49.3030725744006)) ;
#53635=CARTESIAN_POINT('Ctrl Pts',(28.3936210637055,536.447729733682,-49.3030705250852)) ;
#53636=CARTESIAN_POINT('Ctrl Pts',(28.3691053918656,536.398008000487,-49.2993371853412)) ;
#53637=CARTESIAN_POINT('Ctrl Pts',(28.3470945059155,536.346945626636,-49.295481286779)) ;
#53638=CARTESIAN_POINT('Ctrl Pts',(28.3277004536284,536.294829589099,-49.2915660505046)) ;
#53639=CARTESIAN_POINT('Ctrl Pts',(28.3259023440706,536.289997677551,-49.2912030513922)) ;
#53640=CARTESIAN_POINT('Ctrl Pts',(28.3241267206343,536.28515674484,-49.2908395422142)) ;
#53641=CARTESIAN_POINT('Ctrl Pts',(28.3223736671063,536.280307041621,-49.2904755733562)) ;
#53642=CARTESIAN_POINT('Ctrl Pts',(28.3014560780051,536.222439955653,-49.2861326648845)) ;
#53643=CARTESIAN_POINT('Ctrl Pts',(28.2837527935745,536.163318227504,-49.2817249759682)) ;
#53644=CARTESIAN_POINT('Ctrl Pts',(28.2693664506353,536.103336017163,-49.2773238859157)) ;
#53645=CARTESIAN_POINT('Ctrl Pts',(28.2551960586974,536.044254189806,-49.2729888598941)) ;
#53646=CARTESIAN_POINT('Ctrl Pts',(28.2442433287989,535.984337528399,-49.2686605187971)) ;
#53647=CARTESIAN_POINT('Ctrl Pts',(28.2365673045768,535.923963862056,-49.264386520501)) ;
#53648=CARTESIAN_POINT('Ctrl Pts',(28.2288960412449,535.863627641189,-49.260115173061)) ;
#53649=CARTESIAN_POINT('Ctrl Pts',(28.2244972935664,535.802834968857,-49.2558982350145)) ;
#53650=CARTESIAN_POINT('Ctrl Pts',(28.2233947577476,535.741964260642,-49.2517595022522)) ;
#53651=CARTESIAN_POINT('Ctrl Pts',(28.2222924944977,535.681108600886,-49.2476217926676)) ;
#53652=CARTESIAN_POINT('Ctrl Pts',(28.2244848456945,535.620174964973,-49.2435622517888)) ;
#53653=CARTESIAN_POINT('Ctrl Pts',(28.2299609162811,535.559542739129,-49.2395799019118)) ;
#53654=CARTESIAN_POINT('Ctrl Pts',(28.2355899482467,535.497216892151,-49.2354863142924)) ;
#53655=CARTESIAN_POINT('Ctrl Pts',(28.2446890651011,535.435209601131,-49.2314742813798)) ;
#53656=CARTESIAN_POINT('Ctrl Pts',(28.2572067248696,535.373933582006,-49.2275164187219)) ;
#53657=CARTESIAN_POINT('Ctrl Pts',(28.269399732289,535.314246789933,-49.2236612053957)) ;
#53658=CARTESIAN_POINT('Ctrl Pts',(28.2848363846619,535.255253970115,-49.2198570207253)) ;
#53659=CARTESIAN_POINT('Ctrl Pts',(28.3034288465167,535.197335591793,-49.21605708333)) ;
#53660=CARTESIAN_POINT('Ctrl Pts',(28.3227638757555,535.137104001859,-49.2121053796116)) ;
#53661=CARTESIAN_POINT('Ctrl Pts',(28.3455126512619,535.078034749291,-49.2081578506276)) ;
#53662=CARTESIAN_POINT('Ctrl Pts',(28.3715245405358,535.020551048144,-49.2041438876027)) ;
#53663=CARTESIAN_POINT('Ctrl Pts',(28.3940266130001,534.970823694814,-49.2006715336377)) ;
#53664=CARTESIAN_POINT('Ctrl Pts',(28.4189708581868,534.922281953056,-49.1971488057963)) ;
#53665=CARTESIAN_POINT('Ctrl Pts',(28.4462206482126,534.875195835559,-49.193525032886)) ;
#53666=CARTESIAN_POINT('Ctrl Pts',(28.4504560760141,534.86787725252,-49.1929617908017)) ;
#53667=CARTESIAN_POINT('Ctrl Pts',(28.4547471865727,534.860593733717,-49.1923961076298)) ;
#53668=CARTESIAN_POINT('Ctrl Pts',(28.4590934528131,534.853346180448,-49.1918277931033)) ;
#53669=CARTESIAN_POINT('Ctrl Pts',(28.4591087695015,534.853320639326,-49.1918257903045)) ;
#53670=CARTESIAN_POINT('Ctrl Pts',(28.4591240868749,534.853295098651,-49.1918237874731)) ;
#53671=CARTESIAN_POINT('Ctrl Pts',(28.4591394049333,534.853269558422,-49.191821784609)) ;
#53672=CARTESIAN_POINT('Ctrl Pts',(28.4876505307747,534.80573215835,-49.1880939028384)) ;
#53673=CARTESIAN_POINT('Ctrl Pts',(28.5186446965708,534.759574814024,-49.1842429132903)) ;
#53674=CARTESIAN_POINT('Ctrl Pts',(28.551941243101,534.715046859562,-49.1803319601417)) ;
#53675=CARTESIAN_POINT('Ctrl Pts',(28.555055086558,534.710882671557,-49.1799662136262)) ;
#53676=CARTESIAN_POINT('Ctrl Pts',(28.5581890305973,534.706732746596,-49.1795999426863)) ;
#53677=CARTESIAN_POINT('Ctrl Pts',(28.561342905434,534.702597295999,-49.1792331989668)) ;
#53678=CARTESIAN_POINT('Ctrl Pts',(28.598655724194,534.653671664327,-49.1748943324464)) ;
#53679=CARTESIAN_POINT('Ctrl Pts',(28.6387637095503,534.606769532632,-49.1704899595146)) ;
#53680=CARTESIAN_POINT('Ctrl Pts',(28.6813909443396,534.562190298489,-49.166091475398)) ;
#53681=CARTESIAN_POINT('Ctrl Pts',(28.7234055354259,534.518251762416,-49.1617562068197)) ;
#53682=CARTESIAN_POINT('Ctrl Pts',(28.7678672342527,534.47656946284,-49.1574269461224)) ;
#53683=CARTESIAN_POINT('Ctrl Pts',(28.8144898039614,534.437397772436,-49.1531515172141)) ;
#53684=CARTESIAN_POINT('Ctrl Pts',(28.8610837398425,534.398250139811,-49.1488787141134)) ;
#53685=CARTESIAN_POINT('Ctrl Pts',(28.9098358358941,534.361609916743,-49.1446598119804)) ;
#53686=CARTESIAN_POINT('Ctrl Pts',(28.9604402823742,534.327702017728,-49.1405187574703)) ;
#53687=CARTESIAN_POINT('Ctrl Pts',(29.0110324645635,534.293802336496,-49.1363787065697)) ;
#53688=CARTESIAN_POINT('Ctrl Pts',(29.063476100067,534.262633691478,-49.1323164682545)) ;
#53689=CARTESIAN_POINT('Ctrl Pts',(29.1174458832626,534.234392420078,-49.1283311859706)) ;
#53690=CARTESIAN_POINT('Ctrl Pts',(29.1728601611725,534.205395274468,-49.1242392380889)) ;
#53691=CARTESIAN_POINT('Ctrl Pts',(29.2298835036641,534.179484631722,-49.120228407675)) ;
#53692=CARTESIAN_POINT('Ctrl Pts',(29.2881418672384,534.156840117488,-49.1162715094966)) ;
#53693=CARTESIAN_POINT('Ctrl Pts',(29.3449540373261,534.134757725959,-49.1124128365347)) ;
#53694=CARTESIAN_POINT('Ctrl Pts',(29.4029406297045,534.115781507823,-49.108605087979)) ;
#53695=CARTESIAN_POINT('Ctrl Pts',(29.4617338381584,534.100043761848,-49.1048015503335)) ;
#53696=CARTESIAN_POINT('Ctrl Pts',(29.5227719799159,534.083705092892,-49.1008527801253)) ;
#53697=CARTESIAN_POINT('Ctrl Pts',(29.584679651964,534.070857797052,-49.0969081281491)) ;
#53698=CARTESIAN_POINT('Ctrl Pts',(29.6470212864538,534.061604094066,-49.0928973776251)) ;
#53699=CARTESIAN_POINT('Ctrl Pts',(29.7010602111156,534.053582806806,-49.0894207821336)) ;
#53700=CARTESIAN_POINT('Ctrl Pts',(29.7554261004178,534.048261373202,-49.0858938663866)) ;
#53701=CARTESIAN_POINT('Ctrl Pts',(29.809817441644,534.045671351363,-49.082265892419)) ;
#53702=CARTESIAN_POINT('Ctrl Pts',(29.818144826443,534.045274815664,-49.0817104449049)) ;
#53703=CARTESIAN_POINT('Ctrl Pts',(29.8264728825017,534.044942238459,-49.0811526285855)) ;
#53704=CARTESIAN_POINT('Ctrl Pts',(29.8348006109187,534.04467366373,-49.0805922613776)) ;
#53705=CARTESIAN_POINT('Ctrl Pts',(29.8348300835497,534.044672713218,-49.0805902781842)) ;
#53706=CARTESIAN_POINT('Ctrl Pts',(29.8348595561766,534.044671763508,-49.0805882949589)) ;
#53707=CARTESIAN_POINT('Ctrl Pts',(29.8348890287994,534.044670814599,-49.0805863117016)) ;
#53708=CARTESIAN_POINT('Ctrl Pts',(29.890318812835,534.042886182233,-49.076856357823)) ;
#53709=CARTESIAN_POINT('Ctrl Pts',(29.9459332549338,534.043938850658,-49.0730035477567)) ;
#53710=CARTESIAN_POINT('Ctrl Pts',(30.0014245838222,534.047811909075,-49.069091030408)) ;
#53711=CARTESIAN_POINT('Ctrl Pts',(30.0065968818473,534.048172913448,-49.0687263481025)) ;
#53712=CARTESIAN_POINT('Ctrl Pts',(30.0117680804775,534.048558398599,-49.0683611470636)) ;
#53713=CARTESIAN_POINT('Ctrl Pts',(30.0169379125116,534.04896833648,-49.0679954784291)) ;
#53714=CARTESIAN_POINT('Ctrl Pts',(30.0782738004613,534.053831918855,-49.0636571149693)) ;
#53715=CARTESIAN_POINT('Ctrl Pts',(30.1394223551762,534.062140739775,-49.0592535987701)) ;
#53716=CARTESIAN_POINT('Ctrl Pts',(30.1999826224849,534.073824994113,-49.0548561917299)) ;
#53717=CARTESIAN_POINT('Ctrl Pts',(30.2596857992854,534.085343884857,-49.0505210198152)) ;
#53718=CARTESIAN_POINT('Ctrl Pts',(30.3188173992538,534.1001429346,-49.0461920725626)) ;
#53719=CARTESIAN_POINT('Ctrl Pts',(30.3770084588698,534.118119245693,-49.041917081509)) ;
#53720=CARTESIAN_POINT('Ctrl Pts',(30.435163997499,534.136084583686,-49.0376446999954)) ;
#53721=CARTESIAN_POINT('Ctrl Pts',(30.4923802107248,534.157223194246,-49.0334263437376)) ;
#53722=CARTESIAN_POINT('Ctrl Pts',(30.5483022909304,534.181399772607,-49.029285862068)) ;
#53723=CARTESIAN_POINT('Ctrl Pts',(30.6042110070796,534.205570573336,-49.0251463698758)) ;
#53724=CARTESIAN_POINT('Ctrl Pts',(30.6588261784475,534.232777910659,-49.0210847173902)) ;
#53725=CARTESIAN_POINT('Ctrl Pts',(30.7118064549694,534.262854609005,-49.0170999506058)) ;
#53726=CARTESIAN_POINT('Ctrl Pts',(30.7661832550543,534.293724108384,-49.0130101481162)) ;
#53727=CARTESIAN_POINT('Ctrl Pts',(30.8188376283895,534.327616516861,-49.0090013227196)) ;
#53728=CARTESIAN_POINT('Ctrl Pts',(30.8694162793749,534.364314886816,-49.0050462274439)) ;
#53729=CARTESIAN_POINT('Ctrl Pts',(30.9187591536091,534.400116613789,-49.0011877661174)) ;
#53730=CARTESIAN_POINT('Ctrl Pts',(30.9661263148132,534.438588930043,-48.9973800789544)) ;
#53731=CARTESIAN_POINT('Ctrl Pts',(31.0112072094342,534.479494229899,-48.9935763828663)) ;
#53732=CARTESIAN_POINT('Ctrl Pts',(31.0579816592757,534.521936220291,-48.9896297932216)) ;
#53733=CARTESIAN_POINT('Ctrl Pts',(31.1022941894427,534.566998009614,-48.9856870776737)) ;
#53734=CARTESIAN_POINT('Ctrl Pts',(31.1438233851107,534.614369265271,-48.9816781001226)) ;
#53735=CARTESIAN_POINT('Ctrl Pts',(31.1798330563521,534.655444545325,-48.9782019441002)) ;
#53736=CARTESIAN_POINT('Ctrl Pts',(31.2137507985412,534.698256794709,-48.9746753141325)) ;
#53737=CARTESIAN_POINT('Ctrl Pts',(31.2453868414937,534.742569778528,-48.9710475161283)) ;
#53738=CARTESIAN_POINT('Ctrl Pts',(31.2502187328431,534.749337866544,-48.9704934289493)) ;
#53739=CARTESIAN_POINT('Ctrl Pts',(31.2549974929727,534.756140990006,-48.9699369817631)) ;
#53740=CARTESIAN_POINT('Ctrl Pts',(31.2597225482586,534.762978339268,-48.9693779939512)) ;
#53741=CARTESIAN_POINT('Ctrl Pts',(31.2597394148422,534.763002745908,-48.9693759985852)) ;
#53742=CARTESIAN_POINT('Ctrl Pts',(31.2597562807416,534.763027152984,-48.9693740031868)) ;
#53743=CARTESIAN_POINT('Ctrl Pts',(31.2597731459568,534.763051560497,-48.969372007756)) ;
#53744=CARTESIAN_POINT('Ctrl Pts',(31.2915091719242,534.808980262594,-48.9656171168737)) ;
#53745=CARTESIAN_POINT('Ctrl Pts',(31.3209268984216,534.856619043449,-48.9617379323563)) ;
#53746=CARTESIAN_POINT('Ctrl Pts',(31.3478742086198,534.905698408403,-48.9577986482251)) ;
#53747=CARTESIAN_POINT('Ctrl Pts',(31.3505683801692,534.91060532593,-48.957404801598)) ;
#53748=CARTESIAN_POINT('Ctrl Pts',(31.3532378596413,534.915526600376,-48.9570103542243)) ;
#53749=CARTESIAN_POINT('Ctrl Pts',(31.355882496973,534.920461933907,-48.956615370258)) ;
#53750=CARTESIAN_POINT('Ctrl Pts',(31.3849303162123,534.974670000392,-48.9522769973864)) ;
#53751=CARTESIAN_POINT('Ctrl Pts',(31.4109814479544,535.03058020536,-48.9478745219973)) ;
#53752=CARTESIAN_POINT('Ctrl Pts',(31.4338797458221,535.087824156773,-48.9434785903879)) ;
#53753=CARTESIAN_POINT('Ctrl Pts',(31.4567428684039,535.144980172726,-48.9390894116014)) ;
#53754=CARTESIAN_POINT('Ctrl Pts',(31.4764632128134,535.203465830496,-48.9347070927535)) ;
#53755=CARTESIAN_POINT('Ctrl Pts',(31.492922782912,535.262907965774,-48.9303804733937)) ;
#53756=CARTESIAN_POINT('Ctrl Pts',(31.5093675553255,535.322296660651,-48.9260577438044)) ;
#53757=CARTESIAN_POINT('Ctrl Pts',(31.5225575510663,535.382640158892,-48.921790753626)) ;
#53758=CARTESIAN_POINT('Ctrl Pts',(31.5324086973159,535.443559475755,-48.9176032626775)) ;
#53759=CARTESIAN_POINT('Ctrl Pts',(31.5422547457475,535.5044472678,-48.9134179386918)) ;
#53760=CARTESIAN_POINT('Ctrl Pts',(31.5487653550974,535.56591031728,-48.9093120369593)) ;
#53761=CARTESIAN_POINT('Ctrl Pts',(31.5518895224363,535.627562779872,-48.905283292726)) ;
#53762=CARTESIAN_POINT('Ctrl Pts',(31.5533047402245,535.655490753082,-48.9034583102956)) ;
#53763=CARTESIAN_POINT('Ctrl Pts',(31.554025511204,535.683457489442,-48.9016488068729)) ;
#53764=CARTESIAN_POINT('Ctrl Pts',(31.5540494077382,535.71142659878,-48.8998528498641)) ;
#53765=CARTESIAN_POINT('Ctrl Pts',(31.5545274117139,535.711408976249,-48.8995776947983)) ;
#53766=CARTESIAN_POINT('Ctrl Pts',(31.5544905135946,535.784259315344,-48.8949589420851)) ;
#53767=CARTESIAN_POINT('Ctrl Pts',(31.5496754062171,535.857032561577,-48.8904717193232)) ;
#53768=CARTESIAN_POINT('Ctrl Pts',(31.5263269800765,536.033357813305,-48.8795942337981)) ;
#53769=CARTESIAN_POINT('Ctrl Pts',(31.5027341268391,536.135905818928,-48.8732677271662)) ;
#53770=CARTESIAN_POINT('Ctrl Pts',(31.4640228932515,536.252496795028,-48.86542611162)) ;
#53771=CARTESIAN_POINT('Ctrl Pts',(31.4581209925059,536.269360067985,-48.8642750641629)) ;
#53772=CARTESIAN_POINT('Ctrl Pts',(31.4519498095241,536.286123215158,-48.8631108318347)) ;
#53773=CARTESIAN_POINT('Origin',(179.888527625416,585.710565160536,-48.5221601717598)) ;
#53774=CARTESIAN_POINT('',(181.452228406464,586.286162990338,-47.6539333933559)) ;
#53775=CARTESIAN_POINT('',(181.451958155526,586.286100543914,-47.5221601717599)) ;
#53776=CARTESIAN_POINT('',(181.451958155526,586.286100543914,-48.5221601717599)) ;
#53777=CARTESIAN_POINT('',(179.965027641828,587.375705669063,-47.522167780513)) ;
#53778=CARTESIAN_POINT('Origin',(179.888527625416,585.710565160536,-47.5221601717598)) ;
#53779=CARTESIAN_POINT('Ctrl Pts',(179.965027642569,587.375705685183,-47.5221677806499)) ;
#53780=CARTESIAN_POINT('Ctrl Pts',(180.01762246723,587.373258842512,-47.525762311554)) ;
#53781=CARTESIAN_POINT('Ctrl Pts',(180.070188242169,587.368258285171,-47.5294532441289)) ;
#53782=CARTESIAN_POINT('Ctrl Pts',(180.122459260841,587.360736681846,-47.53318691807)) ;
#53783=CARTESIAN_POINT('Ctrl Pts',(180.18231591942,587.35212353342,-47.5374624277505)) ;
#53784=CARTESIAN_POINT('Ctrl Pts',(180.241787318519,587.340204233137,-47.5417934229157)) ;
#53785=CARTESIAN_POINT('Ctrl Pts',(180.300496361892,587.325066084908,-47.5461137620433)) ;
#53786=CARTESIAN_POINT('Ctrl Pts',(180.359145578899,587.309943362931,-47.5504296986093)) ;
#53787=CARTESIAN_POINT('Ctrl Pts',(180.417034131193,587.291608629036,-47.55473470291)) ;
#53788=CARTESIAN_POINT('Ctrl Pts',(180.473802187684,587.270183631508,-47.5589836032974)) ;
#53789=CARTESIAN_POINT('Ctrl Pts',(180.530533932692,587.248772338403,-47.563229785891)) ;
#53790=CARTESIAN_POINT('Ctrl Pts',(180.586146665303,587.224274823582,-47.5674198182745)) ;
#53791=CARTESIAN_POINT('Ctrl Pts',(180.640295894203,587.196844615246,-47.5715324169017)) ;
#53792=CARTESIAN_POINT('Ctrl Pts',(180.694431029055,587.169421546487,-47.575643945095)) ;
#53793=CARTESIAN_POINT('Ctrl Pts',(180.747103370465,587.139067283153,-47.5796780894175)) ;
#53794=CARTESIAN_POINT('Ctrl Pts',(180.797983356651,587.105966823259,-47.5836381646155)) ;
#53795=CARTESIAN_POINT('Ctrl Pts',(180.848906212481,587.07283847411,-47.5876015764303)) ;
#53796=CARTESIAN_POINT('Ctrl Pts',(180.898033538017,587.036959177886,-47.5914909183927)) ;
#53797=CARTESIAN_POINT('Ctrl Pts',(180.945051161067,586.998547180004,-47.5953331537656)) ;
#53798=CARTESIAN_POINT('Ctrl Pts',(180.992086453646,586.960120746644,-47.5991768330755)) ;
#53799=CARTESIAN_POINT('Ctrl Pts',(181.037010181813,586.919159509257,-47.6029736437573)) ;
#53800=CARTESIAN_POINT('Ctrl Pts',(181.079527223904,586.875917151516,-47.606771285106)) ;
#53801=CARTESIAN_POINT('Ctrl Pts',(181.122125003189,586.832592679251,-47.6105761379374)) ;
#53802=CARTESIAN_POINT('Ctrl Pts',(181.162306470872,586.786978160473,-47.6143822988784)) ;
#53803=CARTESIAN_POINT('Ctrl Pts',(181.199799867271,586.739367527627,-47.6182529742086)) ;
#53804=CARTESIAN_POINT('Ctrl Pts',(181.233488265211,586.696588635888,-47.6217308360014)) ;
#53805=CARTESIAN_POINT('Ctrl Pts',(181.265006782421,586.652197947963,-47.6252613718127)) ;
#53806=CARTESIAN_POINT('Ctrl Pts',(181.294180528072,586.606439609925,-47.6288949212148)) ;
#53807=CARTESIAN_POINT('Ctrl Pts',(181.296772590363,586.602374020817,-47.6292177589642)) ;
#53808=CARTESIAN_POINT('Ctrl Pts',(181.299346174913,586.598297624356,-47.6295414099205)) ;
#53809=CARTESIAN_POINT('Ctrl Pts',(181.30190117783,586.594210584967,-47.6298659093913)) ;
#53810=CARTESIAN_POINT('Ctrl Pts',(181.301919148052,586.594181839401,-47.6298681917086)) ;
#53811=CARTESIAN_POINT('Ctrl Pts',(181.301937117354,586.594153093309,-47.6298704740679)) ;
#53812=CARTESIAN_POINT('Ctrl Pts',(181.301955085738,586.594124346691,-47.6298727564692)) ;
#53813=CARTESIAN_POINT('Ctrl Pts',(181.331814495238,586.546353935988,-47.6336655937755)) ;
#53814=CARTESIAN_POINT('Ctrl Pts',(181.35923032566,586.496963105049,-47.6375837284716)) ;
#53815=CARTESIAN_POINT('Ctrl Pts',(181.384064198115,586.446231808426,-47.6415618847391)) ;
#53816=CARTESIAN_POINT('Ctrl Pts',(181.386707431822,586.440832140151,-47.6419853062879)) ;
#53817=CARTESIAN_POINT('Ctrl Pts',(181.389321417815,586.435417334652,-47.6424094078064)) ;
#53818=CARTESIAN_POINT('Ctrl Pts',(181.391905992078,586.429987764067,-47.6428341105854)) ;
#53819=CARTESIAN_POINT('Ctrl Pts',(181.414235691607,586.383078421412,-47.6465033746424)) ;
#53820=CARTESIAN_POINT('Ctrl Pts',(181.434370916039,586.335062710703,-47.6502174215273)) ;
#53821=CARTESIAN_POINT('Ctrl Pts',(181.452228406464,586.286162990338,-47.6539333933559)) ;
#53822=CARTESIAN_POINT('Origin',(179.888527625416,585.710565160536,-48.5221601717598)) ;
#53823=CARTESIAN_POINT('',(181.451958152973,586.286100550849,-48.3557104975402)) ;
#53824=CARTESIAN_POINT('',(181.451938907901,586.286090578308,-48.1612832669077)) ;
#53825=CARTESIAN_POINT('',(181.451958155526,586.286100543914,-48.5221601717599)) ;
#53826=CARTESIAN_POINT('',(181.523656952667,585.391334705907,-47.5221601717598)) ;
#53827=CARTESIAN_POINT('Ctrl Pts',(181.451938907901,586.286090578308,-48.1612832669077)) ;
#53828=CARTESIAN_POINT('Ctrl Pts',(181.430789073677,586.343107213038,-48.156957614088)) ;
#53829=CARTESIAN_POINT('Ctrl Pts',(181.406506905519,586.399019819855,-48.1526546256006)) ;
#53830=CARTESIAN_POINT('Ctrl Pts',(181.379252048762,586.453481920139,-48.1484152340185)) ;
#53831=CARTESIAN_POINT('Ctrl Pts',(181.352010931791,586.507916564852,-48.1441779796091)) ;
#53832=CARTESIAN_POINT('Ctrl Pts',(181.32180018323,586.560902211722,-48.1400043496734)) ;
#53833=CARTESIAN_POINT('Ctrl Pts',(181.288809381259,586.612110273712,-48.1359109220406)) ;
#53834=CARTESIAN_POINT('Ctrl Pts',(181.255822943183,586.663311562101,-48.1318180358703)) ;
#53835=CARTESIAN_POINT('Ctrl Pts',(181.220057144157,586.71273567089,-48.1278052990032)) ;
#53836=CARTESIAN_POINT('Ctrl Pts',(181.181731570267,586.760071659393,-48.123864562092)) ;
#53837=CARTESIAN_POINT('Ctrl Pts',(181.143369057262,586.807453271466,-48.1199200270032)) ;
#53838=CARTESIAN_POINT('Ctrl Pts',(181.102441704118,586.852742558136,-48.1160474809012)) ;
#53839=CARTESIAN_POINT('Ctrl Pts',(181.059201178604,586.895647046378,-48.1122153193404)) ;
#53840=CARTESIAN_POINT('Ctrl Pts',(181.015940085903,586.938571941974,-48.1083813350268)) ;
#53841=CARTESIAN_POINT('Ctrl Pts',(180.970363424739,586.979109451101,-48.1045874640204)) ;
#53842=CARTESIAN_POINT('Ctrl Pts',(180.922757128082,587.016989733627,-48.1007820160161)) ;
#53843=CARTESIAN_POINT('Ctrl Pts',(180.875060999456,587.054941495361,-48.0969693872204)) ;
#53844=CARTESIAN_POINT('Ctrl Pts',(180.825327348887,587.090225448644,-48.0931446119584)) ;
#53845=CARTESIAN_POINT('Ctrl Pts',(180.773880976884,587.122599757846,-48.0892418000498)) ;
#53846=CARTESIAN_POINT('Ctrl Pts',(180.732422092433,587.148689114434,-48.086096656444)) ;
#53847=CARTESIAN_POINT('Ctrl Pts',(180.68985163975,587.172889245008,-48.0829003731834)) ;
#53848=CARTESIAN_POINT('Ctrl Pts',(180.646358283596,587.1950919934,-48.0796162265107)) ;
#53849=CARTESIAN_POINT('Ctrl Pts',(180.646331539371,587.195105645952,-48.0796142070768)) ;
#53850=CARTESIAN_POINT('Ctrl Pts',(180.646304794796,587.19511929775,-48.0796121876096)) ;
#53851=CARTESIAN_POINT('Ctrl Pts',(180.646278049873,587.195132948793,-48.0796101681093)) ;
#53852=CARTESIAN_POINT('Ctrl Pts',(180.596932732107,587.220319600387,-48.0758841194851)) ;
#53853=CARTESIAN_POINT('Ctrl Pts',(180.546214164833,587.243022996417,-48.072035126435)) ;
#53854=CARTESIAN_POINT('Ctrl Pts',(180.494407351764,587.263127440022,-48.0681263164207)) ;
#53855=CARTESIAN_POINT('Ctrl Pts',(180.489565625201,587.265006347696,-48.067761009463)) ;
#53856=CARTESIAN_POINT('Ctrl Pts',(180.484714430368,587.266862563264,-48.0673951800475)) ;
#53857=CARTESIAN_POINT('Ctrl Pts',(180.479854022457,587.268695997693,-48.0670288797041)) ;
#53858=CARTESIAN_POINT('Ctrl Pts',(180.422276653952,587.290415230254,-48.0626896122525)) ;
#53859=CARTESIAN_POINT('Ctrl Pts',(180.363400426402,587.30893667016,-48.058284928138)) ;
#53860=CARTESIAN_POINT('Ctrl Pts',(180.303618343741,587.324152456611,-48.053886366419)) ;
#53861=CARTESIAN_POINT('Ctrl Pts',(180.244736625142,587.339139081636,-48.0495540504164)) ;
#53862=CARTESIAN_POINT('Ctrl Pts',(180.1849761475,587.350919324995,-48.0452279587262)) ;
#53863=CARTESIAN_POINT('Ctrl Pts',(180.124714023234,587.359429224381,-48.0409559399982)) ;
#53864=CARTESIAN_POINT('Ctrl Pts',(180.06448868416,587.367933929156,-48.0366865289949)) ;
#53865=CARTESIAN_POINT('Ctrl Pts',(180.003762299197,587.373172410607,-48.032471260404)) ;
#53866=CARTESIAN_POINT('Ctrl Pts',(179.942912967287,587.375116074953,-48.0283341424415)) ;
#53867=CARTESIAN_POINT('Ctrl Pts',(179.882078079596,587.377059277919,-48.0241980065348)) ;
#53868=CARTESIAN_POINT('Ctrl Pts',(179.82112032378,587.375709197426,-48.0201399873129)) ;
#53869=CARTESIAN_POINT('Ctrl Pts',(179.760419161553,587.371071815098,-48.0161593215276)) ;
#53870=CARTESIAN_POINT('Ctrl Pts',(179.698018654521,587.366304608047,-48.0120672159695)) ;
#53871=CARTESIAN_POINT('Ctrl Pts',(179.635889376445,587.358063108861,-48.0080568482458)) ;
#53872=CARTESIAN_POINT('Ctrl Pts',(179.574444647537,587.346393487565,-48.0041010454521)) ;
#53873=CARTESIAN_POINT('Ctrl Pts',(179.514595695523,587.335026937215,-48.0002479785449)) ;
#53874=CARTESIAN_POINT('Ctrl Pts',(179.455396334987,587.32040788988,-47.9964463123259)) ;
#53875=CARTESIAN_POINT('Ctrl Pts',(179.397228022023,587.302619162424,-47.9926494263338)) ;
#53876=CARTESIAN_POINT('Ctrl Pts',(179.336733261059,587.284118972879,-47.9887006834739)) ;
#53877=CARTESIAN_POINT('Ctrl Pts',(179.277354014927,587.262189665291,-47.9847566954869)) ;
#53878=CARTESIAN_POINT('Ctrl Pts',(179.219515319863,587.236976205275,-47.9807469470701)) ;
#53879=CARTESIAN_POINT('Ctrl Pts',(179.169446859135,587.215150001706,-47.9772758810146)) ;
#53880=CARTESIAN_POINT('Ctrl Pts',(179.120531903364,587.19086254644,-47.9737548797059)) ;
#53881=CARTESIAN_POINT('Ctrl Pts',(179.073042697654,587.164247054371,-47.9701331480617)) ;
#53882=CARTESIAN_POINT('Ctrl Pts',(179.06569991298,587.160131764921,-47.9695731556337)) ;
#53883=CARTESIAN_POINT('Ctrl Pts',(179.058391114115,587.155960834707,-47.9690107550085)) ;
#53884=CARTESIAN_POINT('Ctrl Pts',(179.051117196837,587.151734771194,-47.9684457584189)) ;
#53885=CARTESIAN_POINT('Ctrl Pts',(179.051090282242,587.151719134119,-47.9684436678461)) ;
#53886=CARTESIAN_POINT('Ctrl Pts',(179.051063368125,587.15170349629,-47.9684415772376)) ;
#53887=CARTESIAN_POINT('Ctrl Pts',(179.051036454486,587.151687857706,-47.9684394865936)) ;
#53888=CARTESIAN_POINT('Ctrl Pts',(179.00303414808,587.123795379465,-47.964710680897)) ;
#53889=CARTESIAN_POINT('Ctrl Pts',(178.956383143798,587.093394646366,-47.960858986221)) ;
#53890=CARTESIAN_POINT('Ctrl Pts',(178.911335735443,587.060663725994,-47.9569475109709)) ;
#53891=CARTESIAN_POINT('Ctrl Pts',(178.907128659802,587.057606914007,-47.9565822097728)) ;
#53892=CARTESIAN_POINT('Ctrl Pts',(178.902935584205,587.054529812997,-47.9562163871625)) ;
#53893=CARTESIAN_POINT('Ctrl Pts',(178.898756721833,587.051432589843,-47.9558500945468)) ;
#53894=CARTESIAN_POINT('Ctrl Pts',(178.849339627032,587.014806408698,-47.9515185049169)) ;
#53895=CARTESIAN_POINT('Ctrl Pts',(178.801907620743,586.975360863164,-47.9471218492722)) ;
#53896=CARTESIAN_POINT('Ctrl Pts',(178.756762820748,586.933367326175,-47.9427310698556)) ;
#53897=CARTESIAN_POINT('Ctrl Pts',(178.712190612804,586.891906412334,-47.9383959806935)) ;
#53898=CARTESIAN_POINT('Ctrl Pts',(178.669847599266,586.847961977422,-47.9340669120912)) ;
#53899=CARTESIAN_POINT('Ctrl Pts',(178.629992517954,586.801817601538,-47.9297915887904)) ;
#53900=CARTESIAN_POINT('Ctrl Pts',(178.590161679204,586.755701293791,-47.925518866031)) ;
#53901=CARTESIAN_POINT('Ctrl Pts',(178.552815628851,586.707387777744,-47.9212999582049)) ;
#53902=CARTESIAN_POINT('Ctrl Pts',(178.518183896022,586.657180564922,-47.9171586830542)) ;
#53903=CARTESIAN_POINT('Ctrl Pts',(178.483560447977,586.60698536293,-47.9130183986009)) ;
#53904=CARTESIAN_POINT('Ctrl Pts',(178.451650054233,586.554897366349,-47.9089557114525)) ;
#53905=CARTESIAN_POINT('Ctrl Pts',(178.422653937972,586.501239960583,-47.9049696146823)) ;
#53906=CARTESIAN_POINT('Ctrl Pts',(178.392970250437,586.446310201979,-47.9008889974732)) ;
#53907=CARTESIAN_POINT('Ctrl Pts',(178.366340998771,586.389735597203,-47.8968886187649)) ;
#53908=CARTESIAN_POINT('Ctrl Pts',(178.342949811355,586.331885246925,-47.8929414084268)) ;
#53909=CARTESIAN_POINT('Ctrl Pts',(178.320071526454,586.275303391047,-47.8890807492364)) ;
#53910=CARTESIAN_POINT('Ctrl Pts',(178.300291065518,586.217501151216,-47.8852705986862)) ;
#53911=CARTESIAN_POINT('Ctrl Pts',(178.283746301024,586.158845320057,-47.8814641815396)) ;
#53912=CARTESIAN_POINT('Ctrl Pts',(178.266645167158,586.098217003404,-47.8775297617297)) ;
#53913=CARTESIAN_POINT('Ctrl Pts',(178.253001833031,586.036676586433,-47.8735989005534)) ;
#53914=CARTESIAN_POINT('Ctrl Pts',(178.242923733702,585.974653496531,-47.869602331551)) ;
#53915=CARTESIAN_POINT('Ctrl Pts',(178.234152338515,585.920672183732,-47.8661239488747)) ;
#53916=CARTESIAN_POINT('Ctrl Pts',(178.228081320139,585.866324389926,-47.8625951437717)) ;
#53917=CARTESIAN_POINT('Ctrl Pts',(178.224746826461,585.811911451861,-47.8589653240946)) ;
#53918=CARTESIAN_POINT('Ctrl Pts',(178.224252145035,585.803839140932,-47.8584268302347)) ;
#53919=CARTESIAN_POINT('Ctrl Pts',(178.22381762761,585.795765326998,-47.8578861131905)) ;
#53920=CARTESIAN_POINT('Ctrl Pts',(178.223443328293,585.787690919578,-47.8573430077773)) ;
#53921=CARTESIAN_POINT('Ctrl Pts',(178.223441762582,585.787657143973,-47.8573407359433)) ;
#53922=CARTESIAN_POINT('Ctrl Pts',(178.223440197925,585.787623368358,-47.8573384640674)) ;
#53923=CARTESIAN_POINT('Ctrl Pts',(178.223438634321,585.787589592732,-47.8573361921497)) ;
#53924=CARTESIAN_POINT('Ctrl Pts',(178.220870330784,585.732111292547,-47.8536044439544)) ;
#53925=CARTESIAN_POINT('Ctrl Pts',(178.221143922289,585.67640822179,-47.8497502705975)) ;
#53926=CARTESIAN_POINT('Ctrl Pts',(178.224246539444,585.620789796714,-47.8458371466104)) ;
#53927=CARTESIAN_POINT('Ctrl Pts',(178.224528728945,585.615731184964,-47.8454812398231)) ;
#53928=CARTESIAN_POINT('Ctrl Pts',(178.224834300041,585.610673302273,-47.8451248453797)) ;
#53929=CARTESIAN_POINT('Ctrl Pts',(178.22516323011,585.605616398388,-47.844768011037)) ;
#53930=CARTESIAN_POINT('Ctrl Pts',(178.229157110935,585.544215288006,-47.840435315506)) ;
#53931=CARTESIAN_POINT('Ctrl Pts',(178.236597951157,585.482953409495,-47.836038428256)) ;
#53932=CARTESIAN_POINT('Ctrl Pts',(178.247421429552,585.42223285034,-47.831648368672)) ;
#53933=CARTESIAN_POINT('Ctrl Pts',(178.258085000805,585.362409382739,-47.827323168263)) ;
#53934=CARTESIAN_POINT('Ctrl Pts',(178.272031588538,585.303111185833,-47.8230048746017)) ;
#53935=CARTESIAN_POINT('Ctrl Pts',(178.289163535409,585.244708151981,-47.8187406547706)) ;
#53936=CARTESIAN_POINT('Ctrl Pts',(178.30628553143,585.186339040709,-47.8144789117515)) ;
#53937=CARTESIAN_POINT('Ctrl Pts',(178.326589078513,585.128863989302,-47.8102713110671)) ;
#53938=CARTESIAN_POINT('Ctrl Pts',(178.349943937351,585.072639270109,-47.8061410125672)) ;
#53939=CARTESIAN_POINT('Ctrl Pts',(178.373293946666,585.016426225706,-47.8020115717039)) ;
#53940=CARTESIAN_POINT('Ctrl Pts',(178.39969402403,584.961463025718,-47.7979594006895)) ;
#53941=CARTESIAN_POINT('Ctrl Pts',(178.428981849489,584.908092986886,-47.7939827726763)) ;
#53942=CARTESIAN_POINT('Ctrl Pts',(178.459072004302,584.8532608952,-47.7898972063812)) ;
#53943=CARTESIAN_POINT('Ctrl Pts',(178.492210590527,584.800110655127,-47.7858913648375)) ;
#53944=CARTESIAN_POINT('Ctrl Pts',(178.528184980514,584.748999271006,-47.7819370164778)) ;
#53945=CARTESIAN_POINT('Ctrl Pts',(178.563248122558,584.699182561892,-47.7780828335916)) ;
#53946=CARTESIAN_POINT('Ctrl Pts',(178.601005291661,584.651302907566,-47.7742771976262)) ;
#53947=CARTESIAN_POINT('Ctrl Pts',(178.641223069236,584.605673871915,-47.7704724715031)) ;
#53948=CARTESIAN_POINT('Ctrl Pts',(178.683008662682,584.558266072479,-47.7665194251506)) ;
#53949=CARTESIAN_POINT('Ctrl Pts',(178.72745105857,584.513288439922,-47.7625669319197)) ;
#53950=CARTESIAN_POINT('Ctrl Pts',(178.774242759903,584.471067628475,-47.7585436949899)) ;
#53951=CARTESIAN_POINT('Ctrl Pts',(178.81463325317,584.434622717263,-47.7550708457559)) ;
#53952=CARTESIAN_POINT('Ctrl Pts',(178.856774835547,584.400231167256,-47.7515446221092)) ;
#53953=CARTESIAN_POINT('Ctrl Pts',(178.900435603904,584.368083976891,-47.7479144055063)) ;
#53954=CARTESIAN_POINT('Ctrl Pts',(178.907326412993,584.36301031099,-47.747341462553)) ;
#53955=CARTESIAN_POINT('Ctrl Pts',(178.914255090497,584.357992447896,-47.7467659292308)) ;
#53956=CARTESIAN_POINT('Ctrl Pts',(178.921220758242,584.353031024268,-47.746187606543)) ;
#53957=CARTESIAN_POINT('Ctrl Pts',(178.921249751937,584.353010372981,-47.7461851993493)) ;
#53958=CARTESIAN_POINT('Ctrl Pts',(178.921278746273,584.352989722672,-47.7461827921072)) ;
#53959=CARTESIAN_POINT('Ctrl Pts',(178.92130774125,584.35296907334,-47.7461803848168)) ;
#53960=CARTESIAN_POINT('Ctrl Pts',(178.96609389121,584.321073753566,-47.7424620418301)) ;
#53961=CARTESIAN_POINT('Ctrl Pts',(179.012582022572,584.291398545953,-47.7386180925322)) ;
#53962=CARTESIAN_POINT('Ctrl Pts',(179.060512232693,584.264098009022,-47.7347113417059)) ;
#53963=CARTESIAN_POINT('Ctrl Pts',(179.065190679357,584.261433215657,-47.7343300054813)) ;
#53964=CARTESIAN_POINT('Ctrl Pts',(179.069882824745,584.258791044184,-47.7339480709073)) ;
#53965=CARTESIAN_POINT('Ctrl Pts',(179.074588400769,584.256171635694,-47.7335655963915)) ;
#53966=CARTESIAN_POINT('Ctrl Pts',(179.128346800044,584.22624645613,-47.7291960531883)) ;
#53967=CARTESIAN_POINT('Ctrl Pts',(179.183864273609,584.199292316861,-47.7247567343599)) ;
#53968=CARTESIAN_POINT('Ctrl Pts',(179.240766466883,584.175474967899,-47.7203209274937)) ;
#53969=CARTESIAN_POINT('Ctrl Pts',(179.296614645206,584.152098794232,-47.7159672862961)) ;
#53970=CARTESIAN_POINT('Ctrl Pts',(179.353796625881,584.131743807501,-47.7116173127172)) ;
#53971=CARTESIAN_POINT('Ctrl Pts',(179.411951071135,584.114528036147,-47.7073200655742)) ;
#53972=CARTESIAN_POINT('Ctrl Pts',(179.470068534857,584.097323212633,-47.7030255511334)) ;
#53973=CARTESIAN_POINT('Ctrl Pts',(179.529157213191,584.083253479214,-47.6987838388947)) ;
#53974=CARTESIAN_POINT('Ctrl Pts',(179.588849648619,584.072401912726,-47.6946203248817)) ;
#53975=CARTESIAN_POINT('Ctrl Pts',(179.6485268056,584.061553123726,-47.6904578765318)) ;
#53976=CARTESIAN_POINT('Ctrl Pts',(179.708807388094,584.053920881524,-47.6863735970115)) ;
#53977=CARTESIAN_POINT('Ctrl Pts',(179.76931765361,584.049554231932,-47.6823681831685)) ;
#53978=CARTESIAN_POINT('Ctrl Pts',(179.831905341739,584.045037667669,-47.6782252565047)) ;
#53979=CARTESIAN_POINT('Ctrl Pts',(179.894738737398,584.044015170651,-47.6741667339541)) ;
#53980=CARTESIAN_POINT('Ctrl Pts',(179.95739747218,584.04650117541,-47.6701664126541)) ;
#53981=CARTESIAN_POINT('Ctrl Pts',(180.018055012907,584.048907782172,-47.6662938535765)) ;
#53982=CARTESIAN_POINT('Ctrl Pts',(180.078548744618,584.054602451444,-47.6624754582192)) ;
#53983=CARTESIAN_POINT('Ctrl Pts',(180.138492202174,584.063558629316,-47.6586656558443)) ;
#53984=CARTESIAN_POINT('Ctrl Pts',(180.20140211261,584.072958026194,-47.6546673158092)) ;
#53985=CARTESIAN_POINT('Ctrl Pts',(180.263705718314,584.085950672778,-47.6506780644461)) ;
#53986=CARTESIAN_POINT('Ctrl Pts',(180.324952967773,584.10245292891,-47.6466260430931)) ;
#53987=CARTESIAN_POINT('Ctrl Pts',(180.377763463543,584.116682014059,-47.6431321840478)) ;
#53988=CARTESIAN_POINT('Ctrl Pts',(180.429789581885,584.13352052268,-47.6395909946578)) ;
#53989=CARTESIAN_POINT('Ctrl Pts',(180.480740563972,584.15287508289,-47.635950694698)) ;
#53990=CARTESIAN_POINT('Ctrl Pts',(180.488863080554,584.155960553077,-47.6353703644359)) ;
#53991=CARTESIAN_POINT('Ctrl Pts',(180.496958376483,584.15910993538,-47.63478751536)) ;
#53992=CARTESIAN_POINT('Ctrl Pts',(180.505025392259,584.162322819237,-47.6342019376836)) ;
#53993=CARTESIAN_POINT('Ctrl Pts',(180.505042444981,584.162329610895,-47.6342006998413)) ;
#53994=CARTESIAN_POINT('Ctrl Pts',(180.505059497576,584.162336402837,-47.6341994619868)) ;
#53995=CARTESIAN_POINT('Ctrl Pts',(180.505076550046,584.162343195063,-47.6341982241201)) ;
#53996=CARTESIAN_POINT('Ctrl Pts',(180.557298536641,584.183143908574,-47.630407344555)) ;
#53997=CARTESIAN_POINT('Ctrl Pts',(180.608515361297,584.206686092502,-47.6264922198568)) ;
#53998=CARTESIAN_POINT('Ctrl Pts',(180.65844762838,584.232826843712,-47.6225152161776)) ;
#53999=CARTESIAN_POINT('Ctrl Pts',(180.663457052748,584.2354493987,-47.622116225699)) ;
#54000=CARTESIAN_POINT('Ctrl Pts',(180.668453527044,584.238098070403,-47.6217166124095)) ;
#54001=CARTESIAN_POINT('Ctrl Pts',(180.673436755783,584.240772688929,-47.621316439284)) ;
#54002=CARTESIAN_POINT('Ctrl Pts',(180.727975537573,584.270044962764,-47.6169367577736)) ;
#54003=CARTESIAN_POINT('Ctrl Pts',(180.780931118968,584.302430144093,-47.6124906531587)) ;
#54004=CARTESIAN_POINT('Ctrl Pts',(180.831965618059,584.33770377131,-47.6080472780278)) ;
#54005=CARTESIAN_POINT('Ctrl Pts',(180.882937031464,584.372933795454,-47.6036093955221)) ;
#54006=CARTESIAN_POINT('Ctrl Pts',(180.931992413172,584.411044902159,-47.5991745754653)) ;
#54007=CARTESIAN_POINT('Ctrl Pts',(180.978823392945,584.451786978966,-47.5947911249208)) ;
#54008=CARTESIAN_POINT('Ctrl Pts',(181.025611228522,584.49249152113,-47.5904117127383)) ;
#54009=CARTESIAN_POINT('Ctrl Pts',(181.070178898671,584.535822145435,-47.586083711498)) ;
#54010=CARTESIAN_POINT('Ctrl Pts',(181.112243766078,584.581504876635,-47.5818312442298)) ;
#54011=CARTESIAN_POINT('Ctrl Pts',(181.154283113265,584.627159892704,-47.5775813568792)) ;
#54012=CARTESIAN_POINT('Ctrl Pts',(181.193822672174,584.675164214726,-47.5734069046344)) ;
#54013=CARTESIAN_POINT('Ctrl Pts',(181.230604314454,584.725219699878,-47.5693070038503)) ;
#54014=CARTESIAN_POINT('Ctrl Pts',(181.267389569821,584.775280102016,-47.5652067003299)) ;
#54015=CARTESIAN_POINT('Ctrl Pts',(181.301416192259,584.827392180787,-47.5611808285123)) ;
#54016=CARTESIAN_POINT('Ctrl Pts',(181.332451455274,584.881231780506,-47.5572045791497)) ;
#54017=CARTESIAN_POINT('Ctrl Pts',(181.363485675684,584.935069571525,-47.5532284633661)) ;
#54018=CARTESIAN_POINT('Ctrl Pts',(181.391528392631,584.990634905946,-47.5493016741465)) ;
#54019=CARTESIAN_POINT('Ctrl Pts',(181.416376235186,585.047575835669,-47.5453786416672)) ;
#54020=CARTESIAN_POINT('Ctrl Pts',(181.441249031598,585.104573949262,-47.5414516694177)) ;
#54021=CARTESIAN_POINT('Ctrl Pts',(181.46291995929,585.162950524743,-47.5375279573556)) ;
#54022=CARTESIAN_POINT('Ctrl Pts',(181.481221277255,585.222322749231,-47.5335469067959)) ;
#54023=CARTESIAN_POINT('Ctrl Pts',(181.498352981961,585.277900572617,-47.5298202799631)) ;
#54024=CARTESIAN_POINT('Ctrl Pts',(181.512531780721,585.334350496989,-47.526042753317)) ;
#54025=CARTESIAN_POINT('Ctrl Pts',(181.523656952667,585.391334705907,-47.52216017176)) ;
#54026=CARTESIAN_POINT('Origin',(179.888527625416,585.710565160536,-47.5221601717598)) ;
#54027=CARTESIAN_POINT('Ctrl Pts',(181.45195815042,586.286100557784,-48.3557104975402)) ;
#54028=CARTESIAN_POINT('Ctrl Pts',(181.443430929173,586.309264585671,-48.3540690235658)) ;
#54029=CARTESIAN_POINT('Ctrl Pts',(181.434389273589,586.332238109432,-48.3524103290642)) ;
#54030=CARTESIAN_POINT('Ctrl Pts',(181.397454926864,586.420287834188,-48.345927431339)) ;
#54031=CARTESIAN_POINT('Ctrl Pts',(181.365940902444,586.483750384691,-48.3409809049559)) ;
#54032=CARTESIAN_POINT('Ctrl Pts',(181.277531964931,586.636525632691,-48.3283801251284)) ;
#54033=CARTESIAN_POINT('Ctrl Pts',(181.215982329991,586.722789005932,-48.3206115127961)) ;
#54034=CARTESIAN_POINT('Ctrl Pts',(181.110335328957,586.844503617117,-48.3089652506152)) ;
#54035=CARTESIAN_POINT('Ctrl Pts',(181.071917277504,586.884541604414,-48.3050053477068)) ;
#54036=CARTESIAN_POINT('Ctrl Pts',(181.009695297284,586.943222104851,-48.2990864909969)) ;
#54037=CARTESIAN_POINT('Ctrl Pts',(180.987264284814,586.963257618225,-48.2970444731123)) ;
#54038=CARTESIAN_POINT('Ctrl Pts',(180.931510621498,587.010406023872,-48.2921983726469)) ;
#54039=CARTESIAN_POINT('Ctrl Pts',(180.897659925384,587.036857955258,-48.2894364566215)) ;
#54040=CARTESIAN_POINT('Ctrl Pts',(180.812339532822,587.098369378618,-48.2827988334593)) ;
#54041=CARTESIAN_POINT('Ctrl Pts',(180.759854627338,587.131909335231,-48.2789842951599)) ;
#54042=CARTESIAN_POINT('Ctrl Pts',(180.601584244595,587.220980929433,-48.267887808215)) ;
#54043=CARTESIAN_POINT('Ctrl Pts',(180.491576631445,587.268170331297,-48.2606445675556)) ;
#54044=CARTESIAN_POINT('Ctrl Pts',(180.32808376122,587.318363642565,-48.2496730936678)) ;
#54045=CARTESIAN_POINT('Ctrl Pts',(180.278017792087,587.331219964738,-48.2462922002711)) ;
#54046=CARTESIAN_POINT('Ctrl Pts',(180.171182203686,587.353417532433,-48.2389847729666)) ;
#54047=CARTESIAN_POINT('Ctrl Pts',(180.114364578511,587.36218672341,-48.2350441793587)) ;
#54048=CARTESIAN_POINT('Ctrl Pts',(179.989944623202,587.374849547511,-48.2262802710685)) ;
#54049=CARTESIAN_POINT('Ctrl Pts',(179.922328375845,587.377593582707,-48.2214312160094)) ;
#54050=CARTESIAN_POINT('Ctrl Pts',(179.738188563359,587.373858183083,-48.2080771569703)) ;
#54051=CARTESIAN_POINT('Ctrl Pts',(179.622203633226,587.359267687013,-48.1994865815561)) ;
#54052=CARTESIAN_POINT('Ctrl Pts',(179.477866907529,587.325469419362,-48.1891498383575)) ;
#54053=CARTESIAN_POINT('Ctrl Pts',(179.447253870925,587.317374450272,-48.18698070924)) ;
#54054=CARTESIAN_POINT('Ctrl Pts',(179.381056318005,587.297834644963,-48.1823655551405)) ;
#54055=CARTESIAN_POINT('Ctrl Pts',(179.345589773519,587.286055749152,-48.1799373293568)) ;
#54056=CARTESIAN_POINT('Ctrl Pts',(179.210439791717,587.236063539404,-48.1707485761946)) ;
#54057=CARTESIAN_POINT('Ctrl Pts',(179.114113944203,587.189496009491,-48.1643247946066)) ;
#54058=CARTESIAN_POINT('Ctrl Pts',(178.945287781856,587.086830253905,-48.1522345871993)) ;
#54059=CARTESIAN_POINT('Ctrl Pts',(178.871675679258,587.033371361065,-48.1466188642367)) ;
#54060=CARTESIAN_POINT('Ctrl Pts',(178.764200119052,586.941025428722,-48.1374925328631)) ;
#54061=CARTESIAN_POINT('Ctrl Pts',(178.727151903909,586.906119552598,-48.1341496452756)) ;
#54062=CARTESIAN_POINT('Ctrl Pts',(178.650052876733,586.8265090294,-48.1267011960654)) ;
#54063=CARTESIAN_POINT('Ctrl Pts',(178.610704495145,586.781227050279,-48.1225708510962)) ;
#54064=CARTESIAN_POINT('Ctrl Pts',(178.52867310389,586.675847107055,-48.1131695099987)) ;
#54065=CARTESIAN_POINT('Ctrl Pts',(178.487363830371,586.614839249772,-48.1078615898132)) ;
#54066=CARTESIAN_POINT('Ctrl Pts',(178.397180446647,586.460557692113,-48.0948693689265)) ;
#54067=CARTESIAN_POINT('Ctrl Pts',(178.35283812052,586.364985797675,-48.0871615625068)) ;
#54068=CARTESIAN_POINT('Ctrl Pts',(178.307384305074,586.236414576012,-48.0776679428554)) ;
#54069=CARTESIAN_POINT('Ctrl Pts',(178.297801180886,586.206671821016,-48.0755312737752)) ;
#54070=CARTESIAN_POINT('Ctrl Pts',(178.278327936602,586.139848362584,-48.0708844293593)) ;
#54071=CARTESIAN_POINT('Ctrl Pts',(178.268870864757,586.102661679427,-48.0683965412314)) ;
#54072=CARTESIAN_POINT('Ctrl Pts',(178.249791116583,586.015077597982,-48.0626926234597)) ;
#54073=CARTESIAN_POINT('Ctrl Pts',(178.241194965258,585.964496304437,-48.0595161829983)) ;
#54074=CARTESIAN_POINT('Ctrl Pts',(178.217846403679,585.774334032729,-48.0477528209275)) ;
#54075=CARTESIAN_POINT('Ctrl Pts',(178.218408472952,585.633483604313,-48.0393417606924)) ;
#54076=CARTESIAN_POINT('Ctrl Pts',(178.243298194302,585.443303573488,-48.0270283038372)) ;
#54077=CARTESIAN_POINT('Ctrl Pts',(178.25234552833,585.39257802682,-48.0236555769129)) ;
#54078=CARTESIAN_POINT('Ctrl Pts',(178.27653108666,585.285853806666,-48.0163223463825)) ;
#54079=CARTESIAN_POINT('Ctrl Pts',(178.292272752844,585.230063844592,-48.0123457209125)) ;
#54080=CARTESIAN_POINT('Ctrl Pts',(178.332972339751,585.11012542569,-48.0034627637028)) ;
#54081=CARTESIAN_POINT('Ctrl Pts',(178.359063209572,585.04647405495,-47.9985287102257)) ;
#54082=CARTESIAN_POINT('Ctrl Pts',(178.438165562215,584.883079041712,-47.9853597944614)) ;
#54083=CARTESIAN_POINT('Ctrl Pts',(178.49751302551,584.786787754627,-47.9770572571765)) ;
#54084=CARTESIAN_POINT('Ctrl Pts',(178.585636793927,584.671787558228,-47.9669433352678)) ;
#54085=CARTESIAN_POINT('Ctrl Pts',(178.60586613944,584.646909407949,-47.9647440450321)) ;
#54086=CARTESIAN_POINT('Ctrl Pts',(178.650819919919,584.594774802032,-47.9601361288877)) ;
#54087=CARTESIAN_POINT('Ctrl Pts',(178.675753748137,584.567722847513,-47.9577422910839)) ;
#54088=CARTESIAN_POINT('Ctrl Pts',(178.775363414293,584.466586868774,-47.948677389504)) ;
#54089=CARTESIAN_POINT('Ctrl Pts',(178.856098426246,584.398806394709,-47.9423384820082)) ;
#54090=CARTESIAN_POINT('Ctrl Pts',(179.019328137633,584.286235711831,-47.9302098459965)) ;
#54091=CARTESIAN_POINT('Ctrl Pts',(179.100248499142,584.239907095803,-47.9244616565643)) ;
#54092=CARTESIAN_POINT('Ctrl Pts',(179.230280230815,584.179289344805,-47.9152224617741)) ;
#54093=CARTESIAN_POINT('Ctrl Pts',(179.276890068618,584.160083351187,-47.9119128022261)) ;
#54094=CARTESIAN_POINT('Ctrl Pts',(179.380237467402,584.122883771237,-47.9045345558958)) ;
#54095=CARTESIAN_POINT('Ctrl Pts',(179.437211136613,584.105758956359,-47.9004413492104)) ;
#54096=CARTESIAN_POINT('Ctrl Pts',(179.565291435026,584.074621578854,-47.8911684355796)) ;
#54097=CARTESIAN_POINT('Ctrl Pts',(179.636642999256,584.062127938558,-47.8859541562891)) ;
#54098=CARTESIAN_POINT('Ctrl Pts',(179.816715850088,584.042562822711,-47.872787640558)) ;
#54099=CARTESIAN_POINT('Ctrl Pts',(179.925756002662,584.041431750277,-47.8647990115143)) ;
#54100=CARTESIAN_POINT('Ctrl Pts',(180.065006146868,584.05364882853,-47.8550745457781)) ;
#54101=CARTESIAN_POINT('Ctrl Pts',(180.095800522561,584.057218562334,-47.8529566337892)) ;
#54102=CARTESIAN_POINT('Ctrl Pts',(180.164859570561,584.067184474833,-47.8483016225688)) ;
#54103=CARTESIAN_POINT('Ctrl Pts',(180.203034951374,584.074061211128,-47.8457889588977)) ;
#54104=CARTESIAN_POINT('Ctrl Pts',(180.292004002471,584.093316704981,-47.8400020901898)) ;
#54105=CARTESIAN_POINT('Ctrl Pts',(180.342524364516,584.1067654574,-47.8367693177729)) ;
#54106=CARTESIAN_POINT('Ctrl Pts',(180.522820007814,584.163965650768,-47.8251640115305)) ;
#54107=CARTESIAN_POINT('Ctrl Pts',(180.647695520257,584.221284055813,-47.8169463585962)) ;
#54108=CARTESIAN_POINT('Ctrl Pts',(180.807896397878,584.320255449165,-47.8048675471421)) ;
#54109=CARTESIAN_POINT('Ctrl Pts',(180.850362479379,584.349288999803,-47.8015033227905)) ;
#54110=CARTESIAN_POINT('Ctrl Pts',(180.936829035483,584.414473067217,-47.7942525957142)) ;
#54111=CARTESIAN_POINT('Ctrl Pts',(180.980454847296,584.451008046381,-47.7903530580458)) ;
#54112=CARTESIAN_POINT('Ctrl Pts',(181.070826200184,584.534919374387,-47.7817126029434)) ;
#54113=CARTESIAN_POINT('Ctrl Pts',(181.116774516141,584.583009897295,-47.7769475388171)) ;
#54114=CARTESIAN_POINT('Ctrl Pts',(181.238074762311,584.72620151044,-47.7633355204528)) ;
#54115=CARTESIAN_POINT('Ctrl Pts',(181.306100073429,584.826969848809,-47.7543788991492)) ;
#54116=CARTESIAN_POINT('Ctrl Pts',(181.377146484779,584.961869234682,-47.7437545121612)) ;
#54117=CARTESIAN_POINT('Ctrl Pts',(181.390923965474,584.989914359271,-47.7416162949122)) ;
#54118=CARTESIAN_POINT('Ctrl Pts',(181.420005657885,585.053577939834,-47.7369392242399)) ;
#54119=CARTESIAN_POINT('Ctrl Pts',(181.434871689442,585.089374517483,-47.7344235946812)) ;
#54120=CARTESIAN_POINT('Ctrl Pts',(181.466728698429,585.174337636028,-47.7286427827358)) ;
#54121=CARTESIAN_POINT('Ctrl Pts',(181.482693166675,585.223845970174,-47.7254179100826)) ;
#54122=CARTESIAN_POINT('Ctrl Pts',(181.532240432319,585.406329071536,-47.7137859949888)) ;
#54123=CARTESIAN_POINT('Ctrl Pts',(181.551693191161,585.542550455988,-47.7055347715064)) ;
#54124=CARTESIAN_POINT('Ctrl Pts',(181.555202721283,585.731418582942,-47.6933935229849)) ;
#54125=CARTESIAN_POINT('Ctrl Pts',(181.553747970288,585.783235432592,-47.6899969891168)) ;
#54126=CARTESIAN_POINT('Ctrl Pts',(181.545521981611,585.893154069984,-47.6826029385961)) ;
#54127=CARTESIAN_POINT('Ctrl Pts',(181.538101371667,585.951135292317,-47.6785887999446)) ;
#54128=CARTESIAN_POINT('Ctrl Pts',(181.510468967264,586.103106613832,-47.667743150632)) ;
#54129=CARTESIAN_POINT('Ctrl Pts',(181.485146513092,586.195937380314,-47.6607736436916)) ;
#54130=CARTESIAN_POINT('Ctrl Pts',(181.451973977593,586.286057561759,-47.6537754297552)) ;
#54131=CARTESIAN_POINT('Origin',(179.888527625416,585.710565160536,-48.5221601717598)) ;
#54132=CARTESIAN_POINT('',(181.451958155526,586.286100543914,-49.0537403040459)) ;
#54133=CARTESIAN_POINT('',(181.451958155603,586.286100543705,-48.8631342200737)) ;
#54134=CARTESIAN_POINT('',(181.451958155526,586.286100543914,-48.5221601717599)) ;
#54135=CARTESIAN_POINT('',(181.555012477675,585.711613030546,-49.0927992681987)) ;
#54136=CARTESIAN_POINT('Ctrl Pts',(181.55452730859,585.71159261619,-49.0925209293698)) ;
#54137=CARTESIAN_POINT('Ctrl Pts',(181.554499034075,585.757439200686,-49.0892076633268)) ;
#54138=CARTESIAN_POINT('Ctrl Pts',(181.552578285604,585.80326867997,-49.0859220267552)) ;
#54139=CARTESIAN_POINT('Ctrl Pts',(181.546213055913,585.879626570088,-49.0805462416942)) ;
#54140=CARTESIAN_POINT('Ctrl Pts',(181.542807775801,585.910215500907,-49.0784194957207)) ;
#54141=CARTESIAN_POINT('Ctrl Pts',(181.534158770185,585.972228788091,-49.0741854936695)) ;
#54142=CARTESIAN_POINT('Ctrl Pts',(181.528857649455,586.003630462584,-49.0720857688122)) ;
#54143=CARTESIAN_POINT('Ctrl Pts',(181.50569208945,586.120361536234,-49.0643871935001)) ;
#54144=CARTESIAN_POINT('Ctrl Pts',(181.482047253509,586.204364102039,-49.0590539986409)) ;
#54145=CARTESIAN_POINT('Ctrl Pts',(181.451958155526,586.286100543914,-49.0537403040458)) ;
#54146=CARTESIAN_POINT('',(178.619456745563,586.789923813584,-49.5221601717597)) ;
#54147=CARTESIAN_POINT('Ctrl Pts',(181.555012477675,585.711613030547,-49.0927992681987)) ;
#54148=CARTESIAN_POINT('Ctrl Pts',(181.554916975438,585.651747730793,-49.0970476791215)) ;
#54149=CARTESIAN_POINT('Ctrl Pts',(181.55156888472,585.591782420422,-49.1013352669896)) ;
#54150=CARTESIAN_POINT('Ctrl Pts',(181.544993104438,585.532094412162,-49.1056020815615)) ;
#54151=CARTESIAN_POINT('Ctrl Pts',(181.538424435453,585.472470952776,-49.1098642818385)) ;
#54152=CARTESIAN_POINT('Ctrl Pts',(181.528635291814,585.413124159944,-49.1141054952774)) ;
#54153=CARTESIAN_POINT('Ctrl Pts',(181.51568743049,585.354421552545,-49.1182862646058)) ;
#54154=CARTESIAN_POINT('Ctrl Pts',(181.502748495606,585.295759415561,-49.1224641516522)) ;
#54155=CARTESIAN_POINT('Ctrl Pts',(181.486655266837,585.23774059531,-49.1265815797148)) ;
#54156=CARTESIAN_POINT('Ctrl Pts',(181.467504049314,585.180723452478,-49.1306220736233)) ;
#54157=CARTESIAN_POINT('Ctrl Pts',(181.448358461983,585.123723071894,-49.1346613796828)) ;
#54158=CARTESIAN_POINT('Ctrl Pts',(181.426156640988,585.067723872839,-49.1386238192241)) ;
#54159=CARTESIAN_POINT('Ctrl Pts',(181.401029308306,585.01307466407,-49.1425163763437)) ;
#54160=CARTESIAN_POINT('Ctrl Pts',(181.37588165729,584.95838126514,-49.1464120810427)) ;
#54161=CARTESIAN_POINT('Ctrl Pts',(181.347803621948,584.905040214261,-49.1502379281539)) ;
#54162=CARTESIAN_POINT('Ctrl Pts',(181.316962186217,584.853389923659,-49.1540232238451)) ;
#54163=CARTESIAN_POINT('Ctrl Pts',(181.286109214421,584.801720313557,-49.1578099354048)) ;
#54164=CARTESIAN_POINT('Ctrl Pts',(181.252490551254,584.751743010917,-49.1615563552486)) ;
#54165=CARTESIAN_POINT('Ctrl Pts',(181.216312051274,584.703782191105,-49.1653109644898)) ;
#54166=CARTESIAN_POINT('Ctrl Pts',(181.180066428381,584.655732388335,-49.1690725397553)) ;
#54167=CARTESIAN_POINT('Ctrl Pts',(181.14125117188,584.609707030218,-49.1728428254195)) ;
#54168=CARTESIAN_POINT('Ctrl Pts',(181.100116031628,584.566011852995,-49.1766839806197)) ;
#54169=CARTESIAN_POINT('Ctrl Pts',(181.064117916884,584.527773403004,-49.1800454458973)) ;
#54170=CARTESIAN_POINT('Ctrl Pts',(181.026343714903,584.491319509308,-49.1834617127504)) ;
#54171=CARTESIAN_POINT('Ctrl Pts',(180.986990038803,584.456836965442,-49.1869773558899)) ;
#54172=CARTESIAN_POINT('Ctrl Pts',(180.986964608508,584.456814682867,-49.1869796276939)) ;
#54173=CARTESIAN_POINT('Ctrl Pts',(180.986939177554,584.456792401114,-49.1869818995395)) ;
#54174=CARTESIAN_POINT('Ctrl Pts',(180.98691374594,584.456770120182,-49.1869841714265)) ;
#54175=CARTESIAN_POINT('Ctrl Pts',(180.945140375073,584.420171985243,-49.1907159196502)) ;
#54176=CARTESIAN_POINT('Ctrl Pts',(180.901419378894,584.385655591161,-49.1945700929975)) ;
#54177=CARTESIAN_POINT('Ctrl Pts',(180.856000692707,584.35340379413,-49.1984832169383)) ;
#54178=CARTESIAN_POINT('Ctrl Pts',(180.851869769652,584.350470426763,-49.1988391236204)) ;
#54179=CARTESIAN_POINT('Ctrl Pts',(180.84772483842,584.347555794413,-49.199195517958)) ;
#54180=CARTESIAN_POINT('Ctrl Pts',(180.843566108376,584.34466003511,-49.1995523521944)) ;
#54181=CARTESIAN_POINT('Ctrl Pts',(180.793070642185,584.309499610057,-49.2038850477349)) ;
#54182=CARTESIAN_POINT('Ctrl Pts',(180.740534887717,584.277120936133,-49.2082819349534)) ;
#54183=CARTESIAN_POINT('Ctrl Pts',(180.686313313283,584.247724422448,-49.2126719944644)) ;
#54184=CARTESIAN_POINT('Ctrl Pts',(180.632892815892,584.218762216924,-49.2169971946287)) ;
#54185=CARTESIAN_POINT('Ctrl Pts',(180.577836064427,584.192694277852,-49.2213154880044)) ;
#54186=CARTESIAN_POINT('Ctrl Pts',(180.521493140722,584.169674877758,-49.2255797075153)) ;
#54187=CARTESIAN_POINT('Ctrl Pts',(180.465182943006,584.146668848155,-49.2298414502147)) ;
#54188=CARTESIAN_POINT('Ctrl Pts',(180.407588084837,584.126707692432,-49.2340490505442)) ;
#54189=CARTESIAN_POINT('Ctrl Pts',(180.349068314023,584.109911717571,-49.238179348656)) ;
#54190=CARTESIAN_POINT('Ctrl Pts',(180.290560694548,584.093119230311,-49.2423087891319)) ;
#54191=CARTESIAN_POINT('Ctrl Pts',(180.231128556488,584.079490647407,-49.2463609597265)) ;
#54192=CARTESIAN_POINT('Ctrl Pts',(180.171141520504,584.069113116492,-49.2503375872865)) ;
#54193=CARTESIAN_POINT('Ctrl Pts',(180.10951115719,584.05845129615,-49.2544231533971)) ;
#54194=CARTESIAN_POINT('Ctrl Pts',(180.047295052453,584.051221453135,-49.2584289947099)) ;
#54195=CARTESIAN_POINT('Ctrl Pts',(179.984904894767,584.047479937027,-49.2623833427958)) ;
#54196=CARTESIAN_POINT('Ctrl Pts',(179.924095112789,584.043833195502,-49.2662375251522)) ;
#54197=CARTESIAN_POINT('Ctrl Pts',(179.863120082857,584.043500462936,-49.2700431605542)) ;
#54198=CARTESIAN_POINT('Ctrl Pts',(179.802370493183,584.046494749208,-49.2738478860765)) ;
#54199=CARTESIAN_POINT('Ctrl Pts',(179.739252686439,584.049605762521,-49.2778009322042)) ;
#54200=CARTESIAN_POINT('Ctrl Pts',(179.676378371499,584.056309132488,-49.2817534251688)) ;
#54201=CARTESIAN_POINT('Ctrl Pts',(179.614194658282,584.066568113834,-49.2857766618069)) ;
#54202=CARTESIAN_POINT('Ctrl Pts',(179.560517819468,584.075423643033,-49.2892495104576)) ;
#54203=CARTESIAN_POINT('Ctrl Pts',(179.507354576915,584.086928478519,-49.292775733492)) ;
#54204=CARTESIAN_POINT('Ctrl Pts',(179.454998848441,584.101020396693,-49.2964059494497)) ;
#54205=CARTESIAN_POINT('Ctrl Pts',(179.44673574158,584.103244470908,-49.2969788927218)) ;
#54206=CARTESIAN_POINT('Ctrl Pts',(179.438492652571,584.105532944415,-49.2975544263657)) ;
#54207=CARTESIAN_POINT('Ctrl Pts',(179.430270626706,584.10788552758,-49.2981327493788)) ;
#54208=CARTESIAN_POINT('Ctrl Pts',(179.430236403881,584.107895319819,-49.2981351565528)) ;
#54209=CARTESIAN_POINT('Ctrl Pts',(179.430202181422,584.107905113168,-49.2981375637751)) ;
#54210=CARTESIAN_POINT('Ctrl Pts',(179.430167959327,584.107914907628,-49.2981399710457)) ;
#54211=CARTESIAN_POINT('Ctrl Pts',(179.377307486094,584.123043724261,-49.3018583134886)) ;
#54212=CARTESIAN_POINT('Ctrl Pts',(179.325121598491,584.140887420871,-49.3057022622174)) ;
#54213=CARTESIAN_POINT('Ctrl Pts',(179.273893181901,584.16133916302,-49.309609012445)) ;
#54214=CARTESIAN_POINT('Ctrl Pts',(179.268892802009,584.163335447251,-49.3099903483632)) ;
#54215=CARTESIAN_POINT('Ctrl Pts',(179.263901567599,584.165356546063,-49.3103722826299)) ;
#54216=CARTESIAN_POINT('Ctrl Pts',(179.258919756129,584.167402337824,-49.3107547568374)) ;
#54217=CARTESIAN_POINT('Ctrl Pts',(179.202005494062,584.190774303856,-49.3151242994051)) ;
#54218=CARTESIAN_POINT('Ctrl Pts',(179.146317320101,584.217373982964,-49.3195636175663)) ;
#54219=CARTESIAN_POINT('Ctrl Pts',(179.092218229118,584.247012036341,-49.3239994237309)) ;
#54220=CARTESIAN_POINT('Ctrl Pts',(179.039121233796,584.276101094085,-49.3283530639657)) ;
#54221=CARTESIAN_POINT('Ctrl Pts',(178.987554685352,584.308116639412,-49.3327030365493)) ;
#54222=CARTESIAN_POINT('Ctrl Pts',(178.937836152509,584.34284975659,-49.3370002826777)) ;
#54223=CARTESIAN_POINT('Ctrl Pts',(178.888149236528,584.377560786387,-49.3412947961141)) ;
#54224=CARTESIAN_POINT('Ctrl Pts',(178.840307890223,584.414985838712,-49.3455365073293)) ;
#54225=CARTESIAN_POINT('Ctrl Pts',(178.794606171649,584.454889421259,-49.3497000203128)) ;
#54226=CARTESIAN_POINT('Ctrl Pts',(178.748916150452,584.494782790464,-49.3538624676431)) ;
#54227=CARTESIAN_POINT('Ctrl Pts',(178.705364697062,584.537153420526,-49.3579467461379)) ;
#54228=CARTESIAN_POINT('Ctrl Pts',(178.664223181621,584.581739687353,-49.3619521589631)) ;
#54229=CARTESIAN_POINT('Ctrl Pts',(178.621669202069,584.62785668296,-49.3660950849987)) ;
#54230=CARTESIAN_POINT('Ctrl Pts',(178.581693798529,584.676344295866,-49.3701536069118)) ;
#54231=CARTESIAN_POINT('Ctrl Pts',(178.544570351805,584.726882868498,-49.37415392759)) ;
#54232=CARTESIAN_POINT('Ctrl Pts',(178.50863255681,584.775807335993,-49.3780264856936)) ;
#54233=CARTESIAN_POINT('Ctrl Pts',(178.475367605706,584.826653805537,-49.3818448801019)) ;
#54234=CARTESIAN_POINT('Ctrl Pts',(178.444995694823,584.879103570419,-49.3856546815712)) ;
#54235=CARTESIAN_POINT('Ctrl Pts',(178.41312074896,584.934148951743,-49.3896530212229)) ;
#54236=CARTESIAN_POINT('Ctrl Pts',(178.384433144334,584.990960659604,-49.3936422722471)) ;
#54237=CARTESIAN_POINT('Ctrl Pts',(178.359148090972,585.049134680607,-49.3976942933565)) ;
#54238=CARTESIAN_POINT('Ctrl Pts',(178.337346035383,585.099295272383,-49.4011881514952)) ;
#54239=CARTESIAN_POINT('Ctrl Pts',(178.318073160041,585.150469561677,-49.4047293400311)) ;
#54240=CARTESIAN_POINT('Ctrl Pts',(178.301437748954,585.20237200772,-49.408369639193)) ;
#54241=CARTESIAN_POINT('Ctrl Pts',(178.298785756976,585.210646216864,-49.4089499701583)) ;
#54242=CARTESIAN_POINT('Ctrl Pts',(178.296200705478,585.218938992642,-49.4095328199461)) ;
#54243=CARTESIAN_POINT('Ctrl Pts',(178.293682934059,585.227249250715,-49.410118398344)) ;
#54244=CARTESIAN_POINT('Ctrl Pts',(178.293677611746,585.227266817759,-49.4101196361974)) ;
#54245=CARTESIAN_POINT('Ctrl Pts',(178.293672289732,585.227284384881,-49.410120874063)) ;
#54246=CARTESIAN_POINT('Ctrl Pts',(178.29366696802,585.227301952081,-49.4101221119408)) ;
#54247=CARTESIAN_POINT('Ctrl Pts',(178.277369746688,585.281099775292,-49.4139129910346)) ;
#54248=CARTESIAN_POINT('Ctrl Pts',(178.263842601223,585.335821009913,-49.41782811536)) ;
#54249=CARTESIAN_POINT('Ctrl Pts',(178.253148005755,585.391158117052,-49.4218051187755)) ;
#54250=CARTESIAN_POINT('Ctrl Pts',(178.252075075313,585.396709787236,-49.42220410984)) ;
#54251=CARTESIAN_POINT('Ctrl Pts',(178.251030638063,585.402267616169,-49.4226037237184)) ;
#54252=CARTESIAN_POINT('Ctrl Pts',(178.250014745413,585.407831266905,-49.4230038974354)) ;
#54253=CARTESIAN_POINT('Ctrl Pts',(178.238896357501,585.468722372946,-49.4273835793025)) ;
#54254=CARTESIAN_POINT('Ctrl Pts',(178.231198848605,585.530316549137,-49.4318296844121)) ;
#54255=CARTESIAN_POINT('Ctrl Pts',(178.226957393479,585.592209679162,-49.4362730601451)) ;
#54256=CARTESIAN_POINT('Ctrl Pts',(178.222721181383,585.65402630064,-49.4407109432454)) ;
#54257=CARTESIAN_POINT('Ctrl Pts',(178.221932117161,585.716141233715,-49.4451457640036)) ;
#54258=CARTESIAN_POINT('Ctrl Pts',(178.224586920693,585.77815744219,-49.4495292153227)) ;
#54259=CARTESIAN_POINT('Ctrl Pts',(178.227239278417,585.84011651659,-49.4539086282713)) ;
#54260=CARTESIAN_POINT('Ctrl Pts',(178.233329040899,585.901977131034,-49.458236630351)) ;
#54261=CARTESIAN_POINT('Ctrl Pts',(178.242818227128,585.963347489938,-49.462489098499)) ;
#54262=CARTESIAN_POINT('Ctrl Pts',(178.252301656368,586.024680616099,-49.46673898672)) ;
#54263=CARTESIAN_POINT('Ctrl Pts',(178.265180439986,586.085524097166,-49.4709134398764)) ;
#54264=CARTESIAN_POINT('Ctrl Pts',(178.281382420909,586.145490231204,-49.475013341583)) ;
#54265=CARTESIAN_POINT('Ctrl Pts',(178.297585993295,586.205462255501,-49.4791136460083)) ;
#54266=CARTESIAN_POINT('Ctrl Pts',(178.317113611036,586.264556692915,-49.4831395187431)) ;
#54267=CARTESIAN_POINT('Ctrl Pts',(178.339856941589,586.32238948273,-49.4871157690085)) ;
#54268=CARTESIAN_POINT('Ctrl Pts',(178.362599508045,586.380220329561,-49.4910918856856)) ;
#54269=CARTESIAN_POINT('Ctrl Pts',(178.388557894661,586.436789430184,-49.4950186757842)) ;
#54270=CARTESIAN_POINT('Ctrl Pts',(178.417583737016,586.491718346697,-49.4989417091056)) ;
#54271=CARTESIAN_POINT('Ctrl Pts',(178.446638728903,586.546702426199,-49.5028686821778)) ;
#54272=CARTESIAN_POINT('Ctrl Pts',(178.478767778577,586.600042640508,-49.5067923950255)) ;
#54273=CARTESIAN_POINT('Ctrl Pts',(178.51377617567,586.65136916444,-49.5107734463125)) ;
#54274=CARTESIAN_POINT('Ctrl Pts',(178.546547199693,586.69941543015,-49.514500070157)) ;
#54275=CARTESIAN_POINT('Ctrl Pts',(178.581841161819,586.745696770216,-49.5182775936648)) ;
#54276=CARTESIAN_POINT('Ctrl Pts',(178.619456745563,586.789923813584,-49.5221601717599)) ;
#54277=CARTESIAN_POINT('',(181.142689770678,586.808573586438,-49.5221525629812)) ;
#54278=CARTESIAN_POINT('Origin',(179.888527625416,585.710565160536,-49.5221601717598)) ;
#54279=CARTESIAN_POINT('',(181.554057944425,585.711436268501,-48.8998676108129)) ;
#54280=CARTESIAN_POINT('Ctrl Pts',(181.142689782808,586.808573597058,-49.5221525628444)) ;
#54281=CARTESIAN_POINT('Ctrl Pts',(181.107984462542,586.848168254349,-49.5185580363667)) ;
#54282=CARTESIAN_POINT('Ctrl Pts',(181.071300684857,586.886147988108,-49.5148671084872)) ;
#54283=CARTESIAN_POINT('Ctrl Pts',(181.03282965584,586.922325429852,-49.5111334393229)) ;
#54284=CARTESIAN_POINT('Ctrl Pts',(180.98877560723,586.963753039612,-49.5068579300094)) ;
#54285=CARTESIAN_POINT('Ctrl Pts',(180.94237691035,587.002818089248,-49.5025269351851)) ;
#54286=CARTESIAN_POINT('Ctrl Pts',(180.89393693784,587.039280186148,-49.4982065963733)) ;
#54287=CARTESIAN_POINT('Ctrl Pts',(180.845546327173,587.075705127033,-49.4938906601216)) ;
#54288=CARTESIAN_POINT('Ctrl Pts',(180.795118731165,587.10953269946,-49.4895856561117)) ;
#54289=CARTESIAN_POINT('Ctrl Pts',(180.742973687493,587.140557484973,-49.4853367559894)) ;
#54290=CARTESIAN_POINT('Ctrl Pts',(180.690861998196,587.171562425603,-49.4810905736596)) ;
#54291=CARTESIAN_POINT('Ctrl Pts',(180.637035096445,587.199768259184,-49.4769005415144)) ;
#54292=CARTESIAN_POINT('Ctrl Pts',(180.581827802258,587.225001374835,-49.4727879430955)) ;
#54293=CARTESIAN_POINT('Ctrl Pts',(180.526634877501,587.250227922777,-49.4686764151093)) ;
#54294=CARTESIAN_POINT('Ctrl Pts',(180.470062289381,587.27248324267,-49.4646422709636)) ;
#54295=CARTESIAN_POINT('Ctrl Pts',(180.412460153598,587.291625017121,-49.4606821959048)) ;
#54296=CARTESIAN_POINT('Ctrl Pts',(180.354809484317,587.310782919746,-49.4567187842284)) ;
#54297=CARTESIAN_POINT('Ctrl Pts',(180.296127532896,587.326821832658,-49.4528294423666)) ;
#54298=CARTESIAN_POINT('Ctrl Pts',(180.236780813647,587.339632199945,-49.4489872070466)) ;
#54299=CARTESIAN_POINT('Ctrl Pts',(180.177411791505,587.352447381453,-49.4451435277889)) ;
#54300=CARTESIAN_POINT('Ctrl Pts',(180.117377518728,587.362031250819,-49.441346717111)) ;
#54301=CARTESIAN_POINT('Ctrl Pts',(180.057060338566,587.368311241818,-49.4375490757087)) ;
#54302=CARTESIAN_POINT('Ctrl Pts',(179.996628619868,587.374603158125,-49.4337442228239)) ;
#54303=CARTESIAN_POINT('Ctrl Pts',(179.935913016452,587.377578105159,-49.4299380617709)) ;
#54304=CARTESIAN_POINT('Ctrl Pts',(179.875312773369,587.377206876537,-49.4260673862609)) ;
#54305=CARTESIAN_POINT('Ctrl Pts',(179.820862517637,587.376873321877,-49.4225895244464)) ;
#54306=CARTESIAN_POINT('Ctrl Pts',(179.766505007503,587.373838347776,-49.4190589885622)) ;
#54307=CARTESIAN_POINT('Ctrl Pts',(179.712540166677,587.368117441668,-49.4154254390394)) ;
#54308=CARTESIAN_POINT('Ctrl Pts',(179.707745453804,587.367609145864,-49.4151026024219)) ;
#54309=CARTESIAN_POINT('Ctrl Pts',(179.702953812063,587.367079665455,-49.4147789526031)) ;
#54310=CARTESIAN_POINT('Ctrl Pts',(179.698165434781,587.366529021736,-49.4144544542754)) ;
#54311=CARTESIAN_POINT('Ctrl Pts',(179.698131755894,587.366525148802,-49.4144521719276)) ;
#54312=CARTESIAN_POINT('Ctrl Pts',(179.698098077168,587.366521274822,-49.4144498895378)) ;
#54313=CARTESIAN_POINT('Ctrl Pts',(179.698064398604,587.366517399794,-49.414447607106)) ;
#54314=CARTESIAN_POINT('Ctrl Pts',(179.642896317683,587.360169806438,-49.4107088080871)) ;
#54315=CARTESIAN_POINT('Ctrl Pts',(179.587963110748,587.350981727434,-49.4068474613973)) ;
#54316=CARTESIAN_POINT('Ctrl Pts',(179.53356734119,587.33901541415,-49.4029266301077)) ;
#54317=CARTESIAN_POINT('Ctrl Pts',(179.528499936043,587.337900655447,-49.4025613730148)) ;
#54318=CARTESIAN_POINT('Ctrl Pts',(179.523437221136,587.336761812741,-49.4021955996892)) ;
#54319=CARTESIAN_POINT('Ctrl Pts',(179.518379456723,587.335598953164,-49.4018293611151)) ;
#54320=CARTESIAN_POINT('Ctrl Pts',(179.458430829169,587.32181582094,-49.3974884116204)) ;
#54321=CARTESIAN_POINT('Ctrl Pts',(179.39917320668,587.304654617268,-49.3930827597336)) ;
#54322=CARTESIAN_POINT('Ctrl Pts',(179.340991973531,587.284243100262,-49.3886832329072)) ;
#54323=CARTESIAN_POINT('Ctrl Pts',(179.283548964587,587.264090571852,-49.384339528844)) ;
#54324=CARTESIAN_POINT('Ctrl Pts',(179.227154971626,587.240770057717,-49.3800020875789)) ;
#54325=CARTESIAN_POINT('Ctrl Pts',(179.172160543843,587.214437864316,-49.3757185289197)) ;
#54326=CARTESIAN_POINT('Ctrl Pts',(179.117199455987,587.188121634594,-49.3714375671332)) ;
#54327=CARTESIAN_POINT('Ctrl Pts',(179.063636152059,587.158797475377,-49.3672105577313)) ;
#54328=CARTESIAN_POINT('Ctrl Pts',(179.011802420145,587.126651659001,-49.3630612214273)) ;
#54329=CARTESIAN_POINT('Ctrl Pts',(178.959980983161,587.094513467592,-49.3589128693433)) ;
#54330=CARTESIAN_POINT('Ctrl Pts',(178.909888329004,587.059554939623,-49.35484215551)) ;
#54331=CARTESIAN_POINT('Ctrl Pts',(178.861838281852,587.021991904379,-49.3508479809358)) ;
#54332=CARTESIAN_POINT('Ctrl Pts',(178.812648695837,586.98353803674,-49.3467590818521)) ;
#54333=CARTESIAN_POINT('Ctrl Pts',(178.765599983442,586.942354422518,-49.342750368405)) ;
#54334=CARTESIAN_POINT('Ctrl Pts',(178.721008159666,586.898705850122,-49.3387946729961)) ;
#54335=CARTESIAN_POINT('Ctrl Pts',(178.677394024503,586.85601428528,-49.3349257073513)) ;
#54336=CARTESIAN_POINT('Ctrl Pts',(178.636130423477,586.810964610041,-49.3311071067563)) ;
#54337=CARTESIAN_POINT('Ctrl Pts',(178.597490526956,586.763837833895,-49.32729200388)) ;
#54338=CARTESIAN_POINT('Ctrl Pts',(178.557551357159,586.715126411663,-49.3233486175025)) ;
#54339=CARTESIAN_POINT('Ctrl Pts',(178.520416004959,586.664195401138,-49.3194085375781)) ;
#54340=CARTESIAN_POINT('Ctrl Pts',(178.486354817132,586.611395428241,-49.315402397988)) ;
#54341=CARTESIAN_POINT('Ctrl Pts',(178.456715576896,586.565450140332,-49.3119163500458)) ;
#54342=CARTESIAN_POINT('Ctrl Pts',(178.429403520484,586.518088983246,-49.3083796318267)) ;
#54343=CARTESIAN_POINT('Ctrl Pts',(178.404572302892,586.46957357431,-49.3047416214865)) ;
#54344=CARTESIAN_POINT('Ctrl Pts',(178.400881920831,586.462363279681,-49.3042009452974)) ;
#54345=CARTESIAN_POINT('Ctrl Pts',(178.397246248602,586.455127452085,-49.3036580318183)) ;
#54346=CARTESIAN_POINT('Ctrl Pts',(178.393665701765,586.44786690752,-49.303112714877)) ;
#54347=CARTESIAN_POINT('Ctrl Pts',(178.393651880362,586.447838880819,-49.3031106098786)) ;
#54348=CARTESIAN_POINT('Ctrl Pts',(178.39363805978,586.447810853749,-49.3031085048444)) ;
#54349=CARTESIAN_POINT('Ctrl Pts',(178.393624240019,586.447782826312,-49.3031063997743)) ;
#54350=CARTESIAN_POINT('Ctrl Pts',(178.369108043619,586.398062271909,-49.2993720144895)) ;
#54351=CARTESIAN_POINT('Ctrl Pts',(178.347096457758,586.347001046843,-49.2955151006196)) ;
#54352=CARTESIAN_POINT('Ctrl Pts',(178.327701549311,586.29488609049,-49.2915988750396)) ;
#54353=CARTESIAN_POINT('Ctrl Pts',(178.325903343545,586.290054233959,-49.2912357808058)) ;
#54354=CARTESIAN_POINT('Ctrl Pts',(178.32412762298,586.285213355516,-49.2908721767205)) ;
#54355=CARTESIAN_POINT('Ctrl Pts',(178.322374471421,586.280363705792,-49.2905081131671)) ;
#54356=CARTESIAN_POINT('Ctrl Pts',(178.301455498579,586.22249666607,-49.2861640303352)) ;
#54357=CARTESIAN_POINT('Ctrl Pts',(178.283750767876,586.163374848216,-49.2817551958583)) ;
#54358=CARTESIAN_POINT('Ctrl Pts',(178.269362954821,586.103392394662,-49.2773529891969)) ;
#54359=CARTESIAN_POINT('Ctrl Pts',(178.255191439883,586.04431168286,-49.2730169627817)) ;
#54360=CARTESIAN_POINT('Ctrl Pts',(178.244237416278,585.984396026408,-49.2686876489745)) ;
#54361=CARTESIAN_POINT('Ctrl Pts',(178.236559961635,585.924023222118,-49.2644127041021)) ;
#54362=CARTESIAN_POINT('Ctrl Pts',(178.22888728024,585.863687952967,-49.2601404170599)) ;
#54363=CARTESIAN_POINT('Ctrl Pts',(178.224486968306,585.80289609105,-49.2559225653516)) ;
#54364=CARTESIAN_POINT('Ctrl Pts',(178.223382757553,585.74202602782,-49.2517829466959)) ;
#54365=CARTESIAN_POINT('Ctrl Pts',(178.222278821394,585.681171101718,-49.2476443574778)) ;
#54366=CARTESIAN_POINT('Ctrl Pts',(178.224469379528,585.620238034422,-49.2435839645257)) ;
#54367=CARTESIAN_POINT('Ctrl Pts',(178.229943572563,585.559606195112,-49.2396007952297)) ;
#54368=CARTESIAN_POINT('Ctrl Pts',(178.23557092052,585.49727802091,-49.235506186315)) ;
#54369=CARTESIAN_POINT('Ctrl Pts',(178.244668567839,585.435268238171,-49.2314931739831)) ;
#54370=CARTESIAN_POINT('Ctrl Pts',(178.257185002814,585.373989606572,-49.2275343780659)) ;
#54371=CARTESIAN_POINT('Ctrl Pts',(178.269376243481,585.314303078659,-49.2236784371473)) ;
#54372=CARTESIAN_POINT('Ctrl Pts',(178.284811055711,585.255310343257,-49.2198735637431)) ;
#54373=CARTESIAN_POINT('Ctrl Pts',(178.303401637145,585.197391862252,-49.2160729854487)) ;
#54374=CARTESIAN_POINT('Ctrl Pts',(178.322736058126,585.137155968165,-49.2121203398055)) ;
#54375=CARTESIAN_POINT('Ctrl Pts',(178.345484658224,585.078082371193,-49.2081719214991)) ;
#54376=CARTESIAN_POINT('Ctrl Pts',(178.371496808442,585.020594370926,-49.2041571171506)) ;
#54377=CARTESIAN_POINT('Ctrl Pts',(178.393998334916,584.970865004106,-49.2006841544934)) ;
#54378=CARTESIAN_POINT('Ctrl Pts',(178.418942193086,584.922321201104,-49.1971608572299)) ;
#54379=CARTESIAN_POINT('Ctrl Pts',(178.446191760885,584.875233004446,-49.193536554343)) ;
#54380=CARTESIAN_POINT('Ctrl Pts',(178.450428110662,584.86791244535,-49.192973102664)) ;
#54381=CARTESIAN_POINT('Ctrl Pts',(178.454720172327,584.860626965898,-49.1924072097481)) ;
#54382=CARTESIAN_POINT('Ctrl Pts',(178.459067418464,584.85337746811,-49.1918386852)) ;
#54383=CARTESIAN_POINT('Ctrl Pts',(178.459082862209,584.853351714015,-49.1918366654966)) ;
#54384=CARTESIAN_POINT('Ctrl Pts',(178.459098306649,584.853325960374,-49.19183464576)) ;
#54385=CARTESIAN_POINT('Ctrl Pts',(178.459113751787,584.853300207187,-49.1918326259902)) ;
#54386=CARTESIAN_POINT('Ctrl Pts',(178.487624142231,584.805762046414,-49.1881043051814)) ;
#54387=CARTESIAN_POINT('Ctrl Pts',(178.518617592855,584.759603881883,-49.18425292184)) ;
#54388=CARTESIAN_POINT('Ctrl Pts',(178.551913455752,584.715075054469,-49.1803416167241)) ;
#54389=CARTESIAN_POINT('Ctrl Pts',(178.55502638043,584.710911928073,-49.179975937713)) ;
#54390=CARTESIAN_POINT('Ctrl Pts',(178.558159394931,584.706763056428,-49.179609734931)) ;
#54391=CARTESIAN_POINT('Ctrl Pts',(178.561312329619,584.702628650688,-49.1792430599776)) ;
#54392=CARTESIAN_POINT('Ctrl Pts',(178.598625129582,584.65370082008,-49.1749037156707)) ;
#54393=CARTESIAN_POINT('Ctrl Pts',(178.638733271553,584.606796511376,-49.1704989107955)) ;
#54394=CARTESIAN_POINT('Ctrl Pts',(178.681360830051,584.562215154816,-49.1661000410291)) ;
#54395=CARTESIAN_POINT('Ctrl Pts',(178.723373783523,584.518276573184,-49.1617645942586)) ;
#54396=CARTESIAN_POINT('Ctrl Pts',(178.767833778899,584.476594070801,-49.1574351996113)) ;
#54397=CARTESIAN_POINT('Ctrl Pts',(178.814454604535,584.437422014611,-49.1531596741286)) ;
#54398=CARTESIAN_POINT('Ctrl Pts',(178.861046800754,584.398274013617,-49.1488867742064)) ;
#54399=CARTESIAN_POINT('Ctrl Pts',(178.909797116817,584.361633259874,-49.144667812578)) ;
#54400=CARTESIAN_POINT('Ctrl Pts',(178.960399765495,584.327724663864,-49.1405267321975)) ;
#54401=CARTESIAN_POINT('Ctrl Pts',(179.010990156184,584.293824281874,-49.1363866549526)) ;
#54402=CARTESIAN_POINT('Ctrl Pts',(179.06343198272,584.262654770551,-49.1323244239374)) ;
#54403=CARTESIAN_POINT('Ctrl Pts',(179.117399960444,584.234412463701,-49.1283391819763)) ;
#54404=CARTESIAN_POINT('Ctrl Pts',(179.172816837166,584.205411924806,-49.1242469466957)) ;
#54405=CARTESIAN_POINT('Ctrl Pts',(179.229843040947,584.179498206949,-49.1202358771053)) ;
#54406=CARTESIAN_POINT('Ctrl Pts',(179.288104459943,584.156850973599,-49.1162787826406)) ;
#54407=CARTESIAN_POINT('Ctrl Pts',(179.344915081598,584.134767690571,-49.1124202258056)) ;
#54408=CARTESIAN_POINT('Ctrl Pts',(179.402900122557,584.115790423885,-49.1086126257215)) ;
#54409=CARTESIAN_POINT('Ctrl Pts',(179.461691796814,584.100051466002,-49.1048092711824)) ;
#54410=CARTESIAN_POINT('Ctrl Pts',(179.522735553577,584.083709609288,-49.100860224786)) ;
#54411=CARTESIAN_POINT('Ctrl Pts',(179.584649064956,584.07085977513,-49.096915335282)) ;
#54412=CARTESIAN_POINT('Ctrl Pts',(179.646996633105,584.061604210247,-49.0929043640023)) ;
#54413=CARTESIAN_POINT('Ctrl Pts',(179.701034699138,584.053582200069,-49.0894279632814)) ;
#54414=CARTESIAN_POINT('Ctrl Pts',(179.755399729108,584.048259951212,-49.0859012657915)) ;
#54415=CARTESIAN_POINT('Ctrl Pts',(179.809790218402,584.045669015311,-49.0822735343401)) ;
#54416=CARTESIAN_POINT('Ctrl Pts',(179.818124300906,584.045272014404,-49.0817176685332)) ;
#54417=CARTESIAN_POINT('Ctrl Pts',(179.826459055938,584.044939074602,-49.0811594306042)) ;
#54418=CARTESIAN_POINT('Ctrl Pts',(179.834793482175,584.044670239962,-49.0805986380245)) ;
#54419=CARTESIAN_POINT('Ctrl Pts',(179.834823095581,584.044669284754,-49.0805966454484)) ;
#54420=CARTESIAN_POINT('Ctrl Pts',(179.834852708984,584.044668330355,-49.08059465284)) ;
#54421=CARTESIAN_POINT('Ctrl Pts',(179.834882322383,584.044667376766,-49.0805926601994)) ;
#54422=CARTESIAN_POINT('Ctrl Pts',(179.89031287822,584.042882441949,-49.0768628222176)) ;
#54423=CARTESIAN_POINT('Ctrl Pts',(179.945928073396,584.043934871952,-49.0730101401795)) ;
#54424=CARTESIAN_POINT('Ctrl Pts',(180.001420128914,584.047807748355,-49.0690977612818)) ;
#54425=CARTESIAN_POINT('Ctrl Pts',(180.006592146767,584.048168711482,-49.0687331164094)) ;
#54426=CARTESIAN_POINT('Ctrl Pts',(180.011763065144,584.048554152583,-49.0683679529639)) ;
#54427=CARTESIAN_POINT('Ctrl Pts',(180.016932616892,584.048964043609,-49.0680023220714)) ;
#54428=CARTESIAN_POINT('Ctrl Pts',(180.078269623518,584.053827422453,-49.0636640920727)) ;
#54429=CARTESIAN_POINT('Ctrl Pts',(180.139419264204,584.062136143938,-49.0592607207662)) ;
#54430=CARTESIAN_POINT('Ctrl Pts',(180.199980570948,584.073820390237,-49.0548634692596)) ;
#54431=CARTESIAN_POINT('Ctrl Pts',(180.259684216819,584.085339165851,-49.0505284910224)) ;
#54432=CARTESIAN_POINT('Ctrl Pts',(180.318816251292,584.100138128127,-49.0461997476564)) ;
#54433=CARTESIAN_POINT('Ctrl Pts',(180.377007710914,584.118114368945,-49.0419249684783)) ;
#54434=CARTESIAN_POINT('Ctrl Pts',(180.435163684631,584.136079647619,-49.0376527961159)) ;
#54435=CARTESIAN_POINT('Ctrl Pts',(180.492380297348,584.157218219851,-49.033434657059)) ;
#54436=CARTESIAN_POINT('Ctrl Pts',(180.548302743424,584.181394770773,-49.0292943989477)) ;
#54437=CARTESIAN_POINT('Ctrl Pts',(180.60421185903,584.205565558629,-49.0251551277673)) ;
#54438=CARTESIAN_POINT('Ctrl Pts',(180.658827394703,584.232772897588,-49.021093702746)) ;
#54439=CARTESIAN_POINT('Ctrl Pts',(180.71180800419,584.262849602764,-49.017109168591)) ;
#54440=CARTESIAN_POINT('Ctrl Pts',(180.766185932191,584.293719555458,-49.0130195457364)) ;
#54441=CARTESIAN_POINT('Ctrl Pts',(180.818841350595,584.327612510181,-49.0090109078189)) ;
#54442=CARTESIAN_POINT('Ctrl Pts',(180.869420955123,584.364311501216,-49.0050560054703)) ;
#54443=CARTESIAN_POINT('Ctrl Pts',(180.918764119481,584.400113369644,-49.0011977824092)) ;
#54444=CARTESIAN_POINT('Ctrl Pts',(180.966131535035,584.438585829195,-48.9973903373221)) ;
#54445=CARTESIAN_POINT('Ctrl Pts',(181.011212654959,584.479491266715,-48.9935868859116)) ;
#54446=CARTESIAN_POINT('Ctrl Pts',(181.057988237781,584.521934215867,-48.9896404742703)) ;
#54447=CARTESIAN_POINT('Ctrl Pts',(181.102301774941,584.56699705875,-48.9856979397272)) ;
#54448=CARTESIAN_POINT('Ctrl Pts',(181.143831842375,584.614369438218,-48.9816891407575)) ;
#54449=CARTESIAN_POINT('Ctrl Pts',(181.179841353531,584.655444647874,-48.978213228)) ;
#54450=CARTESIAN_POINT('Ctrl Pts',(181.213758940726,584.698256791488,-48.9746868419877)) ;
#54451=CARTESIAN_POINT('Ctrl Pts',(181.245394843605,584.742569634588,-48.9710592886712)) ;
#54452=CARTESIAN_POINT('Ctrl Pts',(181.250227492098,584.74933879162,-48.9705051495927)) ;
#54453=CARTESIAN_POINT('Ctrl Pts',(181.255006992596,584.756142994574,-48.9699486497634)) ;
#54454=CARTESIAN_POINT('Ctrl Pts',(181.259732771233,584.76298143342,-48.9693896084778)) ;
#54455=CARTESIAN_POINT('Ctrl Pts',(181.259749783921,584.763006051632,-48.9693875959429)) ;
#54456=CARTESIAN_POINT('Ctrl Pts',(181.259766795912,584.763030670289,-48.969385583375)) ;
#54457=CARTESIAN_POINT('Ctrl Pts',(181.259783807207,584.763055289389,-48.9693835707741)) ;
#54458=CARTESIAN_POINT('Ctrl Pts',(181.291520131742,584.808984757977,-48.9656288564589)) ;
#54459=CARTESIAN_POINT('Ctrl Pts',(181.320938077529,584.856624312683,-48.9617498451787)) ;
#54460=CARTESIAN_POINT('Ctrl Pts',(181.347885531636,584.905704447521,-48.9578107311307)) ;
#54461=CARTESIAN_POINT('Ctrl Pts',(181.350579740329,584.910611483467,-48.957416898182)) ;
#54462=CARTESIAN_POINT('Ctrl Pts',(181.353249255775,584.915532876534,-48.9570224644449)) ;
#54463=CARTESIAN_POINT('Ctrl Pts',(181.35589392791,584.920468328871,-48.9566274940753)) ;
#54464=CARTESIAN_POINT('Ctrl Pts',(181.38494191897,584.974677307554,-48.9522893019751)) ;
#54465=CARTESIAN_POINT('Ctrl Pts',(181.41099312482,585.030588422366,-48.9478870035079)) ;
#54466=CARTESIAN_POINT('Ctrl Pts',(181.43389140552,585.08783326796,-48.9434912449672)) ;
#54467=CARTESIAN_POINT('Ctrl Pts',(181.45675452436,585.144990210221,-48.9391022364112)) ;
#54468=CARTESIAN_POINT('Ctrl Pts',(181.476474770402,585.203476780266,-48.9347200839646)) ;
#54469=CARTESIAN_POINT('Ctrl Pts',(181.492934154698,585.262919802661,-48.9303936265267)) ;
#54470=CARTESIAN_POINT('Ctrl Pts',(181.509378746909,585.322309403482,-48.9260710572855)) ;
#54471=CARTESIAN_POINT('Ctrl Pts',(181.522568473053,585.382653783217,-48.9218042230144)) ;
#54472=CARTESIAN_POINT('Ctrl Pts',(181.532419267779,585.443573947974,-48.9176168821652)) ;
#54473=CARTESIAN_POINT('Ctrl Pts',(181.542264969106,585.50446261368,-48.9134317063998)) ;
#54474=CARTESIAN_POINT('Ctrl Pts',(181.548775146656,585.565926503788,-48.9093259471425)) ;
#54475=CARTESIAN_POINT('Ctrl Pts',(181.551898804922,585.627579766142,-48.9052973376481)) ;
#54476=CARTESIAN_POINT('Ctrl Pts',(181.553313650828,585.655505313185,-48.903472598459)) ;
#54477=CARTESIAN_POINT('Ctrl Pts',(181.554034172762,585.683469607269,-48.9016633335739)) ;
#54478=CARTESIAN_POINT('Ctrl Pts',(181.554057944425,585.711436268501,-48.8998676108129)) ;
#54479=CARTESIAN_POINT('Ctrl Pts',(181.554527406634,585.711418964488,-48.8995973781893)) ;
#54480=CARTESIAN_POINT('Ctrl Pts',(181.554489983662,585.784441188358,-48.8949679628962)) ;
#54481=CARTESIAN_POINT('Ctrl Pts',(181.549651778247,585.857385731781,-48.8904707120407)) ;
#54482=CARTESIAN_POINT('Ctrl Pts',(181.526228131845,586.033851596541,-48.8795849394622)) ;
#54483=CARTESIAN_POINT('Ctrl Pts',(181.502610161245,586.136370402795,-48.8732596311718)) ;
#54484=CARTESIAN_POINT('Ctrl Pts',(181.463924712828,586.252776874084,-48.8654287208587)) ;
#54485=CARTESIAN_POINT('Ctrl Pts',(181.458073665102,586.269487882621,-48.8642879440639)) ;
#54486=CARTESIAN_POINT('Ctrl Pts',(181.45195815568,586.286100543496,-48.8631342200737)) ;
#54487=CARTESIAN_POINT('Origin',(179.888527625407,535.710565160536,-48.5221601717598)) ;
#54488=CARTESIAN_POINT('',(181.45221818455,536.286166738762,-47.6539472813452)) ;
#54489=CARTESIAN_POINT('',(181.451956083813,536.286106171625,-47.5221601717599)) ;
#54490=CARTESIAN_POINT('',(181.451956083813,536.286106171625,-48.5221601717599)) ;
#54491=CARTESIAN_POINT('',(179.964851548283,537.375708203335,-47.5221677607717)) ;
#54492=CARTESIAN_POINT('Origin',(179.888527625407,535.710565160536,-47.5221601717598)) ;
#54493=CARTESIAN_POINT('Ctrl Pts',(179.964851549022,537.375708219471,-47.5221677609092)) ;
#54494=CARTESIAN_POINT('Ctrl Pts',(180.017493447496,537.373264646232,-47.5257656577699)) ;
#54495=CARTESIAN_POINT('Ctrl Pts',(180.070106532583,537.368262770555,-47.5294601611829)) ;
#54496=CARTESIAN_POINT('Ctrl Pts',(180.122424397359,537.360735327514,-47.5331974679367)) ;
#54497=CARTESIAN_POINT('Ctrl Pts',(180.182280313502,537.35212331704,-47.5374732525202)) ;
#54498=CARTESIAN_POINT('Ctrl Pts',(180.241751057591,537.340205240901,-47.541804502013)) ;
#54499=CARTESIAN_POINT('Ctrl Pts',(180.300459543354,537.325068387249,-47.5461250770343)) ;
#54500=CARTESIAN_POINT('Ctrl Pts',(180.359108191529,537.309946961567,-47.5504412483859)) ;
#54501=CARTESIAN_POINT('Ctrl Pts',(180.416996272399,537.291613595545,-47.5547464690616)) ;
#54502=CARTESIAN_POINT('Ctrl Pts',(180.473763962208,537.270190023334,-47.5589955665134)) ;
#54503=CARTESIAN_POINT('Ctrl Pts',(180.530495330378,537.248780158556,-47.5632419452675)) ;
#54504=CARTESIAN_POINT('Ctrl Pts',(180.586107791095,537.224284130594,-47.5674321545138)) ;
#54505=CARTESIAN_POINT('Ctrl Pts',(180.640256859013,537.196855454874,-47.571544907143)) ;
#54506=CARTESIAN_POINT('Ctrl Pts',(180.694391823976,537.169433922866,-47.5756565886187)) ;
#54507=CARTESIAN_POINT('Ctrl Pts',(180.747064106785,537.139081243039,-47.5796908633611)) ;
#54508=CARTESIAN_POINT('Ctrl Pts',(180.797944151154,537.105982401317,-47.5836510404053)) ;
#54509=CARTESIAN_POINT('Ctrl Pts',(180.848867058718,537.07285567593,-47.5876145536463)) ;
#54510=CARTESIAN_POINT('Ctrl Pts',(180.897994553398,537.036978038971,-47.5915039683802)) ;
#54511=CARTESIAN_POINT('Ctrl Pts',(180.945012468566,536.998567723417,-47.595346240642)) ;
#54512=CARTESIAN_POINT('Ctrl Pts',(180.992048047913,536.960142977477,-47.5991899564084)) ;
#54513=CARTESIAN_POINT('Ctrl Pts',(181.036972186419,536.91918345128,-47.6029867675705)) ;
#54514=CARTESIAN_POINT('Ctrl Pts',(181.079489768143,536.875942814335,-47.6067843656198)) ;
#54515=CARTESIAN_POINT('Ctrl Pts',(181.122088091324,536.83262006284,-47.6105891753587)) ;
#54516=CARTESIAN_POINT('Ctrl Pts',(181.162270232401,536.787007274233,-47.614395249141)) ;
#54517=CARTESIAN_POINT('Ctrl Pts',(181.199764436783,536.739398363538,-47.6182657863322)) ;
#54518=CARTESIAN_POINT('Ctrl Pts',(181.233454623253,536.696619669994,-47.6217436336917)) ;
#54519=CARTESIAN_POINT('Ctrl Pts',(181.264974901598,536.652229070148,-47.6252741171322)) ;
#54520=CARTESIAN_POINT('Ctrl Pts',(181.294150364587,536.606470722797,-47.6289075781151)) ;
#54521=CARTESIAN_POINT('Ctrl Pts',(181.296749413567,536.602394414358,-47.6292312591159)) ;
#54522=CARTESIAN_POINT('Ctrl Pts',(181.299329886898,536.598307240734,-47.629555757331)) ;
#54523=CARTESIAN_POINT('Ctrl Pts',(181.301891679859,536.594209367662,-47.6298811083493)) ;
#54524=CARTESIAN_POINT('Ctrl Pts',(181.301909469313,536.59418091145,-47.6298833676329)) ;
#54525=CARTESIAN_POINT('Ctrl Pts',(181.301927257866,536.594152454722,-47.6298856269576)) ;
#54526=CARTESIAN_POINT('Ctrl Pts',(181.301945045518,536.594123997479,-47.6298878863235)) ;
#54527=CARTESIAN_POINT('Ctrl Pts',(181.331804988159,536.546353124972,-47.6336806598109)) ;
#54528=CARTESIAN_POINT('Ctrl Pts',(181.359221289387,536.496961798078,-47.6375987039909)) ;
#54529=CARTESIAN_POINT('Ctrl Pts',(181.384055566174,536.44622998794,-47.6415767454939)) ;
#54530=CARTESIAN_POINT('Ctrl Pts',(181.386698090807,536.440831801428,-47.6420000343521)) ;
#54531=CARTESIAN_POINT('Ctrl Pts',(181.389311383618,536.435418486105,-47.6424240025185)) ;
#54532=CARTESIAN_POINT('Ctrl Pts',(181.391895280729,536.429990413812,-47.6428485713542)) ;
#54533=CARTESIAN_POINT('Ctrl Pts',(181.414225124921,536.38308142195,-47.64651766325)) ;
#54534=CARTESIAN_POINT('Ctrl Pts',(181.434360511508,536.335066076585,-47.6502315179149)) ;
#54535=CARTESIAN_POINT('Ctrl Pts',(181.45221818455,536.286166738761,-47.6539472813452)) ;
#54536=CARTESIAN_POINT('Origin',(179.888527625407,535.710565160536,-48.5221601717598)) ;
#54537=CARTESIAN_POINT('',(181.451956081261,536.286106178557,-48.355715363061)) ;
#54538=CARTESIAN_POINT('',(181.451936403117,536.286095981694,-48.1612817710483)) ;
#54539=CARTESIAN_POINT('',(181.451956083813,536.286106171625,-48.5221601717599)) ;
#54540=CARTESIAN_POINT('',(181.523656952658,535.391334705907,-47.5221601717599)) ;
#54541=CARTESIAN_POINT('Ctrl Pts',(181.451936403117,536.286095981694,-48.1612817710483)) ;
#54542=CARTESIAN_POINT('Ctrl Pts',(181.430786255221,536.3431128388,-48.1569560749123)) ;
#54543=CARTESIAN_POINT('Ctrl Pts',(181.406503744676,536.39902563506,-48.1526530389213)) ;
#54544=CARTESIAN_POINT('Ctrl Pts',(181.379248521711,536.453487888781,-48.1484135941381)) ;
#54545=CARTESIAN_POINT('Ctrl Pts',(181.352007036685,536.507922690917,-48.1441762862382)) ;
#54546=CARTESIAN_POINT('Ctrl Pts',(181.321795895814,536.560908459043,-48.140002597123)) ;
#54547=CARTESIAN_POINT('Ctrl Pts',(181.288804681928,536.612116603094,-48.1359091023072)) ;
#54548=CARTESIAN_POINT('Ctrl Pts',(181.255817829905,536.663317976772,-48.131816148704)) ;
#54549=CARTESIAN_POINT('Ctrl Pts',(181.220051596958,536.71274213145,-48.1278033364018)) ;
#54550=CARTESIAN_POINT('Ctrl Pts',(181.181725573904,536.760078123245,-48.1238625130584)) ;
#54551=CARTESIAN_POINT('Ctrl Pts',(181.143362610377,536.807459739758,-48.1199178913588)) ;
#54552=CARTESIAN_POINT('Ctrl Pts',(181.10243479128,536.852748988088,-48.1160452476124)) ;
#54553=CARTESIAN_POINT('Ctrl Pts',(181.059193789639,536.89565339179,-48.1122129738959)) ;
#54554=CARTESIAN_POINT('Ctrl Pts',(181.015932218975,536.9385782044,-48.1083788772308)) ;
#54555=CARTESIAN_POINT('Ctrl Pts',(180.970355069448,536.9791155841,-48.1045848793185)) ;
#54556=CARTESIAN_POINT('Ctrl Pts',(180.92274828037,537.016995687241,-48.1007792862713)) ;
#54557=CARTESIAN_POINT('Ctrl Pts',(180.875051662244,537.054947266187,-48.0969665124669)) ;
#54558=CARTESIAN_POINT('Ctrl Pts',(180.825317518399,537.090230986917,-48.0931415739393)) ;
#54559=CARTESIAN_POINT('Ctrl Pts',(180.773870657243,537.122605010773,-48.089238577472)) ;
#54560=CARTESIAN_POINT('Ctrl Pts',(180.732417795799,537.148690099253,-48.0860937719747)) ;
#54561=CARTESIAN_POINT('Ctrl Pts',(180.689853713353,537.172886512724,-48.0828978288437)) ;
#54562=CARTESIAN_POINT('Ctrl Pts',(180.646366990726,537.195086142804,-48.0796140404029)) ;
#54563=CARTESIAN_POINT('Ctrl Pts',(180.646340288671,537.195099773994,-48.0796120240655)) ;
#54564=CARTESIAN_POINT('Ctrl Pts',(180.646313586266,537.195113404431,-48.0796100076951)) ;
#54565=CARTESIAN_POINT('Ctrl Pts',(180.646286883514,537.195127034117,-48.0796079912915)) ;
#54566=CARTESIAN_POINT('Ctrl Pts',(180.596942026413,537.220313760083,-48.0758818156077)) ;
#54567=CARTESIAN_POINT('Ctrl Pts',(180.546223913397,537.243017267462,-48.072032685545)) ;
#54568=CARTESIAN_POINT('Ctrl Pts',(180.494417541183,537.2631218576,-48.0681237287464)) ;
#54569=CARTESIAN_POINT('Ctrl Pts',(180.489575379792,537.265000963701,-48.0677583721526)) ;
#54570=CARTESIAN_POINT('Ctrl Pts',(180.484723748153,537.266857373542,-48.067392492913)) ;
#54571=CARTESIAN_POINT('Ctrl Pts',(180.479862901525,537.26869099806,-48.0670261425728)) ;
#54572=CARTESIAN_POINT('Ctrl Pts',(180.42228599186,537.290410348894,-48.0626867091243)) ;
#54573=CARTESIAN_POINT('Ctrl Pts',(180.363410209124,537.308931948238,-48.0582818477462)) ;
#54574=CARTESIAN_POINT('Ctrl Pts',(180.303628548833,537.324147931288,-48.0538830980338)) ;
#54575=CARTESIAN_POINT('Ctrl Pts',(180.244746808968,537.339134861248,-48.0495505646944)) ;
#54576=CARTESIAN_POINT('Ctrl Pts',(180.184986275206,537.350915397909,-48.0452242453842)) ;
#54577=CARTESIAN_POINT('Ctrl Pts',(180.124724061371,537.35942557223,-48.0409519905051)) ;
#54578=CARTESIAN_POINT('Ctrl Pts',(180.064498653858,537.367930548796,-48.036682344989)) ;
#54579=CARTESIAN_POINT('Ctrl Pts',(180.003772167374,537.373169285969,-48.032466833336)) ;
#54580=CARTESIAN_POINT('Ctrl Pts',(179.942922703367,537.375113182866,-48.0283294649578)) ;
#54581=CARTESIAN_POINT('Ctrl Pts',(179.882087705436,537.377056617629,-48.0241930801788)) ;
#54582=CARTESIAN_POINT('Ctrl Pts',(179.821129808884,537.375706748115,-48.0201348046835)) ;
#54583=CARTESIAN_POINT('Ctrl Pts',(179.760428479388,537.37106954864,-48.0161538758092)) ;
#54584=CARTESIAN_POINT('Ctrl Pts',(179.69802854173,537.366302586194,-48.0120615484148)) ;
#54585=CARTESIAN_POINT('Ctrl Pts',(179.63589979852,537.358061384484,-48.0080509496658)) ;
#54586=CARTESIAN_POINT('Ctrl Pts',(179.574455561883,537.346392103887,-48.0040949077139)) ;
#54587=CARTESIAN_POINT('Ctrl Pts',(179.514606435191,537.33502576115,-48.0002415657419)) ;
#54588=CARTESIAN_POINT('Ctrl Pts',(179.45540687377,537.320406891227,-47.9964396179116)) ;
#54589=CARTESIAN_POINT('Ctrl Pts',(179.397238341075,537.302618303786,-47.9926424434774)) ;
#54590=CARTESIAN_POINT('Ctrl Pts',(179.336744330713,537.284118559282,-47.9886934645547)) ;
#54591=CARTESIAN_POINT('Ctrl Pts',(179.277365778676,537.262189767387,-47.9847492329119)) ;
#54592=CARTESIAN_POINT('Ctrl Pts',(179.219527711406,537.236976879441,-47.9807392359889)) ;
#54593=CARTESIAN_POINT('Ctrl Pts',(179.169458944596,537.215150800756,-47.9772678959127)) ;
#54594=CARTESIAN_POINT('Ctrl Pts',(179.120543672459,537.190863429084,-47.9737466152818)) ;
#54595=CARTESIAN_POINT('Ctrl Pts',(179.073054148742,537.164247975577,-47.9701245983729)) ;
#54596=CARTESIAN_POINT('Ctrl Pts',(179.06571208263,537.160133122364,-47.969564620392)) ;
#54597=CARTESIAN_POINT('Ctrl Pts',(179.058403995181,537.155962638946,-47.9690022345754)) ;
#54598=CARTESIAN_POINT('Ctrl Pts',(179.051130781925,537.151737032616,-47.9684372532125)) ;
#54599=CARTESIAN_POINT('Ctrl Pts',(179.051104028684,537.151721489462,-47.9684351750275)) ;
#54600=CARTESIAN_POINT('Ctrl Pts',(179.051077275914,537.151705945563,-47.9684330968074)) ;
#54601=CARTESIAN_POINT('Ctrl Pts',(179.051050523616,537.151690400919,-47.9684310185521)) ;
#54602=CARTESIAN_POINT('Ctrl Pts',(179.003049114866,537.123798784166,-47.9647020237161)) ;
#54603=CARTESIAN_POINT('Ctrl Pts',(178.956398910279,537.093398984338,-47.9608501385307)) ;
#54604=CARTESIAN_POINT('Ctrl Pts',(178.911352196445,537.060669048607,-47.9569384696096)) ;
#54605=CARTESIAN_POINT('Ctrl Pts',(178.907144485097,537.057611819561,-47.9565730894896)) ;
#54606=CARTESIAN_POINT('Ctrl Pts',(178.90295077754,537.054534295181,-47.9562071877562)) ;
#54607=CARTESIAN_POINT('Ctrl Pts',(178.89877128705,537.051436642416,-47.9558408158403)) ;
#54608=CARTESIAN_POINT('Ctrl Pts',(178.849353911677,537.014810678108,-47.9515089149689)) ;
#54609=CARTESIAN_POINT('Ctrl Pts',(178.801921587587,536.97536529003,-47.9471119423943)) ;
#54610=CARTESIAN_POINT('Ctrl Pts',(178.756776446934,536.933371843567,-47.9427208450714)) ;
#54611=CARTESIAN_POINT('Ctrl Pts',(178.712204331618,536.891911418122,-47.9383854837588)) ;
#54612=CARTESIAN_POINT('Ctrl Pts',(178.669861345495,536.847967454211,-47.9340561419435)) ;
#54613=CARTESIAN_POINT('Ctrl Pts',(178.630006233896,536.80182351969,-47.9297805484483)) ;
#54614=CARTESIAN_POINT('Ctrl Pts',(178.590175393923,536.755707686666,-47.9255075587749)) ;
#54615=CARTESIAN_POINT('Ctrl Pts',(178.552829281113,536.707394618948,-47.921288386993)) ;
#54616=CARTESIAN_POINT('Ctrl Pts',(178.518197433363,536.657187817612,-47.9171468560982)) ;
#54617=CARTESIAN_POINT('Ctrl Pts',(178.483573895665,536.6069930636,-47.9130063189804)) ;
#54618=CARTESIAN_POINT('Ctrl Pts',(178.451663355893,536.554905480944,-47.9089433872833)) ;
#54619=CARTESIAN_POINT('Ctrl Pts',(178.422667046997,536.501248446199,-47.9049570602619)) ;
#54620=CARTESIAN_POINT('Ctrl Pts',(178.392982608062,536.446318041885,-47.9008761311524)) ;
#54621=CARTESIAN_POINT('Ctrl Pts',(178.366352670331,536.389742684962,-47.8968754586295)) ;
#54622=CARTESIAN_POINT('Ctrl Pts',(178.342960883909,536.331891489663,-47.8929279781005)) ;
#54623=CARTESIAN_POINT('Ctrl Pts',(178.32008248051,536.275309963171,-47.889067133515)) ;
#54624=CARTESIAN_POINT('Ctrl Pts',(178.3003018577,536.217508013867,-47.8852568180468)) ;
#54625=CARTESIAN_POINT('Ctrl Pts',(178.28375689859,536.158852427536,-47.8814502632968)) ;
#54626=CARTESIAN_POINT('Ctrl Pts',(178.266655045212,536.098222526278,-47.8775155819976)) ;
#54627=CARTESIAN_POINT('Ctrl Pts',(178.253011166435,536.036680420503,-47.8735844888598)) ;
#54628=CARTESIAN_POINT('Ctrl Pts',(178.24293271949,535.97465557031,-47.8695877180918)) ;
#54629=CARTESIAN_POINT('Ctrl Pts',(178.23416107659,535.920673062912,-47.8661091815555)) ;
#54630=CARTESIAN_POINT('Ctrl Pts',(178.228089925971,535.866324024968,-47.8625802460645)) ;
#54631=CARTESIAN_POINT('Ctrl Pts',(178.22475542632,535.811909811167,-47.8589503194738)) ;
#54632=CARTESIAN_POINT('Ctrl Pts',(178.224260699275,535.803836581001,-47.8584117610567)) ;
#54633=CARTESIAN_POINT('Ctrl Pts',(178.223826149891,535.795761846863,-47.85787097957)) ;
#54634=CARTESIAN_POINT('Ctrl Pts',(178.223451832322,535.78768651858,-47.8573278097841)) ;
#54635=CARTESIAN_POINT('Ctrl Pts',(178.223450282402,535.787653081413,-47.8573255607042)) ;
#54636=CARTESIAN_POINT('Ctrl Pts',(178.223448733513,535.787619644236,-47.8573233115834)) ;
#54637=CARTESIAN_POINT('Ctrl Pts',(178.223447185658,535.787586207049,-47.8573210624215)) ;
#54638=CARTESIAN_POINT('Ctrl Pts',(178.220879007096,535.732107729501,-47.8535892869709)) ;
#54639=CARTESIAN_POINT('Ctrl Pts',(178.221152741422,535.676404466823,-47.8497351147999)) ;
#54640=CARTESIAN_POINT('Ctrl Pts',(178.224255523442,535.620785841418,-47.845822019635)) ;
#54641=CARTESIAN_POINT('Ctrl Pts',(178.224537666018,535.615728321373,-47.845466193559)) ;
#54642=CARTESIAN_POINT('Ctrl Pts',(178.224843180112,535.610671529998,-47.8451098802692)) ;
#54643=CARTESIAN_POINT('Ctrl Pts',(178.225172043119,535.605615716879,-47.8447531274907)) ;
#54644=CARTESIAN_POINT('Ctrl Pts',(178.2291660325,535.544213663552,-47.8404204212343)) ;
#54645=CARTESIAN_POINT('Ctrl Pts',(178.236607089779,535.482950827978,-47.8360235538722)) ;
#54646=CARTESIAN_POINT('Ctrl Pts',(178.247430894952,535.422229322234,-47.83163354596)) ;
#54647=CARTESIAN_POINT('Ctrl Pts',(178.258094469473,535.362406709838,-47.8273085257134)) ;
#54648=CARTESIAN_POINT('Ctrl Pts',(178.272040970573,535.303109346939,-47.822990442542)) ;
#54649=CARTESIAN_POINT('Ctrl Pts',(178.2891727465,535.244707116931,-47.8187264598205)) ;
#54650=CARTESIAN_POINT('Ctrl Pts',(178.306294572705,535.186338805529,-47.8144649535173)) ;
#54651=CARTESIAN_POINT('Ctrl Pts',(178.326597866137,535.128864524065,-47.810257616129)) ;
#54652=CARTESIAN_POINT('Ctrl Pts',(178.349952392273,535.072640536659,-47.8061276057299)) ;
#54653=CARTESIAN_POINT('Ctrl Pts',(178.373302070798,535.016428219455,-47.8019984525815)) ;
#54654=CARTESIAN_POINT('Ctrl Pts',(178.399701738795,534.961465708792,-47.7979465940857)) ;
#54655=CARTESIAN_POINT('Ctrl Pts',(178.42898908063,534.90809631272,-47.7939703036623)) ;
#54656=CARTESIAN_POINT('Ctrl Pts',(178.459080288826,534.853262056423,-47.7898848737299)) ;
#54657=CARTESIAN_POINT('Ctrl Pts',(178.492220164428,534.800109776089,-47.7858792034445)) ;
#54658=CARTESIAN_POINT('Ctrl Pts',(178.528196051012,534.74899651985,-47.7819250587245)) ;
#54659=CARTESIAN_POINT('Ctrl Pts',(178.563258858755,534.699180533454,-47.7780712713889)) ;
#54660=CARTESIAN_POINT('Ctrl Pts',(178.601015614503,534.651301563366,-47.774266056544)) ;
#54661=CARTESIAN_POINT('Ctrl Pts',(178.641232903684,534.605673160823,-47.7704617801808)) ;
#54662=CARTESIAN_POINT('Ctrl Pts',(178.683021154726,534.558262428303,-47.7665089017314)) ;
#54663=CARTESIAN_POINT('Ctrl Pts',(178.727466530178,534.513282175998,-47.7625566076072)) ;
#54664=CARTESIAN_POINT('Ctrl Pts',(178.774261469017,534.471059114624,-47.7585335895023)) ;
#54665=CARTESIAN_POINT('Ctrl Pts',(178.814651902175,534.434614837092,-47.7550611745812)) ;
#54666=CARTESIAN_POINT('Ctrl Pts',(178.856793369279,534.400223905242,-47.7515354072975)) ;
#54667=CARTESIAN_POINT('Ctrl Pts',(178.900453967763,534.368077307673,-47.7479056720436)) ;
#54668=CARTESIAN_POINT('Ctrl Pts',(178.907348500323,534.36300097406,-47.7473324932792)) ;
#54669=CARTESIAN_POINT('Ctrl Pts',(178.914280941161,534.35798050338,-47.7467567219486)) ;
#54670=CARTESIAN_POINT('Ctrl Pts',(178.921250410667,534.353016533284,-47.7461781587414)) ;
#54671=CARTESIAN_POINT('Ctrl Pts',(178.92127922712,534.352996008908,-47.7461757665738)) ;
#54672=CARTESIAN_POINT('Ctrl Pts',(178.921308044206,534.352975485499,-47.7461733743585)) ;
#54673=CARTESIAN_POINT('Ctrl Pts',(178.921336861924,534.352954963055,-47.7461709820954)) ;
#54674=CARTESIAN_POINT('Ctrl Pts',(178.966123819551,534.321060078073,-47.742453054699)) ;
#54675=CARTESIAN_POINT('Ctrl Pts',(179.012612734901,534.291385373579,-47.7386095408294)) ;
#54676=CARTESIAN_POINT('Ctrl Pts',(179.06054367861,534.264085405347,-47.7347032488684)) ;
#54677=CARTESIAN_POINT('Ctrl Pts',(179.065219895963,534.261421978022,-47.7343221449544)) ;
#54678=CARTESIAN_POINT('Ctrl Pts',(179.069909798089,534.258781150969,-47.7339404435024)) ;
#54679=CARTESIAN_POINT('Ctrl Pts',(179.074613117271,534.256163065068,-47.7335582028372)) ;
#54680=CARTESIAN_POINT('Ctrl Pts',(179.128372717476,534.226237974742,-47.7291891382377)) ;
#54681=CARTESIAN_POINT('Ctrl Pts',(179.183891378524,534.19928405756,-47.7247503225493)) ;
#54682=CARTESIAN_POINT('Ctrl Pts',(179.240794700056,534.175467057658,-47.7203150457455)) ;
#54683=CARTESIAN_POINT('Ctrl Pts',(179.296641211464,534.152092387762,-47.7159621410302)) ;
#54684=CARTESIAN_POINT('Ctrl Pts',(179.353821335501,534.131738726617,-47.7116129293004)) ;
#54685=CARTESIAN_POINT('Ctrl Pts',(179.411973747117,534.114524071162,-47.7073164593425)) ;
#54686=CARTESIAN_POINT('Ctrl Pts',(179.470089277145,534.097320333635,-47.703022714304)) ;
#54687=CARTESIAN_POINT('Ctrl Pts',(179.529175848197,534.08325148744,-47.6987817869211)) ;
#54688=CARTESIAN_POINT('Ctrl Pts',(179.588866018623,534.072400576345,-47.6946190627617)) ;
#54689=CARTESIAN_POINT('Ctrl Pts',(179.648541017051,534.061552423325,-47.6904573966799)) ;
#54690=CARTESIAN_POINT('Ctrl Pts',(179.708819285398,534.053920596761,-47.6863739046806)) ;
#54691=CARTESIAN_POINT('Ctrl Pts',(179.769327101651,534.049554107817,-47.6823692729947)) ;
#54692=CARTESIAN_POINT('Ctrl Pts',(179.831917325208,534.045037343932,-47.6782268198705)) ;
#54693=CARTESIAN_POINT('Ctrl Pts',(179.894753151485,534.044014940913,-47.6741687791312)) ;
#54694=CARTESIAN_POINT('Ctrl Pts',(179.957414141148,534.046501295686,-47.6701689286977)) ;
#54695=CARTESIAN_POINT('Ctrl Pts',(180.018069251131,534.04890805822,-47.6662971199493)) ;
#54696=CARTESIAN_POINT('Ctrl Pts',(180.078560412276,534.054602622417,-47.6624794560378)) ;
#54697=CARTESIAN_POINT('Ctrl Pts',(180.138501190525,534.063558395427,-47.6586703531882)) ;
#54698=CARTESIAN_POINT('Ctrl Pts',(180.2014153536,534.072958422923,-47.6546722983607)) ;
#54699=CARTESIAN_POINT('Ctrl Pts',(180.263722955934,534.085952177943,-47.650683299333)) ;
#54700=CARTESIAN_POINT('Ctrl Pts',(180.324973840245,534.102455945175,-47.6466314574514)) ;
#54701=CARTESIAN_POINT('Ctrl Pts',(180.377779147805,534.116684090849,-47.643138303693)) ;
#54702=CARTESIAN_POINT('Ctrl Pts',(180.429800058266,534.133521136602,-47.6395977799359)) ;
#54703=CARTESIAN_POINT('Ctrl Pts',(180.4807458833,534.152873691095,-47.6359581034402)) ;
#54704=CARTESIAN_POINT('Ctrl Pts',(180.488876769537,534.155962333174,-47.6353772158894)) ;
#54705=CARTESIAN_POINT('Ctrl Pts',(180.496980374762,534.159115018295,-47.6347938027461)) ;
#54706=CARTESIAN_POINT('Ctrl Pts',(180.505055636178,534.162331334421,-47.6342076535002)) ;
#54707=CARTESIAN_POINT('Ctrl Pts',(180.50507280645,534.162338173211,-47.6342064071824)) ;
#54708=CARTESIAN_POINT('Ctrl Pts',(180.505089976594,534.16234501229,-47.6342051608523)) ;
#54709=CARTESIAN_POINT('Ctrl Pts',(180.505107146609,534.162351851656,-47.6342039145097)) ;
#54710=CARTESIAN_POINT('Ctrl Pts',(180.55732647196,534.183152477957,-47.6304134015972)) ;
#54711=CARTESIAN_POINT('Ctrl Pts',(180.608540633887,534.206694341041,-47.6264985681328)) ;
#54712=CARTESIAN_POINT('Ctrl Pts',(180.658470286984,534.232834549517,-47.622521772505)) ;
#54713=CARTESIAN_POINT('Ctrl Pts',(180.663485422641,534.235460177445,-47.622122327119)) ;
#54714=CARTESIAN_POINT('Ctrl Pts',(180.668487577824,534.238111982171,-47.6217222565965)) ;
#54715=CARTESIAN_POINT('Ctrl Pts',(180.673476456043,534.240789793202,-47.6213216241303)) ;
#54716=CARTESIAN_POINT('Ctrl Pts',(180.728017873916,534.270065234301,-47.6169416689989)) ;
#54717=CARTESIAN_POINT('Ctrl Pts',(180.780975776105,534.302453959571,-47.6124951845948)) ;
#54718=CARTESIAN_POINT('Ctrl Pts',(180.832012241287,534.337731455741,-47.6080513472692)) ;
#54719=CARTESIAN_POINT('Ctrl Pts',(180.882985559462,534.37296530335,-47.6036130082677)) ;
#54720=CARTESIAN_POINT('Ctrl Pts',(180.932042496935,534.411080550936,-47.5991776497722)) ;
#54721=CARTESIAN_POINT('Ctrl Pts',(180.978874654322,534.451827037993,-47.5947936045321)) ;
#54722=CARTESIAN_POINT('Ctrl Pts',(181.025663601896,534.492535930195,-47.590413604243)) ;
#54723=CARTESIAN_POINT('Ctrl Pts',(181.070232013022,534.53587116621,-47.5860849587363)) ;
#54724=CARTESIAN_POINT('Ctrl Pts',(181.112297226174,534.581558727159,-47.5818318158203)) ;
#54725=CARTESIAN_POINT('Ctrl Pts',(181.154336851441,534.627218496782,-47.5775812600521)) ;
#54726=CARTESIAN_POINT('Ctrl Pts',(181.193876301892,534.675227782712,-47.5734061078654)) ;
#54727=CARTESIAN_POINT('Ctrl Pts',(181.230657426143,534.725288401908,-47.5693054982439)) ;
#54728=CARTESIAN_POINT('Ctrl Pts',(181.267442042625,534.775353774174,-47.5652044992848)) ;
#54729=CARTESIAN_POINT('Ctrl Pts',(181.301467634746,534.827470979894,-47.561177922665)) ;
#54730=CARTESIAN_POINT('Ctrl Pts',(181.332501452985,534.881315826386,-47.5572009793439)) ;
#54731=CARTESIAN_POINT('Ctrl Pts',(181.363534173554,534.935158768377,-47.5532241766878)) ;
#54732=CARTESIAN_POINT('Ctrl Pts',(181.391574986876,534.990729367568,-47.5492967112841)) ;
#54733=CARTESIAN_POINT('Ctrl Pts',(181.416420496784,535.04767563909,-47.545373030922)) ;
#54734=CARTESIAN_POINT('Ctrl Pts',(181.441290859478,535.104678873562,-47.5414454257303)) ;
#54735=CARTESIAN_POINT('Ctrl Pts',(181.46295894898,535.16306063624,-47.537521109075)) ;
#54736=CARTESIAN_POINT('Ctrl Pts',(181.48125699761,535.222438078838,-47.5335394975804)) ;
#54737=CARTESIAN_POINT('Ctrl Pts',(181.49837261429,535.277978511998,-47.5298151804424)) ;
#54738=CARTESIAN_POINT('Ctrl Pts',(181.512539443077,535.334389744362,-47.5260400792227)) ;
#54739=CARTESIAN_POINT('Ctrl Pts',(181.523656952658,535.391334705907,-47.5221601717599)) ;
#54740=CARTESIAN_POINT('Origin',(179.888527625407,535.710565160536,-47.5221601717598)) ;
#54741=CARTESIAN_POINT('Ctrl Pts',(181.451956078709,536.28610618549,-48.355715363061)) ;
#54742=CARTESIAN_POINT('Ctrl Pts',(181.443432156306,536.309260995037,-48.3540745386352)) ;
#54743=CARTESIAN_POINT('Ctrl Pts',(181.434394207593,536.332225451491,-48.3524165071428)) ;
#54744=CARTESIAN_POINT('Ctrl Pts',(181.397471519135,536.420250845626,-48.3459354847706)) ;
#54745=CARTESIAN_POINT('Ctrl Pts',(181.365967014669,536.483698917522,-48.340990223511)) ;
#54746=CARTESIAN_POINT('Ctrl Pts',(181.277601068931,536.636415683579,-48.3283947666615)) ;
#54747=CARTESIAN_POINT('Ctrl Pts',(181.216091736306,536.722639766728,-48.3206303658353)) ;
#54748=CARTESIAN_POINT('Ctrl Pts',(181.110468882847,536.844361891796,-48.3089844490963)) ;
#54749=CARTESIAN_POINT('Ctrl Pts',(181.072023854145,536.884436283982,-48.3050211410803)) ;
#54750=CARTESIAN_POINT('Ctrl Pts',(181.009770460592,536.943153818467,-48.2990986957174)) ;
#54751=CARTESIAN_POINT('Ctrl Pts',(180.987338099798,536.96319295314,-48.2970563376968)) ;
#54752=CARTESIAN_POINT('Ctrl Pts',(180.931618933764,537.010317618914,-48.2922127808431)) ;
#54753=CARTESIAN_POINT('Ctrl Pts',(180.897806379057,537.036745051117,-48.2894535663643)) ;
#54754=CARTESIAN_POINT('Ctrl Pts',(180.812623574893,537.098175148572,-48.2828255190749)) ;
#54755=CARTESIAN_POINT('Ctrl Pts',(180.760243077164,537.131666138784,-48.279017615289)) ;
#54756=CARTESIAN_POINT('Ctrl Pts',(180.601878725853,537.22086220908,-48.267912086069)) ;
#54757=CARTESIAN_POINT('Ctrl Pts',(180.491638210104,537.26816620639,-48.2606540385479)) ;
#54758=CARTESIAN_POINT('Ctrl Pts',(180.327909616524,537.318410706314,-48.249666551006)) ;
#54759=CARTESIAN_POINT('Ctrl Pts',(180.277858489177,537.331257710468,-48.2462865682751)) ;
#54760=CARTESIAN_POINT('Ctrl Pts',(180.171017288128,537.353446611314,-48.2389785635886)) ;
#54761=CARTESIAN_POINT('Ctrl Pts',(180.114178534133,537.362212861074,-48.235036363122)) ;
#54762=CARTESIAN_POINT('Ctrl Pts',(179.989684828334,537.374867477988,-48.22626691009)) ;
#54763=CARTESIAN_POINT('Ctrl Pts',(179.922015858998,537.377602005444,-48.2214138178156)) ;
#54764=CARTESIAN_POINT('Ctrl Pts',(179.738003164606,537.373828916416,-48.2080684094743)) ;
#54765=CARTESIAN_POINT('Ctrl Pts',(179.622197594573,537.35925410166,-48.1994914040934)) ;
#54766=CARTESIAN_POINT('Ctrl Pts',(179.47801536914,537.325507483639,-48.1891652565625)) ;
#54767=CARTESIAN_POINT('Ctrl Pts',(179.447385903466,537.317411024265,-48.1869948434875)) ;
#54768=CARTESIAN_POINT('Ctrl Pts',(179.381212312762,537.297883505801,-48.1823811388451)) ;
#54769=CARTESIAN_POINT('Ctrl Pts',(179.345785026416,537.286122010407,-48.1799554593728)) ;
#54770=CARTESIAN_POINT('Ctrl Pts',(179.210892862924,537.236248070254,-48.1707838500216)) ;
#54771=CARTESIAN_POINT('Ctrl Pts',(179.114767732667,537.189820857744,-48.1643734454356)) ;
#54772=CARTESIAN_POINT('Ctrl Pts',(178.945854579752,537.087236531047,-48.1522819882884)) ;
#54773=CARTESIAN_POINT('Ctrl Pts',(178.872003144414,537.033641731672,-48.1466503524933)) ;
#54774=CARTESIAN_POINT('Ctrl Pts',(178.764691293621,536.941453526979,-48.1375388800779)) ;
#54775=CARTESIAN_POINT('Ctrl Pts',(178.727988158534,536.906910220609,-48.1342295303475)) ;
#54776=CARTESIAN_POINT('Ctrl Pts',(178.651403205098,536.827986955213,-48.126841609869)) ;
#54777=CARTESIAN_POINT('Ctrl Pts',(178.612227588258,536.783022596584,-48.1227379148407)) ;
#54778=CARTESIAN_POINT('Ctrl Pts',(178.530771423917,536.678731357091,-48.1134273767143)) ;
#54779=CARTESIAN_POINT('Ctrl Pts',(178.489801511131,536.618535994306,-48.1081852650483)) ;
#54780=CARTESIAN_POINT('Ctrl Pts',(178.398398515099,536.463299758907,-48.0950919426553)) ;
#54781=CARTESIAN_POINT('Ctrl Pts',(178.352973573254,536.365676904987,-48.0872091251478)) ;
#54782=CARTESIAN_POINT('Ctrl Pts',(178.306927373818,536.235029980686,-48.0775709980731)) ;
#54783=CARTESIAN_POINT('Ctrl Pts',(178.297413708337,536.205418509373,-48.0754457259631)) ;
#54784=CARTESIAN_POINT('Ctrl Pts',(178.277924050782,536.138364102538,-48.070786331965)) ;
#54785=CARTESIAN_POINT('Ctrl Pts',(178.268413962295,536.100806289195,-48.0682761758745)) ;
#54786=CARTESIAN_POINT('Ctrl Pts',(178.249199603956,536.012019559273,-48.0624999914387)) ;
#54787=CARTESIAN_POINT('Ctrl Pts',(178.240572828918,535.960598908355,-48.0592750798041)) ;
#54788=CARTESIAN_POINT('Ctrl Pts',(178.217961590007,535.771973432546,-48.0476173435945)) ;
#54789=CARTESIAN_POINT('Ctrl Pts',(178.218606939032,535.633597647715,-48.0393438108748)) ;
#54790=CARTESIAN_POINT('Ctrl Pts',(178.242911202225,535.445670148723,-48.0271864231066)) ;
#54791=CARTESIAN_POINT('Ctrl Pts',(178.25191156015,535.394796788973,-48.0238069394469)) ;
#54792=CARTESIAN_POINT('Ctrl Pts',(178.275908015491,535.2882775437,-48.0164941350027)) ;
#54793=CARTESIAN_POINT('Ctrl Pts',(178.291457127882,535.232827525934,-48.0125463568321)) ;
#54794=CARTESIAN_POINT('Ctrl Pts',(178.331518686863,535.11400625026,-48.003758415065)) ;
#54795=CARTESIAN_POINT('Ctrl Pts',(178.357100364966,535.051104601854,-47.9988921172518)) ;
#54796=CARTESIAN_POINT('Ctrl Pts',(178.436497274949,534.885607409271,-47.98558304811)) ;
#54797=CARTESIAN_POINT('Ctrl Pts',(178.497288605296,534.786766271574,-47.9770589579872)) ;
#54798=CARTESIAN_POINT('Ctrl Pts',(178.58719448683,534.669845926503,-47.9667729997946)) ;
#54799=CARTESIAN_POINT('Ctrl Pts',(178.607270803379,534.645226693984,-47.9645964878086)) ;
#54800=CARTESIAN_POINT('Ctrl Pts',(178.652452763857,534.592947794466,-47.959975568195)) ;
#54801=CARTESIAN_POINT('Ctrl Pts',(178.677808222789,534.565528598271,-47.9575485695418)) ;
#54802=CARTESIAN_POINT('Ctrl Pts',(178.778991820137,534.463232767556,-47.9483717314691)) ;
#54803=CARTESIAN_POINT('Ctrl Pts',(178.861018567761,534.394838172088,-47.9419572163795)) ;
#54804=CARTESIAN_POINT('Ctrl Pts',(179.024024650514,534.283526679081,-47.9298769232956)) ;
#54805=CARTESIAN_POINT('Ctrl Pts',(179.103078906543,534.23853538757,-47.9242612771831)) ;
#54806=CARTESIAN_POINT('Ctrl Pts',(179.231051320197,534.178959242756,-47.9151685357388)) ;
#54807=CARTESIAN_POINT('Ctrl Pts',(179.27763865699,534.15978937583,-47.9118603686894)) ;
#54808=CARTESIAN_POINT('Ctrl Pts',(179.381121896328,534.1225948745,-47.9044721066949)) ;
#54809=CARTESIAN_POINT('Ctrl Pts',(179.438260077722,534.105458380698,-47.9003667501405)) ;
#54810=CARTESIAN_POINT('Ctrl Pts',(179.566900481831,534.074287106329,-47.8910524971581)) ;
#54811=CARTESIAN_POINT('Ctrl Pts',(179.638652957529,534.061804830488,-47.8858082824234)) ;
#54812=CARTESIAN_POINT('Ctrl Pts',(179.818048512989,534.042577439444,-47.8726917292847)) ;
#54813=CARTESIAN_POINT('Ctrl Pts',(179.925980153421,534.04150818883,-47.8647871073748)) ;
#54814=CARTESIAN_POINT('Ctrl Pts',(180.064207456186,534.053562677191,-47.8551317954482)) ;
#54815=CARTESIAN_POINT('Ctrl Pts',(180.095071346719,534.057126031649,-47.8530085073833)) ;
#54816=CARTESIAN_POINT('Ctrl Pts',(180.163990519883,534.06704360586,-47.8483618997925)) ;
#54817=CARTESIAN_POINT('Ctrl Pts',(180.201959552842,534.073859952344,-47.845862099041)) ;
#54818=CARTESIAN_POINT('Ctrl Pts',(180.290270657586,534.092900518838,-47.8401167796297)) ;
#54819=CARTESIAN_POINT('Ctrl Pts',(180.340347455955,534.106166220435,-47.8369118277216)) ;
#54820=CARTESIAN_POINT('Ctrl Pts',(180.521655255622,534.163360549852,-47.8252443631657)) ;
#54821=CARTESIAN_POINT('Ctrl Pts',(180.647872931375,534.221241593517,-47.8169460691682)) ;
#54822=CARTESIAN_POINT('Ctrl Pts',(180.809134566258,534.321078010433,-47.8047760670396)) ;
#54823=CARTESIAN_POINT('Ctrl Pts',(180.851508281459,534.350102379805,-47.8014159854988)) ;
#54824=CARTESIAN_POINT('Ctrl Pts',(180.938019581324,534.415428008747,-47.794154959863)) ;
#54825=CARTESIAN_POINT('Ctrl Pts',(180.981764910245,534.452135800576,-47.7902400724785)) ;
#54826=CARTESIAN_POINT('Ctrl Pts',(181.0725322574,534.536610784876,-47.7815491110741)) ;
#54827=CARTESIAN_POINT('Ctrl Pts',(181.118730538064,534.585116370418,-47.7767480572676)) ;
#54828=CARTESIAN_POINT('Ctrl Pts',(181.238930878224,534.72758825234,-47.7632241204118)) ;
#54829=CARTESIAN_POINT('Ctrl Pts',(181.305934200094,534.826939569601,-47.7544008821308)) ;
#54830=CARTESIAN_POINT('Ctrl Pts',(181.376393862534,534.960368147172,-47.7438801866571)) ;
#54831=CARTESIAN_POINT('Ctrl Pts',(181.39026751837,534.988540619103,-47.7417297780651)) ;
#54832=CARTESIAN_POINT('Ctrl Pts',(181.419293528156,535.051944717249,-47.7370674276954)) ;
#54833=CARTESIAN_POINT('Ctrl Pts',(181.434042251425,535.087339462612,-47.7345768628677)) ;
#54834=CARTESIAN_POINT('Ctrl Pts',(181.465561336422,535.171002010718,-47.7288768394179)) ;
#54835=CARTESIAN_POINT('Ctrl Pts',(181.48135931127,535.219595024162,-47.7257060408905)) ;
#54836=CARTESIAN_POINT('Ctrl Pts',(181.531985587087,535.403702080352,-47.7139540562249)) ;
#54837=CARTESIAN_POINT('Ctrl Pts',(181.551937472757,535.542684100415,-47.7055471331473)) ;
#54838=CARTESIAN_POINT('Ctrl Pts',(181.555161103611,535.734172452488,-47.6932298419796)) ;
#54839=CARTESIAN_POINT('Ctrl Pts',(181.553627859236,535.785829342167,-47.6898413574438)) ;
#54840=CARTESIAN_POINT('Ctrl Pts',(181.545222177744,535.895982631582,-47.6824263686904)) ;
#54841=CARTESIAN_POINT('Ctrl Pts',(181.537643366721,535.954352460752,-47.6783814140527)) ;
#54842=CARTESIAN_POINT('Ctrl Pts',(181.509825057427,536.105463556812,-47.6675847664843)) ;
#54843=CARTESIAN_POINT('Ctrl Pts',(181.484724091722,536.197086192928,-47.6607031740783)) ;
#54844=CARTESIAN_POINT('Ctrl Pts',(181.451971427951,536.286064488325,-47.6537940777375)) ;
#54845=CARTESIAN_POINT('Origin',(179.888527625407,535.710565160536,-48.5221601717598)) ;
#54846=CARTESIAN_POINT('',(181.45195607237,536.286106202709,-49.0537499395136)) ;
#54847=CARTESIAN_POINT('',(181.451956083891,536.286106171415,-48.8631290382246)) ;
#54848=CARTESIAN_POINT('',(181.451956083813,536.286106171625,-48.5221601717599)) ;
#54849=CARTESIAN_POINT('',(181.555006899063,535.71162572618,-49.0928089386736)) ;
#54850=CARTESIAN_POINT('Ctrl Pts',(181.55452730056,535.711605540458,-49.0925337921257)) ;
#54851=CARTESIAN_POINT('Ctrl Pts',(181.554499745292,535.755730832439,-49.0893446356981)) ;
#54852=CARTESIAN_POINT('Ctrl Pts',(181.552719153091,535.799840895829,-49.0861810648237)) ;
#54853=CARTESIAN_POINT('Ctrl Pts',(181.546820044684,535.873351227504,-49.0809981568373)) ;
#54854=CARTESIAN_POINT('Ctrl Pts',(181.543664179677,535.902805434826,-49.0789457219699)) ;
#54855=CARTESIAN_POINT('Ctrl Pts',(181.535633050346,535.962648202419,-49.0748456738758)) ;
#54856=CARTESIAN_POINT('Ctrl Pts',(181.530698975711,535.993010761211,-49.0728064240962)) ;
#54857=CARTESIAN_POINT('Ctrl Pts',(181.507825788572,536.112724184301,-49.0648825240018)) ;
#54858=CARTESIAN_POINT('Ctrl Pts',(181.483416661406,536.200645086575,-49.0593063227425)) ;
#54859=CARTESIAN_POINT('Ctrl Pts',(181.451956072328,536.286106202824,-49.0537499415271)) ;
#54860=CARTESIAN_POINT('',(178.619456745555,536.789923813584,-49.5221601717597)) ;
#54861=CARTESIAN_POINT('Ctrl Pts',(181.555006899063,535.71162572618,-49.0928089386736)) ;
#54862=CARTESIAN_POINT('Ctrl Pts',(181.554911677155,535.651761101128,-49.0970575997108)) ;
#54863=CARTESIAN_POINT('Ctrl Pts',(181.551563926785,535.591796400194,-49.1013454409477)) ;
#54864=CARTESIAN_POINT('Ctrl Pts',(181.544988530129,535.53210893011,-49.1056125097224)) ;
#54865=CARTESIAN_POINT('Ctrl Pts',(181.538420248955,535.472486050069,-49.1098749609425)) ;
#54866=CARTESIAN_POINT('Ctrl Pts',(181.528631540799,535.413139765124,-49.1141164261649)) ;
#54867=CARTESIAN_POINT('Ctrl Pts',(181.51568414664,535.354437590846,-49.1182974440124)) ;
#54868=CARTESIAN_POINT('Ctrl Pts',(181.502745687373,535.295775926463,-49.1224755765735)) ;
#54869=CARTESIAN_POINT('Ctrl Pts',(181.486652970128,535.237757503309,-49.1265932469502)) ;
#54870=CARTESIAN_POINT('Ctrl Pts',(181.467502284901,535.180740681,-49.1306339744544)) ;
#54871=CARTESIAN_POINT('Ctrl Pts',(181.44835724259,535.123740659193,-49.134673511323)) ;
#54872=CARTESIAN_POINT('Ctrl Pts',(181.426155991489,535.067741741072,-49.1386361730387)) ;
#54873=CARTESIAN_POINT('Ctrl Pts',(181.401029239235,535.013092736096,-49.1425289370527)) ;
#54874=CARTESIAN_POINT('Ctrl Pts',(181.375882194113,534.958399595491,-49.1464248449407)) ;
#54875=CARTESIAN_POINT('Ctrl Pts',(181.347804781064,534.905058723015,-49.1502508800457)) ;
#54876=CARTESIAN_POINT('Ctrl Pts',(181.316963969973,534.853408532587,-49.1540363410482)) ;
#54877=CARTESIAN_POINT('Ctrl Pts',(181.286111640662,534.801739052193,-49.1578232158193)) ;
#54878=CARTESIAN_POINT('Ctrl Pts',(181.252493625534,534.751761799062,-49.1615697761749)) ;
#54879=CARTESIAN_POINT('Ctrl Pts',(181.216315764961,534.703800951296,-49.1653244954319)) ;
#54880=CARTESIAN_POINT('Ctrl Pts',(181.180070812056,534.655751159489,-49.1690861778665)) ;
#54881=CARTESIAN_POINT('Ctrl Pts',(181.141256221114,534.609725731287,-49.1728565400046)) ;
#54882=CARTESIAN_POINT('Ctrl Pts',(181.100121726458,534.566030406421,-49.1766977336409)) ;
#54883=CARTESIAN_POINT('Ctrl Pts',(181.064119275007,534.52778662039,-49.1800596902799)) ;
#54884=CARTESIAN_POINT('Ctrl Pts',(181.026340236735,534.491327817788,-49.1834764342659)) ;
#54885=CARTESIAN_POINT('Ctrl Pts',(180.986981295376,534.456840870487,-49.1869925547289)) ;
#54886=CARTESIAN_POINT('Ctrl Pts',(180.986956119852,534.456818811282,-49.1869948037776)) ;
#54887=CARTESIAN_POINT('Ctrl Pts',(180.986930943682,534.456796752882,-49.1869970528668)) ;
#54888=CARTESIAN_POINT('Ctrl Pts',(180.986905766866,534.456774695288,-49.1869993019968)) ;
#54889=CARTESIAN_POINT('Ctrl Pts',(180.945132179332,534.420176547417,-49.1907310774929)) ;
#54890=CARTESIAN_POINT('Ctrl Pts',(180.901410943968,534.385660145286,-49.19458524967)) ;
#54891=CARTESIAN_POINT('Ctrl Pts',(180.855991998272,534.353408352203,-49.1984983448031)) ;
#54892=CARTESIAN_POINT('Ctrl Pts',(180.851861958098,534.350475628885,-49.1988541707664)) ;
#54893=CARTESIAN_POINT('Ctrl Pts',(180.847717915726,534.347561632462,-49.1992104839429)) ;
#54894=CARTESIAN_POINT('Ctrl Pts',(180.843560080384,534.344666500875,-49.1995672366075)) ;
#54895=CARTESIAN_POINT('Ctrl Pts',(180.79306380925,534.309505572763,-49.2038999428835)) ;
#54896=CARTESIAN_POINT('Ctrl Pts',(180.74052717115,534.277126471809,-49.208296810223)) ;
#54897=CARTESIAN_POINT('Ctrl Pts',(180.686304652853,534.247729623411,-49.2126868180687)) ;
#54898=CARTESIAN_POINT('Ctrl Pts',(180.632884822058,534.218767953672,-49.2170118380729)) ;
#54899=CARTESIAN_POINT('Ctrl Pts',(180.577828776666,534.192700466876,-49.2213299209602)) ;
#54900=CARTESIAN_POINT('Ctrl Pts',(180.521486588017,534.169681434335,-49.2255939033608)) ;
#54901=CARTESIAN_POINT('Ctrl Pts',(180.465177121547,534.14667577069,-49.2298554093435)) ;
#54902=CARTESIAN_POINT('Ctrl Pts',(180.407583023497,534.126714896719,-49.2340627463742)) ;
#54903=CARTESIAN_POINT('Ctrl Pts',(180.349064032254,534.109919118014,-49.2381927563816)) ;
#54904=CARTESIAN_POINT('Ctrl Pts',(180.290557187574,534.093126825545,-49.2423219091387)) ;
#54905=CARTESIAN_POINT('Ctrl Pts',(180.231125843687,534.079498352383,-49.2463737672092)) ;
#54906=CARTESIAN_POINT('Ctrl Pts',(180.171139611766,534.069120844121,-49.2503500571725)) ;
#54907=CARTESIAN_POINT('Ctrl Pts',(180.109506899204,534.058458497724,-49.2544354869207)) ;
#54908=CARTESIAN_POINT('Ctrl Pts',(180.047288395297,534.051228390706,-49.2584411569732)) ;
#54909=CARTESIAN_POINT('Ctrl Pts',(179.984895840698,534.047486877455,-49.2623953014158)) ;
#54910=CARTESIAN_POINT('Ctrl Pts',(179.924086832196,534.043840325193,-49.2662490882108)) ;
#54911=CARTESIAN_POINT('Ctrl Pts',(179.863112594942,534.043507696091,-49.2700543024794)) ;
#54912=CARTESIAN_POINT('Ctrl Pts',(179.802363804755,534.046501995282,-49.2738585782267)) ;
#54913=CARTESIAN_POINT('Ctrl Pts',(179.739242047665,534.049613257672,-49.2778114564466)) ;
#54914=CARTESIAN_POINT('Ctrl Pts',(179.676363826613,534.056317323824,-49.2817637502975)) ;
#54915=CARTESIAN_POINT('Ctrl Pts',(179.614176335598,534.066577433623,-49.2857867681017)) ;
#54916=CARTESIAN_POINT('Ctrl Pts',(179.560500029662,534.075433310964,-49.2892591824236)) ;
#54917=CARTESIAN_POINT('Ctrl Pts',(179.507337342244,534.086938441788,-49.2927849490772)) ;
#54918=CARTESIAN_POINT('Ctrl Pts',(179.45498218312,534.101030596804,-49.2964146836658)) ;
#54919=CARTESIAN_POINT('Ctrl Pts',(179.446714668846,534.103255918906,-49.2969878627569)) ;
#54920=CARTESIAN_POINT('Ctrl Pts',(179.438467194578,534.105545708956,-49.2975636344171)) ;
#54921=CARTESIAN_POINT('Ctrl Pts',(179.430240807281,534.107899676818,-49.2981421979574)) ;
#54922=CARTESIAN_POINT('Ctrl Pts',(179.430206794206,534.107909409606,-49.2981445901041)) ;
#54923=CARTESIAN_POINT('Ctrl Pts',(179.430172781491,534.107919143492,-49.2981469822985)) ;
#54924=CARTESIAN_POINT('Ctrl Pts',(179.430138769138,534.107928878474,-49.2981493745406)) ;
#54925=CARTESIAN_POINT('Ctrl Pts',(179.377278132391,534.123058597679,-49.301867301362)) ;
#54926=CARTESIAN_POINT('Ctrl Pts',(179.325092149455,534.140903220938,-49.3057108146284)) ;
#54927=CARTESIAN_POINT('Ctrl Pts',(179.273863720226,534.161355891207,-49.3096171059527)) ;
#54928=CARTESIAN_POINT('Ctrl Pts',(179.26886579857,534.163351284101,-49.3099982095371)) ;
#54929=CARTESIAN_POINT('Ctrl Pts',(179.263877014189,534.165371467186,-49.3103799106584)) ;
#54930=CARTESIAN_POINT('Ctrl Pts',(179.258897644146,534.16741631899,-49.3107621509917)) ;
#54931=CARTESIAN_POINT('Ctrl Pts',(179.201982702947,534.19078927966,-49.3151312149316)) ;
#54932=CARTESIAN_POINT('Ctrl Pts',(179.14629396211,534.217390025738,-49.3195700299251)) ;
#54933=CARTESIAN_POINT('Ctrl Pts',(179.092194440457,534.247029178958,-49.3240053059955)) ;
#54934=CARTESIAN_POINT('Ctrl Pts',(179.039099660485,534.276117870886,-49.3283582096791)) ;
#54935=CARTESIAN_POINT('Ctrl Pts',(178.987535306352,534.308132790928,-49.3327074203407)) ;
#54936=CARTESIAN_POINT('Ctrl Pts',(178.937818914218,534.342865013661,-49.337003889208)) ;
#54937=CARTESIAN_POINT('Ctrl Pts',(178.888134053237,534.377575208508,-49.3412976331668)) ;
#54938=CARTESIAN_POINT('Ctrl Pts',(178.840294714745,534.4149991662,-49.3455385594482)) ;
#54939=CARTESIAN_POINT('Ctrl Pts',(178.794594921043,534.454901386224,-49.3497012824977)) ;
#54940=CARTESIAN_POINT('Ctrl Pts',(178.748906743163,534.494793464034,-49.3538629474801)) ;
#54941=CARTESIAN_POINT('Ctrl Pts',(178.705357057807,534.537162543635,-49.3579464383719)) ;
#54942=CARTESIAN_POINT('Ctrl Pts',(178.664217195255,534.581746995344,-49.3619510689569)) ;
#54943=CARTESIAN_POINT('Ctrl Pts',(178.621661478401,534.627865849061,-49.3660935214277)) ;
#54944=CARTESIAN_POINT('Ctrl Pts',(178.581684632514,534.676355421234,-49.3701515615004)) ;
#54945=CARTESIAN_POINT('Ctrl Pts',(178.544560053224,534.726895975379,-49.374151411281)) ;
#54946=CARTESIAN_POINT('Ctrl Pts',(178.508623895755,534.775818639206,-49.3780232189706)) ;
#54947=CARTESIAN_POINT('Ctrl Pts',(178.475360465389,534.826663033093,-49.3818408818493)) ;
#54948=CARTESIAN_POINT('Ctrl Pts',(178.444989908625,534.879110450356,-49.3856499837092)) ;
#54949=CARTESIAN_POINT('Ctrl Pts',(178.413112803794,534.934159550416,-49.3896480381486)) ;
#54950=CARTESIAN_POINT('Ctrl Pts',(178.384423573488,534.990975074804,-49.3936370368329)) ;
#54951=CARTESIAN_POINT('Ctrl Pts',(178.359137434927,535.049152880559,-49.3976888784728)) ;
#54952=CARTESIAN_POINT('Ctrl Pts',(178.337337879878,535.099308829681,-49.4011820312397)) ;
#54953=CARTESIAN_POINT('Ctrl Pts',(178.318067108084,535.15047813457,-49.4047225540605)) ;
#54954=CARTESIAN_POINT('Ctrl Pts',(178.301433344379,535.202375297453,-49.4083622296786)) ;
#54955=CARTESIAN_POINT('Ctrl Pts',(178.298778613439,535.210658029279,-49.4089431180239)) ;
#54956=CARTESIAN_POINT('Ctrl Pts',(178.296190962998,535.218959362182,-49.4095265319714)) ;
#54957=CARTESIAN_POINT('Ctrl Pts',(178.293670733555,535.22727820833,-49.4101126820322)) ;
#54958=CARTESIAN_POINT('Ctrl Pts',(178.293665374797,535.227295896675,-49.4101139283618)) ;
#54959=CARTESIAN_POINT('Ctrl Pts',(178.293660016343,535.227313585099,-49.4101151747038)) ;
#54960=CARTESIAN_POINT('Ctrl Pts',(178.293654658194,535.227331273602,-49.4101164210582)) ;
#54961=CARTESIAN_POINT('Ctrl Pts',(178.277359028103,535.281126961539,-49.413906933453)) ;
#54962=CARTESIAN_POINT('Ctrl Pts',(178.263833292121,535.335845914037,-49.4178217665055)) ;
#54963=CARTESIAN_POINT('Ctrl Pts',(178.253139902238,535.391180638803,-49.4217985618384)) ;
#54964=CARTESIAN_POINT('Ctrl Pts',(178.25206581324,535.396738690994,-49.4221980078663)) ;
#54965=CARTESIAN_POINT('Ctrl Pts',(178.251020283373,535.402302915627,-49.422598079034)) ;
#54966=CARTESIAN_POINT('Ctrl Pts',(178.2500033642,535.407872974596,-49.4229987121484)) ;
#54967=CARTESIAN_POINT('Ctrl Pts',(178.238885809053,535.468768116883,-49.4273786676646)) ;
#54968=CARTESIAN_POINT('Ctrl Pts',(178.231189624062,535.530366317671,-49.4318251526027)) ;
#54969=CARTESIAN_POINT('Ctrl Pts',(178.226949968159,535.592263397604,-49.4362689905779)) ;
#54970=CARTESIAN_POINT('Ctrl Pts',(178.222715557955,535.65408389268,-49.4407073302212)) ;
#54971=CARTESIAN_POINT('Ctrl Pts',(178.221928761452,535.716202624384,-49.4451426894742)) ;
#54972=CARTESIAN_POINT('Ctrl Pts',(178.224586279133,535.77822250377,-49.4495267355503)) ;
#54973=CARTESIAN_POINT('Ctrl Pts',(178.227241344843,535.840185160232,-49.4539067366662)) ;
#54974=CARTESIAN_POINT('Ctrl Pts',(178.233334251276,535.902049229793,-49.4582353830793)) ;
#54975=CARTESIAN_POINT('Ctrl Pts',(178.2428269984,535.963422870731,-49.4624885269454)) ;
#54976=CARTESIAN_POINT('Ctrl Pts',(178.252313971153,536.024759178508,-49.4667390836535)) ;
#54977=CARTESIAN_POINT('Ctrl Pts',(178.265196703797,536.085605670115,-49.4709142368251)) ;
#54978=CARTESIAN_POINT('Ctrl Pts',(178.281403022177,536.145574600527,-49.4750148474439)) ;
#54979=CARTESIAN_POINT('Ctrl Pts',(178.297610879212,536.20554922449,-49.4791158473816)) ;
#54980=CARTESIAN_POINT('Ctrl Pts',(178.31714314831,536.264646053285,-49.4831424249934)) ;
#54981=CARTESIAN_POINT('Ctrl Pts',(178.339891482358,536.322480985118,-49.4871193692917)) ;
#54982=CARTESIAN_POINT('Ctrl Pts',(178.362639011737,536.380313871178,-49.4910961729149)) ;
#54983=CARTESIAN_POINT('Ctrl Pts',(178.388602702046,536.436884766255,-49.4950236392707)) ;
#54984=CARTESIAN_POINT('Ctrl Pts',(178.417634175849,536.491815189789,-49.4989473205462)) ;
#54985=CARTESIAN_POINT('Ctrl Pts',(178.446694689467,536.546800559527,-49.5028749266301)) ;
#54986=CARTESIAN_POINT('Ctrl Pts',(178.478829564945,536.600141789156,-49.5067992441383)) ;
#54987=CARTESIAN_POINT('Ctrl Pts',(178.513844080861,536.651469010558,-49.5107808564248)) ;
#54988=CARTESIAN_POINT('Ctrl Pts',(178.546595900434,536.699479381415,-49.514505170293)) ;
#54989=CARTESIAN_POINT('Ctrl Pts',(178.581867072349,536.745727234891,-49.5182802680799)) ;
#54990=CARTESIAN_POINT('Ctrl Pts',(178.619456745554,536.789923813584,-49.5221601717597)) ;
#54991=CARTESIAN_POINT('',(181.142801535895,536.808437501682,-49.5221525827187)) ;
#54992=CARTESIAN_POINT('Origin',(179.888527625407,535.710565160536,-49.5221601717598)) ;
#54993=CARTESIAN_POINT('',(181.55405613246,535.711433585225,-48.8998644770965)) ;
#54994=CARTESIAN_POINT('Ctrl Pts',(181.142801548039,536.808437512311,-49.5221525825813)) ;
#54995=CARTESIAN_POINT('Ctrl Pts',(181.108069436076,536.848071008662,-49.5185546904077)) ;
#54996=CARTESIAN_POINT('Ctrl Pts',(181.071355132789,536.886086906054,-49.5148601919674)) ;
#54997=CARTESIAN_POINT('Ctrl Pts',(181.032850332806,536.92229732986,-49.5111228902725)) ;
#54998=CARTESIAN_POINT('Ctrl Pts',(180.988797636745,536.963725068605,-49.5068471060657)) ;
#54999=CARTESIAN_POINT('Ctrl Pts',(180.942400305294,537.002790369321,-49.5025158569213)) ;
#55000=CARTESIAN_POINT('Ctrl Pts',(180.893961692549,537.039252837364,-49.4981952822219)) ;
#55001=CARTESIAN_POINT('Ctrl Pts',(180.845572449992,537.075678141689,-49.4938791111909)) ;
#55002=CARTESIAN_POINT('Ctrl Pts',(180.795146217323,537.10950619834,-49.48957389081)) ;
#55003=CARTESIAN_POINT('Ctrl Pts',(180.743002516597,537.140531585784,-49.4853247936267)) ;
#55004=CARTESIAN_POINT('Ctrl Pts',(180.690892178933,537.171537122278,-49.4810784151399)) ;
#55005=CARTESIAN_POINT('Ctrl Pts',(180.637066609147,537.199743670267,-49.4768882061335)) ;
#55006=CARTESIAN_POINT('Ctrl Pts',(180.581860613547,537.22497761557,-49.4727754537126)) ;
#55007=CARTESIAN_POINT('Ctrl Pts',(180.526668996164,537.250204988777,-49.4686637724443)) ;
#55008=CARTESIAN_POINT('Ctrl Pts',(180.470097682587,537.272461250094,-49.4646294978784)) ;
#55009=CARTESIAN_POINT('Ctrl Pts',(180.412496775638,537.291604078887,-49.4606693209704)) ;
#55010=CARTESIAN_POINT('Ctrl Pts',(180.354847343587,537.310763034296,-49.4567058078651)) ;
#55011=CARTESIAN_POINT('Ctrl Pts',(180.296166583948,537.326803113922,-49.4528163932275)) ;
#55012=CARTESIAN_POINT('Ctrl Pts',(180.236820997839,537.339614758446,-49.4489741210126)) ;
#55013=CARTESIAN_POINT('Ctrl Pts',(180.177453116158,537.352431216184,-49.4451304052926)) ;
#55014=CARTESIAN_POINT('Ctrl Pts',(180.11741992538,537.362016473207,-49.4413335941278)) ;
#55015=CARTESIAN_POINT('Ctrl Pts',(180.057103754115,537.36829795894,-49.4375359960147)) ;
#55016=CARTESIAN_POINT('Ctrl Pts',(179.996673041641,537.374591373298,-49.4337311862122)) ;
#55017=CARTESIAN_POINT('Ctrl Pts',(179.935958371058,537.377567925487,-49.4299251123059)) ;
#55018=CARTESIAN_POINT('Ctrl Pts',(179.875358970622,537.377198402245,-49.4260545749207)) ;
#55019=CARTESIAN_POINT('Ctrl Pts',(179.820907754908,537.376866369425,-49.4225767275398)) ;
#55020=CARTESIAN_POINT('Ctrl Pts',(179.76654921578,537.373832827106,-49.4190462440258)) ;
#55021=CARTESIAN_POINT('Ctrl Pts',(179.712583297119,537.368113257836,-49.4154127829198)) ;
#55022=CARTESIAN_POINT('Ctrl Pts',(179.707775847752,537.367603741083,-49.4150891030728)) ;
#55023=CARTESIAN_POINT('Ctrl Pts',(179.702971485346,537.367072927124,-49.414764606017)) ;
#55024=CARTESIAN_POINT('Ctrl Pts',(179.69817040477,537.366520837422,-49.4144392561638)) ;
#55025=CARTESIAN_POINT('Ctrl Pts',(179.698137064797,537.366517003565,-49.4144369968484)) ;
#55026=CARTESIAN_POINT('Ctrl Pts',(179.698103724982,537.366513168683,-49.4144347374918)) ;
#55027=CARTESIAN_POINT('Ctrl Pts',(179.698070385326,537.366509332774,-49.4144324780942)) ;
#55028=CARTESIAN_POINT('Ctrl Pts',(179.642901235647,537.360161822149,-49.4106937158674)) ;
#55029=CARTESIAN_POINT('Ctrl Pts',(179.587966985924,537.350973719898,-49.4068324308234)) ;
#55030=CARTESIAN_POINT('Ctrl Pts',(179.533570215717,537.339007287281,-49.4029116847749)) ;
#55031=CARTESIAN_POINT('Ctrl Pts',(179.528503948941,537.337892788392,-49.4025465243919)) ;
#55032=CARTESIAN_POINT('Ctrl Pts',(179.52344237049,537.336754216371,-49.4021808482317)) ;
#55033=CARTESIAN_POINT('Ctrl Pts',(179.51838574044,537.335591638312,-49.4018147072405)) ;
#55034=CARTESIAN_POINT('Ctrl Pts',(179.458436330543,537.32180857174,-49.3974738841729)) ;
#55035=CARTESIAN_POINT('Ctrl Pts',(179.399177962373,537.304647354077,-49.3930683863622)) ;
#55036=CARTESIAN_POINT('Ctrl Pts',(179.340996033269,537.284235756859,-49.3886690376785)) ;
#55037=CARTESIAN_POINT('Ctrl Pts',(179.283553092056,537.264083414077,-49.3843255665749)) ;
#55038=CARTESIAN_POINT('Ctrl Pts',(179.227159187739,537.240763104393,-49.3799883815136)) ;
#55039=CARTESIAN_POINT('Ctrl Pts',(179.172164866101,537.214431142677,-49.3757050966475)) ;
#55040=CARTESIAN_POINT('Ctrl Pts',(179.117203845471,537.188115125897,-49.3714244054619)) ;
#55041=CARTESIAN_POINT('Ctrl Pts',(179.063640628265,537.158791202608,-49.3671976842975)) ;
#55042=CARTESIAN_POINT('Ctrl Pts',(179.011806997811,537.126645653541,-49.3630486490804)) ;
#55043=CARTESIAN_POINT('Ctrl Pts',(178.959985625649,537.094507706672,-49.3589005950812)) ;
#55044=CARTESIAN_POINT('Ctrl Pts',(178.909893053504,537.059549450668,-49.3548301922803)) ;
#55045=CARTESIAN_POINT('Ctrl Pts',(178.86184309899,537.021986722675,-49.3508363377649)) ;
#55046=CARTESIAN_POINT('Ctrl Pts',(178.81265258268,536.983532368187,-49.3467476811228)) ;
#55047=CARTESIAN_POINT('Ctrl Pts',(178.765603040442,536.942348190254,-49.3427392229935)) ;
#55048=CARTESIAN_POINT('Ctrl Pts',(178.721010496985,536.898699000879,-49.3387837906119)) ;
#55049=CARTESIAN_POINT('Ctrl Pts',(178.67739648949,536.856007646564,-49.3349151559892)) ;
#55050=CARTESIAN_POINT('Ctrl Pts',(178.636133031795,536.810958220954,-49.3310968917719)) ;
#55051=CARTESIAN_POINT('Ctrl Pts',(178.597493283621,536.763831739696,-49.3272821279936)) ;
#55052=CARTESIAN_POINT('Ctrl Pts',(178.557553137294,536.715119244241,-49.3233389805688)) ;
#55053=CARTESIAN_POINT('Ctrl Pts',(178.52041697272,536.664187083124,-49.3193991427361)) ;
#55054=CARTESIAN_POINT('Ctrl Pts',(178.486355144813,536.611385916437,-49.315393240636)) ;
#55055=CARTESIAN_POINT('Ctrl Pts',(178.456716512441,536.565441395415,-49.3119075363459)) ;
#55056=CARTESIAN_POINT('Ctrl Pts',(178.429405010976,536.518081083629,-49.3083711621868)) ;
#55057=CARTESIAN_POINT('Ctrl Pts',(178.404574279484,536.469566591476,-49.3047334976926)) ;
#55058=CARTESIAN_POINT('Ctrl Pts',(178.40088276031,536.462354070246,-49.3041926957337)) ;
#55059=CARTESIAN_POINT('Ctrl Pts',(178.39724598531,536.455116000895,-49.3036496550576)) ;
#55060=CARTESIAN_POINT('Ctrl Pts',(178.393664370397,536.447853200198,-49.3031042093333)) ;
#55061=CARTESIAN_POINT('Ctrl Pts',(178.393650634657,536.447825346857,-49.3031021175115)) ;
#55062=CARTESIAN_POINT('Ctrl Pts',(178.393636899729,536.447797493154,-49.3031000256542)) ;
#55063=CARTESIAN_POINT('Ctrl Pts',(178.393623165612,536.447769639086,-49.3030979337616)) ;
#55064=CARTESIAN_POINT('Ctrl Pts',(178.369107074875,536.398048725274,-49.2993638000577)) ;
#55065=CARTESIAN_POINT('Ctrl Pts',(178.347095644288,536.346987147412,-49.295507131558)) ;
#55066=CARTESIAN_POINT('Ctrl Pts',(178.327700935934,536.294871854987,-49.2915911460869)) ;
#55067=CARTESIAN_POINT('Ctrl Pts',(178.325902770388,536.290040025524,-49.2912280784902)) ;
#55068=CARTESIAN_POINT('Ctrl Pts',(178.324127089886,536.28519917451,-49.2908645010089)) ;
#55069=CARTESIAN_POINT('Ctrl Pts',(178.322373978227,536.280349552575,-49.2905004640256)) ;
#55070=CARTESIAN_POINT('Ctrl Pts',(178.301455345353,536.222482467893,-49.2861566699679)) ;
#55071=CARTESIAN_POINT('Ctrl Pts',(178.283750973025,536.163360640214,-49.2817481185811)) ;
#55072=CARTESIAN_POINT('Ctrl Pts',(178.269363526799,536.103378216542,-49.2773461889775)) ;
#55073=CARTESIAN_POINT('Ctrl Pts',(178.255192293743,536.044297203013,-49.2730104111523)) ;
#55074=CARTESIAN_POINT('Ctrl Pts',(178.244238596283,535.984381273989,-49.26868134018)) ;
#55075=CARTESIAN_POINT('Ctrl Pts',(178.236561503253,535.924008234376,-49.2644066324919)) ;
#55076=CARTESIAN_POINT('Ctrl Pts',(178.228889180239,535.863672706402,-49.260134580812)) ;
#55077=CARTESIAN_POINT('Ctrl Pts',(178.224489264639,535.802880622491,-49.2559169588637)) ;
#55078=CARTESIAN_POINT('Ctrl Pts',(178.223385478994,535.742010380143,-49.2517775636806)) ;
#55079=CARTESIAN_POINT('Ctrl Pts',(178.222281967414,535.681155251669,-49.2476391962954)) ;
#55080=CARTESIAN_POINT('Ctrl Pts',(178.224472981386,535.620222024777,-49.2435790189435)) ;
#55081=CARTESIAN_POINT('Ctrl Pts',(178.22994765229,535.559590072891,-49.2395960575722)) ;
#55082=CARTESIAN_POINT('Ctrl Pts',(178.235575430961,535.497262453281,-49.235501706433)) ;
#55083=CARTESIAN_POINT('Ctrl Pts',(178.244673457541,535.435253267959,-49.2314889419518)) ;
#55084=CARTESIAN_POINT('Ctrl Pts',(178.257190212385,535.3739752658,-49.2275303827539)) ;
#55085=CARTESIAN_POINT('Ctrl Pts',(178.269381906449,535.314288656574,-49.2236746275461)) ;
#55086=CARTESIAN_POINT('Ctrl Pts',(178.284817191276,535.25529588635,-49.2198699305122)) ;
#55087=CARTESIAN_POINT('Ctrl Pts',(178.303408255902,535.197377418763,-49.216069516945)) ;
#55088=CARTESIAN_POINT('Ctrl Pts',(178.322742846318,535.137142576336,-49.2121171107105)) ;
#55089=CARTESIAN_POINT('Ctrl Pts',(178.345491509524,535.078070043124,-49.2081689190033)) ;
#55090=CARTESIAN_POINT('Ctrl Pts',(178.371503615203,535.020583097395,-49.2041543295508)) ;
#55091=CARTESIAN_POINT('Ctrl Pts',(178.394005286313,534.970854238001,-49.2006815245187)) ;
#55092=CARTESIAN_POINT('Ctrl Pts',(178.418949248333,534.9223109549,-49.1971583753286)) ;
#55093=CARTESIAN_POINT('Ctrl Pts',(178.446198877628,534.875223282812,-49.1935342109913)) ;
#55094=CARTESIAN_POINT('Ctrl Pts',(178.450435005529,534.867903205194,-49.1929708116328)) ;
#55095=CARTESIAN_POINT('Ctrl Pts',(178.454726838208,534.860618203501,-49.192404971074)) ;
#55096=CARTESIAN_POINT('Ctrl Pts',(178.459073848331,534.853369179574,-49.1918364989507)) ;
#55097=CARTESIAN_POINT('Ctrl Pts',(178.459089266447,534.853343468501,-49.1918344826754)) ;
#55098=CARTESIAN_POINT('Ctrl Pts',(178.459104685258,534.853317757881,-49.1918324663669)) ;
#55099=CARTESIAN_POINT('Ctrl Pts',(178.459120104762,534.853292047713,-49.1918304500253)) ;
#55100=CARTESIAN_POINT('Ctrl Pts',(178.487630711552,534.805754042735,-49.1881022419431)) ;
#55101=CARTESIAN_POINT('Ctrl Pts',(178.518624376016,534.759596052204,-49.184250960234)) ;
#55102=CARTESIAN_POINT('Ctrl Pts',(178.551920446847,534.715067415536,-49.1803397465476)) ;
#55103=CARTESIAN_POINT('Ctrl Pts',(178.555033589349,534.710904041663,-49.1799740527808)) ;
#55104=CARTESIAN_POINT('Ctrl Pts',(178.558166824182,534.706754924506,-49.1796078350872)) ;
#55105=CARTESIAN_POINT('Ctrl Pts',(178.561319981677,534.702620275257,-49.1792411450768)) ;
#55106=CARTESIAN_POINT('Ctrl Pts',(178.598632802673,534.653692992815,-49.1749019267721)) ;
#55107=CARTESIAN_POINT('Ctrl Pts',(178.638740920888,534.606789228571,-49.1704972367949)) ;
#55108=CARTESIAN_POINT('Ctrl Pts',(178.68136841272,534.562208404265,-49.1660984705568)) ;
#55109=CARTESIAN_POINT('Ctrl Pts',(178.723381799334,534.518269825508,-49.1617630743457)) ;
#55110=CARTESIAN_POINT('Ctrl Pts',(178.767842244335,534.476587367754,-49.1574337193977)) ;
#55111=CARTESIAN_POINT('Ctrl Pts',(178.814463529465,534.437415399226,-49.153158224334)) ;
#55112=CARTESIAN_POINT('Ctrl Pts',(178.861056184788,534.39826748593,-49.148885354822)) ;
#55113=CARTESIAN_POINT('Ctrl Pts',(178.909806969818,534.361626862826,-49.1446664143369)) ;
#55114=CARTESIAN_POINT('Ctrl Pts',(178.960410091427,534.327718441226,-49.1405253465973)) ;
#55115=CARTESIAN_POINT('Ctrl Pts',(179.011000954244,534.293818234066,-49.1363852820466)) ;
#55116=CARTESIAN_POINT('Ctrl Pts',(179.063443256845,534.262648941234,-49.1323230552208)) ;
#55117=CARTESIAN_POINT('Ctrl Pts',(179.117411709091,534.234406897251,-49.1283378089247)) ;
#55118=CARTESIAN_POINT('Ctrl Pts',(179.172827935434,534.205407223615,-49.1242456532007)) ;
#55119=CARTESIAN_POINT('Ctrl Pts',(179.229853421087,534.179494290947,-49.1202346507528)) ;
#55120=CARTESIAN_POINT('Ctrl Pts',(179.288114071575,534.15684775281,-49.1162776121979)) ;
#55121=CARTESIAN_POINT('Ctrl Pts',(179.344925102912,534.134764697144,-49.1124190311579)) ;
#55122=CARTESIAN_POINT('Ctrl Pts',(179.402910553671,534.115787699122,-49.1086113983487)) ;
#55123=CARTESIAN_POINT('Ctrl Pts',(179.461702632577,534.100049052582,-49.1048080018268)) ;
#55124=CARTESIAN_POINT('Ctrl Pts',(179.522744964334,534.083708013086,-49.1008590312068)) ;
#55125=CARTESIAN_POINT('Ctrl Pts',(179.58465699248,534.070858830823,-49.0969142071573)) ;
#55126=CARTESIAN_POINT('Ctrl Pts',(179.647003052361,534.06160374531,-49.092903296481)) ;
#55127=CARTESIAN_POINT('Ctrl Pts',(179.701041313284,534.053581927623,-49.0894268516491)) ;
#55128=CARTESIAN_POINT('Ctrl Pts',(179.755406537252,534.048259891954,-49.0859001036798)) ;
#55129=CARTESIAN_POINT('Ctrl Pts',(179.809797218069,534.04566919133,-49.0822723152298)) ;
#55130=CARTESIAN_POINT('Ctrl Pts',(179.818129605256,534.045272308622,-49.081716555722)) ;
#55131=CARTESIAN_POINT('Ctrl Pts',(179.826462664638,534.044939461026,-49.0811584249208)) ;
#55132=CARTESIAN_POINT('Ctrl Pts',(179.834795395502,534.04467069258,-49.0805977404102)) ;
#55133=CARTESIAN_POINT('Ctrl Pts',(179.834824989246,534.044669738047,-49.0805957491358)) ;
#55134=CARTESIAN_POINT('Ctrl Pts',(179.834854582986,534.044668784323,-49.0805937578292)) ;
#55135=CARTESIAN_POINT('Ctrl Pts',(179.834884176722,534.044667831406,-49.0805917664903)) ;
#55136=CARTESIAN_POINT('Ctrl Pts',(179.89031453931,534.042882977362,-49.0768619016354)) ;
#55137=CARTESIAN_POINT('Ctrl Pts',(179.945929545374,534.043935471606,-49.0730091891776)) ;
#55138=CARTESIAN_POINT('Ctrl Pts',(180.001421418037,534.047808397575,-49.0690967767647)) ;
#55139=CARTESIAN_POINT('Ctrl Pts',(180.00659353029,534.0481693731,-49.0687321209113)) ;
#55140=CARTESIAN_POINT('Ctrl Pts',(180.011764543074,534.048554827526,-49.0683669464357)) ;
#55141=CARTESIAN_POINT('Ctrl Pts',(180.016934189219,534.048964732805,-49.0680013044676)) ;
#55142=CARTESIAN_POINT('Ctrl Pts',(180.078270911918,534.053828169436,-49.0636630423553)) ;
#55143=CARTESIAN_POINT('Ctrl Pts',(180.139420276285,534.062136921654,-49.0592596355204)) ;
#55144=CARTESIAN_POINT('Ctrl Pts',(180.199981318123,534.073821174808,-49.0548623452926)) ;
#55145=CARTESIAN_POINT('Ctrl Pts',(180.259684867654,534.085339988979,-49.0505273169154)) ;
#55146=CARTESIAN_POINT('Ctrl Pts',(180.31881681372,534.100138984745,-49.0461985203468)) ;
#55147=CARTESIAN_POINT('Ctrl Pts',(180.377008192716,534.118115256545,-49.0419236855484)) ;
#55148=CARTESIAN_POINT('Ctrl Pts',(180.435164076688,534.136080563351,-49.037651458273)) ;
#55149=CARTESIAN_POINT('Ctrl Pts',(180.49238060773,534.157219160222,-49.0334332618706)) ;
#55150=CARTESIAN_POINT('Ctrl Pts',(180.54830297958,534.181395734778,-49.0292929444644)) ;
#55151=CARTESIAN_POINT('Ctrl Pts',(180.604212012219,534.205566542475,-49.0251536146517)) ;
#55152=CARTESIAN_POINT('Ctrl Pts',(180.658827472774,534.23277389933,-49.0210921290245)) ;
#55153=CARTESIAN_POINT('Ctrl Pts',(180.711808013897,534.262850622761,-49.0171075326426)) ;
#55154=CARTESIAN_POINT('Ctrl Pts',(180.766185635232,534.293720459932,-49.0130178637069)) ;
#55155=CARTESIAN_POINT('Ctrl Pts',(180.818840769077,534.327613273201,-49.0090091772793)) ;
#55156=CARTESIAN_POINT('Ctrl Pts',(180.869420113903,534.364312101834,-49.0050542246641)) ;
#55157=CARTESIAN_POINT('Ctrl Pts',(180.918763220308,534.400113953606,-49.0011959372863)) ;
#55158=CARTESIAN_POINT('Ctrl Pts',(180.966130585896,534.438586397744,-48.9973884266311)) ;
#55159=CARTESIAN_POINT('Ctrl Pts',(181.01121166194,534.479491822943,-48.9935849087003)) ;
#55160=CARTESIAN_POINT('Ctrl Pts',(181.057986924741,534.521934510243,-48.9896384511976)) ;
#55161=CARTESIAN_POINT('Ctrl Pts',(181.102300177346,534.566997063816,-48.9856958697069)) ;
#55162=CARTESIAN_POINT('Ctrl Pts',(181.143829998704,534.614369133583,-48.9816870242632)) ;
#55163=CARTESIAN_POINT('Ctrl Pts',(181.179839562802,534.655444378478,-48.9782110455028)) ;
#55164=CARTESIAN_POINT('Ctrl Pts',(181.213757200832,534.698256567649,-48.9746845931137)) ;
#55165=CARTESIAN_POINT('Ctrl Pts',(181.245393149751,534.742569466473,-48.9710569730146)) ;
#55166=CARTESIAN_POINT('Ctrl Pts',(181.250225564489,534.749338294742,-48.9705028513451)) ;
#55167=CARTESIAN_POINT('Ctrl Pts',(181.255004836416,534.756142165679,-48.9699463691506)) ;
#55168=CARTESIAN_POINT('Ctrl Pts',(181.259730391743,534.762980269371,-48.9693873457525)) ;
#55169=CARTESIAN_POINT('Ctrl Pts',(181.259747376072,534.763004846505,-48.9693853365415)) ;
#55170=CARTESIAN_POINT('Ctrl Pts',(181.259764359708,534.763029424081,-48.9693833272977)) ;
#55171=CARTESIAN_POINT('Ctrl Pts',(181.25978134265,534.763054002099,-48.9693813180211)) ;
#55172=CARTESIAN_POINT('Ctrl Pts',(181.291517598264,534.808983281234,-48.9656265552922)) ;
#55173=CARTESIAN_POINT('Ctrl Pts',(181.320935495203,534.856622644612,-48.9617474963916)) ;
#55174=CARTESIAN_POINT('Ctrl Pts',(181.347882919564,534.905702589268,-48.9578083354708)) ;
#55175=CARTESIAN_POINT('Ctrl Pts',(181.350577125159,534.910609605973,-48.9574144978538)) ;
#55176=CARTESIAN_POINT('Ctrl Pts',(181.353246637699,534.915530979809,-48.9570200594561)) ;
#55177=CARTESIAN_POINT('Ctrl Pts',(181.355891307121,534.920466412928,-48.9566250844334)) ;
#55178=CARTESIAN_POINT('Ctrl Pts',(181.384939266138,534.974675176342,-48.9522868415599)) ;
#55179=CARTESIAN_POINT('Ctrl Pts',(181.410990463583,535.030586077216,-48.9478844932253)) ;
#55180=CARTESIAN_POINT('Ctrl Pts',(181.433888757778,535.087830713585,-48.9434886857549)) ;
#55181=CARTESIAN_POINT('Ctrl Pts',(181.456751886361,535.14498743761,-48.9390996290608)) ;
#55182=CARTESIAN_POINT('Ctrl Pts',(181.476472164991,535.203473793683,-48.9347174294075)) ;
#55183=CARTESIAN_POINT('Ctrl Pts',(181.492931602766,535.262916609204,-48.9303909258775)) ;
#55184=CARTESIAN_POINT('Ctrl Pts',(181.509376246892,535.322305997857,-48.9260683109845)) ;
#55185=CARTESIAN_POINT('Ctrl Pts',(181.522566046394,535.382650172329,-48.9218014321654)) ;
#55186=CARTESIAN_POINT('Ctrl Pts',(181.532416933869,535.443570141042,-48.9176140482287)) ;
#55187=CARTESIAN_POINT('Ctrl Pts',(181.542262726689,535.504458603335,-48.9134288299117)) ;
#55188=CARTESIAN_POINT('Ctrl Pts',(181.548773015915,535.565922299089,-48.9093230295455)) ;
#55189=CARTESIAN_POINT('Ctrl Pts',(181.551896803974,535.627575378101,-48.9052943808938)) ;
#55190=CARTESIAN_POINT('Ctrl Pts',(181.553311741504,535.655501490141,-48.9034695816231)) ;
#55191=CARTESIAN_POINT('Ctrl Pts',(181.554032326547,535.683466353274,-48.9016602577813)) ;
#55192=CARTESIAN_POINT('Ctrl Pts',(181.55405613246,535.711433585225,-48.8998644770965)) ;
#55193=CARTESIAN_POINT('Ctrl Pts',(181.554527408033,535.711416213393,-48.8995931994887)) ;
#55194=CARTESIAN_POINT('Ctrl Pts',(181.554490128221,535.784394239434,-48.8949665191685)) ;
#55195=CARTESIAN_POINT('Ctrl Pts',(181.549657875426,535.857294737052,-48.8904718398709)) ;
#55196=CARTESIAN_POINT('Ctrl Pts',(181.526253544035,536.033724863836,-48.8795881565153)) ;
#55197=CARTESIAN_POINT('Ctrl Pts',(181.502641909275,536.136251581272,-48.8732625061677)) ;
#55198=CARTESIAN_POINT('Ctrl Pts',(181.463949750002,536.252705458684,-48.8654288299871)) ;
#55199=CARTESIAN_POINT('Ctrl Pts',(181.458085759128,536.269455214264,-48.8642854378288)) ;
#55200=CARTESIAN_POINT('Ctrl Pts',(181.451956083968,536.286106171205,-48.8631290382246)) ;
#55201=CARTESIAN_POINT('Origin',(179.888527625402,502.164639879998,-37.0221601717597)) ;
#55202=CARTESIAN_POINT('',(181.517728960952,505.503023000143,-38.2742386719919)) ;
#55203=CARTESIAN_POINT('',(181.517728888183,505.561201209649,-38.2742387666786)) ;
#55204=CARTESIAN_POINT('',(181.517728902316,502.164639879998,-38.2742387482878)) ;
#55205=CARTESIAN_POINT('',(179.0652954453,505.710565160536,-38.9047876814237)) ;
#55206=CARTESIAN_POINT('Ctrl Pts',(181.517728888183,505.561201209649,-38.2742387666786)) ;
#55207=CARTESIAN_POINT('Ctrl Pts',(181.506945791598,505.562230187057,-38.2882697026309)) ;
#55208=CARTESIAN_POINT('Ctrl Pts',(181.495980453669,505.563264428463,-38.302162624092)) ;
#55209=CARTESIAN_POINT('Ctrl Pts',(181.398708147322,505.572330902422,-38.4221827887736)) ;
#55210=CARTESIAN_POINT('Ctrl Pts',(181.302190203612,505.580630274102,-38.5195793218676)) ;
#55211=CARTESIAN_POINT('Ctrl Pts',(181.157295447536,505.591637868681,-38.6392064954657)) ;
#55212=CARTESIAN_POINT('Ctrl Pts',(181.116672538108,505.594585097538,-38.6702716511746)) ;
#55213=CARTESIAN_POINT('Ctrl Pts',(181.050521260699,505.599116388462,-38.7170531278522)) ;
#55214=CARTESIAN_POINT('Ctrl Pts',(181.025737466234,505.600756416772,-38.7337808892257)) ;
#55215=CARTESIAN_POINT('Ctrl Pts',(180.965777197614,505.604581481536,-38.7723730801744)) ;
#55216=CARTESIAN_POINT('Ctrl Pts',(180.930289321945,505.606736902647,-38.7937258388954)) ;
#55217=CARTESIAN_POINT('Ctrl Pts',(180.798918856659,505.614413412551,-38.8674563566956)) ;
#55218=CARTESIAN_POINT('Ctrl Pts',(180.699540091164,505.619658122738,-38.913242605739)) ;
#55219=CARTESIAN_POINT('Ctrl Pts',(180.472699884994,505.631291927045,-38.9965642264894)) ;
#55220=CARTESIAN_POINT('Ctrl Pts',(180.344303596121,505.637673696071,-39.0300927677737)) ;
#55221=CARTESIAN_POINT('Ctrl Pts',(180.154882828558,505.647462318702,-39.0604403723471)) ;
#55222=CARTESIAN_POINT('Ctrl Pts',(180.095810191248,505.650561966847,-39.0672920317259)) ;
#55223=CARTESIAN_POINT('Ctrl Pts',(179.980836990606,505.656723534007,-39.0755948786593)) ;
#55224=CARTESIAN_POINT('Ctrl Pts',(179.925010163103,505.659773616552,-39.0773446774586)) ;
#55225=CARTESIAN_POINT('Ctrl Pts',(179.742716349138,505.669938782097,-39.075628525469)) ;
#55226=CARTESIAN_POINT('Ctrl Pts',(179.616641991441,505.677310635259,-39.0627641504108)) ;
#55227=CARTESIAN_POINT('Ctrl Pts',(179.386535557587,505.691124319092,-39.0175742582776)) ;
#55228=CARTESIAN_POINT('Ctrl Pts',(179.282308570779,505.697517319274,-38.9884191047433)) ;
#55229=CARTESIAN_POINT('Ctrl Pts',(179.159260972625,505.704950845021,-38.9432787890502)) ;
#55230=CARTESIAN_POINT('Ctrl Pts',(179.137801261035,505.70624253918,-38.9349948726183)) ;
#55231=CARTESIAN_POINT('Ctrl Pts',(179.099325627916,505.708544927455,-38.9193951581186)) ;
#55232=CARTESIAN_POINT('Ctrl Pts',(179.082261060808,505.709561184396,-38.9122063771401)) ;
#55233=CARTESIAN_POINT('Ctrl Pts',(179.0652954453,505.710565160536,-38.9047876814236)) ;
#55234=CARTESIAN_POINT('',(178.234426126892,505.709295655298,-38.244821809929)) ;
#55235=CARTESIAN_POINT('Origin',(179.888527625402,505.710565160536,-37.0221601717597)) ;
#55236=CARTESIAN_POINT('Ctrl Pts',(178.236339423148,505.708026150059,-38.2437459062988)) ;
#55237=CARTESIAN_POINT('Ctrl Pts',(178.246212321761,505.70712926237,-38.2570989491102)) ;
#55238=CARTESIAN_POINT('Ctrl Pts',(178.256247088797,505.706243310869,-38.2703322870222)) ;
#55239=CARTESIAN_POINT('Ctrl Pts',(178.280000811933,505.704201178492,-38.3008810138008)) ;
#55240=CARTESIAN_POINT('Ctrl Pts',(178.293840894228,505.703052463216,-38.3180999086104)) ;
#55241=CARTESIAN_POINT('Ctrl Pts',(178.386783981602,505.695578963799,-38.4299892423993)) ;
#55242=CARTESIAN_POINT('Ctrl Pts',(178.474004687336,505.689671126553,-38.5176022345782)) ;
#55243=CARTESIAN_POINT('Ctrl Pts',(178.659038150305,505.677961340228,-38.6727023863125)) ;
#55244=CARTESIAN_POINT('Ctrl Pts',(178.755871947701,505.67218414584,-38.7405959966526)) ;
#55245=CARTESIAN_POINT('Ctrl Pts',(178.903893650852,505.663356853194,-38.8264075768925)) ;
#55246=CARTESIAN_POINT('Ctrl Pts',(178.950806700938,505.660562516286,-38.8512286646373)) ;
#55247=CARTESIAN_POINT('Ctrl Pts',(179.046351159345,505.654848271938,-38.897137512791)) ;
#55248=CARTESIAN_POINT('Ctrl Pts',(179.094942294336,505.651930805372,-38.9182147125759)) ;
#55249=CARTESIAN_POINT('Ctrl Pts',(179.247425597898,505.642725165823,-38.9774680376964)) ;
#55250=CARTESIAN_POINT('Ctrl Pts',(179.353616946369,505.636232474154,-39.0091442621736)) ;
#55251=CARTESIAN_POINT('Ctrl Pts',(179.555318928392,505.62391815518,-39.0519640424075)) ;
#55252=CARTESIAN_POINT('Ctrl Pts',(179.650079541876,505.618143888782,-39.0652643315994)) ;
#55253=CARTESIAN_POINT('Ctrl Pts',(179.786761310523,505.610059059747,-39.0748068607388)) ;
#55254=CARTESIAN_POINT('Ctrl Pts',(179.828180548463,505.607641981781,-39.0764418972258)) ;
#55255=CARTESIAN_POINT('Ctrl Pts',(179.904055275859,505.603306143197,-39.0771400117366)) ;
#55256=CARTESIAN_POINT('Ctrl Pts',(179.938492507703,505.601372943566,-39.076591254611)) ;
#55257=CARTESIAN_POINT('Ctrl Pts',(180.003921401465,505.597786719259,-39.073902279837)) ;
#55258=CARTESIAN_POINT('Ctrl Pts',(180.034908371763,505.596127113771,-39.0719245855875)) ;
#55259=CARTESIAN_POINT('Ctrl Pts',(180.137752135288,505.590716041551,-39.0630165928796)) ;
#55260=CARTESIAN_POINT('Ctrl Pts',(180.209293152321,505.58710800581,-39.0530021324179)) ;
#55261=CARTESIAN_POINT('Ctrl Pts',(180.443789446986,505.575387287441,-39.0074723494109)) ;
#55262=CARTESIAN_POINT('Ctrl Pts',(180.602935399332,505.567551403571,-38.9559137276696)) ;
#55263=CARTESIAN_POINT('Ctrl Pts',(180.808399358356,505.556076568485,-38.8604792358664)) ;
#55264=CARTESIAN_POINT('Ctrl Pts',(180.861558421441,505.552978927717,-38.8329034306958)) ;
#55265=CARTESIAN_POINT('Ctrl Pts',(180.956628338775,505.547149905503,-38.7781903545838)) ;
#55266=CARTESIAN_POINT('Ctrl Pts',(180.998900001781,505.544446254891,-38.7517710284809)) ;
#55267=CARTESIAN_POINT('Ctrl Pts',(181.100521819816,505.537647960482,-38.6829969191819)) ;
#55268=CARTESIAN_POINT('Ctrl Pts',(181.158654772859,505.533491702225,-38.6389730409796)) ;
#55269=CARTESIAN_POINT('Ctrl Pts',(181.326530288598,505.520674159904,-38.497191454525)) ;
#55270=CARTESIAN_POINT('Ctrl Pts',(181.428243787735,505.511729959464,-38.3906765500404)) ;
#55271=CARTESIAN_POINT('Ctrl Pts',(181.517728960952,505.503023000143,-38.2742386719919)) ;
#55272=CARTESIAN_POINT('Origin',(179.888527625402,502.164639879998,-37.0221601717597)) ;
#55273=CARTESIAN_POINT('',(181.51772890232,504.803342258844,-38.274238748284)) ;
#55274=CARTESIAN_POINT('',(181.517728902317,504.861481368308,-38.2742387482878)) ;
#55275=CARTESIAN_POINT('',(181.517728902316,502.164639879998,-38.2742387482878)) ;
#55276=CARTESIAN_POINT('',(179.887971218886,505.313227684039,-34.9674102470945)) ;
#55277=CARTESIAN_POINT('Ctrl Pts',(181.517728902317,504.861481368308,-38.2742387482878)) ;
#55278=CARTESIAN_POINT('Ctrl Pts',(181.50282363087,504.862713419422,-38.2936334474142)) ;
#55279=CARTESIAN_POINT('Ctrl Pts',(181.487566558281,504.863956449484,-38.3127691192065)) ;
#55280=CARTESIAN_POINT('Ctrl Pts',(181.437041422955,504.868022782347,-38.3738648120083)) ;
#55281=CARTESIAN_POINT('Ctrl Pts',(181.400446089409,504.870893009831,-38.4146766830833)) ;
#55282=CARTESIAN_POINT('Ctrl Pts',(181.326218546114,504.876610157377,-38.4910775843731)) ;
#55283=CARTESIAN_POINT('Ctrl Pts',(181.288785863608,504.879447242012,-38.5268028955588)) ;
#55284=CARTESIAN_POINT('Ctrl Pts',(181.178928258441,504.887664764052,-38.62399685699)) ;
#55285=CARTESIAN_POINT('Ctrl Pts',(181.103541408712,504.893184704261,-38.681904829899)) ;
#55286=CARTESIAN_POINT('Ctrl Pts',(180.910205101557,504.906968927363,-38.8101651976646)) ;
#55287=CARTESIAN_POINT('Ctrl Pts',(180.788689014218,504.915343739997,-38.8743198567907)) ;
#55288=CARTESIAN_POINT('Ctrl Pts',(180.617900324062,504.926134764785,-38.9436822371964)) ;
#55289=CARTESIAN_POINT('Ctrl Pts',(180.573504544794,504.928853816136,-38.9599524418868)) ;
#55290=CARTESIAN_POINT('Ctrl Pts',(180.500862519732,504.933121744483,-38.9837652791507)) ;
#55291=CARTESIAN_POINT('Ctrl Pts',(180.472951274591,504.934717718867,-38.9922611562714)) ;
#55292=CARTESIAN_POINT('Ctrl Pts',(180.403482470405,504.93858097189,-39.0118000715804)) ;
#55293=CARTESIAN_POINT('Ctrl Pts',(180.361743305479,504.940811754778,-39.0221383886533)) ;
#55294=CARTESIAN_POINT('Ctrl Pts',(180.262772521127,504.94595474411,-39.0433799164438)) ;
#55295=CARTESIAN_POINT('Ctrl Pts',(180.205340497337,504.948826149853,-39.0531744030832)) ;
#55296=CARTESIAN_POINT('Ctrl Pts',(179.972778671358,504.960259848407,-39.08272897806)) ;
#55297=CARTESIAN_POINT('Ctrl Pts',(179.795872929643,504.968592730584,-39.0823677814946)) ;
#55298=CARTESIAN_POINT('Ctrl Pts',(179.568754377692,504.980417511158,-39.0525637117123)) ;
#55299=CARTESIAN_POINT('Ctrl Pts',(179.516616330564,504.983204364824,-39.043663269288)) ;
#55300=CARTESIAN_POINT('Ctrl Pts',(179.412716238464,504.988933406861,-39.0217709373221)) ;
#55301=CARTESIAN_POINT('Ctrl Pts',(179.361001525323,504.991874491635,-39.0087540280226)) ;
#55302=CARTESIAN_POINT('Ctrl Pts',(179.192627011546,505.001764611085,-38.9593349294167)) ;
#55303=CARTESIAN_POINT('Ctrl Pts',(179.07871718205,505.008980873443,-38.9145458267304)) ;
#55304=CARTESIAN_POINT('Ctrl Pts',(178.852478096477,505.024159551189,-38.8014044454432)) ;
#55305=CARTESIAN_POINT('Ctrl Pts',(178.741331359726,505.03210293927,-38.7318540881188)) ;
#55306=CARTESIAN_POINT('Ctrl Pts',(178.610969676867,505.041478563465,-38.6318078637487)) ;
#55307=CARTESIAN_POINT('Ctrl Pts',(178.584892698132,505.043356010995,-38.6107621604143)) ;
#55308=CARTESIAN_POINT('Ctrl Pts',(178.534889910419,505.046940292589,-38.5683459656992)) ;
#55309=CARTESIAN_POINT('Ctrl Pts',(178.510927173022,505.048649644795,-38.5470348358357)) ;
#55310=CARTESIAN_POINT('Ctrl Pts',(178.425797979676,505.054732640259,-38.4676802790939)) ;
#55311=CARTESIAN_POINT('Ctrl Pts',(178.367715003357,505.058905309628,-38.4064426497816)) ;
#55312=CARTESIAN_POINT('Ctrl Pts',(178.200174680065,505.071625779624,-38.2064861184753)) ;
#55313=CARTESIAN_POINT('Ctrl Pts',(178.104713582771,505.079982814636,-38.0571331416867)) ;
#55314=CARTESIAN_POINT('Ctrl Pts',(178.007172384774,505.091822113924,-37.8499593367763)) ;
#55315=CARTESIAN_POINT('Ctrl Pts',(177.98665561363,505.094590877831,-37.8016671839152)) ;
#55316=CARTESIAN_POINT('Ctrl Pts',(177.948916516739,505.100325959965,-37.7024474158823)) ;
#55317=CARTESIAN_POINT('Ctrl Pts',(177.931800044227,505.103293208672,-37.6515236510647)) ;
#55318=CARTESIAN_POINT('Ctrl Pts',(177.88195337532,505.113298788486,-37.4814235451365)) ;
#55319=CARTESIAN_POINT('Ctrl Pts',(177.857977493662,505.120610343437,-37.359979317665)) ;
#55320=CARTESIAN_POINT('Ctrl Pts',(177.831742032306,505.135670801813,-37.1105929793872)) ;
#55321=CARTESIAN_POINT('Ctrl Pts',(177.830211815779,505.143391072684,-36.9830826193027)) ;
#55322=CARTESIAN_POINT('Ctrl Pts',(177.843214108276,505.15258837476,-36.8225839898811)) ;
#55323=CARTESIAN_POINT('Ctrl Pts',(177.846770636977,505.154482903932,-36.7889934075561)) ;
#55324=CARTESIAN_POINT('Ctrl Pts',(177.855261939735,505.158063070187,-36.7241161014549)) ;
#55325=CARTESIAN_POINT('Ctrl Pts',(177.860094924488,505.159752705507,-36.6928267068736)) ;
#55326=CARTESIAN_POINT('Ctrl Pts',(177.879441866848,505.16552342851,-36.5842648942137)) ;
#55327=CARTESIAN_POINT('Ctrl Pts',(177.897666316002,505.16943123101,-36.5077174405858)) ;
#55328=CARTESIAN_POINT('Ctrl Pts',(177.973348629029,505.182320458574,-36.2551331059409)) ;
#55329=CARTESIAN_POINT('Ctrl Pts',(178.050158718153,505.191034474329,-36.0858695805616)) ;
#55330=CARTESIAN_POINT('Ctrl Pts',(178.176214430807,505.203300396884,-35.885200307277)) ;
#55331=CARTESIAN_POINT('Ctrl Pts',(178.205492365261,505.206044401104,-35.8422932854756)) ;
#55332=CARTESIAN_POINT('Ctrl Pts',(178.268306221195,505.211757672042,-35.7573412044155)) ;
#55333=CARTESIAN_POINT('Ctrl Pts',(178.301929954114,505.214729261373,-35.7154117370569)) ;
#55334=CARTESIAN_POINT('Ctrl Pts',(178.381136018215,505.221555419153,-35.6242092075448)) ;
#55335=CARTESIAN_POINT('Ctrl Pts',(178.427565683494,505.225442493708,-35.5757559302762)) ;
#55336=CARTESIAN_POINT('Ctrl Pts',(178.574219856507,505.237356109792,-35.4369869716062)) ;
#55337=CARTESIAN_POINT('Ctrl Pts',(178.681038772688,505.245589361687,-35.3541834205342)) ;
#55338=CARTESIAN_POINT('Ctrl Pts',(178.846459501428,505.257187660007,-35.2502240118311)) ;
#55339=CARTESIAN_POINT('Ctrl Pts',(178.899128640742,505.260725524652,-35.2202848727496)) ;
#55340=CARTESIAN_POINT('Ctrl Pts',(178.979904262458,505.265842752296,-35.1789805692709)) ;
#55341=CARTESIAN_POINT('Ctrl Pts',(179.007062480536,505.267512411627,-35.1658393257151)) ;
#55342=CARTESIAN_POINT('Ctrl Pts',(179.068368260311,505.271158027716,-35.1378241064699)) ;
#55343=CARTESIAN_POINT('Ctrl Pts',(179.102648687739,505.273116927721,-35.1232714293314)) ;
#55344=CARTESIAN_POINT('Ctrl Pts',(179.180511213483,505.277429531326,-35.0926874892022)) ;
#55345=CARTESIAN_POINT('Ctrl Pts',(179.22427952349,505.279760331122,-35.0771853693676)) ;
#55346=CARTESIAN_POINT('Ctrl Pts',(179.438002309131,505.290856676824,-35.0095451153084)) ;
#55347=CARTESIAN_POINT('Ctrl Pts',(179.613705040265,505.299195207764,-34.9781278433698)) ;
#55348=CARTESIAN_POINT('Ctrl Pts',(179.82347870271,505.309884020926,-34.9681868744578)) ;
#55349=CARTESIAN_POINT('Ctrl Pts',(179.855723251356,505.311544657051,-34.9674189795339)) ;
#55350=CARTESIAN_POINT('Ctrl Pts',(179.887971218886,505.313227684039,-34.9674102470945)) ;
#55351=CARTESIAN_POINT('Ctrl Pts',(179.887972413115,505.313227746366,-34.9674102467714)) ;
#55352=CARTESIAN_POINT('Ctrl Pts',(179.931624596704,505.315505962097,-34.9673984515508)) ;
#55353=CARTESIAN_POINT('Ctrl Pts',(179.975264213753,505.317824392976,-34.9687777029824)) ;
#55354=CARTESIAN_POINT('Ctrl Pts',(180.071034514204,505.323019000527,-34.9748630274251)) ;
#55355=CARTESIAN_POINT('Ctrl Pts',(180.12309408548,505.325912770164,-34.9801728486144)) ;
#55356=CARTESIAN_POINT('Ctrl Pts',(180.339374193126,505.338248025649,-35.0106121445431)) ;
#55357=CARTESIAN_POINT('Ctrl Pts',(180.500421876701,505.348260125775,-35.0536184191277)) ;
#55358=CARTESIAN_POINT('Ctrl Pts',(180.738149110347,505.36365468944,-35.1491235186524)) ;
#55359=CARTESIAN_POINT('Ctrl Pts',(180.819498133654,505.369028756897,-35.1881973587433)) ;
#55360=CARTESIAN_POINT('Ctrl Pts',(180.926256113304,505.376002474111,-35.2484161508916)) ;
#55361=CARTESIAN_POINT('Ctrl Pts',(180.954110624124,505.377813697724,-35.2650086380489)) ;
#55362=CARTESIAN_POINT('Ctrl Pts',(181.01002191576,505.38141385678,-35.3001329815278)) ;
#55363=CARTESIAN_POINT('Ctrl Pts',(181.038039513195,505.383199869814,-35.3187078542507)) ;
#55364=CARTESIAN_POINT('Ctrl Pts',(181.170976703106,505.39164948612,-35.4116158754433)) ;
#55365=CARTESIAN_POINT('Ctrl Pts',(181.269228688345,505.397831670211,-35.4950058982537)) ;
#55366=CARTESIAN_POINT('Ctrl Pts',(181.443401754122,505.409947652062,-35.6734754734415)) ;
#55367=CARTESIAN_POINT('Ctrl Pts',(181.519965404593,505.41585405327,-35.767173573077)) ;
#55368=CARTESIAN_POINT('Ctrl Pts',(181.618071696416,505.424860150587,-35.911500749566)) ;
#55369=CARTESIAN_POINT('Ctrl Pts',(181.646532203332,505.427692129625,-35.957122028688)) ;
#55370=CARTESIAN_POINT('Ctrl Pts',(181.699728654425,505.433482231359,-36.0503474094442)) ;
#55371=CARTESIAN_POINT('Ctrl Pts',(181.724454417662,505.436437682742,-36.0979084387649)) ;
#55372=CARTESIAN_POINT('Ctrl Pts',(181.795453102887,505.445823773504,-36.2485964610278)) ;
#55373=CARTESIAN_POINT('Ctrl Pts',(181.835094616754,505.452470648951,-36.3545999288584)) ;
#55374=CARTESIAN_POINT('Ctrl Pts',(181.891794920882,505.464954704331,-36.5552141626888)) ;
#55375=CARTESIAN_POINT('Ctrl Pts',(181.911330962379,505.470739045616,-36.6488165827598)) ;
#55376=CARTESIAN_POINT('Ctrl Pts',(181.931993385343,505.479746454951,-36.7997332961412)) ;
#55377=CARTESIAN_POINT('Ctrl Pts',(181.937363084996,505.483052483556,-36.8563279573793)) ;
#55378=CARTESIAN_POINT('Ctrl Pts',(181.941943114895,505.487906593332,-36.9424778543331)) ;
#55379=CARTESIAN_POINT('Ctrl Pts',(181.942874221793,505.489533360928,-36.9719122135335)) ;
#55380=CARTESIAN_POINT('Ctrl Pts',(181.943521358908,505.492982993229,-37.0358350683226)) ;
#55381=CARTESIAN_POINT('Ctrl Pts',(181.943002633073,505.494792895322,-37.0703162863717)) ;
#55382=CARTESIAN_POINT('Ctrl Pts',(181.937076119565,505.502368070327,-37.2176063008932)) ;
#55383=CARTESIAN_POINT('Ctrl Pts',(181.92324108779,505.507758163467,-37.3298881288155)) ;
#55384=CARTESIAN_POINT('Ctrl Pts',(181.872006909521,505.519758210943,-37.5762796076252)) ;
#55385=CARTESIAN_POINT('Ctrl Pts',(181.830091785001,505.526352693664,-37.7088648575302)) ;
#55386=CARTESIAN_POINT('Ctrl Pts',(181.753104771879,505.536221744344,-37.8872865964356)) ;
#55387=CARTESIAN_POINT('Ctrl Pts',(181.729004159842,505.539110381616,-37.9374399116075)) ;
#55388=CARTESIAN_POINT('Ctrl Pts',(181.679482633419,505.544731528113,-38.0306080534783)) ;
#55389=CARTESIAN_POINT('Ctrl Pts',(181.654469790178,505.547447447767,-38.0737944312678)) ;
#55390=CARTESIAN_POINT('Ctrl Pts',(181.59367203227,505.553795920953,-38.1704705610456)) ;
#55391=CARTESIAN_POINT('Ctrl Pts',(181.556903044612,505.557463014257,-38.2232654608651)) ;
#55392=CARTESIAN_POINT('Ctrl Pts',(181.517728888183,505.561201209649,-38.2742387666786)) ;
#55393=CARTESIAN_POINT('Ctrl Pts',(181.517728960952,505.503023000143,-38.2742386719921)) ;
#55394=CARTESIAN_POINT('Ctrl Pts',(181.554510770023,505.49944410876,-38.2263782762974)) ;
#55395=CARTESIAN_POINT('Ctrl Pts',(181.589163153578,505.495917597715,-38.1769246559147)) ;
#55396=CARTESIAN_POINT('Ctrl Pts',(181.635738170017,505.491018477495,-38.1038005625687)) ;
#55397=CARTESIAN_POINT('Ctrl Pts',(181.649453667286,505.489553360676,-38.0813250528931)) ;
#55398=CARTESIAN_POINT('Ctrl Pts',(181.67892390674,505.486364843897,-38.030876639769)) ;
#55399=CARTESIAN_POINT('Ctrl Pts',(181.69446269358,505.48465660206,-38.0027857105539)) ;
#55400=CARTESIAN_POINT('Ctrl Pts',(181.78637602339,505.474307774169,-37.8270242641324)) ;
#55401=CARTESIAN_POINT('Ctrl Pts',(181.845261127654,505.466528423751,-37.6708843680565)) ;
#55402=CARTESIAN_POINT('Ctrl Pts',(181.907842843034,505.453676279027,-37.4144626183609)) ;
#55403=CARTESIAN_POINT('Ctrl Pts',(181.924202799645,505.448836792646,-37.3180640728702)) ;
#55404=CARTESIAN_POINT('Ctrl Pts',(181.938627586626,505.441114805809,-37.1696078189518)) ;
#55405=CARTESIAN_POINT('Ctrl Pts',(181.941679128983,505.438392589766,-37.118175395422)) ;
#55406=CARTESIAN_POINT('Ctrl Pts',(181.943954873281,505.432713613478,-37.013179198085)) ;
#55407=CARTESIAN_POINT('Ctrl Pts',(181.943023622886,505.429753999333,-36.9596520981478)) ;
#55408=CARTESIAN_POINT('Ctrl Pts',(181.930436534106,505.417150816679,-36.7369218776964)) ;
#55409=CARTESIAN_POINT('Ctrl Pts',(181.899947743615,505.406908163481,-36.5694745900173)) ;
#55410=CARTESIAN_POINT('Ctrl Pts',(181.824023270054,505.391680435388,-36.3271975443084)) ;
#55411=CARTESIAN_POINT('Ctrl Pts',(181.793854915335,505.386668174524,-36.2483082814553)) ;
#55412=CARTESIAN_POINT('Ctrl Pts',(181.745708792909,505.380059492607,-36.1424478654832)) ;
#55413=CARTESIAN_POINT('Ctrl Pts',(181.731823382325,505.378278524731,-36.1137127525355)) ;
#55414=CARTESIAN_POINT('Ctrl Pts',(181.702253366721,505.374745292009,-36.0559916111054)) ;
#55415=CARTESIAN_POINT('Ctrl Pts',(181.686529709557,505.372995763219,-36.0270362920814)) ;
#55416=CARTESIAN_POINT('Ctrl Pts',(181.602523575396,505.364217038176,-35.8808355256149)) ;
#55417=CARTESIAN_POINT('Ctrl Pts',(181.523439320893,505.357740639546,-35.77017131911)) ;
#55418=CARTESIAN_POINT('Ctrl Pts',(181.355597259194,505.345408502778,-35.5786006272249)) ;
#55419=CARTESIAN_POINT('Ctrl Pts',(181.269558985418,505.339596000749,-35.4960846905156)) ;
#55420=CARTESIAN_POINT('Ctrl Pts',(181.135607706568,505.330733272368,-35.3882707736326)) ;
#55421=CARTESIAN_POINT('Ctrl Pts',(181.093078107769,505.327945947911,-35.3566690283912)) ;
#55422=CARTESIAN_POINT('Ctrl Pts',(181.006093460233,505.322266517321,-35.2971106039524)) ;
#55423=CARTESIAN_POINT('Ctrl Pts',(180.961693510379,505.319377809688,-35.2691445782153)) ;
#55424=CARTESIAN_POINT('Ctrl Pts',(180.761128228956,505.306349393143,-35.1532921951252)) ;
#55425=CARTESIAN_POINT('Ctrl Pts',(180.594945730838,505.295515671179,-35.0843647071077)) ;
#55426=CARTESIAN_POINT('Ctrl Pts',(180.367281162788,505.281395127858,-35.0231602897937)) ;
#55427=CARTESIAN_POINT('Ctrl Pts',(180.311997303755,505.278027884774,-35.0107229876461)) ;
#55428=CARTESIAN_POINT('Ctrl Pts',(180.214757553672,505.272283117937,-34.993034322229)) ;
#55429=CARTESIAN_POINT('Ctrl Pts',(180.173021458832,505.26987377499,-34.9867630468717)) ;
#55430=CARTESIAN_POINT('Ctrl Pts',(180.10227508799,505.265917412238,-34.9783516391548)) ;
#55431=CARTESIAN_POINT('Ctrl Pts',(180.073364290604,505.264338521813,-34.9755344490615)) ;
#55432=CARTESIAN_POINT('Ctrl Pts',(179.996946110786,505.260257859883,-34.9697207093969)) ;
#55433=CARTESIAN_POINT('Ctrl Pts',(179.949379135104,505.257807667233,-34.9677599976293)) ;
#55434=CARTESIAN_POINT('Ctrl Pts',(179.752988343518,505.247908929112,-34.9664929693984)) ;
#55435=CARTESIAN_POINT('Ctrl Pts',(179.604521400592,505.240910782813,-34.9816982294533)) ;
#55436=CARTESIAN_POINT('Ctrl Pts',(179.374574098227,505.229366836633,-35.0308537664649)) ;
#55437=CARTESIAN_POINT('Ctrl Pts',(179.291385813054,505.225043858586,-35.0541995438076)) ;
#55438=CARTESIAN_POINT('Ctrl Pts',(179.161903251777,505.217905790038,-35.0995052109148)) ;
#55439=CARTESIAN_POINT('Ctrl Pts',(179.114533565336,505.215204220988,-35.1180809578454)) ;
#55440=CARTESIAN_POINT('Ctrl Pts',(179.016880644929,505.20941899721,-35.1606214027236)) ;
#55441=CARTESIAN_POINT('Ctrl Pts',(178.966785009288,505.206325608557,-35.1849109394923)) ;
#55442=CARTESIAN_POINT('Ctrl Pts',(178.811604740099,505.196325638273,-35.268097333245)) ;
#55443=CARTESIAN_POINT('Ctrl Pts',(178.710689149975,505.189174784485,-35.3342059919185)) ;
#55444=CARTESIAN_POINT('Ctrl Pts',(178.529513132168,505.175308823821,-35.4770866111379)) ;
#55445=CARTESIAN_POINT('Ctrl Pts',(178.448513295891,505.168634380227,-35.5522847288833)) ;
#55446=CARTESIAN_POINT('Ctrl Pts',(178.347828681236,505.160026280009,-35.6621096346609)) ;
#55447=CARTESIAN_POINT('Ctrl Pts',(178.322523015511,505.157833235595,-35.6913255909611)) ;
#55448=CARTESIAN_POINT('Ctrl Pts',(178.279421935928,505.154071062762,-35.7440198991991)) ;
#55449=CARTESIAN_POINT('Ctrl Pts',(178.261282946576,505.152480968429,-35.7671946376364)) ;
#55450=CARTESIAN_POINT('Ctrl Pts',(178.211446768641,505.148076875168,-35.8337646388747)) ;
#55451=CARTESIAN_POINT('Ctrl Pts',(178.180945123605,505.145335036363,-35.8780242378745)) ;
#55452=CARTESIAN_POINT('Ctrl Pts',(178.076637222254,505.135588865683,-36.0428616130159)) ;
#55453=CARTESIAN_POINT('Ctrl Pts',(178.013583893043,505.128924879494,-36.1697737966513)) ;
#55454=CARTESIAN_POINT('Ctrl Pts',(177.940576001184,505.118684694105,-36.3649147307929)) ;
#55455=CARTESIAN_POINT('Ctrl Pts',(177.920182288141,505.115339014052,-36.4287776684847)) ;
#55456=CARTESIAN_POINT('Ctrl Pts',(177.888987183786,505.109114088239,-36.5459469176096)) ;
#55457=CARTESIAN_POINT('Ctrl Pts',(177.877111785744,505.106270079784,-36.5989029907302)) ;
#55458=CARTESIAN_POINT('Ctrl Pts',(177.858072068449,505.100590457945,-36.7029395308634)) ;
#55459=CARTESIAN_POINT('Ctrl Pts',(177.850707694297,505.097763759575,-36.7539422858839)) ;
#55460=CARTESIAN_POINT('Ctrl Pts',(177.835212219268,505.08954075187,-36.8998499542524)) ;
#55461=CARTESIAN_POINT('Ctrl Pts',(177.831751415802,505.084003358379,-36.9951082483004)) ;
#55462=CARTESIAN_POINT('Ctrl Pts',(177.83868017466,505.071577020968,-37.2040713634775)) ;
#55463=CARTESIAN_POINT('Ctrl Pts',(177.851909360546,505.064653948259,-37.3173742040268)) ;
#55464=CARTESIAN_POINT('Ctrl Pts',(177.886697652542,505.054223387855,-37.4895963906249)) ;
#55465=CARTESIAN_POINT('Ctrl Pts',(177.901668740072,505.050609444951,-37.5496190689917)) ;
#55466=CARTESIAN_POINT('Ctrl Pts',(177.927935476712,505.045420003552,-37.6377779449765)) ;
#55467=CARTESIAN_POINT('Ctrl Pts',(177.937181561602,505.043749950309,-37.6664860034803)) ;
#55468=CARTESIAN_POINT('Ctrl Pts',(177.95885781082,505.040168131594,-37.7290340023793)) ;
#55469=CARTESIAN_POINT('Ctrl Pts',(177.971552469016,505.038270490356,-37.7627699197628)) ;
#55470=CARTESIAN_POINT('Ctrl Pts',(178.047602738773,505.027853259488,-37.9497914493535)) ;
#55471=CARTESIAN_POINT('Ctrl Pts',(178.128453652584,505.020097653723,-38.095312534693)) ;
#55472=CARTESIAN_POINT('Ctrl Pts',(178.278953832286,505.007558116924,-38.3025556108408)) ;
#55473=CARTESIAN_POINT('Ctrl Pts',(178.336724730834,505.003054955549,-38.3719919427473)) ;
#55474=CARTESIAN_POINT('Ctrl Pts',(178.434107430826,504.995710555175,-38.4744952105936)) ;
#55475=CARTESIAN_POINT('Ctrl Pts',(178.470717108393,504.992997867744,-38.5102555572575)) ;
#55476=CARTESIAN_POINT('Ctrl Pts',(178.549338706159,504.987243354291,-38.5815159802886)) ;
#55477=CARTESIAN_POINT('Ctrl Pts',(178.591517366953,504.984194287864,-38.6167701755253)) ;
#55478=CARTESIAN_POINT('Ctrl Pts',(178.759603259324,504.97216850995,-38.7461769621864)) ;
#55479=CARTESIAN_POINT('Ctrl Pts',(178.89472754835,504.962705481812,-38.8274445554859)) ;
#55480=CARTESIAN_POINT('Ctrl Pts',(179.095257837632,504.949475272808,-38.9186595863778)) ;
#55481=CARTESIAN_POINT('Ctrl Pts',(179.153929308183,504.945701104997,-38.9421479390222)) ;
#55482=CARTESIAN_POINT('Ctrl Pts',(179.256223917001,504.939377492616,-38.9777232330315)) ;
#55483=CARTESIAN_POINT('Ctrl Pts',(179.299336185575,504.936787934222,-38.9911418686249)) ;
#55484=CARTESIAN_POINT('Ctrl Pts',(179.370769502948,504.932658847094,-39.0108185696902)) ;
#55485=CARTESIAN_POINT('Ctrl Pts',(179.398838639979,504.931078355285,-39.017915823146)) ;
#55486=CARTESIAN_POINT('Ctrl Pts',(179.470007068975,504.927175004462,-39.0343184980821)) ;
#55487=CARTESIAN_POINT('Ctrl Pts',(179.513271321743,504.924892562287,-39.042834279208)) ;
#55488=CARTESIAN_POINT('Ctrl Pts',(179.690575515069,504.915784628321,-39.0718414103903)) ;
#55489=CARTESIAN_POINT('Ctrl Pts',(179.82621896306,504.909365180685,-39.0804364677486)) ;
#55490=CARTESIAN_POINT('Ctrl Pts',(180.061658190465,504.89789044222,-39.0720435930674)) ;
#55491=CARTESIAN_POINT('Ctrl Pts',(180.161187072156,504.892938588785,-39.061191888782)) ;
#55492=CARTESIAN_POINT('Ctrl Pts',(180.310511694759,504.885077487925,-39.0337800158408)) ;
#55493=CARTESIAN_POINT('Ctrl Pts',(180.361123731274,504.882337463574,-39.0224944500205)) ;
#55494=CARTESIAN_POINT('Ctrl Pts',(180.463267303572,504.876625428776,-38.9956253111134)) ;
#55495=CARTESIAN_POINT('Ctrl Pts',(180.514721208572,504.87365076055,-38.9799066252577)) ;
#55496=CARTESIAN_POINT('Ctrl Pts',(180.725184840137,504.861055860518,-38.9064658240645)) ;
#55497=CARTESIAN_POINT('Ctrl Pts',(180.877362673786,504.850843475642,-38.8312457951857)) ;
#55498=CARTESIAN_POINT('Ctrl Pts',(181.089366082257,504.83561987089,-38.6916417816203)) ;
#55499=CARTESIAN_POINT('Ctrl Pts',(181.157210572134,504.830584282341,-38.6406866091251)) ;
#55500=CARTESIAN_POINT('Ctrl Pts',(181.246042418268,504.823950332707,-38.5649411098106)) ;
#55501=CARTESIAN_POINT('Ctrl Pts',(181.269881555035,504.822166052496,-38.543633499697)) ;
#55502=CARTESIAN_POINT('Ctrl Pts',(181.31731634043,504.818625242278,-38.499201421119)) ;
#55503=CARTESIAN_POINT('Ctrl Pts',(181.340870923605,504.816871510371,-38.4760471234562)) ;
#55504=CARTESIAN_POINT('Ctrl Pts',(181.418504873589,504.811064661938,-38.395961894576)) ;
#55505=CARTESIAN_POINT('Ctrl Pts',(181.469879937113,504.807174807454,-38.3364996931447)) ;
#55506=CARTESIAN_POINT('Ctrl Pts',(181.517728902323,504.803342258844,-38.2742387482803)) ;
#55507=CARTESIAN_POINT('Origin',(179.888527625402,502.164639879998,-37.0221601717597)) ;
#55508=CARTESIAN_POINT('',(181.517263155791,504.105570724017,-38.2738081386943)) ;
#55509=CARTESIAN_POINT('',(181.517722816555,504.164527114775,-38.2742466670251)) ;
#55510=CARTESIAN_POINT('',(181.517728902316,502.164639879998,-38.2742387482878)) ;
#55511=CARTESIAN_POINT('',(179.888051515576,503.856489564609,-34.9674102269198)) ;
#55512=CARTESIAN_POINT('Ctrl Pts',(179.888012689102,503.857432638953,-34.9679547929697)) ;
#55513=CARTESIAN_POINT('Ctrl Pts',(179.958932145949,503.86150620242,-34.9680734899365)) ;
#55514=CARTESIAN_POINT('Ctrl Pts',(180.029892959977,503.865524608869,-34.9718370771033)) ;
#55515=CARTESIAN_POINT('Ctrl Pts',(180.100498384139,503.869458476652,-34.9792189466439)) ;
#55516=CARTESIAN_POINT('Ctrl Pts',(180.171085622775,503.873391331207,-34.986598914869)) ;
#55517=CARTESIAN_POINT('Ctrl Pts',(180.241317632988,503.877239660488,-34.9975952865709)) ;
#55518=CARTESIAN_POINT('Ctrl Pts',(180.310802165125,503.880998694863,-35.0121470101295)) ;
#55519=CARTESIAN_POINT('Ctrl Pts',(180.380292601802,503.884758048666,-35.0266999702401)) ;
#55520=CARTESIAN_POINT('Ctrl Pts',(180.449035362884,503.888428164958,-35.0448089803899)) ;
#55521=CARTESIAN_POINT('Ctrl Pts',(180.516642979013,503.892028550131,-35.0663778912399)) ;
#55522=CARTESIAN_POINT('Ctrl Pts',(180.584328547214,503.895633086574,-35.0879716712008)) ;
#55523=CARTESIAN_POINT('Ctrl Pts',(180.650876219736,503.899167916646,-35.1130335410347)) ;
#55524=CARTESIAN_POINT('Ctrl Pts',(180.715903572164,503.902675042469,-35.1414296045501)) ;
#55525=CARTESIAN_POINT('Ctrl Pts',(180.780971130696,503.906184336732,-35.169843225217)) ;
#55526=CARTESIAN_POINT('Ctrl Pts',(180.844516253085,503.909666237896,-35.2015954784639)) ;
#55527=CARTESIAN_POINT('Ctrl Pts',(180.90616488458,503.913181328988,-35.236510876872)) ;
#55528=CARTESIAN_POINT('Ctrl Pts',(180.964246578652,503.916493039897,-35.2694061000028)) ;
#55529=CARTESIAN_POINT('Ctrl Pts',(181.020645072211,503.919834702901,-35.305109425717)) ;
#55530=CARTESIAN_POINT('Ctrl Pts',(181.075057591808,503.923266837811,-35.3434349028281)) ;
#55531=CARTESIAN_POINT('Ctrl Pts',(181.078508092662,503.923484482289,-35.3458652643052)) ;
#55532=CARTESIAN_POINT('Ctrl Pts',(181.081950624698,503.923702490582,-35.348306171434)) ;
#55533=CARTESIAN_POINT('Ctrl Pts',(181.085385117762,503.923920878122,-35.3507575774486)) ;
#55534=CARTESIAN_POINT('Ctrl Pts',(181.122127294371,503.926257186113,-35.3769826974451)) ;
#55535=CARTESIAN_POINT('Ctrl Pts',(181.157947462091,503.928637131266,-35.4044082453032)) ;
#55536=CARTESIAN_POINT('Ctrl Pts',(181.192756181077,503.931080249462,-35.4329650866252)) ;
#55537=CARTESIAN_POINT('Ctrl Pts',(181.192783048711,503.93108213522,-35.432987128653)) ;
#55538=CARTESIAN_POINT('Ctrl Pts',(181.192809915743,503.931084021015,-35.4330091713548)) ;
#55539=CARTESIAN_POINT('Ctrl Pts',(181.192836782173,503.931085906848,-35.4330312147305)) ;
#55540=CARTESIAN_POINT('Ctrl Pts',(181.242591194344,503.93457831371,-35.4738537282965)) ;
#55541=CARTESIAN_POINT('Ctrl Pts',(181.290459790534,503.938209109013,-35.5171450374117)) ;
#55542=CARTESIAN_POINT('Ctrl Pts',(181.336212786875,503.9419132054,-35.5626840657719)) ;
#55543=CARTESIAN_POINT('Ctrl Pts',(181.340850913989,503.942288701461,-35.5673005022697)) ;
#55544=CARTESIAN_POINT('Ctrl Pts',(181.345467291612,503.942664950802,-35.5719399941601)) ;
#55545=CARTESIAN_POINT('Ctrl Pts',(181.350061675335,503.943041885617,-35.5766022817505)) ;
#55546=CARTESIAN_POINT('Ctrl Pts',(181.399900926299,503.947130823329,-35.62717814465)) ;
#55547=CARTESIAN_POINT('Ctrl Pts',(181.447153620298,503.95129980935,-35.6804422720945)) ;
#55548=CARTESIAN_POINT('Ctrl Pts',(181.491555882654,503.955474476342,-35.7360751787159)) ;
#55549=CARTESIAN_POINT('Ctrl Pts',(181.535903285675,503.959643985501,-35.7916393504567)) ;
#55550=CARTESIAN_POINT('Ctrl Pts',(181.577407628645,503.963818808005,-35.8495662641025)) ;
#55551=CARTESIAN_POINT('Ctrl Pts',(181.615842287979,503.967944206143,-35.909520218889)) ;
#55552=CARTESIAN_POINT('Ctrl Pts',(181.654251266563,503.972066847829,-35.9694341144542)) ;
#55553=CARTESIAN_POINT('Ctrl Pts',(181.689594824856,503.976139962293,-36.0313722785607)) ;
#55554=CARTESIAN_POINT('Ctrl Pts',(181.72167934075,503.980132110577,-36.0949840814907)) ;
#55555=CARTESIAN_POINT('Ctrl Pts',(181.753753201391,503.98412293307,-36.1585747589726)) ;
#55556=CARTESIAN_POINT('Ctrl Pts',(181.782570198983,503.98803280281,-36.2238379456552)) ;
#55557=CARTESIAN_POINT('Ctrl Pts',(181.807968141192,503.991855024412,-36.290408340099)) ;
#55558=CARTESIAN_POINT('Ctrl Pts',(181.833366183934,503.995677261144,-36.3569789980492)) ;
#55559=CARTESIAN_POINT('Ctrl Pts',(181.855345035104,503.999411913746,-36.4248568749306)) ;
#55560=CARTESIAN_POINT('Ctrl Pts',(181.873774463563,504.003076816851,-36.493661757878)) ;
#55561=CARTESIAN_POINT('Ctrl Pts',(181.892222348924,504.006745390323,-36.5625355482753)) ;
#55562=CARTESIAN_POINT('Ctrl Pts',(181.907113458668,504.010344252824,-36.6323382123433)) ;
#55563=CARTESIAN_POINT('Ctrl Pts',(181.918351807264,504.013914080483,-36.7026733581213)) ;
#55564=CARTESIAN_POINT('Ctrl Pts',(181.929596207887,504.017485830549,-36.7730463804734)) ;
#55565=CARTESIAN_POINT('Ctrl Pts',(181.937183521265,504.021028852069,-36.8439524401983)) ;
#55566=CARTESIAN_POINT('Ctrl Pts',(181.941056960413,504.024602862834,-36.9149794679936)) ;
#55567=CARTESIAN_POINT('Ctrl Pts',(181.944725011961,504.027987363073,-36.9822403153598)) ;
#55568=CARTESIAN_POINT('Ctrl Pts',(181.945062320629,504.031400143998,-37.0496099794262)) ;
#55569=CARTESIAN_POINT('Ctrl Pts',(181.942059490689,504.034902425056,-37.1167253075522)) ;
#55570=CARTESIAN_POINT('Ctrl Pts',(181.941885895529,504.035104893745,-37.1206052795714)) ;
#55571=CARTESIAN_POINT('Ctrl Pts',(181.941701144205,504.035307661548,-37.124484414397)) ;
#55572=CARTESIAN_POINT('Ctrl Pts',(181.941505237282,504.035510740295,-37.1283626466467)) ;
#55573=CARTESIAN_POINT('Ctrl Pts',(181.939333039661,504.037762458423,-37.1713641228339)) ;
#55574=CARTESIAN_POINT('Ctrl Pts',(181.935789371233,504.040052623498,-37.2142525851414)) ;
#55575=CARTESIAN_POINT('Ctrl Pts',(181.930881811781,504.042398035777,-37.2569307975213)) ;
#55576=CARTESIAN_POINT('Ctrl Pts',(181.930878006913,504.042399854193,-37.2569638862606)) ;
#55577=CARTESIAN_POINT('Ctrl Pts',(181.930874201226,504.042401672642,-37.256996974874)) ;
#55578=CARTESIAN_POINT('Ctrl Pts',(181.930870394719,504.042403491124,-37.2570300633614)) ;
#55579=CARTESIAN_POINT('Ctrl Pts',(181.923473697062,504.04593711499,-37.3213266881243)) ;
#55580=CARTESIAN_POINT('Ctrl Pts',(181.912949276553,504.049604849235,-37.3853667088768)) ;
#55581=CARTESIAN_POINT('Ctrl Pts',(181.899360286837,504.053341749049,-37.4488337623104)) ;
#55582=CARTESIAN_POINT('Ctrl Pts',(181.898033000868,504.053706745623,-37.4550328198782)) ;
#55583=CARTESIAN_POINT('Ctrl Pts',(181.896676507989,504.054072402047,-37.4612263827437)) ;
#55584=CARTESIAN_POINT('Ctrl Pts',(181.895290886591,504.054438657802,-37.4674141381045)) ;
#55585=CARTESIAN_POINT('Ctrl Pts',(181.879824271438,504.058526886249,-37.5364832438183)) ;
#55586=CARTESIAN_POINT('Ctrl Pts',(181.860724512427,504.062689049994,-37.6048325829169)) ;
#55587=CARTESIAN_POINT('Ctrl Pts',(181.838116440668,504.066853554458,-37.6720746691617)) ;
#55588=CARTESIAN_POINT('Ctrl Pts',(181.836915879813,504.067074702953,-37.6756454388162)) ;
#55589=CARTESIAN_POINT('Ctrl Pts',(181.8357054331,504.067295858049,-37.6792130763627)) ;
#55590=CARTESIAN_POINT('Ctrl Pts',(181.834485121803,504.067517009024,-37.6827775205824)) ;
#55591=CARTESIAN_POINT('Ctrl Pts',(181.811409853763,504.071698825614,-37.7501787697255)) ;
#55592=CARTESIAN_POINT('Ctrl Pts',(181.784805036596,504.075878961822,-37.8164423868943)) ;
#55593=CARTESIAN_POINT('Ctrl Pts',(181.75483274324,504.080004965875,-37.8811963347265)) ;
#55594=CARTESIAN_POINT('Ctrl Pts',(181.724880324253,504.084128234011,-37.9459073447735)) ;
#55595=CARTESIAN_POINT('Ctrl Pts',(181.691565026174,504.088197283791,-38.0091107813048)) ;
#55596=CARTESIAN_POINT('Ctrl Pts',(181.655079203746,504.092183056001,-38.0704541533036)) ;
#55597=CARTESIAN_POINT('Ctrl Pts',(181.618603297701,504.096167744928,-38.1317808529541)) ;
#55598=CARTESIAN_POINT('Ctrl Pts',(181.578958606656,504.100069169259,-38.1912484957397)) ;
#55599=CARTESIAN_POINT('Ctrl Pts',(181.53636686296,504.103882968901,-38.2485230005513)) ;
#55600=CARTESIAN_POINT('Ctrl Pts',(181.530063203674,504.104447418521,-38.2569997364823)) ;
#55601=CARTESIAN_POINT('Ctrl Pts',(181.523695043267,504.105009992972,-38.2654284654114)) ;
#55602=CARTESIAN_POINT('Ctrl Pts',(181.517263155791,504.105570724017,-38.2738081386943)) ;
#55603=CARTESIAN_POINT('',(177.903353299729,503.710565160536,-36.4919899545742)) ;
#55604=CARTESIAN_POINT('Ctrl Pts',(177.90335329973,503.710565160536,-36.4919899545744)) ;
#55605=CARTESIAN_POINT('Ctrl Pts',(177.922086669525,503.714501737535,-36.4218445492966)) ;
#55606=CARTESIAN_POINT('Ctrl Pts',(177.944559935843,503.718438314534,-36.3526262888013)) ;
#55607=CARTESIAN_POINT('Ctrl Pts',(177.970658359158,503.722374891533,-36.2847491329925)) ;
#55608=CARTESIAN_POINT('Ctrl Pts',(177.996735874362,503.72630831484,-36.2169263553011)) ;
#55609=CARTESIAN_POINT('Ctrl Pts',(178.026432607287,503.730241738147,-36.150442974721)) ;
#55610=CARTESIAN_POINT('Ctrl Pts',(178.059584450202,503.734175161454,-36.0856963847457)) ;
#55611=CARTESIAN_POINT('Ctrl Pts',(178.092726426208,503.738107414065,-36.0209690651541)) ;
#55612=CARTESIAN_POINT('Ctrl Pts',(178.129321265059,503.742039666676,-35.957977921458)) ;
#55613=CARTESIAN_POINT('Ctrl Pts',(178.169157796928,503.745971919287,-35.8970979710654)) ;
#55614=CARTESIAN_POINT('Ctrl Pts',(178.20898983709,503.749903728523,-35.8362248850971)) ;
#55615=CARTESIAN_POINT('Ctrl Pts',(178.25206259196,503.753835537759,-35.7774629049249)) ;
#55616=CARTESIAN_POINT('Ctrl Pts',(178.298121045655,503.757767346995,-35.7211588367889)) ;
#55617=CARTESIAN_POINT('Ctrl Pts',(178.344187323935,503.761699824182,-35.664845203504)) ;
#55618=CARTESIAN_POINT('Ctrl Pts',(178.39324001716,503.765632301368,-35.610990668463)) ;
#55619=CARTESIAN_POINT('Ctrl Pts',(178.444984140575,503.769564778555,-35.5599085621139)) ;
#55620=CARTESIAN_POINT('Ctrl Pts',(178.496751681291,503.773499035422,-35.5088033380654)) ;
#55621=CARTESIAN_POINT('Ctrl Pts',(178.551212744977,503.777433292289,-35.4604733594333)) ;
#55622=CARTESIAN_POINT('Ctrl Pts',(178.608036897457,503.781367549156,-35.4151937570061)) ;
#55623=CARTESIAN_POINT('Ctrl Pts',(178.664945234505,503.785307634596,-35.3698470731778)) ;
#55624=CARTESIAN_POINT('Ctrl Pts',(178.724223287277,503.789247720036,-35.3275600731401)) ;
#55625=CARTESIAN_POINT('Ctrl Pts',(178.785509441009,503.793187805476,-35.2885660879564)) ;
#55626=CARTESIAN_POINT('Ctrl Pts',(178.846846634949,503.79713117229,-35.2495396278827)) ;
#55627=CARTESIAN_POINT('Ctrl Pts',(178.910194859628,503.801074539104,-35.213811870712)) ;
#55628=CARTESIAN_POINT('Ctrl Pts',(178.975167853069,503.805017905918,-35.1815701878734)) ;
#55629=CARTESIAN_POINT('Ctrl Pts',(179.04026464019,503.808968786067,-35.1492670746407)) ;
#55630=CARTESIAN_POINT('Ctrl Pts',(179.106991954837,503.812919666216,-35.1204634808391)) ;
#55631=CARTESIAN_POINT('Ctrl Pts',(179.174943925636,503.816870546365,-35.0952985093853)) ;
#55632=CARTESIAN_POINT('Ctrl Pts',(179.203132609039,503.818509499708,-35.0848592622994)) ;
#55633=CARTESIAN_POINT('Ctrl Pts',(179.231531870175,503.820148453051,-35.0750455736566)) ;
#55634=CARTESIAN_POINT('Ctrl Pts',(179.260112136805,503.821787406393,-35.0658648115978)) ;
#55635=CARTESIAN_POINT('Ctrl Pts',(179.339468635472,503.826338154658,-35.0403733373046)) ;
#55636=CARTESIAN_POINT('Ctrl Pts',(179.420464141971,503.830888902922,-35.0196867084889)) ;
#55637=CARTESIAN_POINT('Ctrl Pts',(179.502557616501,503.835439651186,-35.0039865630905)) ;
#55638=CARTESIAN_POINT('Ctrl Pts',(179.583771084385,503.839941617392,-34.9884547164807)) ;
#55639=CARTESIAN_POINT('Ctrl Pts',(179.666058990972,503.844443583597,-34.9778031051609)) ;
#55640=CARTESIAN_POINT('Ctrl Pts',(179.748876364633,503.848945549802,-34.9721613698416)) ;
#55641=CARTESIAN_POINT('Ctrl Pts',(179.795135818443,503.851460221404,-34.969010055294)) ;
#55642=CARTESIAN_POINT('Ctrl Pts',(179.841560097023,503.853974893007,-34.9674209995305)) ;
#55643=CARTESIAN_POINT('Ctrl Pts',(179.888051515576,503.856489564609,-34.9674102269198)) ;
#55644=CARTESIAN_POINT('',(177.901969296448,503.711777422211,-37.5551703732902)) ;
#55645=CARTESIAN_POINT('Origin',(179.888527625402,503.710565160536,-37.0221601717597)) ;
#55646=CARTESIAN_POINT('Ctrl Pts',(177.903947533684,503.712975317057,-37.5545504628579)) ;
#55647=CARTESIAN_POINT('Ctrl Pts',(177.895757318976,503.714684508975,-37.5240199717342)) ;
#55648=CARTESIAN_POINT('Ctrl Pts',(177.888272211867,503.716353732618,-37.4933026915394)) ;
#55649=CARTESIAN_POINT('Ctrl Pts',(177.843255876735,503.727245875368,-37.2880864789864)) ;
#55650=CARTESIAN_POINT('Ctrl Pts',(177.827886420719,503.735545865294,-37.1094919839223)) ;
#55651=CARTESIAN_POINT('Ctrl Pts',(177.838765269825,503.747636894902,-36.8641427975573)) ;
#55652=CARTESIAN_POINT('Ctrl Pts',(177.845014145554,503.750992058744,-36.7973337620819)) ;
#55653=CARTESIAN_POINT('Ctrl Pts',(177.862161052059,503.757215308265,-36.6775667803755)) ;
#55654=CARTESIAN_POINT('Ctrl Pts',(177.871902648708,503.760047275435,-36.6245056818421)) ;
#55655=CARTESIAN_POINT('Ctrl Pts',(177.895145194004,503.765750615555,-36.5210187901725)) ;
#55656=CARTESIAN_POINT('Ctrl Pts',(177.908502449703,503.768615418516,-36.4706025512604)) ;
#55657=CARTESIAN_POINT('Ctrl Pts',(177.975574149277,503.781473142358,-36.2514832390895)) ;
#55658=CARTESIAN_POINT('Ctrl Pts',(178.049037690473,503.792136946426,-36.0896420780475)) ;
#55659=CARTESIAN_POINT('Ctrl Pts',(178.185397305171,503.807602824018,-35.8697578075168)) ;
#55660=CARTESIAN_POINT('Ctrl Pts',(178.232606658886,503.812442541399,-35.8028931647587)) ;
#55661=CARTESIAN_POINT('Ctrl Pts',(178.303541268729,503.818884373362,-35.7141741542682)) ;
#55662=CARTESIAN_POINT('Ctrl Pts',(178.32397899941,503.820656440321,-35.6897949466128)) ;
#55663=CARTESIAN_POINT('Ctrl Pts',(178.366968887714,503.824199102932,-35.6408684796157)) ;
#55664=CARTESIAN_POINT('Ctrl Pts',(178.389568592076,503.825965686983,-35.6163757531014)) ;
#55665=CARTESIAN_POINT('Ctrl Pts',(178.504372626142,503.834541364303,-35.4978736541451)) ;
#55666=CARTESIAN_POINT('Ctrl Pts',(178.604877938666,503.840838577507,-35.4123199716945)) ;
#55667=CARTESIAN_POINT('Ctrl Pts',(178.781952523299,503.85128445912,-35.28878769492)) ;
#55668=CARTESIAN_POINT('Ctrl Pts',(178.853909444624,503.855376072505,-35.2449002551313)) ;
#55669=CARTESIAN_POINT('Ctrl Pts',(178.987124614945,503.862923219619,-35.1744888603364)) ;
#55670=CARTESIAN_POINT('Ctrl Pts',(179.047364616602,503.866325870217,-35.1462976245517)) ;
#55671=CARTESIAN_POINT('Ctrl Pts',(179.154683211678,503.872440948625,-35.1022844643679)) ;
#55672=CARTESIAN_POINT('Ctrl Pts',(179.201166385959,503.875105718216,-35.0851562241228)) ;
#55673=CARTESIAN_POINT('Ctrl Pts',(179.308922577701,503.881338604638,-35.0498172445049)) ;
#55674=CARTESIAN_POINT('Ctrl Pts',(179.370514853924,503.884941773821,-35.0327531875673)) ;
#55675=CARTESIAN_POINT('Ctrl Pts',(179.575985296009,503.897092887691,-34.9860171575838)) ;
#55676=CARTESIAN_POINT('Ctrl Pts',(179.722241991841,503.905985140548,-34.9688940738769)) ;
#55677=CARTESIAN_POINT('Ctrl Pts',(179.945711503131,503.919331392535,-34.9667758221378)) ;
#55678=CARTESIAN_POINT('Ctrl Pts',(180.022358683162,503.92385672602,-34.9703400004801)) ;
#55679=CARTESIAN_POINT('Ctrl Pts',(180.129951961443,503.929985952611,-34.981399747356)) ;
#55680=CARTESIAN_POINT('Ctrl Pts',(180.161195612573,503.931738654782,-34.985338797295)) ;
#55681=CARTESIAN_POINT('Ctrl Pts',(180.225345320032,503.935264138454,-34.9949292578328)) ;
#55682=CARTESIAN_POINT('Ctrl Pts',(180.258228797664,503.937031953938,-35.0006674890449)) ;
#55683=CARTESIAN_POINT('Ctrl Pts',(180.398909995285,503.944480758777,-35.0287647137643)) ;
#55684=CARTESIAN_POINT('Ctrl Pts',(180.504964254677,503.949812065802,-35.0589672768675)) ;
#55685=CARTESIAN_POINT('Ctrl Pts',(180.734904791795,503.96167731295,-35.1449357705221)) ;
#55686=CARTESIAN_POINT('Ctrl Pts',(180.856706846891,503.968192899056,-35.2047577744652)) ;
#55687=CARTESIAN_POINT('Ctrl Pts',(181.018162071795,503.977916870129,-35.3049216227501)) ;
#55688=CARTESIAN_POINT('Ctrl Pts',(181.063415632662,503.980771990906,-35.3355601434682)) ;
#55689=CARTESIAN_POINT('Ctrl Pts',(181.14791631304,503.98639316946,-35.3978229287159)) ;
#55690=CARTESIAN_POINT('Ctrl Pts',(181.187326581644,503.989146561038,-35.4291592364038)) ;
#55691=CARTESIAN_POINT('Ctrl Pts',(181.290653110701,503.996747493691,-35.5177022235187)) ;
#55692=CARTESIAN_POINT('Ctrl Pts',(181.352198477477,504.001701434117,-35.5775099068324)) ;
#55693=CARTESIAN_POINT('Ctrl Pts',(181.50888619033,504.015475938451,-35.7500931092957)) ;
#55694=CARTESIAN_POINT('Ctrl Pts',(181.595916942229,504.024501712009,-35.8695390577769)) ;
#55695=CARTESIAN_POINT('Ctrl Pts',(181.693611264494,504.035990679966,-36.0392957004221)) ;
#55696=CARTESIAN_POINT('Ctrl Pts',(181.716307480542,504.038786800327,-36.0821755785117)) ;
#55697=CARTESIAN_POINT('Ctrl Pts',(181.750047002402,504.043112868775,-36.1517723911939)) ;
#55698=CARTESIAN_POINT('Ctrl Pts',(181.762080021379,504.044694575938,-36.177985425348)) ;
#55699=CARTESIAN_POINT('Ctrl Pts',(181.789687483722,504.048417407049,-36.2416275199888)) ;
#55700=CARTESIAN_POINT('Ctrl Pts',(181.804713438876,504.05052876669,-36.2792790178148)) ;
#55701=CARTESIAN_POINT('Ctrl Pts',(181.856432654011,504.058221709834,-36.4209101990515)) ;
#55702=CARTESIAN_POINT('Ctrl Pts',(181.885855751607,504.063520368856,-36.527351265362)) ;
#55703=CARTESIAN_POINT('Ctrl Pts',(181.930309792158,504.074954462313,-36.7594548453065)) ;
#55704=CARTESIAN_POINT('Ctrl Pts',(181.942577323793,504.081086582172,-36.8851760842744)) ;
#55705=CARTESIAN_POINT('Ctrl Pts',(181.943529751982,504.090301579191,-37.0640377043029)) ;
#55706=CARTESIAN_POINT('Ctrl Pts',(181.94177426379,504.09307953441,-37.1168440458725)) ;
#55707=CARTESIAN_POINT('Ctrl Pts',(181.93426333949,504.098718328245,-37.2213040161704)) ;
#55708=CARTESIAN_POINT('Ctrl Pts',(181.928579104961,504.101574859447,-37.2729233005051)) ;
#55709=CARTESIAN_POINT('Ctrl Pts',(181.905379487788,504.110441702532,-37.4289973928072)) ;
#55710=CARTESIAN_POINT('Ctrl Pts',(181.881742716806,504.116639518345,-37.5323528521412)) ;
#55711=CARTESIAN_POINT('Ctrl Pts',(181.805672544406,504.1319099548,-37.7764875068448)) ;
#55712=CARTESIAN_POINT('Ctrl Pts',(181.745574868745,504.141078223086,-37.9142545955288)) ;
#55713=CARTESIAN_POINT('Ctrl Pts',(181.654336389126,504.151553830523,-38.0733703472624)) ;
#55714=CARTESIAN_POINT('Ctrl Pts',(181.636933944431,504.153436387901,-38.1020671416748)) ;
#55715=CARTESIAN_POINT('Ctrl Pts',(181.604570192788,504.156721147625,-38.1526003889469)) ;
#55716=CARTESIAN_POINT('Ctrl Pts',(181.58987603404,504.158139461567,-38.1745970845128)) ;
#55717=CARTESIAN_POINT('Ctrl Pts',(181.556362419459,504.16123077008,-38.2227272559929)) ;
#55718=CARTESIAN_POINT('Ctrl Pts',(181.537344535028,504.162891887699,-38.2487151965558)) ;
#55719=CARTESIAN_POINT('Ctrl Pts',(181.517722816555,504.164527114775,-38.2742466670251)) ;
#55720=CARTESIAN_POINT('Origin',(29.8885276254015,502.164639880024,-37.0221601717529)) ;
#55721=CARTESIAN_POINT('',(31.5177152522353,505.503079332004,-38.2742565095294)) ;
#55722=CARTESIAN_POINT('',(31.517715239327,505.561197820373,-38.2742565263254)) ;
#55723=CARTESIAN_POINT('',(31.5177152522233,502.164639880024,-38.2742565095444)) ;
#55724=CARTESIAN_POINT('',(29.0652954452959,505.710565160562,-38.9047876814153)) ;
#55725=CARTESIAN_POINT('Ctrl Pts',(31.517715239327,505.561197820373,-38.2742565263254)) ;
#55726=CARTESIAN_POINT('Ctrl Pts',(31.5075491635084,505.562168759122,-38.2874842980902)) ;
#55727=CARTESIAN_POINT('Ctrl Pts',(31.4972210708087,505.563144379345,-38.3005894529987)) ;
#55728=CARTESIAN_POINT('Ctrl Pts',(31.4015822254585,505.57207825581,-38.4189489716371)) ;
#55729=CARTESIAN_POINT('Ctrl Pts',(31.3062234691222,505.580301471493,-38.5156423553119)) ;
#55730=CARTESIAN_POINT('Ctrl Pts',(31.1611448810046,505.59137763975,-38.636245616164)) ;
#55731=CARTESIAN_POINT('Ctrl Pts',(31.1189359034847,505.594450738869,-38.6686482014559)) ;
#55732=CARTESIAN_POINT('Ctrl Pts',(31.0511435592626,505.599100143542,-38.7166256158861)) ;
#55733=CARTESIAN_POINT('Ctrl Pts',(31.0263991082161,505.600739734931,-38.7333404097893)) ;
#55734=CARTESIAN_POINT('Ctrl Pts',(30.9670432512362,505.604531093695,-38.7715776913673)) ;
#55735=CARTESIAN_POINT('Ctrl Pts',(30.9321403781093,505.606655089118,-38.7926207042398)) ;
#55736=CARTESIAN_POINT('Ctrl Pts',(30.8014997273251,505.614306047177,-38.866177211694)) ;
#55737=CARTESIAN_POINT('Ctrl Pts',(30.7022411842305,505.61955169095,-38.9120784274336)) ;
#55738=CARTESIAN_POINT('Ctrl Pts',(30.4737700196624,505.63127542291,-38.9963775917003)) ;
#55739=CARTESIAN_POINT('Ctrl Pts',(30.3434963493631,505.637745073186,-39.0304039139251)) ;
#55740=CARTESIAN_POINT('Ctrl Pts',(30.1521214543254,505.647634681118,-39.0607995658369)) ;
#55741=CARTESIAN_POINT('Ctrl Pts',(30.0930310772155,505.650735445744,-39.0675720472511)) ;
#55742=CARTESIAN_POINT('Ctrl Pts',(29.9778760565012,505.656907225942,-39.0757302690794)) ;
#55743=CARTESIAN_POINT('Ctrl Pts',(29.9218840845969,505.659966780814,-39.0774022115405)) ;
#55744=CARTESIAN_POINT('Ctrl Pts',(29.7389595994745,505.670169006103,-39.0753873946209)) ;
#55745=CARTESIAN_POINT('Ctrl Pts',(29.6124387002168,505.677569456498,-39.0622289706628)) ;
#55746=CARTESIAN_POINT('Ctrl Pts',(29.3834454037262,505.691317622877,-39.0167136061039)) ;
#55747=CARTESIAN_POINT('Ctrl Pts',(29.2807041840142,505.697616119117,-38.987841832375)) ;
#55748=CARTESIAN_POINT('Ctrl Pts',(29.159114743818,505.704960070217,-38.9432226974015)) ;
#55749=CARTESIAN_POINT('Ctrl Pts',(29.1377005136105,505.706248825033,-38.9349547506654)) ;
#55750=CARTESIAN_POINT('Ctrl Pts',(29.0992885979274,505.708547178493,-38.9193795582333)) ;
#55751=CARTESIAN_POINT('Ctrl Pts',(29.0822426517464,505.709562273817,-38.9121983272501)) ;
#55752=CARTESIAN_POINT('Ctrl Pts',(29.0652954452959,505.710565160562,-38.9047876814153)) ;
#55753=CARTESIAN_POINT('',(28.2343942282376,505.709323904328,-38.2446969949844)) ;
#55754=CARTESIAN_POINT('Origin',(29.8885276254021,505.710565160562,-37.0221601717529)) ;
#55755=CARTESIAN_POINT('Ctrl Pts',(28.2362648420351,505.708082648095,-38.2436450292932)) ;
#55756=CARTESIAN_POINT('Ctrl Pts',(28.2461072735545,505.707189028891,-38.2569585658441)) ;
#55757=CARTESIAN_POINT('Ctrl Pts',(28.2561106100166,505.706306272621,-38.2701531255639)) ;
#55758=CARTESIAN_POINT('Ctrl Pts',(28.2797687895217,505.704273173126,-38.3005873852562)) ;
#55759=CARTESIAN_POINT('Ctrl Pts',(28.2935432205994,505.703130197476,-38.3177318410642)) ;
#55760=CARTESIAN_POINT('Ctrl Pts',(28.3874565500433,505.695579706726,-38.4308533050305)) ;
#55761=CARTESIAN_POINT('Ctrl Pts',(28.4759436690462,505.689601034009,-38.5195722420282)) ;
#55762=CARTESIAN_POINT('Ctrl Pts',(28.6616888882861,505.677871318706,-38.6745901535631)) ;
#55763=CARTESIAN_POINT('Ctrl Pts',(28.7576429151489,505.672149633239,-38.7416817700842)) ;
#55764=CARTESIAN_POINT('Ctrl Pts',(28.9046092534273,505.663388774374,-38.8267953063175)) ;
#55765=CARTESIAN_POINT('Ctrl Pts',(28.9514528702694,505.660599470974,-38.8515572194649)) ;
#55766=CARTESIAN_POINT('Ctrl Pts',(29.046854653936,505.654895369001,-38.8973611838619)) ;
#55767=CARTESIAN_POINT('Ctrl Pts',(29.0953728605494,505.651982990702,-38.9183924936482)) ;
#55768=CARTESIAN_POINT('Ctrl Pts',(29.2471311335853,505.642823163637,-38.9773317225558)) ;
#55769=CARTESIAN_POINT('Ctrl Pts',(29.3526338881399,505.636374314102,-39.0088402662777)) ;
#55770=CARTESIAN_POINT('Ctrl Pts',(29.5540611870938,505.624077896448,-39.0517789010217)) ;
#55771=CARTESIAN_POINT('Ctrl Pts',(29.6492724358515,505.618275709019,-39.0651915525782)) ;
#55772=CARTESIAN_POINT('Ctrl Pts',(29.7864911376515,505.610158775639,-39.0747950590716)) ;
#55773=CARTESIAN_POINT('Ctrl Pts',(29.827989899536,505.607736916038,-39.076437897636)) ;
#55774=CARTESIAN_POINT('Ctrl Pts',(29.9039863067478,505.603393910383,-39.0771412359856)) ;
#55775=CARTESIAN_POINT('Ctrl Pts',(29.9384655742036,505.601458246651,-39.0765926141257)) ;
#55776=CARTESIAN_POINT('Ctrl Pts',(30.0039453381849,505.597869070187,-39.0739010684627)) ;
#55777=CARTESIAN_POINT('Ctrl Pts',(30.0349411926149,505.596208888362,-39.0719223766892)) ;
#55778=CARTESIAN_POINT('Ctrl Pts',(30.1377728071355,505.590798020501,-39.0630133279018)) ;
#55779=CARTESIAN_POINT('Ctrl Pts',(30.2092929813512,505.587190485173,-39.0530014143618)) ;
#55780=CARTESIAN_POINT('Ctrl Pts',(30.4436935426478,505.575472247853,-39.0074927039831)) ;
#55781=CARTESIAN_POINT('Ctrl Pts',(30.6027687905733,505.567637529545,-38.9559686275298)) ;
#55782=CARTESIAN_POINT('Ctrl Pts',(30.8080671253967,505.556169459069,-38.8606415929312)) ;
#55783=CARTESIAN_POINT('Ctrl Pts',(30.8611267158057,505.55307722102,-38.8331314403171)) ;
#55784=CARTESIAN_POINT('Ctrl Pts',(30.9560853312287,505.547254960259,-38.7785197094462)) ;
#55785=CARTESIAN_POINT('Ctrl Pts',(30.9983410067869,505.544552403246,-38.7521289382581)) ;
#55786=CARTESIAN_POINT('Ctrl Pts',(31.0999911331131,505.537752606351,-38.6833855875682)) ;
#55787=CARTESIAN_POINT('Ctrl Pts',(31.1581656446523,505.533593522434,-38.6393587383011)) ;
#55788=CARTESIAN_POINT('Ctrl Pts',(31.3262527658227,505.520759757052,-38.4974807879345)) ;
#55789=CARTESIAN_POINT('Ctrl Pts',(31.4281137130496,505.511800710465,-38.3908431607179)) ;
#55790=CARTESIAN_POINT('Ctrl Pts',(31.5177152522354,505.503079332004,-38.2742565095294)) ;
#55791=CARTESIAN_POINT('Origin',(29.8885276254015,502.164639880024,-37.0221601717529)) ;
#55792=CARTESIAN_POINT('',(31.5177152522275,504.803366924184,-38.2742565095395)) ;
#55793=CARTESIAN_POINT('',(31.5177151883675,504.861461047188,-38.2742565926321)) ;
#55794=CARTESIAN_POINT('',(31.5177152522233,502.164639880024,-38.2742565095444)) ;
#55795=CARTESIAN_POINT('',(29.8879422111462,505.313162079696,-34.9674106910863)) ;
#55796=CARTESIAN_POINT('Ctrl Pts',(31.5177151883675,504.861461047188,-38.2742565926321)) ;
#55797=CARTESIAN_POINT('Ctrl Pts',(31.4981288392375,504.863080078642,-38.2997417197153)) ;
#55798=CARTESIAN_POINT('Ctrl Pts',(31.4779403354198,504.864717676193,-38.3247726904712)) ;
#55799=CARTESIAN_POINT('Ctrl Pts',(31.4229841836044,504.869108417019,-38.389727759927)) ;
#55800=CARTESIAN_POINT('Ctrl Pts',(31.3872577899705,504.871896629293,-38.428789209312)) ;
#55801=CARTESIAN_POINT('Ctrl Pts',(31.3127084554957,504.877617517573,-38.504230083968)) ;
#55802=CARTESIAN_POINT('Ctrl Pts',(31.2739013978775,504.880548583038,-38.5405675691751)) ;
#55803=CARTESIAN_POINT('Ctrl Pts',(31.1114993158224,504.892653281833,-38.6812218976206)) ;
#55804=CARTESIAN_POINT('Ctrl Pts',(30.977213607994,504.902365127006,-38.7722722982688)) ;
#55805=CARTESIAN_POINT('Ctrl Pts',(30.775739907595,504.915998408535,-38.8766437564329)) ;
#55806=CARTESIAN_POINT('Ctrl Pts',(30.7164040375659,504.919902391153,-38.9038818298611)) ;
#55807=CARTESIAN_POINT('Ctrl Pts',(30.6131208359359,504.926410452218,-38.9454609649906)) ;
#55808=CARTESIAN_POINT('Ctrl Pts',(30.5698010780222,504.929057339692,-38.9612291199981)) ;
#55809=CARTESIAN_POINT('Ctrl Pts',(30.4982885612648,504.93325235498,-38.9845663290332)) ;
#55810=CARTESIAN_POINT('Ctrl Pts',(30.4704044295927,504.934843976556,-38.9930142893482)) ;
#55811=CARTESIAN_POINT('Ctrl Pts',(30.4000362826776,504.938751291701,-39.0127095219153)) ;
#55812=CARTESIAN_POINT('Ctrl Pts',(30.3573554881974,504.941027422794,-39.0231921079112)) ;
#55813=CARTESIAN_POINT('Ctrl Pts',(30.174725418928,504.950495875648,-39.0618816537634)) ;
#55814=CARTESIAN_POINT('Ctrl Pts',(30.0323705460408,504.957231637499,-39.0768349300546)) ;
#55815=CARTESIAN_POINT('Ctrl Pts',(29.7942445336737,504.968856210848,-39.0769599584486)) ;
#55816=CARTESIAN_POINT('Ctrl Pts',(29.6990022579582,504.973596036018,-39.070371367097)) ;
#55817=CARTESIAN_POINT('Ctrl Pts',(29.5532879585618,504.98122573199,-39.0500390639636)) ;
#55818=CARTESIAN_POINT('Ctrl Pts',(29.5022999535718,504.983966801187,-39.0409484153902)) ;
#55819=CARTESIAN_POINT('Ctrl Pts',(29.3981895478093,504.989737809555,-39.0182980496468)) ;
#55820=CARTESIAN_POINT('Ctrl Pts',(29.3451578055391,504.992773019505,-39.0045189385599)) ;
#55821=CARTESIAN_POINT('Ctrl Pts',(29.2285873250816,504.999669504526,-38.9692015513979)) ;
#55822=CARTESIAN_POINT('Ctrl Pts',(29.1654263786983,505.003560027214,-38.9466379259184)) ;
#55823=CARTESIAN_POINT('Ctrl Pts',(28.9701919727207,505.016033904202,-38.8659229178025)) ;
#55824=CARTESIAN_POINT('Ctrl Pts',(28.8430800448016,505.024855683166,-38.796938435276)) ;
#55825=CARTESIAN_POINT('Ctrl Pts',(28.6823138706657,505.036331665862,-38.6863823069992)) ;
#55826=CARTESIAN_POINT('Ctrl Pts',(28.6414674940954,505.039274614431,-38.6559988319908)) ;
#55827=CARTESIAN_POINT('Ctrl Pts',(28.5788053219365,505.043780856716,-38.6056670649222)) ;
#55828=CARTESIAN_POINT('Ctrl Pts',(28.5562210606389,505.045401832638,-38.5867131976417)) ;
#55829=CARTESIAN_POINT('Ctrl Pts',(28.5040213635981,505.049134190153,-38.5409539373917)) ;
#55830=CARTESIAN_POINT('Ctrl Pts',(28.4747655129482,505.051219069491,-38.5137597226582)) ;
#55831=CARTESIAN_POINT('Ctrl Pts',(28.367434140807,505.058924077578,-38.4079947538045)) ;
#55832=CARTESIAN_POINT('Ctrl Pts',(28.2949566488903,505.064252121472,-38.3240043771201)) ;
#55833=CARTESIAN_POINT('Ctrl Pts',(28.1545170054817,505.075773328517,-38.1318429710699)) ;
#55834=CARTESIAN_POINT('Ctrl Pts',(28.0891451551578,505.081962757305,-38.022364013775)) ;
#55835=CARTESIAN_POINT('Ctrl Pts',(28.0113738670124,505.091266539733,-37.8594937474548)) ;
#55836=CARTESIAN_POINT('Ctrl Pts',(27.9903045640372,505.094069474289,-37.8105650598151)) ;
#55837=CARTESIAN_POINT('Ctrl Pts',(27.952160217412,505.099787195104,-37.7115598519733)) ;
#55838=CARTESIAN_POINT('Ctrl Pts',(27.9350710232107,505.102698793676,-37.6615326971442)) ;
#55839=CARTESIAN_POINT('Ctrl Pts',(27.8867640559,505.112187590116,-37.5000078895508)) ;
#55840=CARTESIAN_POINT('Ctrl Pts',(27.8630323962951,505.118999437547,-37.3865206407382)) ;
#55841=CARTESIAN_POINT('Ctrl Pts',(27.8326085890627,505.134013313537,-37.1378134512963)) ;
#55842=CARTESIAN_POINT('Ctrl Pts',(27.8294495923459,505.142226304971,-37.0026827339092)) ;
#55843=CARTESIAN_POINT('Ctrl Pts',(27.8421989123527,505.151984546786,-36.8329942994246)) ;
#55844=CARTESIAN_POINT('Ctrl Pts',(27.8457528177593,505.153973832392,-36.7978471027659)) ;
#55845=CARTESIAN_POINT('Ctrl Pts',(27.8540837367395,505.157597892617,-36.7323725571569)) ;
#55846=CARTESIAN_POINT('Ctrl Pts',(27.8586372679264,505.159242400686,-36.7020289675269)) ;
#55847=CARTESIAN_POINT('Ctrl Pts',(27.875234421428,505.164357693097,-36.6061180427956)) ;
#55848=CARTESIAN_POINT('Ctrl Pts',(27.8897904153988,505.167707933541,-36.5410243868138)) ;
#55849=CARTESIAN_POINT('Ctrl Pts',(27.9434616400019,505.177671969424,-36.3460800042188)) ;
#55850=CARTESIAN_POINT('Ctrl Pts',(27.9922763839509,505.184077751913,-36.2192909156471)) ;
#55851=CARTESIAN_POINT('Ctrl Pts',(28.0879134531826,505.194594048104,-36.0293164469265)) ;
#55852=CARTESIAN_POINT('Ctrl Pts',(28.1264562467776,505.198490804028,-35.9624182742105)) ;
#55853=CARTESIAN_POINT('Ctrl Pts',(28.1961091597132,505.205145417817,-35.8558700498401)) ;
#55854=CARTESIAN_POINT('Ctrl Pts',(28.2250777124948,505.207821638959,-35.8149126029029)) ;
#55855=CARTESIAN_POINT('Ctrl Pts',(28.2907357308412,505.213723078796,-35.7289369255706)) ;
#55856=CARTESIAN_POINT('Ctrl Pts',(28.3278927579695,505.21696604294,-35.6843324016277)) ;
#55857=CARTESIAN_POINT('Ctrl Pts',(28.4114477775995,505.224068857127,-35.5922545232644)) ;
#55858=CARTESIAN_POINT('Ctrl Pts',(28.4583584232185,505.227946905042,-35.5453359090442)) ;
#55859=CARTESIAN_POINT('Ctrl Pts',(28.6090525556392,505.2400312187,-35.4085399603043)) ;
#55860=CARTESIAN_POINT('Ctrl Pts',(28.7196318187401,505.248423732633,-35.3267228092832)) ;
#55861=CARTESIAN_POINT('Ctrl Pts',(28.8802171211402,505.259404735925,-35.2311341015567)) ;
#55862=CARTESIAN_POINT('Ctrl Pts',(28.9238066828535,505.26227305394,-35.2072831153994)) ;
#55863=CARTESIAN_POINT('Ctrl Pts',(28.9944447630443,505.266696358429,-35.1718970397575)) ;
#55864=CARTESIAN_POINT('Ctrl Pts',(29.020946590006,505.268305835211,-35.1593232858362)) ;
#55865=CARTESIAN_POINT('Ctrl Pts',(29.0857306034042,505.272117860183,-35.1302694469521)) ;
#55866=CARTESIAN_POINT('Ctrl Pts',(29.1242604351063,505.274288569587,-35.1143788115343)) ;
#55867=CARTESIAN_POINT('Ctrl Pts',(29.2674528017067,505.282097454294,-35.0603580956463)) ;
#55868=CARTESIAN_POINT('Ctrl Pts',(29.3746877541625,505.287456545371,-35.0295805341481)) ;
#55869=CARTESIAN_POINT('Ctrl Pts',(29.5710591498126,505.297175520829,-34.9901376900022)) ;
#55870=CARTESIAN_POINT('Ctrl Pts',(29.6592638939451,505.301507515347,-34.9783063252283)) ;
#55871=CARTESIAN_POINT('Ctrl Pts',(29.7945505680441,505.308336201423,-34.9690290583049)) ;
#55872=CARTESIAN_POINT('Ctrl Pts',(29.841239982547,505.310725012016,-34.9674235888564)) ;
#55873=CARTESIAN_POINT('Ctrl Pts',(29.8879409844869,505.313161259658,-34.9674102554973)) ;
#55874=CARTESIAN_POINT('Ctrl Pts',(29.887942250361,505.313161325695,-34.9674102551363)) ;
#55875=CARTESIAN_POINT('Ctrl Pts',(29.931406367057,505.315428715769,-34.9673978727004)) ;
#55876=CARTESIAN_POINT('Ctrl Pts',(29.9748581011214,505.317735983423,-34.9687645769083)) ;
#55877=CARTESIAN_POINT('Ctrl Pts',(30.0700919010336,505.322898407409,-34.9747881630337)) ;
#55878=CARTESIAN_POINT('Ctrl Pts',(30.1218045219554,505.325770716653,-34.9800340927953)) ;
#55879=CARTESIAN_POINT('Ctrl Pts',(30.334287187648,505.337878376111,-35.0097652070976)) ;
#55880=CARTESIAN_POINT('Ctrl Pts',(30.4920496847355,505.34765765226,-35.0513278068641)) ;
#55881=CARTESIAN_POINT('Ctrl Pts',(30.7304100775754,505.363062359331,-35.1454566553703)) ;
#55882=CARTESIAN_POINT('Ctrl Pts',(30.8151350119253,505.368659702266,-35.1858094976814)) ;
#55883=CARTESIAN_POINT('Ctrl Pts',(30.9251968312958,505.375848723428,-35.2477939194235)) ;
#55884=CARTESIAN_POINT('Ctrl Pts',(30.9531977633756,505.377669473963,-35.2644524325701)) ;
#55885=CARTESIAN_POINT('Ctrl Pts',(31.0091429552209,505.381271848921,-35.2995635466388)) ;
#55886=CARTESIAN_POINT('Ctrl Pts',(31.0370557630183,505.383051193532,-35.3180471310376)) ;
#55887=CARTESIAN_POINT('Ctrl Pts',(31.1712081834549,505.391577547857,-35.4116759925704)) ;
#55888=CARTESIAN_POINT('Ctrl Pts',(31.2706067671416,505.397828971673,-35.4961217616894)) ;
#55889=CARTESIAN_POINT('Ctrl Pts',(31.4448329300348,505.40997006538,-35.6752217409588)) ;
#55890=CARTESIAN_POINT('Ctrl Pts',(31.5206448004573,505.415828566778,-35.7681587730373)) ;
#55891=CARTESIAN_POINT('Ctrl Pts',(31.6180757464789,505.424775114195,-35.9115131174265)) ;
#55892=CARTESIAN_POINT('Ctrl Pts',(31.6464709333382,505.427600924226,-35.9570272181227)) ;
#55893=CARTESIAN_POINT('Ctrl Pts',(31.6995891429412,505.43338203227,-36.0500904320883)) ;
#55894=CARTESIAN_POINT('Ctrl Pts',(31.7242972324535,505.43633484725,-36.0975994165408)) ;
#55895=CARTESIAN_POINT('Ctrl Pts',(31.7950878352657,505.445690767992,-36.2477698231289)) ;
#55896=CARTESIAN_POINT('Ctrl Pts',(31.8346116503925,505.452307999899,-36.3532779626431)) ;
#55897=CARTESIAN_POINT('Ctrl Pts',(31.8915375668637,505.464802920524,-36.5539789154328)) ;
#55898=CARTESIAN_POINT('Ctrl Pts',(31.9112492784356,505.470629418937,-36.6482083690304)) ;
#55899=CARTESIAN_POINT('Ctrl Pts',(31.9320235603767,505.479690610628,-36.7999605742402)) ;
#55900=CARTESIAN_POINT('Ctrl Pts',(31.937402730746,505.483009407519,-36.8567511403242)) ;
#55901=CARTESIAN_POINT('Ctrl Pts',(31.9419669224967,505.487875768405,-36.943094869896)) ;
#55902=CARTESIAN_POINT('Ctrl Pts',(31.9428891147143,505.489502817408,-36.9725265498881)) ;
#55903=CARTESIAN_POINT('Ctrl Pts',(31.9435170542582,505.492952496085,-37.0364320994741)) ;
#55904=CARTESIAN_POINT('Ctrl Pts',(31.9429886571748,505.49476227536,-37.0708985509635)) ;
#55905=CARTESIAN_POINT('Ctrl Pts',(31.9370274694344,505.502333002227,-37.2180382696468)) ;
#55906=CARTESIAN_POINT('Ctrl Pts',(31.9231889087325,505.507720579316,-37.3301837395203)) ;
#55907=CARTESIAN_POINT('Ctrl Pts',(31.872100781106,505.519691521973,-37.5757734343199)) ;
#55908=CARTESIAN_POINT('Ctrl Pts',(31.830444490881,505.526259986763,-37.7077295174122)) ;
#55909=CARTESIAN_POINT('Ctrl Pts',(31.7539265691495,505.536093527371,-37.8855069550971)) ;
#55910=CARTESIAN_POINT('Ctrl Pts',(31.7299169398524,505.538978067801,-37.9355962640774)) ;
#55911=CARTESIAN_POINT('Ctrl Pts',(31.6805661196336,505.54459248417,-38.0286784891973)) ;
#55912=CARTESIAN_POINT('Ctrl Pts',(31.6556299448185,505.547305891994,-38.0718410072548)) ;
#55913=CARTESIAN_POINT('Ctrl Pts',(31.5945563448165,505.553696441116,-38.1692005939754)) ;
#55914=CARTESIAN_POINT('Ctrl Pts',(31.5573682182337,505.557410654666,-38.2226613420936)) ;
#55915=CARTESIAN_POINT('Ctrl Pts',(31.517715239327,505.561197820373,-38.2742565263254)) ;
#55916=CARTESIAN_POINT('Ctrl Pts',(31.5177152522353,505.503079332004,-38.2742565095294)) ;
#55917=CARTESIAN_POINT('Ctrl Pts',(31.5432594015477,505.500592988626,-38.241019281098)) ;
#55918=CARTESIAN_POINT('Ctrl Pts',(31.5677759902234,505.498132158959,-38.2070146138837)) ;
#55919=CARTESIAN_POINT('Ctrl Pts',(31.6077365179056,505.494018655011,-38.1478540702654)) ;
#55920=CARTESIAN_POINT('Ctrl Pts',(31.6237048133343,505.492343866605,-38.1230808209613)) ;
#55921=CARTESIAN_POINT('Ctrl Pts',(31.654357641665,505.489078477689,-38.0732011775607)) ;
#55922=CARTESIAN_POINT('Ctrl Pts',(31.6690523403465,505.487489075299,-38.048110885117)) ;
#55923=CARTESIAN_POINT('Ctrl Pts',(31.7041112169815,505.483637673754,-37.9852260120648)) ;
#55924=CARTESIAN_POINT('Ctrl Pts',(31.7238322599976,505.48141223199,-37.9470909865917)) ;
#55925=CARTESIAN_POINT('Ctrl Pts',(31.8051851392548,505.471837009847,-37.7769117488908)) ;
#55926=CARTESIAN_POINT('Ctrl Pts',(31.8538695483115,505.46497816158,-37.6391398552467)) ;
#55927=CARTESIAN_POINT('Ctrl Pts',(31.9094431812189,505.45325591178,-37.4053594828939)) ;
#55928=CARTESIAN_POINT('Ctrl Pts',(31.9249351970208,505.448557249049,-37.3119586025348)) ;
#55929=CARTESIAN_POINT('Ctrl Pts',(31.9388241458078,505.440997860556,-37.1667717136594)) ;
#55930=CARTESIAN_POINT('Ctrl Pts',(31.941794673664,505.438284193569,-37.1155524345259)) ;
#55931=CARTESIAN_POINT('Ctrl Pts',(31.9439502214248,505.432592308066,-37.0104156998921)) ;
#55932=CARTESIAN_POINT('Ctrl Pts',(31.9429356820414,505.429609822057,-36.9565344427641)) ;
#55933=CARTESIAN_POINT('Ctrl Pts',(31.9301488437827,505.417164331509,-36.7368609263858)) ;
#55934=CARTESIAN_POINT('Ctrl Pts',(31.9004030573165,505.407133710477,-36.572767822369)) ;
#55935=CARTESIAN_POINT('Ctrl Pts',(31.8334697505138,505.393559500329,-36.3567256915239)) ;
#55936=CARTESIAN_POINT('Ctrl Pts',(31.8131938104639,505.38997828119,-36.3001742412565)) ;
#55937=CARTESIAN_POINT('Ctrl Pts',(31.7739185188301,505.383928604321,-36.2041066614166)) ;
#55938=CARTESIAN_POINT('Ctrl Pts',(31.7560782378548,505.381423891878,-36.1641592143029)) ;
#55939=CARTESIAN_POINT('Ctrl Pts',(31.7243610022495,505.377381847522,-36.0988251011835)) ;
#55940=CARTESIAN_POINT('Ctrl Pts',(31.7112012525127,505.375807563079,-36.073111764612)) ;
#55941=CARTESIAN_POINT('Ctrl Pts',(31.6760828259188,505.371855363693,-36.0079197723625)) ;
#55942=CARTESIAN_POINT('Ctrl Pts',(31.6533577202339,505.369521543204,-35.9688736446147)) ;
#55943=CARTESIAN_POINT('Ctrl Pts',(31.5569927740764,505.360344610654,-35.8151887329742)) ;
#55944=CARTESIAN_POINT('Ctrl Pts',(31.4733198468932,505.353900202707,-35.7072476536089)) ;
#55945=CARTESIAN_POINT('Ctrl Pts',(31.3120446226615,505.342476280166,-35.5371587822526)) ;
#55946=CARTESIAN_POINT('Ctrl Pts',(31.2395057059155,505.337609991647,-35.4708751030663)) ;
#55947=CARTESIAN_POINT('Ctrl Pts',(31.1219360454515,505.329847836059,-35.3779655124312)) ;
#55948=CARTESIAN_POINT('Ctrl Pts',(31.0801646953316,505.327113139803,-35.3474444174973)) ;
#55949=CARTESIAN_POINT('Ctrl Pts',(30.9925627975267,505.321397130336,-35.2883741749554)) ;
#55950=CARTESIAN_POINT('Ctrl Pts',(30.9466698406774,505.318412465061,-35.259990538721)) ;
#55951=CARTESIAN_POINT('Ctrl Pts',(30.7478939960761,505.305505553309,-35.1476193254565)) ;
#55952=CARTESIAN_POINT('Ctrl Pts',(30.58577954101,505.294947537872,-35.0814812310761)) ;
#55953=CARTESIAN_POINT('Ctrl Pts',(30.3404172809854,505.279745486182,-35.0161382456613)) ;
#55954=CARTESIAN_POINT('Ctrl Pts',(30.2624002655157,505.275034187498,-35.0001439488519)) ;
#55955=CARTESIAN_POINT('Ctrl Pts',(30.1523268032647,505.268721449373,-34.9841687239715)) ;
#55956=CARTESIAN_POINT('Ctrl Pts',(30.1209034492736,505.266957199868,-34.9803470099263)) ;
#55957=CARTESIAN_POINT('Ctrl Pts',(30.0560717160086,505.263412270665,-34.9739785065418)) ;
#55958=CARTESIAN_POINT('Ctrl Pts',(30.0226647066311,505.261636127242,-34.9715196161678)) ;
#55959=CARTESIAN_POINT('Ctrl Pts',(29.8599061509482,505.253164541916,-34.9635348511347)) ;
#55960=CARTESIAN_POINT('Ctrl Pts',(29.7302774337086,505.246961535828,-34.9694250504372)) ;
#55961=CARTESIAN_POINT('Ctrl Pts',(29.4877074911626,505.235100694508,-35.0035776956375)) ;
#55962=CARTESIAN_POINT('Ctrl Pts',(29.3749275155548,505.229475604998,-35.0292868657789)) ;
#55963=CARTESIAN_POINT('Ctrl Pts',(29.2125147991268,505.220742448635,-35.0810192248685)) ;
#55964=CARTESIAN_POINT('Ctrl Pts',(29.1608129479363,505.217865460563,-35.0998042935609)) ;
#55965=CARTESIAN_POINT('Ctrl Pts',(29.0625858169282,505.212174789031,-35.14002444078)) ;
#55966=CARTESIAN_POINT('Ctrl Pts',(29.0159860179916,505.209372764817,-35.1611697744908)) ;
#55967=CARTESIAN_POINT('Ctrl Pts',(28.8896523223537,505.201472695054,-35.2242841378477)) ;
#55968=CARTESIAN_POINT('Ctrl Pts',(28.811821334232,505.196253829399,-35.2697873726756)) ;
#55969=CARTESIAN_POINT('Ctrl Pts',(28.6383150594367,505.183842710017,-35.3871591080225)) ;
#55970=CARTESIAN_POINT('Ctrl Pts',(28.545423907068,505.176578538692,-35.4625670479707)) ;
#55971=CARTESIAN_POINT('Ctrl Pts',(28.4269569699713,505.166783558656,-35.5772125941878)) ;
#55972=CARTESIAN_POINT('Ctrl Pts',(28.3953596266303,505.164113058441,-35.609888224118)) ;
#55973=CARTESIAN_POINT('Ctrl Pts',(28.3403197168179,505.1593935597,-35.6707206305667)) ;
#55974=CARTESIAN_POINT('Ctrl Pts',(28.3164966479929,505.157325692856,-35.6985078248541)) ;
#55975=CARTESIAN_POINT('Ctrl Pts',(28.2745393729093,505.153660272653,-35.7501785436828)) ;
#55976=CARTESIAN_POINT('Ctrl Pts',(28.2561631940795,505.152048213576,-35.7738486152144)) ;
#55977=CARTESIAN_POINT('Ctrl Pts',(28.2027390154522,505.147318538617,-35.8458614415899)) ;
#55978=CARTESIAN_POINT('Ctrl Pts',(28.1692712221652,505.144294241577,-35.8953414156333)) ;
#55979=CARTESIAN_POINT('Ctrl Pts',(28.0673887747061,505.134640099647,-36.0611000942924)) ;
#55980=CARTESIAN_POINT('Ctrl Pts',(28.0082538770677,505.128266383487,-36.1826624000175)) ;
#55981=CARTESIAN_POINT('Ctrl Pts',(27.9381615227228,505.118327366196,-36.3721019957412)) ;
#55982=CARTESIAN_POINT('Ctrl Pts',(27.9179684468764,505.114969852566,-36.4361575043987)) ;
#55983=CARTESIAN_POINT('Ctrl Pts',(27.88735574353,505.108760086949,-36.5529256348119)) ;
#55984=CARTESIAN_POINT('Ctrl Pts',(27.8757988018647,505.10594521769,-36.6052765730506)) ;
#55985=CARTESIAN_POINT('Ctrl Pts',(27.857097744626,505.100269343256,-36.7091305197846)) ;
#55986=CARTESIAN_POINT('Ctrl Pts',(27.849835510262,505.09741457224,-36.7605713997011)) ;
#55987=CARTESIAN_POINT('Ctrl Pts',(27.8257131609026,505.084158714168,-36.9954390527392)) ;
#55988=CARTESIAN_POINT('Ctrl Pts',(27.8316177713847,505.073010012815,-37.1803234450564)) ;
#55989=CARTESIAN_POINT('Ctrl Pts',(27.8751604348053,505.057240439044,-37.4400463182781)) ;
#55990=CARTESIAN_POINT('Ctrl Pts',(27.8927726421801,505.052548364635,-37.5173777387894)) ;
#55991=CARTESIAN_POINT('Ctrl Pts',(27.9235984391196,505.046255727532,-37.6238660426529)) ;
#55992=CARTESIAN_POINT('Ctrl Pts',(27.9330877258813,505.044493493175,-37.6540239419565)) ;
#55993=CARTESIAN_POINT('Ctrl Pts',(27.9540349362348,505.040954001598,-37.7155956044435)) ;
#55994=CARTESIAN_POINT('Ctrl Pts',(27.9655709722411,505.039181211303,-37.7469723276986)) ;
#55995=CARTESIAN_POINT('Ctrl Pts',(28.0257454140721,505.030676542357,-37.8990738843119)) ;
#55996=CARTESIAN_POINT('Ctrl Pts',(28.0850173936249,505.024443865928,-38.015283221071)) ;
#55997=CARTESIAN_POINT('Ctrl Pts',(28.2212010833597,505.012161033301,-38.2293385685761)) ;
#55998=CARTESIAN_POINT('Ctrl Pts',(28.2967701320055,505.006137981683,-38.3273658581876)) ;
#55999=CARTESIAN_POINT('Ctrl Pts',(28.4165817130021,504.997041877175,-38.4567911796279)) ;
#56000=CARTESIAN_POINT('Ctrl Pts',(28.4539660250601,504.994259088158,-38.4941734989611)) ;
#56001=CARTESIAN_POINT('Ctrl Pts',(28.5313488090397,504.988575411499,-38.5658019568158)) ;
#56002=CARTESIAN_POINT('Ctrl Pts',(28.571304899042,504.985677285731,-38.600034648668)) ;
#56003=CARTESIAN_POINT('Ctrl Pts',(28.7425712982585,504.973379570882,-38.7357261707658)) ;
#56004=CARTESIAN_POINT('Ctrl Pts',(28.8845975969161,504.963404056848,-38.8226133190237)) ;
#56005=CARTESIAN_POINT('Ctrl Pts',(29.0933743062256,504.949620468823,-38.9178862281061)) ;
#56006=CARTESIAN_POINT('Ctrl Pts',(29.1524584016029,504.945817270856,-38.9415999111235)) ;
#56007=CARTESIAN_POINT('Ctrl Pts',(29.2553632642701,504.939452978291,-38.9774493796882)) ;
#56008=CARTESIAN_POINT('Ctrl Pts',(29.2986617632715,504.936851163619,-38.9909445365498)) ;
#56009=CARTESIAN_POINT('Ctrl Pts',(29.370281174925,504.932710142485,-39.0106913320309)) ;
#56010=CARTESIAN_POINT('Ctrl Pts',(29.3983463375474,504.931129353618,-39.0177949315178)) ;
#56011=CARTESIAN_POINT('Ctrl Pts',(29.4693084782319,504.927236179828,-39.0341685816871)) ;
#56012=CARTESIAN_POINT('Ctrl Pts',(29.5123678087349,504.924963566524,-39.0426618116219)) ;
#56013=CARTESIAN_POINT('Ctrl Pts',(29.6893278364498,504.915869181874,-39.0717121081284)) ;
#56014=CARTESIAN_POINT('Ctrl Pts',(29.8248377999944,504.909454863808,-39.0803858137404)) ;
#56015=CARTESIAN_POINT('Ctrl Pts',(30.0605273344726,504.897970111336,-39.0721569499138)) ;
#56016=CARTESIAN_POINT('Ctrl Pts',(30.1604321294592,504.893001244726,-39.0613109501082)) ;
#56017=CARTESIAN_POINT('Ctrl Pts',(30.310144023599,504.885120863418,-39.0338575420454)) ;
#56018=CARTESIAN_POINT('Ctrl Pts',(30.3607745174687,504.882380238046,-39.0225773586328)) ;
#56019=CARTESIAN_POINT('Ctrl Pts',(30.4628939918487,504.876670346212,-38.9957327307716)) ;
#56020=CARTESIAN_POINT('Ctrl Pts',(30.5143066547907,504.873698577772,-38.9800379010375)) ;
#56021=CARTESIAN_POINT('Ctrl Pts',(30.725159134075,504.861082949099,-38.9065167783299)) ;
#56022=CARTESIAN_POINT('Ctrl Pts',(30.8777293303398,504.850842812948,-38.8310864827132)) ;
#56023=CARTESIAN_POINT('Ctrl Pts',(31.0898427805649,504.835608128116,-38.6912866238233)) ;
#56024=CARTESIAN_POINT('Ctrl Pts',(31.1574830734569,504.830587488018,-38.6404604145834)) ;
#56025=CARTESIAN_POINT('Ctrl Pts',(31.2461151503098,504.823968419732,-38.5648767573069)) ;
#56026=CARTESIAN_POINT('Ctrl Pts',(31.269940717696,504.82218515875,-38.5435794273517)) ;
#56027=CARTESIAN_POINT('Ctrl Pts',(31.317365891355,504.818645079631,-38.4991536137446)) ;
#56028=CARTESIAN_POINT('Ctrl Pts',(31.3409237007241,504.816891108491,-38.4759945289144)) ;
#56029=CARTESIAN_POINT('Ctrl Pts',(31.4185346947066,504.811085943858,-38.395926731457)) ;
#56030=CARTESIAN_POINT('Ctrl Pts',(31.4698864950361,504.807197796271,-38.3364897555531)) ;
#56031=CARTESIAN_POINT('Ctrl Pts',(31.5177152522312,504.803366924184,-38.2742565095347)) ;
#56032=CARTESIAN_POINT('Origin',(29.8885276254015,502.164639880024,-37.0221601717529)) ;
#56033=CARTESIAN_POINT('',(31.5172280011895,504.105620599056,-38.2738060481768)) ;
#56034=CARTESIAN_POINT('',(31.5177152521424,504.164515898581,-38.2742565096501)) ;
#56035=CARTESIAN_POINT('',(31.5177152522233,502.164639880024,-38.2742565095444)) ;
#56036=CARTESIAN_POINT('',(29.8878696237816,503.856489559997,-34.9674102771103)) ;
#56037=CARTESIAN_POINT('Ctrl Pts',(29.8878312245244,503.857426760662,-34.9679514454232)) ;
#56038=CARTESIAN_POINT('Ctrl Pts',(29.9587306547387,503.861501994475,-34.968065421851)) ;
#56039=CARTESIAN_POINT('Ctrl Pts',(30.0296724459679,503.865522183533,-34.9718222713218)) ;
#56040=CARTESIAN_POINT('Ctrl Pts',(30.100260036513,503.869457885301,-34.9791956158892)) ;
#56041=CARTESIAN_POINT('Ctrl Pts',(30.1708288602434,503.873392540701,-34.9865670001376)) ;
#56042=CARTESIAN_POINT('Ctrl Pts',(30.2410436494645,503.877242723409,-34.9975529416747)) ;
#56043=CARTESIAN_POINT('Ctrl Pts',(30.3105123120153,503.881003593668,-35.0120926107395)) ;
#56044=CARTESIAN_POINT('Ctrl Pts',(30.3799863322682,503.88476475398,-35.0266334011618)) ;
#56045=CARTESIAN_POINT('Ctrl Pts',(30.4487140397119,503.888436660364,-35.0447285611316)) ;
#56046=CARTESIAN_POINT('Ctrl Pts',(30.5163081024759,503.892038742141,-35.0662821556403)) ;
#56047=CARTESIAN_POINT('Ctrl Pts',(30.5839794203305,503.895644940836,-35.0878603843376)) ;
#56048=CARTESIAN_POINT('Ctrl Pts',(30.6505143686305,503.89918134044,-35.112905163166)) ;
#56049=CARTESIAN_POINT('Ctrl Pts',(30.7155306513185,503.902689862847,-35.1412828089591)) ;
#56050=CARTESIAN_POINT('Ctrl Pts',(30.7805867418378,503.906200533434,-35.1696778296696)) ;
#56051=CARTESIAN_POINT('Ctrl Pts',(30.8441220708106,503.909683637407,-35.2014101137795)) ;
#56052=CARTESIAN_POINT('Ctrl Pts',(30.9057627031913,503.913199682518,-35.236304393048)) ;
#56053=CARTESIAN_POINT('Ctrl Pts',(30.9638589191116,503.916513550467,-35.2691922059154)) ;
#56054=CARTESIAN_POINT('Ctrl Pts',(31.0202722455625,503.919857171378,-35.3048892324424)) ;
#56055=CARTESIAN_POINT('Ctrl Pts',(31.0746996633575,503.923291086605,-35.343209505544)) ;
#56056=CARTESIAN_POINT('Ctrl Pts',(31.0781287493569,503.923507433276,-35.3456237944687)) ;
#56057=CARTESIAN_POINT('Ctrl Pts',(31.0815499697125,503.923724138357,-35.3480484972001)) ;
#56058=CARTESIAN_POINT('Ctrl Pts',(31.0849632555621,503.923941216991,-35.3504835678714)) ;
#56059=CARTESIAN_POINT('Ctrl Pts',(31.121809935943,503.926284597351,-35.3767703409934)) ;
#56060=CARTESIAN_POINT('Ctrl Pts',(31.157729995907,503.928671744451,-35.4042641881606)) ;
#56061=CARTESIAN_POINT('Ctrl Pts',(31.1926332392124,503.931122357307,-35.4328954209148)) ;
#56062=CARTESIAN_POINT('Ctrl Pts',(31.1926595354685,503.931124203609,-35.4329169918108)) ;
#56063=CARTESIAN_POINT('Ctrl Pts',(31.1926858311482,503.931126049948,-35.4329385633523)) ;
#56064=CARTESIAN_POINT('Ctrl Pts',(31.1927121262513,503.931127896322,-35.4329601355393)) ;
#56065=CARTESIAN_POINT('Ctrl Pts',(31.2424669614003,503.934621552848,-35.4737784051372)) ;
#56066=CARTESIAN_POINT('Ctrl Pts',(31.2903362767567,503.938253505451,-35.517065402354)) ;
#56067=CARTESIAN_POINT('Ctrl Pts',(31.3360902907372,503.941958684045,-35.5626000995648)) ;
#56068=CARTESIAN_POINT('Ctrl Pts',(31.3407283961832,503.942334279703,-35.567215972769)) ;
#56069=CARTESIAN_POINT('Ctrl Pts',(31.3453447563855,503.94271062783,-35.5718548999249)) ;
#56070=CARTESIAN_POINT('Ctrl Pts',(31.3499391269652,503.943087660642,-35.5765166214108)) ;
#56071=CARTESIAN_POINT('Ctrl Pts',(31.3997794398737,503.947177760261,-35.6270875654645)) ;
#56072=CARTESIAN_POINT('Ctrl Pts',(31.4470335721025,503.951347819346,-35.6803467425906)) ;
#56073=CARTESIAN_POINT('Ctrl Pts',(31.491437646493,503.955523483257,-35.7359747223897)) ;
#56074=CARTESIAN_POINT('Ctrl Pts',(31.5357868487461,503.95969398711,-35.7915339601601)) ;
#56075=CARTESIAN_POINT('Ctrl Pts',(31.5772933649038,503.963869728294,-35.8494559619384)) ;
#56076=CARTESIAN_POINT('Ctrl Pts',(31.6157305657986,503.967995970738,-35.909405072221)) ;
#56077=CARTESIAN_POINT('Ctrl Pts',(31.6541420787343,503.972119455573,-35.969314117924)) ;
#56078=CARTESIAN_POINT('Ctrl Pts',(31.6894885400054,503.976193338822,-36.0312474986286)) ;
#56079=CARTESIAN_POINT('Ctrl Pts',(31.7215763217742,503.980186173349,-36.0948546235593)) ;
#56080=CARTESIAN_POINT('Ctrl Pts',(31.7536534439539,503.984177681453,-36.1584406181473)) ;
#56081=CARTESIAN_POINT('Ctrl Pts',(31.7824740663728,503.988088154215,-36.2236992266939)) ;
#56082=CARTESIAN_POINT('Ctrl Pts',(31.8078759919812,503.991910879953,-36.2902651839037)) ;
#56083=CARTESIAN_POINT('Ctrl Pts',(31.8332780166312,503.995733620596,-36.3568314006528)) ;
#56084=CARTESIAN_POINT('Ctrl Pts',(31.8552612087533,503.999468678092,-36.4247049768362)) ;
#56085=CARTESIAN_POINT('Ctrl Pts',(31.8736953332307,504.003133864588,-36.4935057365259)) ;
#56086=CARTESIAN_POINT('Ctrl Pts',(31.8921479241621,504.006802722698,-36.5623754176373)) ;
#56087=CARTESIAN_POINT('Ctrl Pts',(31.9070440935627,504.010401747856,-36.6321741504546)) ;
#56088=CARTESIAN_POINT('Ctrl Pts',(31.9182878507565,504.013971589968,-36.7025055842154)) ;
#56089=CARTESIAN_POINT('Ctrl Pts',(31.9295376629882,504.017543354527,-36.7728748931713)) ;
#56090=CARTESIAN_POINT('Ctrl Pts',(31.9371307375621,504.021086241873,-36.8437774587815)) ;
#56091=CARTESIAN_POINT('Ctrl Pts',(31.9410102774574,504.024659943532,-36.9148012608961)) ;
#56092=CARTESIAN_POINT('Ctrl Pts',(31.9446846091069,504.028044614257,-36.9820682593097)) ;
#56093=CARTESIAN_POINT('Ctrl Pts',(31.9450275903617,504.031457416092,-37.0494443437025)) ;
#56094=CARTESIAN_POINT('Ctrl Pts',(31.9420298057886,504.034959576058,-37.1165662660705)) ;
#56095=CARTESIAN_POINT('Ctrl Pts',(31.9418569339711,504.035161533451,-37.1204369540504)) ;
#56096=CARTESIAN_POINT('Ctrl Pts',(31.9416729594104,504.035363787999,-37.124306809581)) ;
#56097=CARTESIAN_POINT('Ctrl Pts',(31.941477882663,504.035566351442,-37.1281757677485)) ;
#56098=CARTESIAN_POINT('Ctrl Pts',(31.939306877194,504.037820676204,-37.171233330753)) ;
#56099=CARTESIAN_POINT('Ctrl Pts',(31.9357608346423,504.040113478892,-37.2141776975869)) ;
#56100=CARTESIAN_POINT('Ctrl Pts',(31.9308473628059,504.04246162487,-37.2569112546444)) ;
#56101=CARTESIAN_POINT('Ctrl Pts',(31.9308436908624,504.04246337969,-37.2569431903537)) ;
#56102=CARTESIAN_POINT('Ctrl Pts',(31.9308400181555,504.042465134541,-37.2569751259456)) ;
#56103=CARTESIAN_POINT('Ctrl Pts',(31.9308363446852,504.042466889423,-37.2570070614202)) ;
#56104=CARTESIAN_POINT('Ctrl Pts',(31.9234398621271,504.046000320481,-37.3213087063446)) ;
#56105=CARTESIAN_POINT('Ctrl Pts',(31.912915186025,504.049667772526,-37.3853536185928)) ;
#56106=CARTESIAN_POINT('Ctrl Pts',(31.8993255122597,504.053404304604,-37.4488253707413)) ;
#56107=CARTESIAN_POINT('Ctrl Pts',(31.8979992225737,504.053768972957,-37.4550199219631)) ;
#56108=CARTESIAN_POINT('Ctrl Pts',(31.8966437686663,504.054134299289,-37.4612089854468)) ;
#56109=CARTESIAN_POINT('Ctrl Pts',(31.8952592287782,504.05450022323,-37.4673922490841)) ;
#56110=CARTESIAN_POINT('Ctrl Pts',(31.8797919975381,504.058588101277,-37.5364678815868)) ;
#56111=CARTESIAN_POINT('Ctrl Pts',(31.8606909691678,504.062749822263,-37.6048235139712)) ;
#56112=CARTESIAN_POINT('Ctrl Pts',(31.8380810444409,504.066913795307,-37.6720715610843)) ;
#56113=CARTESIAN_POINT('Ctrl Pts',(31.8368818375184,504.067134648113,-37.6756383276524)) ;
#56114=CARTESIAN_POINT('Ctrl Pts',(31.8356727670002,504.067355507253,-37.679201968751)) ;
#56115=CARTESIAN_POINT('Ctrl Pts',(31.8344538540919,504.067576362047,-37.6827624233691)) ;
#56116=CARTESIAN_POINT('Ctrl Pts',(31.8113790685836,504.071757281756,-37.7501640613874)) ;
#56117=CARTESIAN_POINT('Ctrl Pts',(31.7847747385406,504.075936436921,-37.8164279458178)) ;
#56118=CARTESIAN_POINT('Ctrl Pts',(31.7548029742689,504.080061397014,-37.8811820458108)) ;
#56119=CARTESIAN_POINT('Ctrl Pts',(31.7248510222535,504.084183630383,-37.9458933413559)) ;
#56120=CARTESIAN_POINT('Ctrl Pts',(31.69153621929,504.08825158237,-38.0090969421066)) ;
#56121=CARTESIAN_POINT('Ctrl Pts',(31.6550509567708,504.092236212904,-38.0704403685554)) ;
#56122=CARTESIAN_POINT('Ctrl Pts',(31.6185755072556,504.09621977174,-38.1317672961973)) ;
#56123=CARTESIAN_POINT('Ctrl Pts',(31.5789313196791,504.100120021672,-38.1912350467056)) ;
#56124=CARTESIAN_POINT('Ctrl Pts',(31.5363401614159,504.103932619486,-38.2485095559607)) ;
#56125=CARTESIAN_POINT('Ctrl Pts',(31.5300337405706,504.104497146193,-38.2569901226744)) ;
#56126=CARTESIAN_POINT('Ctrl Pts',(31.5236627620926,504.105059795431,-38.2654226367447)) ;
#56127=CARTESIAN_POINT('Ctrl Pts',(31.5172280011895,504.105620599056,-38.2738060481768)) ;
#56128=CARTESIAN_POINT('',(27.9033532997302,503.710565160562,-36.4919899545636)) ;
#56129=CARTESIAN_POINT('Ctrl Pts',(27.9033532997302,503.710565160562,-36.4919899545636)) ;
#56130=CARTESIAN_POINT('Ctrl Pts',(27.9220919685295,503.714502851079,-36.4218247076459)) ;
#56131=CARTESIAN_POINT('Ctrl Pts',(27.9445724045105,503.718440541595,-36.3525880402978)) ;
#56132=CARTESIAN_POINT('Ctrl Pts',(27.9706795420364,503.722378232112,-36.2846940426108)) ;
#56133=CARTESIAN_POINT('Ctrl Pts',(27.9967660504768,503.726312811183,-36.2168536927464)) ;
#56134=CARTESIAN_POINT('Ctrl Pts',(28.0264733976995,503.730247390253,-36.1503543313746)) ;
#56135=CARTESIAN_POINT('Ctrl Pts',(28.0596371618002,503.734181969324,-36.0855934444734)) ;
#56136=CARTESIAN_POINT('Ctrl Pts',(28.0927915167263,503.738115432081,-36.020850931436)) ;
#56137=CARTESIAN_POINT('Ctrl Pts',(28.1294001364632,503.742048894839,-35.9578463250151)) ;
#56138=CARTESIAN_POINT('Ctrl Pts',(28.1692515493607,503.745982357596,-35.8969547074697)) ;
#56139=CARTESIAN_POINT('Ctrl Pts',(28.2090987948209,503.749915409014,-35.8360694576283)) ;
#56140=CARTESIAN_POINT('Ctrl Pts',(28.2521879077288,503.753848460432,-35.7772971427937)) ;
#56141=CARTESIAN_POINT('Ctrl Pts',(28.2982635873496,503.75778151185,-35.720984606436)) ;
#56142=CARTESIAN_POINT('Ctrl Pts',(28.3443474330767,503.761715260333,-35.6646620896685)) ;
#56143=CARTESIAN_POINT('Ctrl Pts',(28.3934186057526,503.765649008815,-35.6108005738718)) ;
#56144=CARTESIAN_POINT('Ctrl Pts',(28.4451818536921,503.769582757297,-35.559713404931)) ;
#56145=CARTESIAN_POINT('Ctrl Pts',(28.49696886516,503.773518311689,-35.508602782837)) ;
#56146=CARTESIAN_POINT('Ctrl Pts',(28.5514500804081,503.777453866081,-35.4602693617864)) ;
#56147=CARTESIAN_POINT('Ctrl Pts',(28.6082948160149,503.781389420473,-35.4149882717156)) ;
#56148=CARTESIAN_POINT('Ctrl Pts',(28.6652241539097,503.785330832169,-35.3696397895851)) ;
#56149=CARTESIAN_POINT('Ctrl Pts',(28.724523672739,503.789272243865,-35.3273529930464)) ;
#56150=CARTESIAN_POINT('Ctrl Pts',(28.7858315231192,503.793213655561,-35.2883612017132)) ;
#56151=CARTESIAN_POINT('Ctrl Pts',(28.8471906866653,503.797158366122,-35.2493367752077)) ;
#56152=CARTESIAN_POINT('Ctrl Pts',(28.9105611288309,503.801103076683,-35.2136130723263)) ;
#56153=CARTESIAN_POINT('Ctrl Pts',(28.9755563680077,503.805047787244,-35.181377445391)) ;
#56154=CARTESIAN_POINT('Ctrl Pts',(29.0406755945526,503.809000022884,-35.1490803245588)) ;
#56155=CARTESIAN_POINT('Ctrl Pts',(29.1074253848159,503.812952258523,-35.1202847483778)) ;
#56156=CARTESIAN_POINT('Ctrl Pts',(29.1753996605939,503.816904494162,-35.0951297961986)) ;
#56157=CARTESIAN_POINT('Ctrl Pts',(29.2033933039097,503.818532131581,-35.0847703072468)) ;
#56158=CARTESIAN_POINT('Ctrl Pts',(29.2315944556788,503.820159769001,-35.0750276829276)) ;
#56159=CARTESIAN_POINT('Ctrl Pts',(29.2599741689153,503.82178740642,-35.0659091360116)) ;
#56160=CARTESIAN_POINT('Ctrl Pts',(29.3393312769002,503.826338706757,-35.0404112916096)) ;
#56161=CARTESIAN_POINT('Ctrl Pts',(29.4203288439844,503.830890007094,-35.019718141297)) ;
#56162=CARTESIAN_POINT('Ctrl Pts',(29.5024259274531,503.835441307431,-35.0040117526962)) ;
#56163=CARTESIAN_POINT('Ctrl Pts',(29.5836359998494,503.839943433625,-34.9884750624574)) ;
#56164=CARTESIAN_POINT('Ctrl Pts',(29.6659218421143,503.844445559818,-34.9778180432059)) ;
#56165=CARTESIAN_POINT('Ctrl Pts',(29.7487386216568,503.848947686012,-34.9721707578944)) ;
#56166=CARTESIAN_POINT('Ctrl Pts',(29.7949829729049,503.851461644007,-34.9690173504933)) ;
#56167=CARTESIAN_POINT('Ctrl Pts',(29.8413925003401,503.853975602002,-34.9674251606845)) ;
#56168=CARTESIAN_POINT('Ctrl Pts',(29.8878696237816,503.856489559997,-34.9674102771103)) ;
#56169=CARTESIAN_POINT('',(27.9020254134846,503.711738695905,-37.5552366910798)) ;
#56170=CARTESIAN_POINT('Origin',(29.8885276254018,503.710565160562,-37.0221601717529)) ;
#56171=CARTESIAN_POINT('',(29.8898911409064,503.915940460665,-34.9674106241619)) ;
#56172=CARTESIAN_POINT('Ctrl Pts',(27.9039683500008,503.712921345492,-37.5546280533383)) ;
#56173=CARTESIAN_POINT('Ctrl Pts',(27.8995037155845,503.713852301909,-37.5379879292133)) ;
#56174=CARTESIAN_POINT('Ctrl Pts',(27.8952483859091,503.714771424712,-37.5212917219665)) ;
#56175=CARTESIAN_POINT('Ctrl Pts',(27.886036764227,503.716841188879,-37.4831506871666)) ;
#56176=CARTESIAN_POINT('Ctrl Pts',(27.8812139526205,503.717985213449,-37.4616755791405)) ;
#56177=CARTESIAN_POINT('Ctrl Pts',(27.8568247709929,503.724143278074,-37.3442834841899)) ;
#56178=CARTESIAN_POINT('Ctrl Pts',(27.8437854282688,503.728897792319,-37.2471320603135)) ;
#56179=CARTESIAN_POINT('Ctrl Pts',(27.8296332156294,503.739968633839,-37.0190582167473)) ;
#56180=CARTESIAN_POINT('Ctrl Pts',(27.8339921163726,503.746265877539,-36.888231605803)) ;
#56181=CARTESIAN_POINT('Ctrl Pts',(27.8579825952917,503.755817822207,-36.7026628037148)) ;
#56182=CARTESIAN_POINT('Ctrl Pts',(27.8675376787861,503.758764102179,-36.6469395229417)) ;
#56183=CARTESIAN_POINT('Ctrl Pts',(27.8898799130842,503.764464200626,-36.5426621624512)) ;
#56184=CARTESIAN_POINT('Ctrl Pts',(27.9021730887732,503.767200103077,-36.4940446020989)) ;
#56185=CARTESIAN_POINT('Ctrl Pts',(27.9394879791671,503.774613120687,-36.3663252054139)) ;
#56186=CARTESIAN_POINT('Ctrl Pts',(27.9675402507877,503.779385189147,-36.2882119439521)) ;
#56187=CARTESIAN_POINT('Ctrl Pts',(28.0495855302198,503.791628527376,-36.0969801900279)) ;
#56188=CARTESIAN_POINT('Ctrl Pts',(28.1093470840185,503.799222721748,-35.9866988954612)) ;
#56189=CARTESIAN_POINT('Ctrl Pts',(28.2043468026331,503.809383269486,-35.8441703913619)) ;
#56190=CARTESIAN_POINT('Ctrl Pts',(28.231214526888,503.812090938927,-35.8066608073265)) ;
#56191=CARTESIAN_POINT('Ctrl Pts',(28.2818373445074,503.816865971107,-35.7407901992321)) ;
#56192=CARTESIAN_POINT('Ctrl Pts',(28.3051390535472,503.818952610576,-35.7121053384563)) ;
#56193=CARTESIAN_POINT('Ctrl Pts',(28.3486802868947,503.822632837904,-35.6613654561645)) ;
#56194=CARTESIAN_POINT('Ctrl Pts',(28.3686500757782,503.824241688844,-35.6390967753399)) ;
#56195=CARTESIAN_POINT('Ctrl Pts',(28.4296630890996,503.828947793278,-35.5739780438843)) ;
#56196=CARTESIAN_POINT('Ctrl Pts',(28.4720856913458,503.831953423431,-35.5324586622611)) ;
#56197=CARTESIAN_POINT('Ctrl Pts',(28.5937487897015,503.840064678512,-35.4232894697111)) ;
#56198=CARTESIAN_POINT('Ctrl Pts',(28.676425041411,503.845036795839,-35.3597376320947)) ;
#56199=CARTESIAN_POINT('Ctrl Pts',(28.8506239461131,503.855149598635,-35.2457657528314)) ;
#56200=CARTESIAN_POINT('Ctrl Pts',(28.9418766686474,503.860277451658,-35.1955046718228)) ;
#56201=CARTESIAN_POINT('Ctrl Pts',(29.0844113825613,503.868361659425,-35.1305569912995)) ;
#56202=CARTESIAN_POINT('Ctrl Pts',(29.1331037638954,503.871133589946,-35.1105902289528)) ;
#56203=CARTESIAN_POINT('Ctrl Pts',(29.2320299767583,503.876814001513,-35.0743949495267)) ;
#56204=CARTESIAN_POINT('Ctrl Pts',(29.2822295473098,503.87972065266,-35.0581895918306)) ;
#56205=CARTESIAN_POINT('Ctrl Pts',(29.4512549976591,503.889603698697,-35.0107231550851)) ;
#56206=CARTESIAN_POINT('Ctrl Pts',(29.5722404547271,503.896851265574,-34.9881883691788)) ;
#56207=CARTESIAN_POINT('Ctrl Pts',(29.7594459305128,503.908121077591,-34.9704312157898)) ;
#56208=CARTESIAN_POINT('Ctrl Pts',(29.8246508535686,503.912051762148,-34.9673673312246)) ;
#56209=CARTESIAN_POINT('Ctrl Pts',(29.8898911409064,503.915940460665,-34.9674106241619)) ;
#56210=CARTESIAN_POINT('Ctrl Pts',(29.8898907546911,503.915940437644,-34.9674106239056)) ;
#56211=CARTESIAN_POINT('Ctrl Pts',(29.9412118975136,503.918999474773,-34.9674446705626)) ;
#56212=CARTESIAN_POINT('Ctrl Pts',(29.9925166924859,503.922029783632,-34.9694014736775)) ;
#56213=CARTESIAN_POINT('Ctrl Pts',(30.0772710138307,503.926938004848,-34.9758202236688)) ;
#56214=CARTESIAN_POINT('Ctrl Pts',(30.110779615718,503.928852925703,-34.9791879325618)) ;
#56215=CARTESIAN_POINT('Ctrl Pts',(30.1731762546706,503.932352264999,-34.9870125093617)) ;
#56216=CARTESIAN_POINT('Ctrl Pts',(30.2020783033838,503.933944411954,-34.9912645428387)) ;
#56217=CARTESIAN_POINT('Ctrl Pts',(30.275719399037,503.937928801769,-35.0037083854746)) ;
#56218=CARTESIAN_POINT('Ctrl Pts',(30.3202933140566,503.940276653806,-35.0127711910703)) ;
#56219=CARTESIAN_POINT('Ctrl Pts',(30.499928782168,503.949609406583,-35.0555494144053)) ;
#56220=CARTESIAN_POINT('Ctrl Pts',(30.6317068364755,503.956177054412,-35.1014677215833)) ;
#56221=CARTESIAN_POINT('Ctrl Pts',(30.8449847968994,503.967650789419,-35.2010512629974)) ;
#56222=CARTESIAN_POINT('Ctrl Pts',(30.9291608931864,503.972423959962,-35.2478073802305)) ;
#56223=CARTESIAN_POINT('Ctrl Pts',(31.0530156507559,503.980081622879,-35.3284567998562)) ;
#56224=CARTESIAN_POINT('Ctrl Pts',(31.095203256516,503.982812703552,-35.3582500933929)) ;
#56225=CARTESIAN_POINT('Ctrl Pts',(31.1792661583935,503.988538944048,-35.4224956388487)) ;
#56226=CARTESIAN_POINT('Ctrl Pts',(31.2209892942773,503.991538273957,-35.4570794438543)) ;
#56227=CARTESIAN_POINT('Ctrl Pts',(31.384374251533,504.003959453222,-35.6037802147022)) ;
#56228=CARTESIAN_POINT('Ctrl Pts',(31.4936433169988,504.013941525847,-35.7287360089024)) ;
#56229=CARTESIAN_POINT('Ctrl Pts',(31.6207528046515,504.027493959158,-35.9153429551586)) ;
#56230=CARTESIAN_POINT('Ctrl Pts',(31.6525509761974,504.031098492875,-35.9667594242137)) ;
#56231=CARTESIAN_POINT('Ctrl Pts',(31.7034883341003,504.037184023251,-36.0578741591218)) ;
#56232=CARTESIAN_POINT('Ctrl Pts',(31.7237034616467,504.03970172154,-36.0969250055133)) ;
#56233=CARTESIAN_POINT('Ctrl Pts',(31.7551791831204,504.043766137583,-36.1628264484052)) ;
#56234=CARTESIAN_POINT('Ctrl Pts',(31.7671480753834,504.04535007867,-36.1893169209582)) ;
#56235=CARTESIAN_POINT('Ctrl Pts',(31.7964942216375,504.049341231933,-36.2581232157323)) ;
#56236=CARTESIAN_POINT('Ctrl Pts',(31.8130274850055,504.051702887088,-36.3007796192349)) ;
#56237=CARTESIAN_POINT('Ctrl Pts',(31.8732001605406,504.060918625975,-36.4728673129829)) ;
#56238=CARTESIAN_POINT('Ctrl Pts',(31.9053147636052,504.067376953104,-36.6059599726057)) ;
#56239=CARTESIAN_POINT('Ctrl Pts',(31.9373099817429,504.078788352167,-36.8378057805151)) ;
#56240=CARTESIAN_POINT('Ctrl Pts',(31.9437466642977,504.083623846665,-36.9351671541599)) ;
#56241=CARTESIAN_POINT('Ctrl Pts',(31.9429870674464,504.09136281609,-37.0845125529047)) ;
#56242=CARTESIAN_POINT('Ctrl Pts',(31.9407566908302,504.094108476059,-37.1363820140462)) ;
#56243=CARTESIAN_POINT('Ctrl Pts',(31.9321639818676,504.09986743614,-37.2424281855392)) ;
#56244=CARTESIAN_POINT('Ctrl Pts',(31.9256036212411,504.102885005581,-37.2965470116399)) ;
#56245=CARTESIAN_POINT('Ctrl Pts',(31.8907667679561,504.115225099739,-37.5118637552816)) ;
#56246=CARTESIAN_POINT('Ctrl Pts',(31.8454350063363,504.125089287533,-37.6696699718548)) ;
#56247=CARTESIAN_POINT('Ctrl Pts',(31.7582035803814,504.138562293709,-37.8765757688344)) ;
#56248=CARTESIAN_POINT('Ctrl Pts',(31.7320303805895,504.142198731399,-37.9316723938254)) ;
#56249=CARTESIAN_POINT('Ctrl Pts',(31.6827119127414,504.148330635356,-38.0245851249103)) ;
#56250=CARTESIAN_POINT('Ctrl Pts',(31.6607219471618,504.150863312766,-38.0629679880221)) ;
#56251=CARTESIAN_POINT('Ctrl Pts',(31.622203027077,504.154947338704,-38.1254360075018)) ;
#56252=CARTESIAN_POINT('Ctrl Pts',(31.6063716377376,504.156536360766,-38.1499279277824)) ;
#56253=CARTESIAN_POINT('Ctrl Pts',(31.5669298128708,504.160289956304,-38.2081872630936)) ;
#56254=CARTESIAN_POINT('Ctrl Pts',(31.5428169386247,504.162424078541,-38.2415949996772)) ;
#56255=CARTESIAN_POINT('Ctrl Pts',(31.5177152521424,504.164515898581,-38.2742565096501)) ;
#56256=CARTESIAN_POINT('Origin',(29.888527625402,504.710565160562,-37.0221601717529)) ;
#56257=CARTESIAN_POINT('',(30.464143066922,505.578718967617,-35.4585122521231)) ;
#56258=CARTESIAN_POINT('',(30.4640904799735,505.710565160562,-35.4587397547064)) ;
#56259=CARTESIAN_POINT('',(30.4640904799733,504.710565160562,-35.4587397547064)) ;
#56260=CARTESIAN_POINT('',(31.5536816258517,505.710557682283,-36.9466234719841)) ;
#56261=CARTESIAN_POINT('Origin',(29.8885276254021,505.710565160562,-37.0221601717529)) ;
#56262=CARTESIAN_POINT('Ctrl Pts',(31.5536816419713,505.710557682144,-36.9466234712529)) ;
#56263=CARTESIAN_POINT('Ctrl Pts',(31.5512527851025,505.706944742544,-36.8937691566076)) ;
#56264=CARTESIAN_POINT('Ctrl Pts',(31.5462448774997,505.70323427545,-36.8409426256499)) ;
#56265=CARTESIAN_POINT('Ctrl Pts',(31.5386909643017,505.699480728201,-36.7884134558091)) ;
#56266=CARTESIAN_POINT('Ctrl Pts',(31.5300837950213,505.695203816919,-36.7285600467054)) ;
#56267=CARTESIAN_POINT('Ctrl Pts',(31.5181708641553,505.690871535778,-36.6690914842317)) ;
#56268=CARTESIAN_POINT('Ctrl Pts',(31.5030394057526,505.686550012591,-36.6103848174665)) ;
#56269=CARTESIAN_POINT('Ctrl Pts',(31.4879233747511,505.682232895447,-36.5517380055599)) ;
#56270=CARTESIAN_POINT('Ctrl Pts',(31.4695956550047,505.677926812381,-36.4938513990106)) ;
#56271=CARTESIAN_POINT('Ctrl Pts',(31.4481779335575,505.673676937873,-36.4370847936346)) ;
#56272=CARTESIAN_POINT('Ctrl Pts',(31.426773921506,505.669429783692,-36.3803545243301)) ;
#56273=CARTESIAN_POINT('Ctrl Pts',(31.4022839523053,505.665238884364,-36.3247427727838)) ;
#56274=CARTESIAN_POINT('Ctrl Pts',(31.3748614996201,505.661125540527,-36.27059400033)) ;
#56275=CARTESIAN_POINT('Ctrl Pts',(31.3474461947096,505.657013268851,-36.2164593419756)) ;
#56276=CARTESIAN_POINT('Ctrl Pts',(31.3170999076325,505.652978502872,-36.1637869518671)) ;
#56277=CARTESIAN_POINT('Ctrl Pts',(31.2840075847354,505.649017956302,-36.1129063626823)) ;
#56278=CARTESIAN_POINT('Ctrl Pts',(31.2508873781163,505.645054072561,-36.0619829013119)) ;
#56279=CARTESIAN_POINT('Ctrl Pts',(31.2150163856363,505.641164409488,-36.0128544152588)) ;
#56280=CARTESIAN_POINT('Ctrl Pts',(31.1766127984997,505.637322040209,-35.965835046155)) ;
#56281=CARTESIAN_POINT('Ctrl Pts',(31.1381947871522,505.633478227753,-35.9187980167923)) ;
#56282=CARTESIAN_POINT('Ctrl Pts',(31.0972420804711,505.629681471652,-35.8738719648829)) ;
#56283=CARTESIAN_POINT('Ctrl Pts',(31.0540082979801,505.62588411196,-35.8313519796076)) ;
#56284=CARTESIAN_POINT('Ctrl Pts',(31.0106923755428,505.622079537657,-35.7887512105309)) ;
#56285=CARTESIAN_POINT('Ctrl Pts',(30.9650864474462,505.618273883806,-35.7485661354866)) ;
#56286=CARTESIAN_POINT('Ctrl Pts',(30.9174843642785,505.614403978776,-35.7110684842806)) ;
#56287=CARTESIAN_POINT('Ctrl Pts',(30.8747062787521,505.610926250128,-35.6773708470431)) ;
#56288=CARTESIAN_POINT('Ctrl Pts',(30.8303158357592,505.607396043612,-35.6458432612686)) ;
#56289=CARTESIAN_POINT('Ctrl Pts',(30.7845572496917,505.603763009415,-35.6166606978547)) ;
#56290=CARTESIAN_POINT('Ctrl Pts',(30.7804377721901,505.603435940685,-35.614033498814)) ;
#56291=CARTESIAN_POINT('Ctrl Pts',(30.7763071950674,505.603108038564,-35.6114252724309)) ;
#56292=CARTESIAN_POINT('Ctrl Pts',(30.7721656894153,505.602779266313,-35.6088361268173)) ;
#56293=CARTESIAN_POINT('Ctrl Pts',(30.7721384702333,505.602777105526,-35.6088191101978)) ;
#56294=CARTESIAN_POINT('Ctrl Pts',(30.7721112505793,505.602774944701,-35.6088020944026)) ;
#56295=CARTESIAN_POINT('Ctrl Pts',(30.7720840304533,505.602772783839,-35.6087850794315)) ;
#56296=CARTESIAN_POINT('Ctrl Pts',(30.7243106697558,505.598980308744,-35.5789225302735)) ;
#56297=CARTESIAN_POINT('Ctrl Pts',(30.6749166898039,505.595062673764,-35.5515039524481)) ;
#56298=CARTESIAN_POINT('Ctrl Pts',(30.6241821421764,505.591085141819,-35.526667745808)) ;
#56299=CARTESIAN_POINT('Ctrl Pts',(30.6187902896983,505.590662426598,-35.5240282591351)) ;
#56300=CARTESIAN_POINT('Ctrl Pts',(30.6133833445669,505.59023903487,-35.521417936482)) ;
#56301=CARTESIAN_POINT('Ctrl Pts',(30.6079616773488,505.58981504497,-35.5188369411351)) ;
#56302=CARTESIAN_POINT('Ctrl Pts',(30.5610542874591,505.586146752775,-35.4965065858826)) ;
#56303=CARTESIAN_POINT('Ctrl Pts',(30.5130406271979,505.58243378182,-35.476370609909)) ;
#56304=CARTESIAN_POINT('Ctrl Pts',(30.464143066922,505.578718967617,-35.4585122521231)) ;
#56305=CARTESIAN_POINT('Origin',(29.888527625402,504.710565160562,-37.0221601717529)) ;
#56306=CARTESIAN_POINT('',(30.464090486888,504.876987562729,-35.458739757252)) ;
#56307=CARTESIAN_POINT('',(30.4640782702768,505.071453548379,-35.4587633355736)) ;
#56308=CARTESIAN_POINT('',(30.4640904799733,504.710565160562,-35.4587397547064)) ;
#56309=CARTESIAN_POINT('',(29.5692971707754,505.710565160562,-35.3870308445011)) ;
#56310=CARTESIAN_POINT('Ctrl Pts',(30.4640782702767,505.071453548379,-35.4587633355736)) ;
#56311=CARTESIAN_POINT('Ctrl Pts',(30.521095886814,505.075779371587,-35.4799146325238)) ;
#56312=CARTESIAN_POINT('Ctrl Pts',(30.5770093172339,505.080082548189,-35.5041983938192)) ;
#56313=CARTESIAN_POINT('Ctrl Pts',(30.6314720687145,505.084322153635,-35.5314549496953)) ;
#56314=CARTESIAN_POINT('Ctrl Pts',(30.6859073887704,505.088559623705,-35.5586977771765)) ;
#56315=CARTESIAN_POINT('Ctrl Pts',(30.7388935375263,505.092733495002,-35.5889103448657)) ;
#56316=CARTESIAN_POINT('Ctrl Pts',(30.7901019141151,505.09682720154,-35.6219030512834)) ;
#56317=CARTESIAN_POINT('Ctrl Pts',(30.841303537339,505.1009203682,-35.6548914066203)) ;
#56318=CARTESIAN_POINT('Ctrl Pts',(30.8907277923682,505.104933423079,-35.6906592105178)) ;
#56319=CARTESIAN_POINT('Ctrl Pts',(30.9380637241444,505.108874530588,-35.7289868532582)) ;
#56320=CARTESIAN_POINT('Ctrl Pts',(30.9854452919855,505.112819437677,-35.7673514472685)) ;
#56321=CARTESIAN_POINT('Ctrl Pts',(31.0307343299584,505.116692408518,-35.8082809470378)) ;
#56322=CARTESIAN_POINT('Ctrl Pts',(31.0736383498221,505.120525064871,-35.8515236587419)) ;
#56323=CARTESIAN_POINT('Ctrl Pts',(31.1165627879252,505.124359545204,-35.8947869498706)) ;
#56324=CARTESIAN_POINT('Ctrl Pts',(31.157099618341,505.128153982491,-35.9403658504486)) ;
#56325=CARTESIAN_POINT('Ctrl Pts',(31.1949789855704,505.131960084758,-35.9879743964208)) ;
#56326=CARTESIAN_POINT('Ctrl Pts',(31.232929820935,505.135773368113,-36.0356727668608)) ;
#56327=CARTESIAN_POINT('Ctrl Pts',(31.2682126114471,505.139598886506,-36.0854086683138)) ;
#56328=CARTESIAN_POINT('Ctrl Pts',(31.3005855087351,505.143502545096,-36.136857261922)) ;
#56329=CARTESIAN_POINT('Ctrl Pts',(31.3266547494785,505.146646082564,-36.1782877758715)) ;
#56330=CARTESIAN_POINT('Ctrl Pts',(31.3508373525747,505.149840752387,-36.2208282201655)) ;
#56331=CARTESIAN_POINT('Ctrl Pts',(31.373025387342,505.153123202999,-36.264290323874)) ;
#56332=CARTESIAN_POINT('Ctrl Pts',(31.3730389005797,505.153125202119,-36.2643167937142)) ;
#56333=CARTESIAN_POINT('Ctrl Pts',(31.3730524130785,505.153127201271,-36.2643432638968)) ;
#56334=CARTESIAN_POINT('Ctrl Pts',(31.3730659248384,505.153129200455,-36.2643697344215)) ;
#56335=CARTESIAN_POINT('Ctrl Pts',(31.3982528864256,505.156855834804,-36.3137128318952)) ;
#56336=CARTESIAN_POINT('Ctrl Pts',(31.420956765697,505.16070546399,-36.3644292075354)) ;
#56337=CARTESIAN_POINT('Ctrl Pts',(31.4410618580961,505.164614959203,-36.4162338892592)) ;
#56338=CARTESIAN_POINT('Ctrl Pts',(31.4429416870201,505.164980497547,-36.4210776341757)) ;
#56339=CARTESIAN_POINT('Ctrl Pts',(31.4447988044912,505.165346559256,-36.4259308565645)) ;
#56340=CARTESIAN_POINT('Ctrl Pts',(31.4466331213465,505.165713092729,-36.4307933009082)) ;
#56341=CARTESIAN_POINT('Ctrl Pts',(31.4683528422139,505.170053130654,-36.488368377742)) ;
#56342=CARTESIAN_POINT('Ctrl Pts',(31.4868749718261,505.174458641855,-36.547242373152)) ;
#56343=CARTESIAN_POINT('Ctrl Pts',(31.5020916321177,505.178858084683,-36.6070223227843)) ;
#56344=CARTESIAN_POINT('Ctrl Pts',(31.5170796559837,505.183191424117,-36.6659040546905)) ;
#56345=CARTESIAN_POINT('Ctrl Pts',(31.5288612462848,505.187518591047,-36.7256647050432)) ;
#56346=CARTESIAN_POINT('Ctrl Pts',(31.5373724102927,505.191791728717,-36.785927153992)) ;
#56347=CARTESIAN_POINT('Ctrl Pts',(31.5458783654769,505.196062251232,-36.8461527223839)) ;
#56348=CARTESIAN_POINT('Ctrl Pts',(31.5511180254007,505.200278675115,-36.9068794869961)) ;
#56349=CARTESIAN_POINT('Ctrl Pts',(31.5530627641506,505.20441698709,-36.9677293364333)) ;
#56350=CARTESIAN_POINT('Ctrl Pts',(31.5550070381138,505.20855431002,-37.0285646429413)) ;
#56351=CARTESIAN_POINT('Ctrl Pts',(31.5536579351739,505.2126135552,-37.0895229550957)) ;
#56352=CARTESIAN_POINT('Ctrl Pts',(31.5490214038572,505.216595484114,-37.1502247919745)) ;
#56353=CARTESIAN_POINT('Ctrl Pts',(31.5442553468897,505.220688651775,-37.2126223889773)) ;
#56354=CARTESIAN_POINT('Ctrl Pts',(31.5360152655613,505.224700130541,-37.2747489134894)) ;
#56355=CARTESIAN_POINT('Ctrl Pts',(31.5243472856465,505.228657089693,-37.3361910850951)) ;
#56356=CARTESIAN_POINT('Ctrl Pts',(31.5129817265898,505.232511488934,-37.3960407450232)) ;
#56357=CARTESIAN_POINT('Ctrl Pts',(31.498363534411,505.236314524773,-37.4552409302377)) ;
#56358=CARTESIAN_POINT('Ctrl Pts',(31.4805754935564,505.24011282074,-37.5134101492967)) ;
#56359=CARTESIAN_POINT('Ctrl Pts',(31.4620774821819,505.244062717335,-37.5739010647714)) ;
#56360=CARTESIAN_POINT('Ctrl Pts',(31.4401507137193,505.248007903713,-37.6332767301028)) ;
#56361=CARTESIAN_POINT('Ctrl Pts',(31.4149400872327,505.252018883781,-37.6911121580904)) ;
#56362=CARTESIAN_POINT('Ctrl Pts',(31.3931146376458,505.255491286314,-37.7411816880382)) ;
#56363=CARTESIAN_POINT('Ctrl Pts',(31.368827773735,505.259013656685,-37.7900977673775)) ;
#56364=CARTESIAN_POINT('Ctrl Pts',(31.3422126922891,505.262636793551,-37.8375881137863)) ;
#56365=CARTESIAN_POINT('Ctrl Pts',(31.3380993813103,505.263196742567,-37.844927657859)) ;
#56366=CARTESIAN_POINT('Ctrl Pts',(31.3339304770256,505.263759098402,-37.852233248156)) ;
#56367=CARTESIAN_POINT('Ctrl Pts',(31.3297064861299,505.264324048576,-37.8595039900052)) ;
#56368=CARTESIAN_POINT('Ctrl Pts',(31.3296913405529,505.264326074266,-37.859530060038)) ;
#56369=CARTESIAN_POINT('Ctrl Pts',(31.3296761942676,505.26432809999,-37.8595561296227)) ;
#56370=CARTESIAN_POINT('Ctrl Pts',(31.3296610472742,505.264330125747,-37.8595821987594)) ;
#56371=CARTESIAN_POINT('Ctrl Pts',(31.3017728603314,505.268059887965,-37.907579906101)) ;
#56372=CARTESIAN_POINT('Ctrl Pts',(31.2713767813286,505.271912555743,-37.9542267962505)) ;
#56373=CARTESIAN_POINT('Ctrl Pts',(31.2386507747087,505.275825029993,-37.9992706142958)) ;
#56374=CARTESIAN_POINT('Ctrl Pts',(31.2355914882052,505.276190775188,-38.0034813921709)) ;
#56375=CARTESIAN_POINT('Ctrl Pts',(31.2325118759833,505.276557043023,-38.007678147697)) ;
#56376=CARTESIAN_POINT('Ctrl Pts',(31.2294121053228,505.27692378195,-38.0118606671151)) ;
#56377=CARTESIAN_POINT('Ctrl Pts',(31.1927870786063,505.281256948653,-38.0612788022653)) ;
#56378=CARTESIAN_POINT('Ctrl Pts',(31.1533424184425,505.285655220766,-38.1087120445306)) ;
#56379=CARTESIAN_POINT('Ctrl Pts',(31.1113494546076,505.290047632902,-38.1538582110569)) ;
#56380=CARTESIAN_POINT('Ctrl Pts',(31.0698905146768,505.294384186797,-38.1984302544467)) ;
#56381=CARTESIAN_POINT('Ctrl Pts',(31.0259479181896,505.298714736299,-38.2407733821669)) ;
#56382=CARTESIAN_POINT('Ctrl Pts',(30.9798051895301,505.302991533763,-38.2806288131767)) ;
#56383=CARTESIAN_POINT('Ctrl Pts',(30.9336907071007,505.307265713189,-38.32045984672)) ;
#56384=CARTESIAN_POINT('Ctrl Pts',(30.8853788424685,505.311486071251,-38.3578063463012)) ;
#56385=CARTESIAN_POINT('Ctrl Pts',(30.8351730602288,505.315628761888,-38.3924387332868)) ;
#56386=CARTESIAN_POINT('Ctrl Pts',(30.784979484531,505.319770445312,-38.4270627000931)) ;
#56387=CARTESIAN_POINT('Ctrl Pts',(30.7328929083336,505.323834497195,-38.4589738385256)) ;
#56388=CARTESIAN_POINT('Ctrl Pts',(30.6792366782967,505.327821892011,-38.4879708705226)) ;
#56389=CARTESIAN_POINT('Ctrl Pts',(30.6243043061247,505.331904121714,-38.5176575583956)) ;
#56390=CARTESIAN_POINT('Ctrl Pts',(30.5677266025114,505.335906031441,-38.5442895646531)) ;
#56391=CARTESIAN_POINT('Ctrl Pts',(30.5098727161521,505.339854660265,-38.5676831579019)) ;
#56392=CARTESIAN_POINT('Ctrl Pts',(30.4532918764318,505.343716401431,-38.5905619865059)) ;
#56393=CARTESIAN_POINT('Ctrl Pts',(30.3954904280474,505.347527534501,-38.6103431478182)) ;
#56394=CARTESIAN_POINT('Ctrl Pts',(30.3368351358503,505.35133479927,-38.6268887086384)) ;
#56395=CARTESIAN_POINT('Ctrl Pts',(30.2762002621473,505.35527055698,-38.6439926723747)) ;
#56396=CARTESIAN_POINT('Ctrl Pts',(30.2146528039645,505.359202610514,-38.657638126504)) ;
#56397=CARTESIAN_POINT('Ctrl Pts',(30.1526223166261,505.363200214559,-38.6677175266866)) ;
#56398=CARTESIAN_POINT('Ctrl Pts',(30.0986341516869,505.366679524746,-38.6764901213073)) ;
#56399=CARTESIAN_POINT('Ctrl Pts',(30.0442792308175,505.370209139025,-38.6825616770159)) ;
#56400=CARTESIAN_POINT('Ctrl Pts',(29.989858990173,505.373839649464,-38.6858959847392)) ;
#56401=CARTESIAN_POINT('Ctrl Pts',(29.9817842858887,505.374378333194,-38.6863907188407)) ;
#56402=CARTESIAN_POINT('Ctrl Pts',(29.9737080742526,505.374919238222,-38.6868252534974)) ;
#56403=CARTESIAN_POINT('Ctrl Pts',(29.9656312655556,505.375462529814,-38.6871995343826)) ;
#56404=CARTESIAN_POINT('Ctrl Pts',(29.9655992751451,505.375464681669,-38.6872010168245)) ;
#56405=CARTESIAN_POINT('Ctrl Pts',(29.9655672847251,505.375466833562,-38.6872024983211)) ;
#56406=CARTESIAN_POINT('Ctrl Pts',(29.9655352942958,505.375468985492,-38.6872039788726)) ;
#56407=CARTESIAN_POINT('Ctrl Pts',(29.910055865614,505.379200971678,-38.6897716264538)) ;
#56408=CARTESIAN_POINT('Ctrl Pts',(29.8543515765862,505.383055234418,-38.689497265412)) ;
#56409=CARTESIAN_POINT('Ctrl Pts',(29.7987318761332,505.386968302999,-38.6863937388079)) ;
#56410=CARTESIAN_POINT('Ctrl Pts',(29.7936788099732,505.387323806432,-38.6861117825022)) ;
#56411=CARTESIAN_POINT('Ctrl Pts',(29.7886264707689,505.387679795235,-38.6858064957554)) ;
#56412=CARTESIAN_POINT('Ctrl Pts',(29.7835751074526,505.388036221814,-38.6854779010942)) ;
#56413=CARTESIAN_POINT('Ctrl Pts',(29.722169189496,505.39236905236,-38.6814834038582)) ;
#56414=CARTESIAN_POINT('Ctrl Pts',(29.6609024128934,505.396765913205,-38.6740413916708)) ;
#56415=CARTESIAN_POINT('Ctrl Pts',(29.6001769888483,505.401155779833,-38.6632161713429)) ;
#56416=CARTESIAN_POINT('Ctrl Pts',(29.5403576390167,505.405480145972,-38.6525524723736)) ;
#56417=CARTESIAN_POINT('Ctrl Pts',(29.4810634358088,505.409797446368,-38.6386061825611)) ;
#56418=CARTESIAN_POINT('Ctrl Pts',(29.4226642303696,505.414060532842,-38.6214749234021)) ;
#56419=CARTESIAN_POINT('Ctrl Pts',(29.3642989539147,505.418321142533,-38.6043536172249)) ;
#56420=CARTESIAN_POINT('Ctrl Pts',(29.3068275724457,505.422527470063,-38.5840511502648)) ;
#56421=CARTESIAN_POINT('Ctrl Pts',(29.250606322394,505.426656364448,-38.5606977303438)) ;
#56422=CARTESIAN_POINT('Ctrl Pts',(29.1943967501594,505.430784401213,-38.5373491612037)) ;
#56423=CARTESIAN_POINT('Ctrl Pts',(29.1394368218155,505.434835037256,-38.5109508832397)) ;
#56424=CARTESIAN_POINT('Ctrl Pts',(29.0860698172838,505.438809997494,-38.4816651878905)) ;
#56425=CARTESIAN_POINT('Ctrl Pts',(29.0312266948075,505.442894904134,-38.4515694575618)) ;
#56426=CARTESIAN_POINT('Ctrl Pts',(28.978066042403,505.44689990356,-38.4184240703072)) ;
#56427=CARTESIAN_POINT('Ctrl Pts',(28.926945092787,505.4508532385,-38.3824417917118)) ;
#56428=CARTESIAN_POINT('Ctrl Pts',(28.8771318783715,505.454705442391,-38.3473799829564)) ;
#56429=CARTESIAN_POINT('Ctrl Pts',(28.8292555258394,505.458508962815,-38.3096245023365)) ;
#56430=CARTESIAN_POINT('Ctrl Pts',(28.7836295441577,505.462311419072,-38.2694087431619)) ;
#56431=CARTESIAN_POINT('Ctrl Pts',(28.7362068494048,505.466263612882,-38.2276093209621)) ;
#56432=CARTESIAN_POINT('Ctrl Pts',(28.6912159086222,505.470215085446,-38.1831514246148)) ;
#56433=CARTESIAN_POINT('Ctrl Pts',(28.6489836710172,505.474237187497,-38.1363428692093)) ;
#56434=CARTESIAN_POINT('Ctrl Pts',(28.6125417380707,505.47770783413,-38.0959520603359)) ;
#56435=CARTESIAN_POINT('Ctrl Pts',(28.5781531172907,505.481231733459,-38.0538103871801)) ;
#56436=CARTESIAN_POINT('Ctrl Pts',(28.5460087664382,505.484859486374,-38.0101497501515)) ;
#56437=CARTESIAN_POINT('Ctrl Pts',(28.540921715463,505.485433601685,-38.0032401725653)) ;
#56438=CARTESIAN_POINT('Ctrl Pts',(28.5358907697851,505.486010318021,-37.9962925253697)) ;
#56439=CARTESIAN_POINT('Ctrl Pts',(28.5309165710722,505.486589835939,-37.9893076939497)) ;
#56440=CARTESIAN_POINT('Ctrl Pts',(28.5308966183035,505.486592160532,-37.9892796760247)) ;
#56441=CARTESIAN_POINT('Ctrl Pts',(28.5308766664477,505.48659448517,-37.9892516575015)) ;
#56442=CARTESIAN_POINT('Ctrl Pts',(28.530856715505,505.486596809853,-37.98922363838)) ;
#56443=CARTESIAN_POINT('Ctrl Pts',(28.4989644475012,505.49031289568,-37.9444341092091)) ;
#56444=CARTESIAN_POINT('Ctrl Pts',(28.4692925350709,505.494154464843,-37.8979427697449)) ;
#56445=CARTESIAN_POINT('Ctrl Pts',(28.4419955250567,505.498058691952,-37.8500096556061)) ;
#56446=CARTESIAN_POINT('Ctrl Pts',(28.4393387204183,505.498438688468,-37.8453443490429)) ;
#56447=CARTESIAN_POINT('Ctrl Pts',(28.43670441025,505.498819278544,-37.8406654251301)) ;
#56448=CARTESIAN_POINT('Ctrl Pts',(28.4340927344234,505.499200404256,-37.8359731497715)) ;
#56449=CARTESIAN_POINT('Ctrl Pts',(28.4041673982211,505.50356745278,-37.7822077029919)) ;
#56450=CARTESIAN_POINT('Ctrl Pts',(28.3772138650138,505.508004129347,-37.7266831668167)) ;
#56451=CARTESIAN_POINT('Ctrl Pts',(28.3533978736318,505.512437125704,-37.6697741685417)) ;
#56452=CARTESIAN_POINT('Ctrl Pts',(28.3300305247356,505.516786613864,-37.6139372144259)) ;
#56453=CARTESIAN_POINT('Ctrl Pts',(28.3096831476368,505.521132276051,-37.5567675619365)) ;
#56454=CARTESIAN_POINT('Ctrl Pts',(28.2924735956573,505.525425110746,-37.4986264512002)) ;
#56455=CARTESIAN_POINT('Ctrl Pts',(28.2752748252914,505.529715256021,-37.4405217652929)) ;
#56456=CARTESIAN_POINT('Ctrl Pts',(28.261209815786,505.533952497417,-37.3814468522232)) ;
#56457=CARTESIAN_POINT('Ctrl Pts',(28.2503614602831,505.538111497103,-37.3217690562125)) ;
#56458=CARTESIAN_POINT('Ctrl Pts',(28.2395157738388,505.542269473536,-37.2621059429372)) ;
#56459=CARTESIAN_POINT('Ctrl Pts',(28.2318851855977,505.546349236226,-37.2018402665271)) ;
#56460=CARTESIAN_POINT('Ctrl Pts',(28.2275185485494,505.55035014595,-37.14134563109)) ;
#56461=CARTESIAN_POINT('Ctrl Pts',(28.2229996175459,505.554490594263,-37.078741141502)) ;
#56462=CARTESIAN_POINT('Ctrl Pts',(28.2219766819324,505.558546560858,-37.0158914609938)) ;
#56463=CARTESIAN_POINT('Ctrl Pts',(28.2244639682465,505.562544359745,-36.9532174210266)) ;
#56464=CARTESIAN_POINT('Ctrl Pts',(28.226870615007,505.566412547209,-36.8925753170618)) ;
#56465=CARTESIAN_POINT('Ctrl Pts',(28.2325636526095,505.570226658843,-36.8320977765136)) ;
#56466=CARTESIAN_POINT('Ctrl Pts',(28.2415163079168,505.574032336457,-36.7721710651033)) ;
#56467=CARTESIAN_POINT('Ctrl Pts',(28.250918928383,505.578029289427,-36.7092324056952)) ;
#56468=CARTESIAN_POINT('Ctrl Pts',(28.2639180144742,505.582017313911,-36.6469015568741)) ;
#56469=CARTESIAN_POINT('Ctrl Pts',(28.2804294752268,505.586068514865,-36.5856292757383)) ;
#56470=CARTESIAN_POINT('Ctrl Pts',(28.2946525214386,505.589558237503,-36.5328490584605)) ;
#56471=CARTESIAN_POINT('Ctrl Pts',(28.3114819201761,505.593095501817,-36.4808533077519)) ;
#56472=CARTESIAN_POINT('Ctrl Pts',(28.3308241855398,505.596732103637,-36.4299323744501)) ;
#56473=CARTESIAN_POINT('Ctrl Pts',(28.3339294830955,505.597315940666,-36.4217572901598)) ;
#56474=CARTESIAN_POINT('Ctrl Pts',(28.3370995170736,505.597902338079,-36.4136098043667)) ;
#56475=CARTESIAN_POINT('Ctrl Pts',(28.3403338676742,505.598491510205,-36.4054909973772)) ;
#56476=CARTESIAN_POINT('Ctrl Pts',(28.3403409220056,505.598492795228,-36.4054732897251)) ;
#56477=CARTESIAN_POINT('Ctrl Pts',(28.340347976643,505.598494080264,-36.4054555822094)) ;
#56478=CARTESIAN_POINT('Ctrl Pts',(28.3403550315863,505.598495365314,-36.4054378748302)) ;
#56479=CARTESIAN_POINT('Ctrl Pts',(28.361155477361,505.602284141862,-36.353230313964)) ;
#56480=CARTESIAN_POINT('Ctrl Pts',(28.3846961235323,505.606197592738,-36.3020279818582)) ;
#56481=CARTESIAN_POINT('Ctrl Pts',(28.4108341231365,505.610173397742,-36.2521099908632)) ;
#56482=CARTESIAN_POINT('Ctrl Pts',(28.4134743662545,505.610575000465,-36.2470676909862)) ;
#56483=CARTESIAN_POINT('Ctrl Pts',(28.4161410727314,505.610977239409,-36.2420385169523)) ;
#56484=CARTESIAN_POINT('Ctrl Pts',(28.4188340691836,505.611380050343,-36.2370227700409)) ;
#56485=CARTESIAN_POINT('Ctrl Pts',(28.4481249715863,505.615761302224,-36.1824680181646)) ;
#56486=CARTESIAN_POINT('Ctrl Pts',(28.480531020835,505.620209584656,-36.1294983574458)) ;
#56487=CARTESIAN_POINT('Ctrl Pts',(28.5158274435636,505.624655609921,-36.078451901193)) ;
#56488=CARTESIAN_POINT('Ctrl Pts',(28.5510800142243,505.629096111471,-36.0274688647571)) ;
#56489=CARTESIAN_POINT('Ctrl Pts',(28.5892155533788,505.633534020205,-35.9784039506105)) ;
#56490=CARTESIAN_POINT('Ctrl Pts',(28.6299836584483,505.63792088294,-35.9315656998075)) ;
#56491=CARTESIAN_POINT('Ctrl Pts',(28.6707138952097,505.642303670845,-35.8847709556944)) ;
#56492=CARTESIAN_POINT('Ctrl Pts',(28.714071767279,505.64663537072,-35.8401985986474)) ;
#56493=CARTESIAN_POINT('Ctrl Pts',(28.7597830356109,505.650891718927,-35.798131407424)) ;
#56494=CARTESIAN_POINT('Ctrl Pts',(28.8054661625882,505.655145446786,-35.7560901141419)) ;
#56495=CARTESIAN_POINT('Ctrl Pts',(28.853499841945,505.659323922623,-35.7165509234305)) ;
#56496=CARTESIAN_POINT('Ctrl Pts',(28.9035856874473,505.663427902196,-35.6797720977196)) ;
#56497=CARTESIAN_POINT('Ctrl Pts',(28.9536755208936,505.667532208537,-35.6429903435986)) ;
#56498=CARTESIAN_POINT('Ctrl Pts',(29.0058179585603,505.671562141034,-35.6089695679321)) ;
#56499=CARTESIAN_POINT('Ctrl Pts',(29.0596886201874,505.675542395257,-35.577942630958)) ;
#56500=CARTESIAN_POINT('Ctrl Pts',(29.1135569296164,505.679522475687,-35.546917048738)) ;
#56501=CARTESIAN_POINT('Ctrl Pts',(29.1691534513111,505.683453174641,-35.5188853886785)) ;
#56502=CARTESIAN_POINT('Ctrl Pts',(29.2261260138388,505.687379963192,-35.4940511678207)) ;
#56503=CARTESIAN_POINT('Ctrl Pts',(29.2831544935491,505.69131060579,-35.4691925727801)) ;
#56504=CARTESIAN_POINT('Ctrl Pts',(29.3415618192553,505.695237834327,-35.4475382706051)) ;
#56505=CARTESIAN_POINT('Ctrl Pts',(29.4009649620739,505.69922216151,-35.4292561559619)) ;
#56506=CARTESIAN_POINT('Ctrl Pts',(29.4563224157855,505.702935133537,-35.4122191564516)) ;
#56507=CARTESIAN_POINT('Ctrl Pts',(29.5125442978946,505.706698340933,-35.3981108521241)) ;
#56508=CARTESIAN_POINT('Ctrl Pts',(29.5692971707753,505.710565160562,-35.3870308445009)) ;
#56509=CARTESIAN_POINT('Origin',(29.8885276254021,505.710565160562,-37.0221601717529)) ;
#56510=CARTESIAN_POINT('Ctrl Pts',(30.4640904938027,504.876987562729,-35.4587397597976)) ;
#56511=CARTESIAN_POINT('Ctrl Pts',(30.4869337999252,504.878606326814,-35.4671493716302)) ;
#56512=CARTESIAN_POINT('Ctrl Pts',(30.5095919064472,504.880241842228,-35.4760593026279)) ;
#56513=CARTESIAN_POINT('Ctrl Pts',(30.5969398749291,504.886669676781,-35.5126379224649)) ;
#56514=CARTESIAN_POINT('Ctrl Pts',(30.6600356443181,504.891583087799,-35.5438915012115)) ;
#56515=CARTESIAN_POINT('Ctrl Pts',(30.8112018494661,504.904035861512,-35.631088162206)) ;
#56516=CARTESIAN_POINT('Ctrl Pts',(30.8963581682533,504.91168516546,-35.6914896998207)) ;
#56517=CARTESIAN_POINT('Ctrl Pts',(31.0183684306797,504.923328324557,-35.7964997827966)) ;
#56518=CARTESIAN_POINT('Ctrl Pts',(31.0595092459496,504.927391497997,-35.8357424522067)) ;
#56519=CARTESIAN_POINT('Ctrl Pts',(31.1193420758518,504.933422332971,-35.8989659670094)) ;
#56520=CARTESIAN_POINT('Ctrl Pts',(31.139517178829,504.935477752932,-35.9214807707376)) ;
#56521=CARTESIAN_POINT('Ctrl Pts',(31.1861826459071,504.94027152647,-35.9765005393346)) ;
#56522=CARTESIAN_POINT('Ctrl Pts',(31.2120797784735,504.942972035025,-36.0094790518896)) ;
#56523=CARTESIAN_POINT('Ctrl Pts',(31.2717458874835,504.949392045973,-36.0916655653749)) ;
#56524=CARTESIAN_POINT('Ctrl Pts',(31.3041695307979,504.953055753782,-36.1417784788156)) ;
#56525=CARTESIAN_POINT('Ctrl Pts',(31.3963108705091,504.964382928952,-36.3024919662609)) ;
#56526=CARTESIAN_POINT('Ctrl Pts',(31.4462548894849,504.971984508305,-36.4181612414627)) ;
#56527=CARTESIAN_POINT('Ctrl Pts',(31.4976383669698,504.983351232614,-36.5874707561682)) ;
#56528=CARTESIAN_POINT('Ctrl Pts',(31.5102685142421,504.986715794551,-36.6372604475614)) ;
#56529=CARTESIAN_POINT('Ctrl Pts',(31.5322736830597,504.994062191278,-36.7445899001118)) ;
#56530=CARTESIAN_POINT('Ctrl Pts',(31.5409685806546,504.998061606725,-36.8021970301492)) ;
#56531=CARTESIAN_POINT('Ctrl Pts',(31.5533834565238,505.00702110329,-36.9292462563812)) ;
#56532=CARTESIAN_POINT('Ctrl Pts',(31.5558086545656,505.012010252248,-36.9987050410494)) ;
#56533=CARTESIAN_POINT('Ctrl Pts',(31.5506638408612,505.025550526036,-37.1851850933535)) ;
#56534=CARTESIAN_POINT('Ctrl Pts',(31.5350964495807,505.034174280405,-37.3016039753621)) ;
#56535=CARTESIAN_POINT('Ctrl Pts',(31.5003271382971,505.04439270362,-37.4447325775823)) ;
#56536=CARTESIAN_POINT('Ctrl Pts',(31.4924147812081,505.046447069871,-37.4738366955062)) ;
#56537=CARTESIAN_POINT('Ctrl Pts',(31.4720493303971,505.051146763743,-37.5414390832326)) ;
#56538=CARTESIAN_POINT('Ctrl Pts',(31.458976426799,505.053759286329,-37.5797288360284)) ;
#56539=CARTESIAN_POINT('Ctrl Pts',(31.4244820998282,505.059876520636,-37.6698827050114)) ;
#56540=CARTESIAN_POINT('Ctrl Pts',(31.4018098630181,505.063332533912,-37.7212155100859)) ;
#56541=CARTESIAN_POINT('Ctrl Pts',(31.3158637014097,505.075034591258,-37.8919333679364)) ;
#56542=CARTESIAN_POINT('Ctrl Pts',(31.2407040325545,505.083174245486,-38.0047123934386)) ;
#56543=CARTESIAN_POINT('Ctrl Pts',(31.1199440684997,505.095114223618,-38.145418171556)) ;
#56544=CARTESIAN_POINT('Ctrl Pts',(31.085413035751,505.098423444659,-38.1821426676398)) ;
#56545=CARTESIAN_POINT('Ctrl Pts',(31.0066437838756,505.105799002943,-38.2586487533931)) ;
#56546=CARTESIAN_POINT('Ctrl Pts',(30.9618338916185,505.109889866297,-38.2977384194287)) ;
#56547=CARTESIAN_POINT('Ctrl Pts',(30.8580579644143,505.119157797996,-38.3789211309444)) ;
#56548=CARTESIAN_POINT('Ctrl Pts',(30.7982420997301,505.124369394691,-38.4197320168323)) ;
#56549=CARTESIAN_POINT('Ctrl Pts',(30.6425261494663,505.137513556364,-38.5117311762407)) ;
#56550=CARTESIAN_POINT('Ctrl Pts',(30.5439051631561,505.145481882937,-38.5576794254582)) ;
#56551=CARTESIAN_POINT('Ctrl Pts',(30.4122557784069,505.155189801372,-38.6040029390564)) ;
#56552=CARTESIAN_POINT('Ctrl Pts',(30.3827166441987,505.157308963363,-38.6134789835817)) ;
#56553=CARTESIAN_POINT('Ctrl Pts',(30.3155720821077,505.161973058499,-38.6329679746827)) ;
#56554=CARTESIAN_POINT('Ctrl Pts',(30.2778475830031,505.164493237266,-38.6424994365393)) ;
#56555=CARTESIAN_POINT('Ctrl Pts',(30.1885140705319,505.170302414477,-38.6617695595558)) ;
#56556=CARTESIAN_POINT('Ctrl Pts',(30.1367097335577,505.173549603447,-38.6704068862994)) ;
#56557=CARTESIAN_POINT('Ctrl Pts',(29.9488542251005,505.185155725715,-38.6926682035512)) ;
#56558=CARTESIAN_POINT('Ctrl Pts',(29.8116775425696,505.193362887803,-38.6919888024947)) ;
#56559=CARTESIAN_POINT('Ctrl Pts',(29.624855350619,505.205444366386,-38.6679745984017)) ;
#56560=CARTESIAN_POINT('Ctrl Pts',(29.5739237617302,505.208826330338,-38.6590021411539)) ;
#56561=CARTESIAN_POINT('Ctrl Pts',(29.4675277637266,505.216127724888,-38.6351094876978)) ;
#56562=CARTESIAN_POINT('Ctrl Pts',(29.41225300412,505.22006081354,-38.6196605510268)) ;
#56563=CARTESIAN_POINT('Ctrl Pts',(29.2939961228177,505.228801051977,-38.5799251294602)) ;
#56564=CARTESIAN_POINT('Ctrl Pts',(29.2314701995677,505.233633562076,-38.554600462466)) ;
#56565=CARTESIAN_POINT('Ctrl Pts',(29.064866655393,505.247017025115,-38.4750474777764)) ;
#56566=CARTESIAN_POINT('Ctrl Pts',(28.9647006331844,505.255656762407,-38.4135068552996)) ;
#56567=CARTESIAN_POINT('Ctrl Pts',(28.8467901819903,505.266031924647,-38.3226744868733)) ;
#56568=CARTESIAN_POINT('Ctrl Pts',(28.8223090351299,505.2681963671,-38.3026807437247)) ;
#56569=CARTESIAN_POINT('Ctrl Pts',(28.7699718567068,505.272822773724,-38.2573941485137)) ;
#56570=CARTESIAN_POINT('Ctrl Pts',(28.7423745303495,505.275265998877,-38.2318310516059)) ;
#56571=CARTESIAN_POINT('Ctrl Pts',(28.6804139252238,505.280827135552,-38.1704113439542)) ;
#56572=CARTESIAN_POINT('Ctrl Pts',(28.6467408006178,505.283908462598,-38.1339090892676)) ;
#56573=CARTESIAN_POINT('Ctrl Pts',(28.5177073059866,505.296218322076,-37.9808440181915)) ;
#56574=CARTESIAN_POINT('Ctrl Pts',(28.436728725186,505.305222181149,-37.853123558032)) ;
#56575=CARTESIAN_POINT('Ctrl Pts',(28.3529740128628,505.318205848838,-37.6703728001715)) ;
#56576=CARTESIAN_POINT('Ctrl Pts',(28.334040353043,505.321532015094,-37.6235526394832)) ;
#56577=CARTESIAN_POINT('Ctrl Pts',(28.2966593623614,505.329109436808,-37.5174915946331)) ;
#56578=CARTESIAN_POINT('Ctrl Pts',(28.2793370467759,505.333393656728,-37.4579373245657)) ;
#56579=CARTESIAN_POINT('Ctrl Pts',(28.2288907648697,505.349207042725,-37.2398193604818)) ;
#56580=CARTESIAN_POINT('Ctrl Pts',(28.2156013177303,505.361293063839,-37.0776284436838)) ;
#56581=CARTESIAN_POINT('Ctrl Pts',(28.228191571231,505.375231915385,-36.8802928531777)) ;
#56582=CARTESIAN_POINT('Ctrl Pts',(28.2316303213961,505.377718228363,-36.8445820480625)) ;
#56583=CARTESIAN_POINT('Ctrl Pts',(28.2403577626611,505.382325518337,-36.7769292816497)) ;
#56584=CARTESIAN_POINT('Ctrl Pts',(28.2454292806503,505.384455016644,-36.7449776845084)) ;
#56585=CARTESIAN_POINT('Ctrl Pts',(28.2586443512131,505.389058212253,-36.674956229427)) ;
#56586=CARTESIAN_POINT('Ctrl Pts',(28.2671984852559,505.39151304728,-36.6369818548884)) ;
#56587=CARTESIAN_POINT('Ctrl Pts',(28.301076026269,505.399822747872,-36.5078679897967)) ;
#56588=CARTESIAN_POINT('Ctrl Pts',(28.3328221189001,505.405512572982,-36.4186033051751)) ;
#56589=CARTESIAN_POINT('Ctrl Pts',(28.4059772909885,505.41637075183,-36.2577331543419)) ;
#56590=CARTESIAN_POINT('Ctrl Pts',(28.4454622972825,505.421493596654,-36.1855813807272)) ;
#56591=CARTESIAN_POINT('Ctrl Pts',(28.5172672186643,505.430045411399,-36.0746905944075)) ;
#56592=CARTESIAN_POINT('Ctrl Pts',(28.5463022170203,505.433346024103,-36.0339882514493)) ;
#56593=CARTESIAN_POINT('Ctrl Pts',(28.6163113509271,505.441011148693,-35.9446353501423)) ;
#56594=CARTESIAN_POINT('Ctrl Pts',(28.6583272987636,505.445415879141,-35.8969049674629)) ;
#56595=CARTESIAN_POINT('Ctrl Pts',(28.7613552212687,505.455804280732,-35.7925477787027)) ;
#56596=CARTESIAN_POINT('Ctrl Pts',(28.8240886310708,505.461845247271,-35.7378582062474)) ;
#56597=CARTESIAN_POINT('Ctrl Pts',(28.9576212240075,505.473996343706,-35.6379754768635)) ;
#56598=CARTESIAN_POINT('Ctrl Pts',(29.0282934864003,505.4800887769,-35.5929807957488)) ;
#56599=CARTESIAN_POINT('Ctrl Pts',(29.1305594213015,505.488201968313,-35.53821748958)) ;
#56600=CARTESIAN_POINT('Ctrl Pts',(29.159508920795,505.490424919367,-35.5237830352619)) ;
#56601=CARTESIAN_POINT('Ctrl Pts',(29.2218806074471,505.495033449199,-35.4949204369125)) ;
#56602=CARTESIAN_POINT('Ctrl Pts',(29.2553911764646,505.497406626614,-35.4807263531862)) ;
#56603=CARTESIAN_POINT('Ctrl Pts',(29.3876437604648,505.506478834398,-35.4297500362299)) ;
#56604=CARTESIAN_POINT('Ctrl Pts',(29.4893271533635,505.512841545071,-35.4012658788438)) ;
#56605=CARTESIAN_POINT('Ctrl Pts',(29.6850219576468,505.525024427307,-35.3659962036172)) ;
#56606=CARTESIAN_POINT('Ctrl Pts',(29.7782362896289,505.530803751587,-35.3571897627624)) ;
#56607=CARTESIAN_POINT('Ctrl Pts',(29.9228101220036,505.540125589335,-35.3557286069205)) ;
#56608=CARTESIAN_POINT('Ctrl Pts',(29.9739208018959,505.543487594534,-35.3575651743944)) ;
#56609=CARTESIAN_POINT('Ctrl Pts',(30.0852175886486,505.550999961024,-35.3667036136506)) ;
#56610=CARTESIAN_POINT('Ctrl Pts',(30.1452504613554,505.555176250007,-35.3749458216379)) ;
#56611=CARTESIAN_POINT('Ctrl Pts',(30.2929665423896,505.56577908599,-35.4034977446196)) ;
#56612=CARTESIAN_POINT('Ctrl Pts',(30.3797023347075,505.572304017086,-35.4276750353455)) ;
#56613=CARTESIAN_POINT('Ctrl Pts',(30.4640543092331,505.578851962161,-35.4587264391634)) ;
#56614=CARTESIAN_POINT('Origin',(29.888527625402,504.710565160562,-37.0221601717529)) ;
#56615=CARTESIAN_POINT('',(30.4640904799732,504.178934308784,-35.4587397547064)) ;
#56616=CARTESIAN_POINT('',(30.4640904797602,504.369620557053,-35.458739754628)) ;
#56617=CARTESIAN_POINT('',(30.4640904799733,504.710565160562,-35.4587397547064)) ;
#56618=CARTESIAN_POINT('',(29.8896377004414,504.139875734639,-35.3557043533874)) ;
#56619=CARTESIAN_POINT('Ctrl Pts',(29.8896184786969,504.140137457474,-35.3561605288841)) ;
#56620=CARTESIAN_POINT('Ctrl Pts',(29.9354901762523,504.143454067397,-35.3561905644802)) ;
#56621=CARTESIAN_POINT('Ctrl Pts',(29.9813446690112,504.146743004584,-35.3581151472982)) ;
#56622=CARTESIAN_POINT('Ctrl Pts',(30.0577028173439,504.152121209803,-35.3644868009658)) ;
#56623=CARTESIAN_POINT('Ctrl Pts',(30.0882673386681,504.154247226243,-35.3678912625542)) ;
#56624=CARTESIAN_POINT('Ctrl Pts',(30.1501713170452,504.158475770452,-35.3765275127624)) ;
#56625=CARTESIAN_POINT('Ctrl Pts',(30.1814886437172,504.160570984008,-35.3818131807617)) ;
#56626=CARTESIAN_POINT('Ctrl Pts',(30.2982115134967,504.168273320549,-35.4049631832909)) ;
#56627=CARTESIAN_POINT('Ctrl Pts',(30.3822863928015,504.173613655647,-35.4286241227147)) ;
#56628=CARTESIAN_POINT('Ctrl Pts',(30.4640904799732,504.178934308784,-35.4587397547064)) ;
#56629=CARTESIAN_POINT('',(30.967886278449,503.710565160562,-38.2912310516064)) ;
#56630=CARTESIAN_POINT('Ctrl Pts',(29.8896377004414,504.13987573464,-35.3557043533874)) ;
#56631=CARTESIAN_POINT('Ctrl Pts',(29.8297753933383,504.135625997494,-35.3557985198437)) ;
#56632=CARTESIAN_POINT('Ctrl Pts',(29.7698127451484,504.131337054551,-35.3591450254465)) ;
#56633=CARTESIAN_POINT('Ctrl Pts',(29.7101270449706,504.127068870349,-35.3657190559218)) ;
#56634=CARTESIAN_POINT('Ctrl Pts',(29.6505061160716,504.122805318007,-35.3722859522198)) ;
#56635=CARTESIAN_POINT('Ctrl Pts',(29.5911614984541,504.118562737948,-35.3820731346348)) ;
#56636=CARTESIAN_POINT('Ctrl Pts',(29.5324607005304,504.114380610146,-35.3950189269347)) ;
#56637=CARTESIAN_POINT('Ctrl Pts',(29.4738005852685,504.110201380773,-35.4079557471369)) ;
#56638=CARTESIAN_POINT('Ctrl Pts',(29.4157834169584,504.106082618206,-35.4240467306655)) ;
#56639=CARTESIAN_POINT('Ctrl Pts',(29.3587675571641,504.102040827175,-35.4431956488098)) ;
#56640=CARTESIAN_POINT('Ctrl Pts',(29.3017686658876,504.098000239025,-35.4623388680352)) ;
#56641=CARTESIAN_POINT('Ctrl Pts',(29.2457705803453,504.094036554324,-35.4845382446598)) ;
#56642=CARTESIAN_POINT('Ctrl Pts',(29.1911221195583,504.090142823904,-35.5096631290411)) ;
#56643=CARTESIAN_POINT('Ctrl Pts',(29.1364297668549,504.086245966163,-35.5348081929353)) ;
#56644=CARTESIAN_POINT('Ctrl Pts',(29.0830893815187,504.082419037368,-35.5628836052255)) ;
#56645=CARTESIAN_POINT('Ctrl Pts',(29.0314393914955,504.078632770265,-35.5937224525954)) ;
#56646=CARTESIAN_POINT('Ctrl Pts',(28.9797702420691,504.074845098657,-35.6245727395399)) ;
#56647=CARTESIAN_POINT('Ctrl Pts',(28.9297930245083,504.071097829093,-35.6581887352351)) ;
#56648=CARTESIAN_POINT('Ctrl Pts',(28.8818319358433,504.067342520788,-35.6943646557727)) ;
#56649=CARTESIAN_POINT('Ctrl Pts',(28.8337820826919,504.063580262306,-35.7306075292737)) ;
#56650=CARTESIAN_POINT('Ctrl Pts',(28.7877563004684,504.059809445068,-35.7694201009957)) ;
#56651=CARTESIAN_POINT('Ctrl Pts',(28.7440603511994,504.055967948101,-35.8105526977708)) ;
#56652=CARTESIAN_POINT('Ctrl Pts',(28.705798343014,504.052604172034,-35.8465701268648)) ;
#56653=CARTESIAN_POINT('Ctrl Pts',(28.6693227631056,504.049185674405,-35.884365880256)) ;
#56654=CARTESIAN_POINT('Ctrl Pts',(28.6348207573405,504.045667820509,-35.923743040089)) ;
#56655=CARTESIAN_POINT('Ctrl Pts',(28.6347996521938,504.04566566861,-35.9237671274057)) ;
#56656=CARTESIAN_POINT('Ctrl Pts',(28.634778547784,504.045663516674,-35.9237912153142)) ;
#56657=CARTESIAN_POINT('Ctrl Pts',(28.6347574441113,504.045661364701,-35.9238153038146)) ;
#56658=CARTESIAN_POINT('Ctrl Pts',(28.5981591185791,504.041929378649,-35.9655899651101)) ;
#56659=CARTESIAN_POINT('Ctrl Pts',(28.5636425667076,504.038075115991,-36.0093123926301)) ;
#56660=CARTESIAN_POINT('Ctrl Pts',(28.5313906856171,504.034162047438,-36.0547326419516)) ;
#56661=CARTESIAN_POINT('Ctrl Pts',(28.5284605915725,504.033806543868,-36.0588590865973)) ;
#56662=CARTESIAN_POINT('Ctrl Pts',(28.5255491912652,504.033450554927,-36.0629995091889)) ;
#56663=CARTESIAN_POINT('Ctrl Pts',(28.5226566222899,504.033094128209,-36.0671537010576)) ;
#56664=CARTESIAN_POINT('Ctrl Pts',(28.4874936832043,504.028761297747,-36.1176533077655)) ;
#56665=CARTESIAN_POINT('Ctrl Pts',(28.4551128729339,504.024364436927,-36.1701936196456)) ;
#56666=CARTESIAN_POINT('Ctrl Pts',(28.4257146889389,504.019974570264,-36.2244200807017)) ;
#56667=CARTESIAN_POINT('Ctrl Pts',(28.3967551490687,504.015650203879,-36.2778374401289)) ;
#56668=CARTESIAN_POINT('Ctrl Pts',(28.3706894657574,504.011332903179,-36.3328908853468)) ;
#56669=CARTESIAN_POINT('Ctrl Pts',(28.347671913857,504.007069816351,-36.3892303890599)) ;
#56670=CARTESIAN_POINT('Ctrl Pts',(28.3246677347717,504.002809206305,-36.4455371604577)) ;
#56671=CARTESIAN_POINT('Ctrl Pts',(28.3047080218695,503.99860287837,-36.503128477941)) ;
#56672=CARTESIAN_POINT('Ctrl Pts',(28.2879130843532,503.994473983533,-36.561644641388)) ;
#56673=CARTESIAN_POINT('Ctrl Pts',(28.2711216353392,503.990345946314,-36.6201486503526)) ;
#56674=CARTESIAN_POINT('Ctrl Pts',(28.2574936850388,503.98629530977,-36.6795771107382)) ;
#56675=CARTESIAN_POINT('Ctrl Pts',(28.2471163804212,503.982320348983,-36.7395604484235)) ;
#56676=CARTESIAN_POINT('Ctrl Pts',(28.2364520430735,503.978235442128,-36.8012029049085)) ;
#56677=CARTESIAN_POINT('Ctrl Pts',(28.2292210259891,503.974230442421,-36.8634313832066)) ;
#56678=CARTESIAN_POINT('Ctrl Pts',(28.2254797132738,503.970277107139,-36.9258339304508)) ;
#56679=CARTESIAN_POINT('Ctrl Pts',(28.2218341075122,503.966424902584,-36.9866401509081)) ;
#56680=CARTESIAN_POINT('Ctrl Pts',(28.221502112962,503.962621381447,-37.0476115487152)) ;
#56681=CARTESIAN_POINT('Ctrl Pts',(28.2244967250289,503.95881892442,-37.1083574943258)) ;
#56682=CARTESIAN_POINT('Ctrl Pts',(28.227609262024,503.95486673031,-37.1714955565514)) ;
#56683=CARTESIAN_POINT('Ctrl Pts',(28.2343164508115,503.950915257385,-37.2343899285392)) ;
#56684=CARTESIAN_POINT('Ctrl Pts',(28.2445814813765,503.946893154926,-37.2965930716829)) ;
#56685=CARTESIAN_POINT('Ctrl Pts',(28.253439112898,503.943422507539,-37.3502677800003)) ;
#56686=CARTESIAN_POINT('Ctrl Pts',(28.2649458444713,503.939898607407,-37.4034287902758)) ;
#56687=CARTESIAN_POINT('Ctrl Pts',(28.2790394292767,503.936270853637,-37.4557822181718)) ;
#56688=CARTESIAN_POINT('Ctrl Pts',(28.2812698280105,503.93569673871,-37.4640674785155)) ;
#56689=CARTESIAN_POINT('Ctrl Pts',(28.283564971728,503.935120022762,-37.4723326100216)) ;
#56690=CARTESIAN_POINT('Ctrl Pts',(28.2859245682816,503.934540505235,-37.4805765589885)) ;
#56691=CARTESIAN_POINT('Ctrl Pts',(28.2859340333552,503.93453818061,-37.4806096280249)) ;
#56692=CARTESIAN_POINT('Ctrl Pts',(28.285943499466,503.934535855941,-37.4806426967205)) ;
#56693=CARTESIAN_POINT('Ctrl Pts',(28.2859529666137,503.934533531226,-37.4806757650752)) ;
#56694=CARTESIAN_POINT('Ctrl Pts',(28.3010863252409,503.930817444538,-37.5335359597196)) ;
#56695=CARTESIAN_POINT('Ctrl Pts',(28.3189345818505,503.92697587446,-37.5857212719082)) ;
#56696=CARTESIAN_POINT('Ctrl Pts',(28.3393907908243,503.923071646374,-37.6369487425217)) ;
#56697=CARTESIAN_POINT('Ctrl Pts',(28.3413817859688,503.92269164932,-37.6419346930168)) ;
#56698=CARTESIAN_POINT('Ctrl Pts',(28.3433974527172,503.922311058702,-37.6469115468851)) ;
#56699=CARTESIAN_POINT('Ctrl Pts',(28.3454376703857,503.921929932447,-37.6518790289816)) ;
#56700=CARTESIAN_POINT('Ctrl Pts',(28.3688150453601,503.917562883034,-37.7087978045812)) ;
#56701=CARTESIAN_POINT('Ctrl Pts',(28.3954206204328,503.913126205515,-37.7644899055475)) ;
#56702=CARTESIAN_POINT('Ctrl Pts',(28.4250648367456,503.908693208131,-37.818592175824)) ;
#56703=CARTESIAN_POINT('Ctrl Pts',(28.4541506235245,503.904343718324,-37.8716752825222)) ;
#56704=CARTESIAN_POINT('Ctrl Pts',(28.4861612781874,503.89999805442,-37.9232282038626)) ;
#56705=CARTESIAN_POINT('Ctrl Pts',(28.5208878521764,503.895705217961,-37.9729335687876)) ;
#56706=CARTESIAN_POINT('Ctrl Pts',(28.5555926701839,503.891415070938,-38.0226077936124)) ;
#56707=CARTESIAN_POINT('Ctrl Pts',(28.5930099109725,503.887177827747,-38.070436872033)) ;
#56708=CARTESIAN_POINT('Ctrl Pts',(28.632904056294,503.883018826242,-38.1161269601138)) ;
#56709=CARTESIAN_POINT('Ctrl Pts',(28.6727883861652,503.878860848006,-38.1618058067258)) ;
#56710=CARTESIAN_POINT('Ctrl Pts',(28.7151484004903,503.874781083488,-38.2053466799925)) ;
#56711=CARTESIAN_POINT('Ctrl Pts',(28.7597224631518,503.870780171933,-38.2464784466566)) ;
#56712=CARTESIAN_POINT('Ctrl Pts',(28.8058511114513,503.866639722734,-38.2890447438503)) ;
#56713=CARTESIAN_POINT('Ctrl Pts',(28.8543511747747,503.862583755205,-38.3290306366314)) ;
#56714=CARTESIAN_POINT('Ctrl Pts',(28.904902504156,503.858585955385,-38.366162618192)) ;
#56715=CARTESIAN_POINT('Ctrl Pts',(28.9538149356172,503.854717766119,-38.4020907634124)) ;
#56716=CARTESIAN_POINT('Ctrl Pts',(29.0046477380894,503.850903652708,-38.435346900776)) ;
#56717=CARTESIAN_POINT('Ctrl Pts',(29.0570822240754,503.847097973371,-38.4657111295024)) ;
#56718=CARTESIAN_POINT('Ctrl Pts',(29.1121520759834,503.843101019962,-38.4976014693774)) ;
#56719=CARTESIAN_POINT('Ctrl Pts',(29.1689890816134,503.839112995089,-38.5263010170895)) ;
#56720=CARTESIAN_POINT('Ctrl Pts',(29.2271883953978,503.835061793906,-38.5515944752049)) ;
#56721=CARTESIAN_POINT('Ctrl Pts',(29.2773215666856,503.83157206955,-38.573382382754)) ;
#56722=CARTESIAN_POINT('Ctrl Pts',(29.3284664523474,503.828034803596,-38.5926434539553)) ;
#56723=CARTESIAN_POINT('Ctrl Pts',(29.3803377593518,503.82439820022,-38.609269748101)) ;
#56724=CARTESIAN_POINT('Ctrl Pts',(29.3886653951022,503.823814364762,-38.6119390026372)) ;
#56725=CARTESIAN_POINT('Ctrl Pts',(29.397011815879,503.823227968938,-38.6145404372129)) ;
#56726=CARTESIAN_POINT('Ctrl Pts',(29.4053759153336,503.822638798422,-38.6170737064832)) ;
#56727=CARTESIAN_POINT('Ctrl Pts',(29.4053941577726,503.822637513417,-38.6170792316459)) ;
#56728=CARTESIAN_POINT('Ctrl Pts',(29.4054124002957,503.822636228399,-38.6170847564843)) ;
#56729=CARTESIAN_POINT('Ctrl Pts',(29.4054306429029,503.822634943368,-38.6170902809985)) ;
#56730=CARTESIAN_POINT('Ctrl Pts',(29.4592170276719,503.81884616597,-38.6333787228135)) ;
#56731=CARTESIAN_POINT('Ctrl Pts',(29.5139259802935,503.814932714415,-38.6468980394685)) ;
#56732=CARTESIAN_POINT('Ctrl Pts',(29.5692502182216,503.810956908925,-38.6575858894562)) ;
#56733=CARTESIAN_POINT('Ctrl Pts',(29.5748385967441,503.810555307261,-38.6586654841069)) ;
#56734=CARTESIAN_POINT('Ctrl Pts',(29.5804332126718,503.81015306938,-38.6597162051964)) ;
#56735=CARTESIAN_POINT('Ctrl Pts',(29.5860337223545,503.809750259515,-38.660738000437)) ;
#56736=CARTESIAN_POINT('Ctrl Pts',(29.6469489136165,503.80536900827,-38.67185178401)) ;
#56737=CARTESIAN_POINT('Ctrl Pts',(29.7085670930393,503.800920726721,-38.6795417607742)) ;
#56738=CARTESIAN_POINT('Ctrl Pts',(29.7704837692506,503.796474702529,-38.6837728553795)) ;
#56739=CARTESIAN_POINT('Ctrl Pts',(29.8323235206938,503.792034202041,-38.6879986933076)) ;
#56740=CARTESIAN_POINT('Ctrl Pts',(29.8944611253984,503.787596294557,-38.6887746071938)) ;
#56741=CARTESIAN_POINT('Ctrl Pts',(29.9564992329331,503.783209433205,-38.6861039974028)) ;
#56742=CARTESIAN_POINT('Ctrl Pts',(30.0184797152543,503.778826646668,-38.6834358682558)) ;
#56743=CARTESIAN_POINT('Ctrl Pts',(30.0803609695488,503.774494948293,-38.6773277365287)) ;
#56744=CARTESIAN_POINT('Ctrl Pts',(30.1417509253501,503.770238601661,-38.6678177012168)) ;
#56745=CARTESIAN_POINT('Ctrl Pts',(30.2031030876977,503.76598487536,-38.658313520561)) ;
#56746=CARTESIAN_POINT('Ctrl Pts',(30.2639645733628,503.761806401157,-38.6454115696398)) ;
#56747=CARTESIAN_POINT('Ctrl Pts',(30.3239474239815,503.757702423242,-38.6291841121664)) ;
#56748=CARTESIAN_POINT('Ctrl Pts',(30.3839350510104,503.753598118529,-38.6129553625071)) ;
#56749=CARTESIAN_POINT('Ctrl Pts',(30.443043836497,503.749568187684,-38.5934003812633)) ;
#56750=CARTESIAN_POINT('Ctrl Pts',(30.5008894752955,503.745587935094,-38.5706275931094)) ;
#56751=CARTESIAN_POINT('Ctrl Pts',(30.5587325885659,503.741607856281,-38.5478557992106)) ;
#56752=CARTESIAN_POINT('Ctrl Pts',(30.6153124825885,503.737677158926,-38.521866155478)) ;
#56753=CARTESIAN_POINT('Ctrl Pts',(30.6702504661428,503.733750371915,-38.4928071097867)) ;
#56754=CARTESIAN_POINT('Ctrl Pts',(30.7252423704966,503.729819730822,-38.4637195430818)) ;
#56755=CARTESIAN_POINT('Ctrl Pts',(30.7785887549332,503.725892503731,-38.4315561080091)) ;
#56756=CARTESIAN_POINT('Ctrl Pts',(30.8299195396226,503.721908177903,-38.3965115879629)) ;
#56757=CARTESIAN_POINT('Ctrl Pts',(30.8777544982746,503.718195200156,-38.3638537360025)) ;
#56758=CARTESIAN_POINT('Ctrl Pts',(30.9238386672376,503.714431986771,-38.3286940263402)) ;
#56759=CARTESIAN_POINT('Ctrl Pts',(30.9678862784492,503.710565160562,-38.2912310516066)) ;
#56760=CARTESIAN_POINT('',(30.9857908490243,503.71057263878,-35.7673864800448)) ;
#56761=CARTESIAN_POINT('Origin',(29.8885276254018,503.710565160562,-37.0221601717529)) ;
#56762=CARTESIAN_POINT('',(29.8893873868701,504.332876521313,-35.3566407257823)) ;
#56763=CARTESIAN_POINT('Ctrl Pts',(30.9857908596378,503.710572638919,-35.7673864679078)) ;
#56764=CARTESIAN_POINT('Ctrl Pts',(31.025599741794,503.714185585541,-35.8022396077763)) ;
#56765=CARTESIAN_POINT('Ctrl Pts',(31.0637788842238,503.717896060089,-35.8390918157986)) ;
#56766=CARTESIAN_POINT('Ctrl Pts',(31.1001381250373,503.721649614921,-35.8777491764167)) ;
#56767=CARTESIAN_POINT('Ctrl Pts',(31.1415669230504,503.725926526691,-35.9217965203363)) ;
#56768=CARTESIAN_POINT('Ctrl Pts',(31.1806337273785,503.730258808275,-35.9681884647833)) ;
#56769=CARTESIAN_POINT('Ctrl Pts',(31.2170981387204,503.734580331867,-36.0166217211997)) ;
#56770=CARTESIAN_POINT('Ctrl Pts',(31.2535253724787,503.738897449415,-36.0650055971003)) ;
#56771=CARTESIAN_POINT('Ctrl Pts',(31.287355798737,503.743203532846,-36.1154264921043)) ;
#56772=CARTESIAN_POINT('Ctrl Pts',(31.3183839884289,503.74745340768,-36.1675649384462)) ;
#56773=CARTESIAN_POINT('Ctrl Pts',(31.3493923171067,503.751700562187,-36.2196700111873)) ;
#56774=CARTESIAN_POINT('Ctrl Pts',(31.3776020907355,503.755891461803,-36.2734903980026)) ;
#56775=CARTESIAN_POINT('Ctrl Pts',(31.4028396878627,503.760004805882,-36.3286913402369)) ;
#56776=CARTESIAN_POINT('Ctrl Pts',(31.4280707067097,503.764117077802,-36.3838778941257)) ;
#56777=CARTESIAN_POINT('Ctrl Pts',(31.4503310408738,503.76815184398,-36.4404442728615)) ;
#56778=CARTESIAN_POINT('Ctrl Pts',(31.4694783634939,503.772112390693,-36.4980404193198)) ;
#56779=CARTESIAN_POINT('Ctrl Pts',(31.4886418197309,503.77607627458,-36.55568509654)) ;
#56780=CARTESIAN_POINT('Ctrl Pts',(31.5046868209787,503.779965937745,-36.6143612760132)) ;
#56781=CARTESIAN_POINT('Ctrl Pts',(31.5175038014117,503.783808307049,-36.6737025049001)) ;
#56782=CARTESIAN_POINT('Ctrl Pts',(31.5303255958451,503.78765211953,-36.7330660220873)) ;
#56783=CARTESIAN_POINT('Ctrl Pts',(31.5399166051113,503.791448875589,-36.7930950710586)) ;
#56784=CARTESIAN_POINT('Ctrl Pts',(31.5462042483842,503.795246235159,-36.8534073790127)) ;
#56785=CARTESIAN_POINT('Ctrl Pts',(31.5525038375664,503.799050809343,-36.9138342744737)) ;
#56786=CARTESIAN_POINT('Ctrl Pts',(31.5554869660787,503.802856462993,-36.9745454079707)) ;
#56787=CARTESIAN_POINT('Ctrl Pts',(31.5551243998437,503.80672636773,-37.0351416171265)) ;
#56788=CARTESIAN_POINT('Ctrl Pts',(31.5547985760722,503.810204096306,-37.0895970062231)) ;
#56789=CARTESIAN_POINT('Ctrl Pts',(31.5517708491299,503.813734302681,-37.1439599822949)) ;
#56790=CARTESIAN_POINT('Ctrl Pts',(31.5460566864391,503.817367336672,-37.1979305182359)) ;
#56791=CARTESIAN_POINT('Ctrl Pts',(31.5455422591127,503.817694406807,-37.202789308581)) ;
#56792=CARTESIAN_POINT('Ctrl Pts',(31.5450060776737,503.818022310341,-37.2076449476738)) ;
#56793=CARTESIAN_POINT('Ctrl Pts',(31.5444481642713,503.81835108401,-37.2124972343404)) ;
#56794=CARTESIAN_POINT('Ctrl Pts',(31.5444444975928,503.818353244753,-37.2125291241909)) ;
#56795=CARTESIAN_POINT('Ctrl Pts',(31.5444408299757,503.818355405533,-37.2125610138967)) ;
#56796=CARTESIAN_POINT('Ctrl Pts',(31.54443716142,503.818357566351,-37.2125929034576)) ;
#56797=CARTESIAN_POINT('Ctrl Pts',(31.5380899299618,503.822096152456,-37.2677673207176)) ;
#56798=CARTESIAN_POINT('Ctrl Pts',(31.5289015841708,503.825957158538,-37.3227066992381)) ;
#56799=CARTESIAN_POINT('Ctrl Pts',(31.5169344347899,503.829877527874,-37.3771083831853)) ;
#56800=CARTESIAN_POINT('Ctrl Pts',(31.515821033412,503.830242271764,-37.3821698149383)) ;
#56801=CARTESIAN_POINT('Ctrl Pts',(31.5146836050773,503.830607529508,-37.3872265662973)) ;
#56802=CARTESIAN_POINT('Ctrl Pts',(31.5135222167086,503.830973250324,-37.3922783779415)) ;
#56803=CARTESIAN_POINT('Ctrl Pts',(31.49973941815,503.835313449062,-37.45223084873)) ;
#56804=CARTESIAN_POINT('Ctrl Pts',(31.4825781631431,503.839718206081,-37.5114921005573)) ;
#56805=CARTESIAN_POINT('Ctrl Pts',(31.4621662833962,503.844116716503,-37.5696766912456)) ;
#56806=CARTESIAN_POINT('Ctrl Pts',(31.4420144640731,503.848459187085,-37.6271199729757)) ;
#56807=CARTESIAN_POINT('Ctrl Pts',(31.4186946915218,503.852795277295,-37.6835140848051)) ;
#56808=CARTESIAN_POINT('Ctrl Pts',(31.3923633244276,503.857077398012,-37.7385084890886)) ;
#56809=CARTESIAN_POINT('Ctrl Pts',(31.3660478185768,503.861356939305,-37.7934697663558)) ;
#56810=CARTESIAN_POINT('Ctrl Pts',(31.3367244447431,503.865582441056,-37.8470331064885)) ;
#56811=CARTESIAN_POINT('Ctrl Pts',(31.3045795269098,503.869730209488,-37.898866740617)) ;
#56812=CARTESIAN_POINT('Ctrl Pts',(31.2724421101615,503.873877010031,-37.9506882792568)) ;
#56813=CARTESIAN_POINT('Ctrl Pts',(31.2374844484629,503.877946111568,-38.0007808877875)) ;
#56814=CARTESIAN_POINT('Ctrl Pts',(31.1999224196693,503.881938636219,-38.048830770933)) ;
#56815=CARTESIAN_POINT('Ctrl Pts',(31.1614664592841,503.886026178206,-38.0980241841244)) ;
#56816=CARTESIAN_POINT('Ctrl Pts',(31.1202804556097,503.890033481837,-38.1450762515352)) ;
#56817=CARTESIAN_POINT('Ctrl Pts',(31.0766293059828,503.893987742501,-38.18967092766)) ;
#56818=CARTESIAN_POINT('Ctrl Pts',(31.0339382825784,503.897855027463,-38.2332847242824)) ;
#56819=CARTESIAN_POINT('Ctrl Pts',(30.9888893079486,503.901671931168,-38.2745478434933)) ;
#56820=CARTESIAN_POINT('Ctrl Pts',(30.9417634312189,503.905485337521,-38.3131871643293)) ;
#56821=CARTESIAN_POINT('Ctrl Pts',(30.8930477545831,503.909427389822,-38.3531299895858)) ;
#56822=CARTESIAN_POINT('Ctrl Pts',(30.8421122291399,503.913366135261,-38.3902682995096)) ;
#56823=CARTESIAN_POINT('Ctrl Pts',(30.7893076246311,503.917370974311,-38.4243317308909)) ;
#56824=CARTESIAN_POINT('Ctrl Pts',(30.7433662941329,503.920855284745,-38.4539677706559)) ;
#56825=CARTESIAN_POINT('Ctrl Pts',(30.6960094976692,503.92439027392,-38.4812768971128)) ;
#56826=CARTESIAN_POINT('Ctrl Pts',(30.6474988141172,503.928026555932,-38.506105537957)) ;
#56827=CARTESIAN_POINT('Ctrl Pts',(30.6402786321784,503.928567769038,-38.5098009570083)) ;
#56828=CARTESIAN_POINT('Ctrl Pts',(30.6330328503057,503.929111226026,-38.5134415132153)) ;
#56829=CARTESIAN_POINT('Ctrl Pts',(30.6257622879721,503.929657093778,-38.5170267894782)) ;
#56830=CARTESIAN_POINT('Ctrl Pts',(30.625735166798,503.929659130013,-38.5170401635333)) ;
#56831=CARTESIAN_POINT('Ctrl Pts',(30.6257080452791,503.929661166282,-38.5170535368193)) ;
#56832=CARTESIAN_POINT('Ctrl Pts',(30.6256809234154,503.929663202584,-38.5170669093361)) ;
#56833=CARTESIAN_POINT('Ctrl Pts',(30.5759590614946,503.933396306572,-38.5415824235088)) ;
#56834=CARTESIAN_POINT('Ctrl Pts',(30.5248965668603,503.937251977912,-38.563593125864)) ;
#56835=CARTESIAN_POINT('Ctrl Pts',(30.4727804230394,503.941166994424,-38.5829869725566)) ;
#56836=CARTESIAN_POINT('Ctrl Pts',(30.467948435261,503.941529978148,-38.5847850877533)) ;
#56837=CARTESIAN_POINT('Ctrl Pts',(30.4631074261961,503.941893472015,-38.586560716022)) ;
#56838=CARTESIAN_POINT('Ctrl Pts',(30.458257646515,503.942257425637,-38.5883137735758)) ;
#56839=CARTESIAN_POINT('Ctrl Pts',(30.400390604308,503.946600080566,-38.6092310651075)) ;
#56840=CARTESIAN_POINT('Ctrl Pts',(30.3412689458996,503.951007524468,-38.6269340433287)) ;
#56841=CARTESIAN_POINT('Ctrl Pts',(30.2812868347915,503.955408377488,-38.6413200789142)) ;
#56842=CARTESIAN_POINT('Ctrl Pts',(30.2222048256791,503.959743190542,-38.6554902351465)) ;
#56843=CARTESIAN_POINT('Ctrl Pts',(30.162288003225,503.96407132633,-38.6664426977938)) ;
#56844=CARTESIAN_POINT('Ctrl Pts',(30.1019142031018,503.968345126172,-38.674118429795)) ;
#56845=CARTESIAN_POINT('Ctrl Pts',(30.0415778315493,503.972616276483,-38.6817894032474)) ;
#56846=CARTESIAN_POINT('Ctrl Pts',(29.9807850354928,503.976833024217,-38.6861878342942)) ;
#56847=CARTESIAN_POINT('Ctrl Pts',(29.9199142353892,503.980971573472,-38.6872900336216)) ;
#56848=CARTESIAN_POINT('Ctrl Pts',(29.8590584670246,503.985109100733,-38.6883919607665)) ;
#56849=CARTESIAN_POINT('Ctrl Pts',(29.7981247542624,503.989168466053,-38.6861992518199)) ;
#56850=CARTESIAN_POINT('Ctrl Pts',(29.7374924867608,503.993150647898,-38.6807228087513)) ;
#56851=CARTESIAN_POINT('Ctrl Pts',(29.675167154414,503.99724402618,-38.6750934442497)) ;
#56852=CARTESIAN_POINT('Ctrl Pts',(29.6131604094991,504.001255859216,-38.6659940414399)) ;
#56853=CARTESIAN_POINT('Ctrl Pts',(29.5518849590064,504.005213532141,-38.6534761480589)) ;
#56854=CARTESIAN_POINT('Ctrl Pts',(29.492198149365,504.009068597565,-38.6412827963442)) ;
#56855=CARTESIAN_POINT('Ctrl Pts',(29.4332053466138,504.012872642956,-38.6258457871656)) ;
#56856=CARTESIAN_POINT('Ctrl Pts',(29.375287021516,504.016672451451,-38.6072529623585)) ;
#56857=CARTESIAN_POINT('Ctrl Pts',(29.3150563408614,504.020623965097,-38.5879178297986)) ;
#56858=CARTESIAN_POINT('Ctrl Pts',(29.2559880036878,504.02457131541,-38.5651690412425)) ;
#56859=CARTESIAN_POINT('Ctrl Pts',(29.1985052067541,504.028585110261,-38.5391572294889)) ;
#56860=CARTESIAN_POINT('Ctrl Pts',(29.1487782751464,504.032057343915,-38.5166550609609)) ;
#56861=CARTESIAN_POINT('Ctrl Pts',(29.1002369640037,504.035579960012,-38.4917107520701)) ;
#56862=CARTESIAN_POINT('Ctrl Pts',(29.053151280261,504.039203629908,-38.4644609317492)) ;
#56863=CARTESIAN_POINT('Ctrl Pts',(29.04583309661,504.039766830432,-38.4602256913595)) ;
#56864=CARTESIAN_POINT('Ctrl Pts',(29.0385499740892,504.040332472034,-38.4559347740699)) ;
#56865=CARTESIAN_POINT('Ctrl Pts',(29.0313028138539,504.040900744955,-38.4515887068868)) ;
#56866=CARTESIAN_POINT('Ctrl Pts',(29.0312773349585,504.040902742836,-38.4515734273859)) ;
#56867=CARTESIAN_POINT('Ctrl Pts',(29.0312518565074,504.04090474075,-38.4515581472033)) ;
#56868=CARTESIAN_POINT('Ctrl Pts',(29.0312263785009,504.040906738696,-38.4515428663391)) ;
#56869=CARTESIAN_POINT('Ctrl Pts',(28.9836891917994,504.044634532379,-38.4230316367382)) ;
#56870=CARTESIAN_POINT('Ctrl Pts',(28.937532068309,504.04848544368,-38.3920373753948)) ;
#56871=CARTESIAN_POINT('Ctrl Pts',(28.8930043403531,504.052396327771,-38.3587407430544)) ;
#56872=CARTESIAN_POINT('Ctrl Pts',(28.8888399002697,504.052762091829,-38.3556266872351)) ;
#56873=CARTESIAN_POINT('Ctrl Pts',(28.8846897251509,504.053128380461,-38.3524925282806)) ;
#56874=CARTESIAN_POINT('Ctrl Pts',(28.8805540263586,504.05349514201,-38.3493384360104)) ;
#56875=CARTESIAN_POINT('Ctrl Pts',(28.8316288596092,504.057833917845,-38.3120256388237)) ;
#56876=CARTESIAN_POINT('Ctrl Pts',(28.7847271856301,504.062238210287,-38.2719177104918)) ;
#56877=CARTESIAN_POINT('Ctrl Pts',(28.7401483956201,504.066636623972,-38.2292905661611)) ;
#56878=CARTESIAN_POINT('Ctrl Pts',(28.6962098818012,504.070971864126,-38.1872756669273)) ;
#56879=CARTESIAN_POINT('Ctrl Pts',(28.6545276339809,504.075301106021,-38.1428136461075)) ;
#56880=CARTESIAN_POINT('Ctrl Pts',(28.6153560262653,504.079576524087,-38.0961907454377)) ;
#56881=CARTESIAN_POINT('Ctrl Pts',(28.5762084777309,504.083849316194,-38.0495964805294)) ;
#56882=CARTESIAN_POINT('Ctrl Pts',(28.5395683694364,504.088068215286,-38.0008440466416)) ;
#56883=CARTESIAN_POINT('Ctrl Pts',(28.505660616964,504.092209273672,-37.9502392578844)) ;
#56884=CARTESIAN_POINT('Ctrl Pts',(28.4717610838035,504.096349328258,-37.8996467358365)) ;
#56885=CARTESIAN_POINT('Ctrl Pts',(28.4405926183445,504.100411577183,-37.847202756189)) ;
#56886=CARTESIAN_POINT('Ctrl Pts',(28.4123515590043,504.104396876594,-37.7932326286487)) ;
#56887=CARTESIAN_POINT('Ctrl Pts',(28.3833551024332,504.108488775552,-37.7378188978635)) ;
#56888=CARTESIAN_POINT('Ctrl Pts',(28.3574450825579,504.112499566624,-37.6807961546299)) ;
#56889=CARTESIAN_POINT('Ctrl Pts',(28.3348011177148,504.116456433674,-37.6225384285027)) ;
#56890=CARTESIAN_POINT('Ctrl Pts',(28.3127189071721,504.120315138274,-37.5657259673018)) ;
#56891=CARTESIAN_POINT('Ctrl Pts',(28.2937429000415,504.124122924579,-37.5077390823149)) ;
#56892=CARTESIAN_POINT('Ctrl Pts',(28.2780053966865,504.127926506306,-37.4489455837021)) ;
#56893=CARTESIAN_POINT('Ctrl Pts',(28.2616673685219,504.131875228284,-37.387908593618)) ;
#56894=CARTESIAN_POINT('Ctrl Pts',(28.2488205811515,504.135819839118,-37.3260021173562)) ;
#56895=CARTESIAN_POINT('Ctrl Pts',(28.2395672492876,504.139830550969,-37.2636616964272)) ;
#56896=CARTESIAN_POINT('Ctrl Pts',(28.2315460959638,504.143307194318,-37.2096225587529)) ;
#56897=CARTESIAN_POINT('Ctrl Pts',(28.2262248196662,504.146834162073,-37.1552564547135)) ;
#56898=CARTESIAN_POINT('Ctrl Pts',(28.2236349801933,504.150462192433,-37.1008648994454)) ;
#56899=CARTESIAN_POINT('Ctrl Pts',(28.2232385397136,504.151017554304,-37.0925388952725)) ;
#56900=CARTESIAN_POINT('Ctrl Pts',(28.2229060366054,504.15157528428,-37.0842122200828)) ;
#56901=CARTESIAN_POINT('Ctrl Pts',(28.2226375148372,504.15213556435,-37.0758858722792)) ;
#56902=CARTESIAN_POINT('Ctrl Pts',(28.222636566139,504.152137543842,-37.075856454956)) ;
#56903=CARTESIAN_POINT('Ctrl Pts',(28.2226356182393,504.152139523366,-37.0758270376369)) ;
#56904=CARTESIAN_POINT('Ctrl Pts',(28.2226346711383,504.152141502922,-37.075797620322)) ;
#56905=CARTESIAN_POINT('Ctrl Pts',(28.2208500943408,504.155871484354,-37.0203679936469)) ;
#56906=CARTESIAN_POINT('Ctrl Pts',(28.2219028062132,504.159724323723,-36.9647537042311)) ;
#56907=CARTESIAN_POINT('Ctrl Pts',(28.2257758975944,504.163636871801,-36.9092625220861)) ;
#56908=CARTESIAN_POINT('Ctrl Pts',(28.2261369073593,504.164001559314,-36.9040902045117)) ;
#56909=CARTESIAN_POINT('Ctrl Pts',(28.2265223981255,504.164366765579,-36.8989189862949)) ;
#56910=CARTESIAN_POINT('Ctrl Pts',(28.2269323418467,504.164732439457,-36.8937491346411)) ;
#56911=CARTESIAN_POINT('Ctrl Pts',(28.2317959566801,504.169070832282,-36.8324134783378)) ;
#56912=CARTESIAN_POINT('Ctrl Pts',(28.2401047895027,504.173474379365,-36.7712651476695)) ;
#56913=CARTESIAN_POINT('Ctrl Pts',(28.2517890378207,504.177871818711,-36.7107050943761)) ;
#56914=CARTESIAN_POINT('Ctrl Pts',(28.2633079385338,504.182207028459,-36.6510020461283)) ;
#56915=CARTESIAN_POINT('Ctrl Pts',(28.2781069899057,504.186536014908,-36.591870566549)) ;
#56916=CARTESIAN_POINT('Ctrl Pts',(28.296083296526,504.190811046205,-36.5336796190072)) ;
#56917=CARTESIAN_POINT('Ctrl Pts',(28.3140486279441,504.195083467438,-36.4755241991982)) ;
#56918=CARTESIAN_POINT('Ctrl Pts',(28.3351872250997,504.199301864474,-36.4183080962711)) ;
#56919=CARTESIAN_POINT('Ctrl Pts',(28.3593637853539,504.203442387736,-36.362386118099)) ;
#56920=CARTESIAN_POINT('Ctrl Pts',(28.3835345651836,504.207581921032,-36.3064775104298)) ;
#56921=CARTESIAN_POINT('Ctrl Pts',(28.410741876212,504.211643615454,-36.2518624389859)) ;
#56922=CARTESIAN_POINT('Ctrl Pts',(28.440818544815,504.215628424807,-36.1988822544473)) ;
#56923=CARTESIAN_POINT('Ctrl Pts',(28.4716879497097,504.219718262513,-36.1445056614308)) ;
#56924=CARTESIAN_POINT('Ctrl Pts',(28.505580247537,504.223727124136,-36.0918514796608)) ;
#56925=CARTESIAN_POINT('Ctrl Pts',(28.5422784938317,504.22768225627,-36.0412730036637)) ;
#56926=CARTESIAN_POINT('Ctrl Pts',(28.5780801642525,504.23154076046,-35.9919302118176)) ;
#56927=CARTESIAN_POINT('Ctrl Pts',(28.6165524211438,504.235348490898,-35.9445631243113)) ;
#56928=CARTESIAN_POINT('Ctrl Pts',(28.6574576603838,504.239152230433,-35.8994822958023)) ;
#56929=CARTESIAN_POINT('Ctrl Pts',(28.6998994752998,504.243098854689,-35.8527080386316)) ;
#56930=CARTESIAN_POINT('Ctrl Pts',(28.744961073878,504.247041605063,-35.8083956799027)) ;
#56931=CARTESIAN_POINT('Ctrl Pts',(28.7923321274247,504.251050616792,-35.7668666333778)) ;
#56932=CARTESIAN_POINT('Ctrl Pts',(28.8334073936705,504.254526816113,-35.7308569499269)) ;
#56933=CARTESIAN_POINT('Ctrl Pts',(28.8762196343179,504.25805348928,-35.6969391952642)) ;
#56934=CARTESIAN_POINT('Ctrl Pts',(28.9205326144722,504.261681330358,-35.6653031412673)) ;
#56935=CARTESIAN_POINT('Ctrl Pts',(28.9273005643906,504.262235412856,-35.6604713464225)) ;
#56936=CARTESIAN_POINT('Ctrl Pts',(28.9341035484484,504.262791855262,-35.6556926806711)) ;
#56937=CARTESIAN_POINT('Ctrl Pts',(28.9409407570499,504.263350838184,-35.6509677176084)) ;
#56938=CARTESIAN_POINT('Ctrl Pts',(28.9409650997126,504.263352828343,-35.6509508952195)) ;
#56939=CARTESIAN_POINT('Ctrl Pts',(28.9409894428091,504.263354818535,-35.6509340735113)) ;
#56940=CARTESIAN_POINT('Ctrl Pts',(28.9410137863394,504.263356808758,-35.6509172524838)) ;
#56941=CARTESIAN_POINT('Ctrl Pts',(28.9869423202729,504.267111730322,-35.6191812995285)) ;
#56942=CARTESIAN_POINT('Ctrl Pts',(29.0345809314372,504.270990944817,-35.5897636294556)) ;
#56943=CARTESIAN_POINT('Ctrl Pts',(29.0836601273048,504.274930258251,-35.562816359925)) ;
#56944=CARTESIAN_POINT('Ctrl Pts',(29.0885670056895,504.275324106023,-35.5601222046511)) ;
#56945=CARTESIAN_POINT('Ctrl Pts',(29.093488240868,504.275718554529,-35.5574527410732)) ;
#56946=CARTESIAN_POINT('Ctrl Pts',(29.098423535015,504.276113539616,-35.5548081192529)) ;
#56947=CARTESIAN_POINT('Ctrl Pts',(29.1526313881012,504.280451942346,-35.5257603529336)) ;
#56948=CARTESIAN_POINT('Ctrl Pts',(29.2085413791482,504.284854446758,-35.499709252215)) ;
#56949=CARTESIAN_POINT('Ctrl Pts',(29.2657851188358,504.289250406587,-35.4768109646585)) ;
#56950=CARTESIAN_POINT('Ctrl Pts',(29.3229409176651,504.293639613111,-35.4539478546615)) ;
#56951=CARTESIAN_POINT('Ctrl Pts',(29.3814263602263,504.298021958897,-35.4342275015703)) ;
#56952=CARTESIAN_POINT('Ctrl Pts',(29.440868284465,504.302348604279,-35.4177679028226)) ;
#56953=CARTESIAN_POINT('Ctrl Pts',(29.5002567651601,504.306671359625,-35.4013231027089)) ;
#56954=CARTESIAN_POINT('Ctrl Pts',(29.5606000532667,504.310938374649,-35.3881330589776)) ;
#56955=CARTESIAN_POINT('Ctrl Pts',(29.6215191659238,504.315125889259,-35.3782818457609)) ;
#56956=CARTESIAN_POINT('Ctrl Pts',(29.6824067496338,504.319311236603,-35.3684357310817)) ;
#56957=CARTESIAN_POINT('Ctrl Pts',(29.7438695966127,504.323417160521,-35.3619250360645)) ;
#56958=CARTESIAN_POINT('Ctrl Pts',(29.8055218641932,504.327445925357,-35.3588007649088)) ;
#56959=CARTESIAN_POINT('Ctrl Pts',(29.8334504027829,504.329270959839,-35.3573854669651)) ;
#56960=CARTESIAN_POINT('Ctrl Pts',(29.8614177078716,504.331080514259,-35.3566646446211)) ;
#56961=CARTESIAN_POINT('Ctrl Pts',(29.8893873868701,504.332876521313,-35.3566407257823)) ;
#56962=CARTESIAN_POINT('Ctrl Pts',(29.8893696774914,504.333153023327,-35.3561603845536)) ;
#56963=CARTESIAN_POINT('Ctrl Pts',(29.9621840579132,504.33776953377,-35.3561971873801)) ;
#56964=CARTESIAN_POINT('Ctrl Pts',(30.0349214669345,504.342254646832,-35.3610074838177)) ;
#56965=CARTESIAN_POINT('Ctrl Pts',(30.2112166298579,504.353130330676,-35.3843401317637)) ;
#56966=CARTESIAN_POINT('Ctrl Pts',(30.3137700963673,504.359457033253,-35.4079275358013)) ;
#56967=CARTESIAN_POINT('Ctrl Pts',(30.4303996283287,504.367300860559,-35.4466440056302)) ;
#56968=CARTESIAN_POINT('Ctrl Pts',(30.4472953070465,504.368454090922,-35.4525567232203)) ;
#56969=CARTESIAN_POINT('Ctrl Pts',(30.4640904795472,504.369620557053,-35.4587397545496)) ;
#56970=CARTESIAN_POINT('Origin',(179.888527625402,504.710565160536,-37.0221601717597)) ;
#56971=CARTESIAN_POINT('',(180.464132351894,505.578765842461,-35.4584785386352)) ;
#56972=CARTESIAN_POINT('',(180.464073435736,505.710565160536,-35.4587334800957)) ;
#56973=CARTESIAN_POINT('',(180.464073435736,504.710565160536,-35.4587334800957)) ;
#56974=CARTESIAN_POINT('',(181.553672909139,505.710557590725,-36.9459937350495)) ;
#56975=CARTESIAN_POINT('Origin',(179.888527625402,505.710565160536,-37.0221601717597)) ;
#56976=CARTESIAN_POINT('Ctrl Pts',(181.553672925284,505.710557590587,-36.9459937343111)) ;
#56977=CARTESIAN_POINT('Ctrl Pts',(181.551232283181,505.706956684071,-36.8933096088381)) ;
#56978=CARTESIAN_POINT('Ctrl Pts',(181.546229220061,505.703258987467,-36.8406540870477)) ;
#56979=CARTESIAN_POINT('Ctrl Pts',(181.538696531225,505.699518432147,-36.7882942048495)) ;
#56980=CARTESIAN_POINT('Ctrl Pts',(181.53008552317,505.695242408978,-36.7284389025576)) ;
#56981=CARTESIAN_POINT('Ctrl Pts',(181.518168521576,505.690910939552,-36.6689686983251)) ;
#56982=CARTESIAN_POINT('Ctrl Pts',(181.503032801552,505.686590161194,-36.610260669948)) ;
#56983=CARTESIAN_POINT('Ctrl Pts',(181.487912510483,505.682273787325,-36.5516124869901)) ;
#56984=CARTESIAN_POINT('Ctrl Pts',(181.469580338947,505.677968380708,-36.4937247889096)) ;
#56985=CARTESIAN_POINT('Ctrl Pts',(181.448158009494,505.673719114553,-36.4369573931851)) ;
#56986=CARTESIAN_POINT('Ctrl Pts',(181.426749389391,505.669472567741,-36.380226326101)) ;
#56987=CARTESIAN_POINT('Ctrl Pts',(181.402254655126,505.665282207666,-36.3246140776572)) ;
#56988=CARTESIAN_POINT('Ctrl Pts',(181.374827311688,505.661169324461,-36.2704651280015)) ;
#56989=CARTESIAN_POINT('Ctrl Pts',(181.347407114689,505.657057512904,-36.216330287334)) ;
#56990=CARTESIAN_POINT('Ctrl Pts',(181.31705580914,505.653023128339,-36.1636580345744)) ;
#56991=CARTESIAN_POINT('Ctrl Pts',(181.283958371087,505.649062866651,-36.1127779211213)) ;
#56992=CARTESIAN_POINT('Ctrl Pts',(181.250833052662,505.645099268947,-36.0618549476582)) ;
#56993=CARTESIAN_POINT('Ctrl Pts',(181.214956852527,505.641209795007,-36.0127272875708)) ;
#56994=CARTESIAN_POINT('Ctrl Pts',(181.176547993421,505.63736749505,-35.9657091024632)) ;
#56995=CARTESIAN_POINT('Ctrl Pts',(181.138124707358,505.633523751867,-35.9186732566059)) ;
#56996=CARTESIAN_POINT('Ctrl Pts',(181.097166661149,505.629726944885,-35.8737487466492)) ;
#56997=CARTESIAN_POINT('Ctrl Pts',(181.053927512491,505.625929389367,-35.8312306832966)) ;
#56998=CARTESIAN_POINT('Ctrl Pts',(181.010606247503,505.622124621837,-35.7886318730427)) ;
#56999=CARTESIAN_POINT('Ctrl Pts',(180.964994953339,505.618318628867,-35.7484491347412)) ;
#57000=CARTESIAN_POINT('Ctrl Pts',(180.917387530296,505.614448217065,-35.7109542182485)) ;
#57001=CARTESIAN_POINT('Ctrl Pts',(180.874609000482,505.610970387011,-35.6772624680851)) ;
#57002=CARTESIAN_POINT('Ctrl Pts',(180.830218468774,505.607439954069,-35.6457406515821)) ;
#57003=CARTESIAN_POINT('Ctrl Pts',(180.784460105248,505.603806575094,-35.6165636899711)) ;
#57004=CARTESIAN_POINT('Ctrl Pts',(180.780374495576,505.603482162962,-35.6139585776513)) ;
#57005=CARTESIAN_POINT('Ctrl Pts',(180.776277970414,505.603156930133,-35.6113721261506)) ;
#57006=CARTESIAN_POINT('Ctrl Pts',(180.772170696643,505.602830840774,-35.6088044409151)) ;
#57007=CARTESIAN_POINT('Ctrl Pts',(180.772142495247,505.602828601777,-35.6087868106542)) ;
#57008=CARTESIAN_POINT('Ctrl Pts',(180.772114293344,505.602826362739,-35.6087691812779)) ;
#57009=CARTESIAN_POINT('Ctrl Pts',(180.772086090935,505.602824123661,-35.6087515527864)) ;
#57010=CARTESIAN_POINT('Ctrl Pts',(180.724314775962,505.599031408457,-35.5788911175874)) ;
#57011=CARTESIAN_POINT('Ctrl Pts',(180.674922975228,505.595113445829,-35.5514743831438)) ;
#57012=CARTESIAN_POINT('Ctrl Pts',(180.62419067516,505.591135506992,-35.5266397360626)) ;
#57013=CARTESIAN_POINT('Ctrl Pts',(180.618793793035,505.590712335423,-35.5239978360755)) ;
#57014=CARTESIAN_POINT('Ctrl Pts',(180.613381789521,505.590288485126,-35.521385153931)) ;
#57015=CARTESIAN_POINT('Ctrl Pts',(180.607955036194,505.589864034679,-35.5188018533853)) ;
#57016=CARTESIAN_POINT('Ctrl Pts',(180.561046359589,505.586195099023,-35.4964718887473)) ;
#57017=CARTESIAN_POINT('Ctrl Pts',(180.51303134374,505.582481418132,-35.4763363661572)) ;
#57018=CARTESIAN_POINT('Ctrl Pts',(180.464132351894,505.578765842461,-35.4584785386352)) ;
#57019=CARTESIAN_POINT('Origin',(179.888527625402,504.710565160536,-37.0221601717597)) ;
#57020=CARTESIAN_POINT('',(180.464073442659,504.877005588434,-35.4587334826444)) ;
#57021=CARTESIAN_POINT('',(180.464062970719,505.071445141582,-35.4587536919275)) ;
#57022=CARTESIAN_POINT('',(180.464073435736,504.710565160536,-35.4587334800957)) ;
#57023=CARTESIAN_POINT('',(179.569297170772,505.710565160536,-35.3870308445086)) ;
#57024=CARTESIAN_POINT('Ctrl Pts',(180.464062970719,505.071445141582,-35.4587536919275)) ;
#57025=CARTESIAN_POINT('Ctrl Pts',(180.521080010244,505.075770871481,-35.4799041023179)) ;
#57026=CARTESIAN_POINT('Ctrl Pts',(180.576992960962,505.080073944616,-35.5041868991519)) ;
#57027=CARTESIAN_POINT('Ctrl Pts',(180.631455338622,505.084313431263,-35.5314424279691)) ;
#57028=CARTESIAN_POINT('Ctrl Pts',(180.685890268488,505.088550781305,-35.5586842206219)) ;
#57029=CARTESIAN_POINT('Ctrl Pts',(180.738876133664,505.092724517274,-35.588895689098)) ;
#57030=CARTESIAN_POINT('Ctrl Pts',(180.790084341574,505.096818065672,-35.6218872465369)) ;
#57031=CARTESIAN_POINT('Ctrl Pts',(180.841285782239,505.1009110731,-35.6548744440893)) ;
#57032=CARTESIAN_POINT('Ctrl Pts',(180.890709970514,505.104923945953,-35.690641038872)) ;
#57033=CARTESIAN_POINT('Ctrl Pts',(180.938045959887,505.108864839164,-35.7289674359767)) ;
#57034=CARTESIAN_POINT('Ctrl Pts',(180.985427575524,505.112809530928,-35.7673307751703)) ;
#57035=CARTESIAN_POINT('Ctrl Pts',(181.030716786754,505.116682254085,-35.8082589823685)) ;
#57036=CARTESIAN_POINT('Ctrl Pts',(181.073621114329,505.120514619554,-35.8515003800246)) ;
#57037=CARTESIAN_POINT('Ctrl Pts',(181.116545852412,505.124348808161,-35.8947623485404)) ;
#57038=CARTESIAN_POINT('Ctrl Pts',(181.157083118322,505.128142910395,-35.9403399040468)) ;
#57039=CARTESIAN_POINT('Ctrl Pts',(181.19496306555,505.131948623222,-35.9879471018041)) ;
#57040=CARTESIAN_POINT('Ctrl Pts',(181.232914486131,505.135761516816,-36.035644126667)) ;
#57041=CARTESIAN_POINT('Ctrl Pts',(181.268198006477,505.139586590695,-36.0853786797498)) ;
#57042=CARTESIAN_POINT('Ctrl Pts',(181.300571785506,505.143489740683,-36.1368259459113)) ;
#57043=CARTESIAN_POINT('Ctrl Pts',(181.326653284119,505.146634260849,-36.1782737422847)) ;
#57044=CARTESIAN_POINT('Ctrl Pts',(181.350846570535,505.149829917129,-36.2208324674788)) ;
#57045=CARTESIAN_POINT('Ctrl Pts',(181.373043576586,505.15311340371,-36.2643136111372)) ;
#57046=CARTESIAN_POINT('Ctrl Pts',(181.373057187027,505.153115417031,-36.2643402722792)) ;
#57047=CARTESIAN_POINT('Ctrl Pts',(181.373070796718,505.153117430385,-36.2643669337685)) ;
#57048=CARTESIAN_POINT('Ctrl Pts',(181.37308440566,505.153119443772,-36.264393595605)) ;
#57049=CARTESIAN_POINT('Ctrl Pts',(181.398271192042,505.156845725506,-36.3137380628099)) ;
#57050=CARTESIAN_POINT('Ctrl Pts',(181.420974790708,505.160694970282,-36.3644557912384)) ;
#57051=CARTESIAN_POINT('Ctrl Pts',(181.441079501555,505.164604050267,-36.4162617899537)) ;
#57052=CARTESIAN_POINT('Ctrl Pts',(181.442958774348,505.164969448592,-36.4211043168937)) ;
#57053=CARTESIAN_POINT('Ctrl Pts',(181.444815347382,505.165335369723,-36.425956315746)) ;
#57054=CARTESIAN_POINT('Ctrl Pts',(181.446649131573,505.165701762102,-36.430817531191)) ;
#57055=CARTESIAN_POINT('Ctrl Pts',(181.468368576099,505.170041334334,-36.4883940441226)) ;
#57056=CARTESIAN_POINT('Ctrl Pts',(181.486890304425,505.174446344264,-36.5472694413303)) ;
#57057=CARTESIAN_POINT('Ctrl Pts',(181.502106448514,505.178845251849,-36.6070507344203)) ;
#57058=CARTESIAN_POINT('Ctrl Pts',(181.51709363293,505.183177968392,-36.6659324891493)) ;
#57059=CARTESIAN_POINT('Ctrl Pts',(181.528874414093,505.187504479843,-36.7256930668193)) ;
#57060=CARTESIAN_POINT('Ctrl Pts',(181.537384817382,505.191776934332,-36.7859553523217)) ;
#57061=CARTESIAN_POINT('Ctrl Pts',(181.545890020311,505.196046778099,-36.8461808139944)) ;
#57062=CARTESIAN_POINT('Ctrl Pts',(181.551128970221,505.200262495487,-36.9069073820963)) ;
#57063=CARTESIAN_POINT('Ctrl Pts',(181.553073060345,505.20440007612,-36.96775695298)) ;
#57064=CARTESIAN_POINT('Ctrl Pts',(181.555016687712,505.208536671873,-37.0285920396698)) ;
#57065=CARTESIAN_POINT('Ctrl Pts',(181.553666993242,505.212595164903,-37.0895500501727)) ;
#57066=CARTESIAN_POINT('Ctrl Pts',(181.549029945194,505.216576317454,-37.1502515153961)) ;
#57067=CARTESIAN_POINT('Ctrl Pts',(181.544263187326,505.22066883279,-37.212650952271)) ;
#57068=CARTESIAN_POINT('Ctrl Pts',(181.536022236578,505.224679627689,-37.2747792232977)) ;
#57069=CARTESIAN_POINT('Ctrl Pts',(181.524353245269,505.228635873202,-37.3362230233926)) ;
#57070=CARTESIAN_POINT('Ctrl Pts',(181.512987076644,505.232489449954,-37.3960722917928)) ;
#57071=CARTESIAN_POINT('Ctrl Pts',(181.498368355485,505.236291638583,-37.455272016429)) ;
#57072=CARTESIAN_POINT('Ctrl Pts',(181.480579885503,505.240089060205,-37.5134407275502)) ;
#57073=CARTESIAN_POINT('Ctrl Pts',(181.462080522641,505.244038240803,-37.573934074945)) ;
#57074=CARTESIAN_POINT('Ctrl Pts',(181.440152174811,505.247982681211,-37.633312011773)) ;
#57075=CARTESIAN_POINT('Ctrl Pts',(181.4149397813,505.251992891751,-37.6911495202233)) ;
#57076=CARTESIAN_POINT('Ctrl Pts',(181.393113818423,505.25546446641,-37.7412185194943)) ;
#57077=CARTESIAN_POINT('Ctrl Pts',(181.368826529878,505.258985986666,-37.7901340331353)) ;
#57078=CARTESIAN_POINT('Ctrl Pts',(181.342211123621,505.262608248821,-37.8376238003478)) ;
#57079=CARTESIAN_POINT('Ctrl Pts',(181.338096637096,505.263168215807,-37.8449652628593)) ;
#57080=CARTESIAN_POINT('Ctrl Pts',(181.333926529225,505.263730590343,-37.8522727526905)) ;
#57081=CARTESIAN_POINT('Ctrl Pts',(181.32970130716,505.264295560091,-37.8595453745187)) ;
#57082=CARTESIAN_POINT('Ctrl Pts',(181.329685846643,505.264297627373,-37.8595719857805)) ;
#57083=CARTESIAN_POINT('Ctrl Pts',(181.329670385388,505.264299694689,-37.8595985965754)) ;
#57084=CARTESIAN_POINT('Ctrl Pts',(181.329654923396,505.26430176204,-37.8596252069035)) ;
#57085=CARTESIAN_POINT('Ctrl Pts',(181.301764050089,505.268030921166,-37.907625831437)) ;
#57086=CARTESIAN_POINT('Ctrl Pts',(181.271365056046,505.271882972526,-37.9542753361818)) ;
#57087=CARTESIAN_POINT('Ctrl Pts',(181.238635970714,505.275794811077,-37.9993214409816)) ;
#57088=CARTESIAN_POINT('Ctrl Pts',(181.235578353838,505.276160262889,-38.0035297385506)) ;
#57089=CARTESIAN_POINT('Ctrl Pts',(181.232500435814,505.276526236505,-38.0077240288423)) ;
#57090=CARTESIAN_POINT('Ctrl Pts',(181.229402383651,505.276892680471,-38.0119040984859)) ;
#57091=CARTESIAN_POINT('Ctrl Pts',(181.192776611733,505.281224851914,-38.0613216903563)) ;
#57092=CARTESIAN_POINT('Ctrl Pts',(181.153331366697,505.285622100762,-38.1087542638443)) ;
#57093=CARTESIAN_POINT('Ctrl Pts',(181.111338007007,505.290013476012,-38.1538996748488)) ;
#57094=CARTESIAN_POINT('Ctrl Pts',(181.069877970916,505.294349079967,-38.1984717306076)) ;
#57095=CARTESIAN_POINT('Ctrl Pts',(181.02593437793,505.298678666118,-38.2408147102694)) ;
#57096=CARTESIAN_POINT('Ctrl Pts',(180.979790785691,505.302954501936,-38.2806698616093)) ;
#57097=CARTESIAN_POINT('Ctrl Pts',(180.93367532461,505.307227731016,-38.3205007155007)) ;
#57098=CARTESIAN_POINT('Ctrl Pts',(180.885362603077,505.311447140245,-38.3578468915722)) ;
#57099=CARTESIAN_POINT('Ctrl Pts',(180.835156113497,505.315588901942,-38.3924788439465)) ;
#57100=CARTESIAN_POINT('Ctrl Pts',(180.78496170375,505.319729667119,-38.427102463768)) ;
#57101=CARTESIAN_POINT('Ctrl Pts',(180.732874433412,505.323792820316,-38.4590131305097)) ;
#57102=CARTESIAN_POINT('Ctrl Pts',(180.679217671769,505.327779356826,-38.4880096023417)) ;
#57103=CARTESIAN_POINT('Ctrl Pts',(180.624286752494,505.331860559427,-38.5176946374549)) ;
#57104=CARTESIAN_POINT('Ctrl Pts',(180.567710791877,505.335861490449,-38.5443251205988)) ;
#57105=CARTESIAN_POINT('Ctrl Pts',(180.509858914482,505.339809209461,-38.5677173832672)) ;
#57106=CARTESIAN_POINT('Ctrl Pts',(180.453277628558,505.343670225356,-38.5905958854359)) ;
#57107=CARTESIAN_POINT('Ctrl Pts',(180.395475884077,505.347480694652,-38.6103766403132)) ;
#57108=CARTESIAN_POINT('Ctrl Pts',(180.336820461364,505.351287379752,-38.6269217550556)) ;
#57109=CARTESIAN_POINT('Ctrl Pts',(180.276189286104,505.355222289445,-38.6440241763704)) ;
#57110=CARTESIAN_POINT('Ctrl Pts',(180.21464581881,505.359153585616,-38.6576684834696)) ;
#57111=CARTESIAN_POINT('Ctrl Pts',(180.152619545364,505.363150532887,-38.6677472000519)) ;
#57112=CARTESIAN_POINT('Ctrl Pts',(180.098635944115,505.366629213707,-38.676519054088)) ;
#57113=CARTESIAN_POINT('Ctrl Pts',(180.044285767577,505.370158273136,-38.6825903101323)) ;
#57114=CARTESIAN_POINT('Ctrl Pts',(179.989870386624,505.373788303311,-38.6859247996509)) ;
#57115=CARTESIAN_POINT('Ctrl Pts',(179.981796515883,505.374326908278,-38.6864195538341)) ;
#57116=CARTESIAN_POINT('Ctrl Pts',(179.973721140369,505.374867736123,-38.6868541208458)) ;
#57117=CARTESIAN_POINT('Ctrl Pts',(179.965645170118,505.375410952105,-38.6872284464903)) ;
#57118=CARTESIAN_POINT('Ctrl Pts',(179.965612031944,505.375413181086,-38.6872299824628)) ;
#57119=CARTESIAN_POINT('Ctrl Pts',(179.965578893759,505.375415410108,-38.6872315174211)) ;
#57120=CARTESIAN_POINT('Ctrl Pts',(179.965545755565,505.375417639169,-38.6872330513651)) ;
#57121=CARTESIAN_POINT('Ctrl Pts',(179.910067113818,505.379149445156,-38.6898011192401)) ;
#57122=CARTESIAN_POINT('Ctrl Pts',(179.854363673121,505.383003622821,-38.689527257712)) ;
#57123=CARTESIAN_POINT('Ctrl Pts',(179.798744861262,505.386916699123,-38.6864243279499)) ;
#57124=CARTESIAN_POINT('Ctrl Pts',(179.793688291258,505.387272455451,-38.686142225887)) ;
#57125=CARTESIAN_POINT('Ctrl Pts',(179.788632449574,505.387628698604,-38.6858367610734)) ;
#57126=CARTESIAN_POINT('Ctrl Pts',(179.783577585658,505.387985380887,-38.6855079560975)) ;
#57127=CARTESIAN_POINT('Ctrl Pts',(179.722174709537,505.392318102478,-38.6815138681186)) ;
#57128=CARTESIAN_POINT('Ctrl Pts',(179.660911037464,505.396714958137,-38.6740726173969)) ;
#57129=CARTESIAN_POINT('Ctrl Pts',(179.600188702896,505.401104926319,-38.663248522297)) ;
#57130=CARTESIAN_POINT('Ctrl Pts',(179.540366824506,505.405429795324,-38.6525849385376)) ;
#57131=CARTESIAN_POINT('Ctrl Pts',(179.481070175861,505.409747700509,-38.6386385048869)) ;
#57132=CARTESIAN_POINT('Ctrl Pts',(179.42266863279,505.414011481721,-38.6215068676923)) ;
#57133=CARTESIAN_POINT('Ctrl Pts',(179.364301006689,505.418272786722,-38.6043851797766)) ;
#57134=CARTESIAN_POINT('Ctrl Pts',(179.306827383361,505.422479899325,-38.5840820957034)) ;
#57135=CARTESIAN_POINT('Ctrl Pts',(179.250604020104,505.426609662978,-38.5607278453121)) ;
#57136=CARTESIAN_POINT('Ctrl Pts',(179.194392324855,505.430738569583,-38.5373784416168)) ;
#57137=CARTESIAN_POINT('Ctrl Pts',(179.139430402327,505.434790159582,-38.5109791146164)) ;
#57138=CARTESIAN_POINT('Ctrl Pts',(179.086061553448,505.438766159265,-38.4816921757098)) ;
#57139=CARTESIAN_POINT('Ctrl Pts',(179.031225404504,505.442851473366,-38.4516000343628)) ;
#57140=CARTESIAN_POINT('Ctrl Pts',(178.978071339079,505.44685699701,-38.4184590177896)) ;
#57141=CARTESIAN_POINT('Ctrl Pts',(178.926956443945,505.450810966356,-38.3824818069815)) ;
#57142=CARTESIAN_POINT('Ctrl Pts',(178.87714107789,505.454664411224,-38.3474192695086)) ;
#57143=CARTESIAN_POINT('Ctrl Pts',(178.829262694466,505.458469260829,-38.3096628501496)) ;
#57144=CARTESIAN_POINT('Ctrl Pts',(178.783634834466,505.462273146348,-38.2694459596162)) ;
#57145=CARTESIAN_POINT('Ctrl Pts',(178.736221539503,505.466225879307,-38.2276553673468)) ;
#57146=CARTESIAN_POINT('Ctrl Pts',(178.691238997983,505.470178000043,-38.1832073670448)) ;
#57147=CARTESIAN_POINT('Ctrl Pts',(178.64901397051,505.474200826604,-38.1364095751759)) ;
#57148=CARTESIAN_POINT('Ctrl Pts',(178.612570228503,505.477672863499,-38.0960191537744)) ;
#57149=CARTESIAN_POINT('Ctrl Pts',(178.578179820612,505.481198232857,-38.05387774283)) ;
#57150=CARTESIAN_POINT('Ctrl Pts',(178.546033727488,505.484827547551,-38.0102172444428)) ;
#57151=CARTESIAN_POINT('Ctrl Pts',(178.540955075824,505.485400930607,-38.003319471144)) ;
#57152=CARTESIAN_POINT('Ctrl Pts',(178.535932339391,505.485976908114,-37.9963837548511)) ;
#57153=CARTESIAN_POINT('Ctrl Pts',(178.530966156704,505.486555679654,-37.9894109764195)) ;
#57154=CARTESIAN_POINT('Ctrl Pts',(178.530945746489,505.486558058313,-37.9893823194171)) ;
#57155=CARTESIAN_POINT('Ctrl Pts',(178.530925337229,505.486560437018,-37.9893536617887)) ;
#57156=CARTESIAN_POINT('Ctrl Pts',(178.530904928924,505.486562815771,-37.9893250035343)) ;
#57157=CARTESIAN_POINT('Ctrl Pts',(178.49901047633,505.490280371737,-37.9445373870732)) ;
#57158=CARTESIAN_POINT('Ctrl Pts',(178.469336257246,505.494123495406,-37.8980478367498)) ;
#57159=CARTESIAN_POINT('Ctrl Pts',(178.442036825202,505.498029375113,-37.8501163050674)) ;
#57160=CARTESIAN_POINT('Ctrl Pts',(178.4393746574,505.498410266084,-37.8454421499372)) ;
#57161=CARTESIAN_POINT('Ctrl Pts',(178.43673506987,505.498791753843,-37.8407543228835)) ;
#57162=CARTESIAN_POINT('Ctrl Pts',(178.434118203299,505.499173780139,-37.8360530912797)) ;
#57163=CARTESIAN_POINT('Ctrl Pts',(178.404193150937,505.503542423556,-37.7822923824075)) ;
#57164=CARTESIAN_POINT('Ctrl Pts',(178.377239393279,505.507980795142,-37.7267726190367)) ;
#57165=CARTESIAN_POINT('Ctrl Pts',(178.353422670534,505.512415602303,-37.6698682440388)) ;
#57166=CARTESIAN_POINT('Ctrl Pts',(178.330049388099,505.516767838394,-37.6140233638335)) ;
#57167=CARTESIAN_POINT('Ctrl Pts',(178.309696939059,505.521116357443,-37.5568450454947)) ;
#57168=CARTESIAN_POINT('Ctrl Pts',(178.292483291909,505.525412119828,-37.4986946008478)) ;
#57169=CARTESIAN_POINT('Ctrl Pts',(178.275280535674,505.529705164323,-37.440580947449)) ;
#57170=CARTESIAN_POINT('Ctrl Pts',(178.261212476853,505.533945376166,-37.3814964112241)) ;
#57171=CARTESIAN_POINT('Ctrl Pts',(178.250362129364,505.53810737924,-37.3218084178744)) ;
#57172=CARTESIAN_POINT('Ctrl Pts',(178.239514522384,505.542268331102,-37.2621355001256)) ;
#57173=CARTESIAN_POINT('Ctrl Pts',(178.231883028496,505.546351103104,-37.2018594527911)) ;
#57174=CARTESIAN_POINT('Ctrl Pts',(178.227516627559,505.550355018515,-37.1413539778099)) ;
#57175=CARTESIAN_POINT('Ctrl Pts',(178.222999602097,505.554497054055,-37.0787612899084)) ;
#57176=CARTESIAN_POINT('Ctrl Pts',(178.221977221747,505.558554667682,-37.0159230896694)) ;
#57177=CARTESIAN_POINT('Ctrl Pts',(178.224463849545,505.562554099107,-36.9532598849088)) ;
#57178=CARTESIAN_POINT('Ctrl Pts',(178.226870699266,505.566425217422,-36.8926070936028)) ;
#57179=CARTESIAN_POINT('Ctrl Pts',(178.232565100846,505.570242206833,-36.8321183759182)) ;
#57180=CARTESIAN_POINT('Ctrl Pts',(178.241520426093,505.574050662793,-36.7721801361307)) ;
#57181=CARTESIAN_POINT('Ctrl Pts',(178.250921004708,505.578048472886,-36.7092618032315)) ;
#57182=CARTESIAN_POINT('Ctrl Pts',(178.263915778421,505.582037255386,-36.6469502675765)) ;
#57183=CARTESIAN_POINT('Ctrl Pts',(178.280420961934,505.586088946602,-36.5856957895303)) ;
#57184=CARTESIAN_POINT('Ctrl Pts',(178.294648206635,505.589581449568,-36.5328952588654)) ;
#57185=CARTESIAN_POINT('Ctrl Pts',(178.311483868444,505.593121357734,-36.4808791417708)) ;
#57186=CARTESIAN_POINT('Ctrl Pts',(178.330834538074,505.596760456215,-36.4299380618792)) ;
#57187=CARTESIAN_POINT('Ctrl Pts',(178.333926185787,505.597341873329,-36.4217992286427)) ;
#57188=CARTESIAN_POINT('Ctrl Pts',(178.337082000965,505.597925822406,-36.413687733639)) ;
#57189=CARTESIAN_POINT('Ctrl Pts',(178.340301570173,505.598512514642,-36.4056046427992)) ;
#57190=CARTESIAN_POINT('Ctrl Pts',(178.340308451531,505.598513768611,-36.4055873663754)) ;
#57191=CARTESIAN_POINT('Ctrl Pts',(178.340315333181,505.598515022592,-36.4055700900813)) ;
#57192=CARTESIAN_POINT('Ctrl Pts',(178.340322215121,505.598516276586,-36.405552813917)) ;
#57193=CARTESIAN_POINT('Ctrl Pts',(178.361122777435,505.602306454293,-36.3533358655596)) ;
#57194=CARTESIAN_POINT('Ctrl Pts',(178.384664367637,505.606221021278,-36.3021240858524)) ;
#57195=CARTESIAN_POINT('Ctrl Pts',(178.41080410433,505.610197626341,-36.2521967746116)) ;
#57196=CARTESIAN_POINT('Ctrl Pts',(178.413432545432,505.61059748776,-36.2471764104621)) ;
#57197=CARTESIAN_POINT('Ctrl Pts',(178.416087218387,505.610997976445,-36.2421690546694)) ;
#57198=CARTESIAN_POINT('Ctrl Pts',(178.418767952148,505.611399029005,-36.2371750046425)) ;
#57199=CARTESIAN_POINT('Ctrl Pts',(178.448046319473,505.615779234284,-36.1826311207183)) ;
#57200=CARTESIAN_POINT('Ctrl Pts',(178.480438320548,505.620226065791,-36.1296710461462)) ;
#57201=CARTESIAN_POINT('Ctrl Pts',(178.515719393852,505.62467032553,-36.0786327386408)) ;
#57202=CARTESIAN_POINT('Ctrl Pts',(178.550956777783,505.62910908184,-36.0276576330572)) ;
#57203=CARTESIAN_POINT('Ctrl Pts',(178.589075856204,505.633544932528,-35.9785992330982)) ;
#57204=CARTESIAN_POINT('Ctrl Pts',(178.629826423725,505.637929521447,-35.9317659650367)) ;
#57205=CARTESIAN_POINT('Ctrl Pts',(178.670539342107,505.642310059478,-35.8849759658764)) ;
#57206=CARTESIAN_POINT('Ctrl Pts',(178.713878846991,505.64663929412,-35.8404068485302)) ;
#57207=CARTESIAN_POINT('Ctrl Pts',(178.759570878723,505.650893055017,-35.7983412968363)) ;
#57208=CARTESIAN_POINT('Ctrl Pts',(178.805235050172,505.655144222224,-35.7563013942139)) ;
#57209=CARTESIAN_POINT('Ctrl Pts',(178.853248932888,505.659320014824,-35.7167620262066)) ;
#57210=CARTESIAN_POINT('Ctrl Pts',(178.903314306228,505.663421273273,-35.6799813653945)) ;
#57211=CARTESIAN_POINT('Ctrl Pts',(178.953384283495,505.667522908868,-35.6431973222944)) ;
#57212=CARTESIAN_POINT('Ctrl Pts',(179.005506239459,505.671550130967,-35.6091726680432)) ;
#57213=CARTESIAN_POINT('Ctrl Pts',(179.059355946802,505.675527710287,-35.5781401733316)) ;
#57214=CARTESIAN_POINT('Ctrl Pts',(179.113203662447,505.679505142491,-35.5471088263952)) ;
#57215=CARTESIAN_POINT('Ctrl Pts',(179.168779140413,505.683433228105,-35.5190697626465)) ;
#57216=CARTESIAN_POINT('Ctrl Pts',(179.225730361398,505.687357503393,-35.4942264014249)) ;
#57217=CARTESIAN_POINT('Ctrl Pts',(179.282738343372,505.691285689847,-35.4693582798255)) ;
#57218=CARTESIAN_POINT('Ctrl Pts',(179.341124914445,505.69521056244,-35.4476928080947)) ;
#57219=CARTESIAN_POINT('Ctrl Pts',(179.400507193109,505.699192690673,-35.4293977783462)) ;
#57220=CARTESIAN_POINT('Ctrl Pts',(179.45601305068,505.7029148692,-35.4122970314849)) ;
#57221=CARTESIAN_POINT('Ctrl Pts',(179.512388503592,505.706687725966,-35.398141268249)) ;
#57222=CARTESIAN_POINT('Ctrl Pts',(179.569297170772,505.710565160536,-35.3870308445087)) ;
#57223=CARTESIAN_POINT('Origin',(179.888527625402,505.710565160536,-37.0221601717597)) ;
#57224=CARTESIAN_POINT('Ctrl Pts',(180.464073449582,504.877005588434,-35.458733485193)) ;
#57225=CARTESIAN_POINT('Ctrl Pts',(180.486923937135,504.878624850681,-35.4671454579477)) ;
#57226=CARTESIAN_POINT('Ctrl Pts',(180.509589115676,504.880260874332,-35.4760580625355)) ;
#57227=CARTESIAN_POINT('Ctrl Pts',(180.596969805277,504.886691145551,-35.5126506627681)) ;
#57228=CARTESIAN_POINT('Ctrl Pts',(180.660089881212,504.891606583489,-35.5439184757573)) ;
#57229=CARTESIAN_POINT('Ctrl Pts',(180.811340399425,504.904066896042,-35.6311744752597)) ;
#57230=CARTESIAN_POINT('Ctrl Pts',(180.896550775369,504.911721908279,-35.6916297508855)) ;
#57231=CARTESIAN_POINT('Ctrl Pts',(181.018554427028,504.923365842585,-35.7966739263697)) ;
#57232=CARTESIAN_POINT('Ctrl Pts',(181.059648271787,504.927424644711,-35.835882436113)) ;
#57233=CARTESIAN_POINT('Ctrl Pts',(181.119436118134,504.93345114912,-35.8990690361585)) ;
#57234=CARTESIAN_POINT('Ctrl Pts',(181.139609137954,504.935506399607,-35.9215853046345)) ;
#57235=CARTESIAN_POINT('Ctrl Pts',(181.186316283446,504.940304605392,-35.9766635224297)) ;
#57236=CARTESIAN_POINT('Ctrl Pts',(181.212252938322,504.943009445288,-36.009702430912)) ;
#57237=CARTESIAN_POINT('Ctrl Pts',(181.272044681172,504.949444149712,-36.0920988537308)) ;
#57238=CARTESIAN_POINT('Ctrl Pts',(181.304543412835,504.953117869027,-36.1423682932357)) ;
#57239=CARTESIAN_POINT('Ctrl Pts',(181.396485733974,504.964430254262,-36.302928793793)) ;
#57240=CARTESIAN_POINT('Ctrl Pts',(181.446249868579,504.972008724939,-36.4182320730915)) ;
#57241=CARTESIAN_POINT('Ctrl Pts',(181.497560460995,504.983350705534,-36.587178359447)) ;
#57242=CARTESIAN_POINT('Ctrl Pts',(181.510207705152,504.986717248839,-36.6369996831346)) ;
#57243=CARTESIAN_POINT('Ctrl Pts',(181.532230036138,504.994063837716,-36.7443365911058)) ;
#57244=CARTESIAN_POINT('Ctrl Pts',(181.540930631925,504.998061275522,-36.8019184880018)) ;
#57245=CARTESIAN_POINT('Ctrl Pts',(181.553359292123,505.007013245318,-36.9288686931117)) ;
#57246=CARTESIAN_POINT('Ctrl Pts',(181.555799197202,505.011996690765,-36.9982535435589)) ;
#57247=CARTESIAN_POINT('Ctrl Pts',(181.55070834816,505.025548792702,-37.1849080138226)) ;
#57248=CARTESIAN_POINT('Ctrl Pts',(181.53511901935,505.034191249214,-37.3015742218307)) ;
#57249=CARTESIAN_POINT('Ctrl Pts',(181.500275399704,505.044425139138,-37.4449292715406)) ;
#57250=CARTESIAN_POINT('Ctrl Pts',(181.492361784658,505.046478681483,-37.4740242787658)) ;
#57251=CARTESIAN_POINT('Ctrl Pts',(181.471965229593,505.051183285923,-37.5417024901008)) ;
#57252=CARTESIAN_POINT('Ctrl Pts',(181.458855805208,505.053801190539,-37.5800749980219)) ;
#57253=CARTESIAN_POINT('Ctrl Pts',(181.424230357451,505.059936245267,-37.6704973274354)) ;
#57254=CARTESIAN_POINT('Ctrl Pts',(181.401450364654,505.063404285732,-37.7220098758374)) ;
#57255=CARTESIAN_POINT('Ctrl Pts',(181.315532245264,505.075086103401,-37.8923972549)) ;
#57256=CARTESIAN_POINT('Ctrl Pts',(181.240640650181,505.083196344975,-38.0047289218465)) ;
#57257=CARTESIAN_POINT('Ctrl Pts',(181.12022837144,505.095103941257,-38.1451082654634)) ;
#57258=CARTESIAN_POINT('Ctrl Pts',(181.085677863873,505.098415370472,-38.1818711441832)) ;
#57259=CARTESIAN_POINT('Ctrl Pts',(181.006937293535,505.105788735553,-38.2583804156556)) ;
#57260=CARTESIAN_POINT('Ctrl Pts',(180.962182408179,505.109874869627,-38.2974423129976)) ;
#57261=CARTESIAN_POINT('Ctrl Pts',(180.858604203979,505.119125960952,-38.3785221255862)) ;
#57262=CARTESIAN_POINT('Ctrl Pts',(180.79893903227,505.12432511874,-38.4192698682888)) ;
#57263=CARTESIAN_POINT('Ctrl Pts',(180.643044619778,505.137487624959,-38.5115000736188)) ;
#57264=CARTESIAN_POINT('Ctrl Pts',(180.544040107551,505.145488389746,-38.5576523344385)) ;
#57265=CARTESIAN_POINT('Ctrl Pts',(180.411996283235,505.155223222595,-38.6040884135458)) ;
#57266=CARTESIAN_POINT('Ctrl Pts',(180.382475976189,505.157340538829,-38.6135532887174)) ;
#57267=CARTESIAN_POINT('Ctrl Pts',(180.315245594623,505.162009624704,-38.6330571026779)) ;
#57268=CARTESIAN_POINT('Ctrl Pts',(180.277414166837,505.164536198418,-38.642606105986)) ;
#57269=CARTESIAN_POINT('Ctrl Pts',(180.18773445598,505.170366053779,-38.6619196979945)) ;
#57270=CARTESIAN_POINT('Ctrl Pts',(180.135688521192,505.17362706911,-38.6705679818234)) ;
#57271=CARTESIAN_POINT('Ctrl Pts',(179.948206921303,505.185206679317,-38.692639760043)) ;
#57272=CARTESIAN_POINT('Ctrl Pts',(179.811670724101,505.193377618667,-38.6919367670938)) ;
#57273=CARTESIAN_POINT('Ctrl Pts',(179.625414179962,505.205419327044,-38.6680657311009)) ;
#57274=CARTESIAN_POINT('Ctrl Pts',(179.574426294266,505.208804115516,-38.6591003585801)) ;
#57275=CARTESIAN_POINT('Ctrl Pts',(179.468049427096,505.216102419562,-38.6352426992973)) ;
#57276=CARTESIAN_POINT('Ctrl Pts',(179.412846936446,505.220029163233,-38.619834619492)) ;
#57277=CARTESIAN_POINT('Ctrl Pts',(179.294835284153,505.228748196148,-38.580236683263)) ;
#57278=CARTESIAN_POINT('Ctrl Pts',(179.232476310779,505.23356548482,-38.5550228622864)) ;
#57279=CARTESIAN_POINT('Ctrl Pts',(179.065399116446,505.246979858641,-38.4754019923391)) ;
#57280=CARTESIAN_POINT('Ctrl Pts',(178.964661038147,505.25566904535,-38.4135356981219)) ;
#57281=CARTESIAN_POINT('Ctrl Pts',(178.846316034503,505.266082739799,-38.3222931380907)) ;
#57282=CARTESIAN_POINT('Ctrl Pts',(178.821886702845,505.268242531688,-38.3023275462298)) ;
#57283=CARTESIAN_POINT('Ctrl Pts',(178.769472712104,505.272875614223,-38.2569473764955)) ;
#57284=CARTESIAN_POINT('Ctrl Pts',(178.74175697741,505.275329412413,-38.2312511513939)) ;
#57285=CARTESIAN_POINT('Ctrl Pts',(178.679437613317,505.280923981761,-38.1693998246943)) ;
#57286=CARTESIAN_POINT('Ctrl Pts',(178.645540687169,505.284027484449,-38.1325842648028)) ;
#57287=CARTESIAN_POINT('Ctrl Pts',(178.518133287261,505.296197058153,-37.9810484340822)) ;
#57288=CARTESIAN_POINT('Ctrl Pts',(178.438435651292,505.305051170906,-37.8556334975304)) ;
#57289=CARTESIAN_POINT('Ctrl Pts',(178.355075997403,505.317860434018,-37.6753450716706)) ;
#57290=CARTESIAN_POINT('Ctrl Pts',(178.335919122793,505.321194422621,-37.6284029544816)) ;
#57291=CARTESIAN_POINT('Ctrl Pts',(178.298555005547,505.328694032454,-37.5233966030894)) ;
#57292=CARTESIAN_POINT('Ctrl Pts',(178.281329447934,505.332887893431,-37.4650633895282)) ;
#57293=CARTESIAN_POINT('Ctrl Pts',(178.227850044723,505.349256782826,-37.2391424609511)) ;
#57294=CARTESIAN_POINT('Ctrl Pts',(178.214347049073,505.362094189734,-37.0672986674056)) ;
#57295=CARTESIAN_POINT('Ctrl Pts',(178.229778637586,505.376419274407,-36.8633981141818)) ;
#57296=CARTESIAN_POINT('Ctrl Pts',(178.233263998269,505.378701134479,-36.830440431642)) ;
#57297=CARTESIAN_POINT('Ctrl Pts',(178.242426744404,505.383266641816,-36.7630814145887)) ;
#57298=CARTESIAN_POINT('Ctrl Pts',(178.248205197249,505.385544378412,-36.7287104772704)) ;
#57299=CARTESIAN_POINT('Ctrl Pts',(178.275608284385,505.394482074718,-36.5920812460578)) ;
#57300=CARTESIAN_POINT('Ctrl Pts',(178.3057558051,505.400790987909,-36.4917688232903)) ;
#57301=CARTESIAN_POINT('Ctrl Pts',(178.381850620507,505.413139471535,-36.3045218641273)) ;
#57302=CARTESIAN_POINT('Ctrl Pts',(178.426461340629,505.419147620642,-36.217524065389)) ;
#57303=CARTESIAN_POINT('Ctrl Pts',(178.505172048478,505.428661250585,-36.0924258962436)) ;
#57304=CARTESIAN_POINT('Ctrl Pts',(178.533824685386,505.431958307056,-36.0511516694038)) ;
#57305=CARTESIAN_POINT('Ctrl Pts',(178.599904055385,505.43927009448,-35.9645926527049)) ;
#57306=CARTESIAN_POINT('Ctrl Pts',(178.637948235698,505.443307499942,-35.9198673577203)) ;
#57307=CARTESIAN_POINT('Ctrl Pts',(178.726853588352,505.452403122182,-35.8258877671727)) ;
#57308=CARTESIAN_POINT('Ctrl Pts',(178.778654107249,505.457493181885,-35.7776790852677)) ;
#57309=CARTESIAN_POINT('Ctrl Pts',(178.921445261153,505.470907251014,-35.6608131771621)) ;
#57310=CARTESIAN_POINT('Ctrl Pts',(179.016698742053,505.479288438908,-35.5979298242953)) ;
#57311=CARTESIAN_POINT('Ctrl Pts',(179.144581653435,505.489315980419,-35.5311789726886)) ;
#57312=CARTESIAN_POINT('Ctrl Pts',(179.17192020229,505.491391850237,-35.517848055946)) ;
#57313=CARTESIAN_POINT('Ctrl Pts',(179.236059184774,505.496089950105,-35.4887185677652)) ;
#57314=CARTESIAN_POINT('Ctrl Pts',(179.27309282732,505.498681941617,-35.4734836777184)) ;
#57315=CARTESIAN_POINT('Ctrl Pts',(179.362167115387,505.504716207531,-35.4405412402789)) ;
#57316=CARTESIAN_POINT('Ctrl Pts',(179.414605851469,505.508112620284,-35.4240447770765)) ;
#57317=CARTESIAN_POINT('Ctrl Pts',(179.600606287242,505.51991486733,-35.3754951136464)) ;
#57318=CARTESIAN_POINT('Ctrl Pts',(179.737206831435,505.528200660572,-35.3573770654938)) ;
#57319=CARTESIAN_POINT('Ctrl Pts',(179.925493396058,505.540354144688,-35.3557891850531)) ;
#57320=CARTESIAN_POINT('Ctrl Pts',(179.976496111569,505.543712973918,-35.357702502675)) ;
#57321=CARTESIAN_POINT('Ctrl Pts',(180.088440052483,505.55127769403,-35.3670613851399)) ;
#57322=CARTESIAN_POINT('Ctrl Pts',(180.149217077004,505.555512452928,-35.3755405144951)) ;
#57323=CARTESIAN_POINT('Ctrl Pts',(180.296031826649,505.566070634002,-35.4043549666717)) ;
#57324=CARTESIAN_POINT('Ctrl Pts',(180.38118326896,505.572482028514,-35.4282214813861)) ;
#57325=CARTESIAN_POINT('Ctrl Pts',(180.464032893301,505.578914864621,-35.458718555766)) ;
#57326=CARTESIAN_POINT('Origin',(179.888527625402,504.710565160536,-37.0221601717597)) ;
#57327=CARTESIAN_POINT('',(180.464073435742,504.178966917533,-35.4587334800982)) ;
#57328=CARTESIAN_POINT('',(180.464073435525,504.369601015799,-35.4587334800181)) ;
#57329=CARTESIAN_POINT('',(180.464073435736,504.710565160536,-35.4587334800957)) ;
#57330=CARTESIAN_POINT('',(179.889599033433,504.139907930539,-35.3556857802299)) ;
#57331=CARTESIAN_POINT('Ctrl Pts',(179.889579047996,504.140180283237,-35.3561605035393)) ;
#57332=CARTESIAN_POINT('Ctrl Pts',(179.935879931379,504.143526942088,-35.3561897243104)) ;
#57333=CARTESIAN_POINT('Ctrl Pts',(179.982163158329,504.146845416725,-35.3581491101495)) ;
#57334=CARTESIAN_POINT('Ctrl Pts',(180.059263424997,504.152272397822,-35.3646408418133)) ;
#57335=CARTESIAN_POINT('Ctrl Pts',(180.090142868883,504.154418486497,-35.3681128098242)) ;
#57336=CARTESIAN_POINT('Ctrl Pts',(180.152752703499,504.158690116225,-35.376932162373)) ;
#57337=CARTESIAN_POINT('Ctrl Pts',(180.184459988916,504.160808303287,-35.3823387500492)) ;
#57338=CARTESIAN_POINT('Ctrl Pts',(180.300362090089,504.168446632402,-35.4055734397612)) ;
#57339=CARTESIAN_POINT('Ctrl Pts',(180.383304656688,504.173715175109,-35.4289999897851)) ;
#57340=CARTESIAN_POINT('Ctrl Pts',(180.464073435749,504.178966917533,-35.4587334801008)) ;
#57341=CARTESIAN_POINT('',(180.967886278451,503.710565160535,-38.2912310516111)) ;
#57342=CARTESIAN_POINT('Ctrl Pts',(179.889599033433,504.139907930539,-35.3556857802299)) ;
#57343=CARTESIAN_POINT('Ctrl Pts',(179.829734963427,504.135659048629,-35.3557807655152)) ;
#57344=CARTESIAN_POINT('Ctrl Pts',(179.769770760995,504.131370982823,-35.3591282310602)) ;
#57345=CARTESIAN_POINT('Ctrl Pts',(179.710083728143,504.127103688023,-35.3657033091904)) ;
#57346=CARTESIAN_POINT('Ctrl Pts',(179.650461321867,504.122841013668,-35.3722712681061)) ;
#57347=CARTESIAN_POINT('Ctrl Pts',(179.591115449233,504.118599323853,-35.3820596163943)) ;
#57348=CARTESIAN_POINT('Ctrl Pts',(179.532413623388,504.114418083644,-35.3950066269203)) ;
#57349=CARTESIAN_POINT('Ctrl Pts',(179.473752342522,504.110239731391,-35.407944695028)) ;
#57350=CARTESIAN_POINT('Ctrl Pts',(179.415734238346,504.106121843499,-35.4240369935909)) ;
#57351=CARTESIAN_POINT('Ctrl Pts',(179.358717669987,504.102080905547,-35.4431872457158)) ;
#57352=CARTESIAN_POINT('Ctrl Pts',(179.301717936172,504.09804116071,-35.4623318435938)) ;
#57353=CARTESIAN_POINT('Ctrl Pts',(179.245719239883,504.09407829802,-35.4845326321906)) ;
#57354=CARTESIAN_POINT('Ctrl Pts',(179.191070391662,504.090185345868,-35.5096589162831)) ;
#57355=CARTESIAN_POINT('Ctrl Pts',(179.13637745663,504.086289253159,-35.5348054704776)) ;
#57356=CARTESIAN_POINT('Ctrl Pts',(179.083036722165,504.082463045992,-35.5628823816942)) ;
#57357=CARTESIAN_POINT('Ctrl Pts',(179.031386604159,504.078677432237,-35.5937226921901)) ;
#57358=CARTESIAN_POINT('Ctrl Pts',(178.979717222524,504.074890406585,-35.6245745050081)) ;
#57359=CARTESIAN_POINT('Ctrl Pts',(178.929740000811,504.071143714672,-35.6581920020274)) ;
#57360=CARTESIAN_POINT('Ctrl Pts',(178.88177912004,504.067388889991,-35.6943693550852)) ;
#57361=CARTESIAN_POINT('Ctrl Pts',(178.833729330466,504.063627104699,-35.7306137729074)) ;
#57362=CARTESIAN_POINT('Ctrl Pts',(178.787703836856,504.059856666008,-35.7694278355667)) ;
#57363=CARTESIAN_POINT('Ctrl Pts',(178.744008382537,504.056015428548,-35.810561822063)) ;
#57364=CARTESIAN_POINT('Ctrl Pts',(178.705760217749,504.05265305858,-35.8465678441633)) ;
#57365=CARTESIAN_POINT('Ctrl Pts',(178.669297385938,504.049235914134,-35.8843508652821)) ;
#57366=CARTESIAN_POINT('Ctrl Pts',(178.634806823727,504.045719394504,-35.9237141442276)) ;
#57367=CARTESIAN_POINT('Ctrl Pts',(178.634784961163,504.045717165485,-35.9237390954658)) ;
#57368=CARTESIAN_POINT('Ctrl Pts',(178.634763099389,504.045714936425,-35.9237640473391)) ;
#57369=CARTESIAN_POINT('Ctrl Pts',(178.634741238406,504.045712707326,-35.9237889998475)) ;
#57370=CARTESIAN_POINT('Ctrl Pts',(178.598143074702,504.041980901396,-35.9655627841434)) ;
#57371=CARTESIAN_POINT('Ctrl Pts',(178.563626661024,504.038126723739,-36.0092842373027)) ;
#57372=CARTESIAN_POINT('Ctrl Pts',(178.531374867164,504.034213647399,-36.0547034201323)) ;
#57373=CARTESIAN_POINT('Ctrl Pts',(178.528442702617,504.033857890948,-36.0588326948703)) ;
#57374=CARTESIAN_POINT('Ctrl Pts',(178.525529257917,504.03350164767,-36.0629759666304)) ;
#57375=CARTESIAN_POINT('Ctrl Pts',(178.522634670932,504.033144965263,-36.0671330263022)) ;
#57376=CARTESIAN_POINT('Ctrl Pts',(178.487473308412,504.028812243707,-36.1176299997569)) ;
#57377=CARTESIAN_POINT('Ctrl Pts',(178.455093838431,504.024415388031,-36.1701674097863)) ;
#57378=CARTESIAN_POINT('Ctrl Pts',(178.425696700947,504.020025419779,-36.2243907539794)) ;
#57379=CARTESIAN_POINT('Ctrl Pts',(178.396735494467,504.015700550493,-36.277810018629)) ;
#57380=CARTESIAN_POINT('Ctrl Pts',(178.370668398909,504.011382644977,-36.3328654656163)) ;
#57381=CARTESIAN_POINT('Ctrl Pts',(178.347649685094,504.00711886339,-36.3892070328538)) ;
#57382=CARTESIAN_POINT('Ctrl Pts',(178.324644339505,504.002857558013,-36.4455158794604)) ;
#57383=CARTESIAN_POINT('Ctrl Pts',(178.304683711337,503.99865044499,-36.5031093346559)) ;
#57384=CARTESIAN_POINT('Ctrl Pts',(178.287888105595,503.994520680875,-36.5616276682746)) ;
#57385=CARTESIAN_POINT('Ctrl Pts',(178.271095985438,503.990391773808,-36.62013385761)) ;
#57386=CARTESIAN_POINT('Ctrl Pts',(178.257467612023,503.986340183306,-36.6795645313902)) ;
#57387=CARTESIAN_POINT('Ctrl Pts',(178.247090129816,503.982364183077,-36.7395500866227)) ;
#57388=CARTESIAN_POINT('Ctrl Pts',(178.236427334499,503.97827886876,-36.8011848535858)) ;
#57389=CARTESIAN_POINT('Ctrl Pts',(178.229197007305,503.974273344842,-36.8634054572202)) ;
#57390=CARTESIAN_POINT('Ctrl Pts',(178.225455507491,503.970319375166,-36.9258001115029)) ;
#57391=CARTESIAN_POINT('Ctrl Pts',(178.221809130089,503.966465929654,-36.98660846875)) ;
#57392=CARTESIAN_POINT('Ctrl Pts',(178.221476603408,503.96266107936,-37.0475820399051)) ;
#57393=CARTESIAN_POINT('Ctrl Pts',(178.224470929098,503.958857193105,-37.1083301596863)) ;
#57394=CARTESIAN_POINT('Ctrl Pts',(178.227582423468,503.954904459871,-37.1714553679145)) ;
#57395=CARTESIAN_POINT('Ctrl Pts',(178.234287112341,503.950952338808,-37.2343370034491)) ;
#57396=CARTESIAN_POINT('Ctrl Pts',(178.244548223404,503.946929511884,-37.2965277989752)) ;
#57397=CARTESIAN_POINT('Ctrl Pts',(178.253404424326,503.943457474277,-37.3502036804004)) ;
#57398=CARTESIAN_POINT('Ctrl Pts',(178.264909836953,503.939932104169,-37.403365924728)) ;
#57399=CARTESIAN_POINT('Ctrl Pts',(178.279002227418,503.936302788681,-37.4557206286662)) ;
#57400=CARTESIAN_POINT('Ctrl Pts',(178.281228634172,503.935729406008,-37.4639919625257)) ;
#57401=CARTESIAN_POINT('Ctrl Pts',(178.283519568417,503.935153428887,-37.4722432372026)) ;
#57402=CARTESIAN_POINT('Ctrl Pts',(178.285874739581,503.934574657738,-37.4804734042846)) ;
#57403=CARTESIAN_POINT('Ctrl Pts',(178.285884419069,503.934572279054,-37.4805072293439)) ;
#57404=CARTESIAN_POINT('Ctrl Pts',(178.285894099642,503.934569900322,-37.4805410540468)) ;
#57405=CARTESIAN_POINT('Ctrl Pts',(178.2859037813,503.934567521544,-37.4805748783931)) ;
#57406=CARTESIAN_POINT('Ctrl Pts',(178.301034282463,503.930849964868,-37.5334355875821)) ;
#57407=CARTESIAN_POINT('Ctrl Pts',(178.318879702032,503.927006840452,-37.5856215868244)) ;
#57408=CARTESIAN_POINT('Ctrl Pts',(178.339333163539,503.923100959956,-37.6368499635939)) ;
#57409=CARTESIAN_POINT('Ctrl Pts',(178.341327732312,503.922720068571,-37.6418456226678)) ;
#57410=CARTESIAN_POINT('Ctrl Pts',(178.343347068838,503.922338580399,-37.6468321520644)) ;
#57411=CARTESIAN_POINT('Ctrl Pts',(178.345391051792,503.921956553687,-37.6518092750848)) ;
#57412=CARTESIAN_POINT('Ctrl Pts',(178.368764899837,503.917587909471,-37.7087248755417)) ;
#57413=CARTESIAN_POINT('Ctrl Pts',(178.395366603873,503.913149537041,-37.7644141769854)) ;
#57414=CARTESIAN_POINT('Ctrl Pts',(178.425006750074,503.908714728987,-37.8185141372354)) ;
#57415=CARTESIAN_POINT('Ctrl Pts',(178.454095033182,503.904362491608,-37.8716068227185)) ;
#57416=CARTESIAN_POINT('Ctrl Pts',(178.4861092995,503.900013971222,-37.9231691105662)) ;
#57417=CARTESIAN_POINT('Ctrl Pts',(178.520840616235,503.895718207472,-37.9728834949947)) ;
#57418=CARTESIAN_POINT('Ctrl Pts',(178.555549958685,503.891425161625,-38.022566425446)) ;
#57419=CARTESIAN_POINT('Ctrl Pts',(178.592972820244,503.887184948401,-38.0704038862008)) ;
#57420=CARTESIAN_POINT('Ctrl Pts',(178.632873694272,503.883022943935,-38.1161018881213)) ;
#57421=CARTESIAN_POINT('Ctrl Pts',(178.672764490276,503.878861990693,-38.1617883477998)) ;
#57422=CARTESIAN_POINT('Ctrl Pts',(178.715132046167,503.874779217299,-38.2053363939955)) ;
#57423=CARTESIAN_POINT('Ctrl Pts',(178.759714728454,503.870775300502,-38.2464747332912)) ;
#57424=CARTESIAN_POINT('Ctrl Pts',(178.805835339648,503.866633264169,-38.289032185076)) ;
#57425=CARTESIAN_POINT('Ctrl Pts',(178.854326775488,503.862575649729,-38.3290104882774)) ;
#57426=CARTESIAN_POINT('Ctrl Pts',(178.904869225075,503.858576217504,-38.366136231121)) ;
#57427=CARTESIAN_POINT('Ctrl Pts',(178.953790136573,503.854705097851,-38.4020708800111)) ;
#57428=CARTESIAN_POINT('Ctrl Pts',(179.0046325257,503.850888107131,-38.4353329188909)) ;
#57429=CARTESIAN_POINT('Ctrl Pts',(179.057077687018,503.847079649913,-38.4657022473033)) ;
#57430=CARTESIAN_POINT('Ctrl Pts',(179.112130378247,503.843081839363,-38.497581513529)) ;
#57431=CARTESIAN_POINT('Ctrl Pts',(179.168949600054,503.839093056456,-38.5262723939944)) ;
#57432=CARTESIAN_POINT('Ctrl Pts',(179.227131085679,503.835041364962,-38.5515596619594)) ;
#57433=CARTESIAN_POINT('Ctrl Pts',(179.277282753221,503.831548860729,-38.5733569509497)) ;
#57434=CARTESIAN_POINT('Ctrl Pts',(179.328447463615,503.828008951363,-38.5926258227454)) ;
#57435=CARTESIAN_POINT('Ctrl Pts',(179.38033975834,503.824369851754,-38.6092581066902)) ;
#57436=CARTESIAN_POINT('Ctrl Pts',(179.388630549264,503.823788435685,-38.6119154335535)) ;
#57437=CARTESIAN_POINT('Ctrl Pts',(179.396939973992,503.823204487666,-38.6145055474257)) ;
#57438=CARTESIAN_POINT('Ctrl Pts',(179.40526694138,503.822617796502,-38.6170281069471)) ;
#57439=CARTESIAN_POINT('Ctrl Pts',(179.405284738878,503.822616542548,-38.6170334984955)) ;
#57440=CARTESIAN_POINT('Ctrl Pts',(179.405302536456,503.822615288581,-38.6170388897353)) ;
#57441=CARTESIAN_POINT('Ctrl Pts',(179.405320334114,503.822614034602,-38.6170442806666)) ;
#57442=CARTESIAN_POINT('Ctrl Pts',(179.459114130303,503.818823856251,-38.6333384837133)) ;
#57443=CARTESIAN_POINT('Ctrl Pts',(179.51383105719,503.814909288754,-38.6468629521616)) ;
#57444=CARTESIAN_POINT('Ctrl Pts',(179.569163664211,503.810932683327,-38.6575552545591)) ;
#57445=CARTESIAN_POINT('Ctrl Pts',(179.574727537931,503.810532822709,-38.6586304003642)) ;
#57446=CARTESIAN_POINT('Ctrl Pts',(179.580297596578,503.810132334828,-38.6596769268195)) ;
#57447=CARTESIAN_POINT('Ctrl Pts',(179.585873500983,503.809731283076,-38.6606947822229)) ;
#57448=CARTESIAN_POINT('Ctrl Pts',(179.646772382743,503.805351078281,-38.6718115897136)) ;
#57449=CARTESIAN_POINT('Ctrl Pts',(179.708374311401,503.800904247445,-38.6795065722235)) ;
#57450=CARTESIAN_POINT('Ctrl Pts',(179.770275049275,503.796459988522,-38.6837445858013)) ;
#57451=CARTESIAN_POINT('Ctrl Pts',(179.832099134149,503.792021233019,-38.6879773513567)) ;
#57452=CARTESIAN_POINT('Ctrl Pts',(179.894221385486,503.787585383282,-38.6887620718713)) ;
#57453=CARTESIAN_POINT('Ctrl Pts',(179.956244665505,503.783200795414,-38.6861020651215)) ;
#57454=CARTESIAN_POINT('Ctrl Pts',(180.018210642834,503.778820258423,-38.6834445159254)) ;
#57455=CARTESIAN_POINT('Ctrl Pts',(180.080077914972,503.774491024919,-38.6773487223369)) ;
#57456=CARTESIAN_POINT('Ctrl Pts',(180.141454597477,503.770237265217,-38.6678527022962)) ;
#57457=CARTESIAN_POINT('Ctrl Pts',(180.202793856304,503.765986099193,-38.6583624723372)) ;
#57458=CARTESIAN_POINT('Ctrl Pts',(180.263643139769,503.761810307832,-38.6454761070374)) ;
#57459=CARTESIAN_POINT('Ctrl Pts',(180.323614662971,503.757709050637,-38.6292657966812)) ;
#57460=CARTESIAN_POINT('Ctrl Pts',(180.383591701399,503.753607416273,-38.6130539955585)) ;
#57461=CARTESIAN_POINT('Ctrl Pts',(180.442690750923,503.749580195423,-38.5935174427467)) ;
#57462=CARTESIAN_POINT('Ctrl Pts',(180.500527671737,503.745602617334,-38.5707644991912)) ;
#57463=CARTESIAN_POINT('Ctrl Pts',(180.558362453561,503.741625186349,-38.5480123971105)) ;
#57464=CARTESIAN_POINT('Ctrl Pts',(180.614935016818,503.737697101935,-38.5220438186177)) ;
#57465=CARTESIAN_POINT('Ctrl Pts',(180.669866841495,503.733772827799,-38.4930071535775)) ;
#57466=CARTESIAN_POINT('Ctrl Pts',(180.724853414895,503.729844642471,-38.4639415486586)) ;
#57467=CARTESIAN_POINT('Ctrl Pts',(180.778195592547,503.725919770956,-38.4318013003984)) ;
#57468=CARTESIAN_POINT('Ctrl Pts',(180.829523466653,503.721937643725,-38.3967811409211)) ;
#57469=CARTESIAN_POINT('Ctrl Pts',(180.877500769541,503.718215461039,-38.3640470207639)) ;
#57470=CARTESIAN_POINT('Ctrl Pts',(180.923717771023,503.714442599911,-38.328796849899)) ;
#57471=CARTESIAN_POINT('Ctrl Pts',(180.967886278451,503.710565160535,-38.2912310516112)) ;
#57472=CARTESIAN_POINT('',(180.986277812533,503.710572730308,-35.767785970461)) ;
#57473=CARTESIAN_POINT('Origin',(179.888527625402,503.710565160536,-37.0221601717597)) ;
#57474=CARTESIAN_POINT('',(179.889393904536,504.332863786117,-35.3566333596088)) ;
#57475=CARTESIAN_POINT('Ctrl Pts',(180.986277823167,503.710572730446,-35.7677859583096)) ;
#57476=CARTESIAN_POINT('Ctrl Pts',(181.025946282702,503.714173642747,-35.80254219037)) ;
#57477=CARTESIAN_POINT('Ctrl Pts',(181.063994730973,503.717871345489,-35.8392839762004)) ;
#57478=CARTESIAN_POINT('Ctrl Pts',(181.100234837561,503.721611907053,-35.8778191803887)) ;
#57479=CARTESIAN_POINT('Ctrl Pts',(181.141662721888,503.725887930674,-35.9218707059471)) ;
#57480=CARTESIAN_POINT('Ctrl Pts',(181.180728271362,503.730219400517,-35.968266856604)) ;
#57481=CARTESIAN_POINT('Ctrl Pts',(181.217191089831,503.734540179259,-36.0167042937996)) ;
#57482=CARTESIAN_POINT('Ctrl Pts',(181.253616739054,503.738856553511,-36.0650923551351)) ;
#57483=CARTESIAN_POINT('Ctrl Pts',(181.28744524273,503.743161960478,-36.1155174111814)) ;
#57484=CARTESIAN_POINT('Ctrl Pts',(181.318471176994,503.747411226951,-36.1676599529123)) ;
#57485=CARTESIAN_POINT('Ctrl Pts',(181.349477256015,503.75165777408,-36.2197691256952)) ;
#57486=CARTESIAN_POINT('Ctrl Pts',(181.37768444688,503.755848134438,-36.2735935477084)) ;
#57487=CARTESIAN_POINT('Ctrl Pts',(181.402919132954,503.759961017888,-36.3287984240804)) ;
#57488=CARTESIAN_POINT('Ctrl Pts',(181.428147243903,503.764072829689,-36.3839889163229)) ;
#57489=CARTESIAN_POINT('Ctrl Pts',(181.450404341474,503.768107214459,-36.4405591329151)) ;
#57490=CARTESIAN_POINT('Ctrl Pts',(181.469548102683,503.772067476304,-36.4981589818455)) ;
#57491=CARTESIAN_POINT('Ctrl Pts',(181.48870799007,503.776031074165,-36.5558073513022)) ;
#57492=CARTESIAN_POINT('Ctrl Pts',(181.504749098426,503.779920548214,-36.6144870871759)) ;
#57493=CARTESIAN_POINT('Ctrl Pts',(181.517561865967,503.783762848219,-36.6738316995243)) ;
#57494=CARTESIAN_POINT('Ctrl Pts',(181.530379446178,503.78760659145,-36.7331986026101)) ;
#57495=CARTESIAN_POINT('Ctrl Pts',(181.539965920586,503.791403398421,-36.7932308646697)) ;
#57496=CARTESIAN_POINT('Ctrl Pts',(181.546248715336,503.795200953853,-36.8535461696402)) ;
#57497=CARTESIAN_POINT('Ctrl Pts',(181.552543441867,503.7990057213,-36.9139760206226)) ;
#57498=CARTESIAN_POINT('Ctrl Pts',(181.555521397616,503.802811714112,-36.9746898924054)) ;
#57499=CARTESIAN_POINT('Ctrl Pts',(181.555153363817,503.806682125672,-37.0352885712453)) ;
#57500=CARTESIAN_POINT('Ctrl Pts',(181.554822660227,503.810159955687,-37.0897406368495)) ;
#57501=CARTESIAN_POINT('Ctrl Pts',(181.551790367297,503.813690388526,-37.1441000848864)) ;
#57502=CARTESIAN_POINT('Ctrl Pts',(181.546071963646,503.817323767339,-37.1980669538674)) ;
#57503=CARTESIAN_POINT('Ctrl Pts',(181.545561384502,503.817648180857,-37.2028854940467)) ;
#57504=CARTESIAN_POINT('Ctrl Pts',(181.545029409859,503.817973415077,-37.2077009334435)) ;
#57505=CARTESIAN_POINT('Ctrl Pts',(181.544476061327,503.818299505835,-37.2125130758366)) ;
#57506=CARTESIAN_POINT('Ctrl Pts',(181.544472262003,503.818301744794,-37.2125461162941)) ;
#57507=CARTESIAN_POINT('Ctrl Pts',(181.544468461671,503.818303983793,-37.2125791565962)) ;
#57508=CARTESIAN_POINT('Ctrl Pts',(181.544464660332,503.818306222832,-37.2126121967428)) ;
#57509=CARTESIAN_POINT('Ctrl Pts',(181.538117217828,503.822044950919,-37.2677823393863)) ;
#57510=CARTESIAN_POINT('Ctrl Pts',(181.528929085212,503.825906180113,-37.322717557164)) ;
#57511=CARTESIAN_POINT('Ctrl Pts',(181.516962532995,503.829826849693,-37.3771152557338)) ;
#57512=CARTESIAN_POINT('Ctrl Pts',(181.515848262687,503.830191924413,-37.3821805192507)) ;
#57513=CARTESIAN_POINT('Ctrl Pts',(181.514709928829,503.83055751451,-37.387241096116)) ;
#57514=CARTESIAN_POINT('Ctrl Pts',(181.513547598479,503.830923569071,-37.3922967264089)) ;
#57515=CARTESIAN_POINT('Ctrl Pts',(181.499764589189,503.835264274287,-37.4522468079656)) ;
#57516=CARTESIAN_POINT('Ctrl Pts',(181.482603360873,503.839669629951,-37.5115058139305)) ;
#57517=CARTESIAN_POINT('Ctrl Pts',(181.462191697142,503.844068815616,-37.5696883361893)) ;
#57518=CARTESIAN_POINT('Ctrl Pts',(181.442039499626,503.848412080309,-37.627131261763)) ;
#57519=CARTESIAN_POINT('Ctrl Pts',(181.418719347169,503.852749038788,-37.6835251288724)) ;
#57520=CARTESIAN_POINT('Ctrl Pts',(181.392387562637,503.857032081953,-37.7385193943068)) ;
#57521=CARTESIAN_POINT('Ctrl Pts',(181.366071706209,503.861312534304,-37.7934803936946)) ;
#57522=CARTESIAN_POINT('Ctrl Pts',(181.336747959414,503.865539001473,-37.847043568874)) ;
#57523=CARTESIAN_POINT('Ctrl Pts',(181.304602610932,503.86968777188,-37.8988771403132)) ;
#57524=CARTESIAN_POINT('Ctrl Pts',(181.272464844239,503.873835563761,-37.9506984863057)) ;
#57525=CARTESIAN_POINT('Ctrl Pts',(181.237506788954,503.87790569354,-38.0007910131001)) ;
#57526=CARTESIAN_POINT('Ctrl Pts',(181.199944289675,503.881899267768,-38.048840908492)) ;
#57527=CARTESIAN_POINT('Ctrl Pts',(181.161489538531,503.885987704534,-38.0980321711941)) ;
#57528=CARTESIAN_POINT('Ctrl Pts',(181.120304903677,503.889995932486,-38.1450823750831)) ;
#57529=CARTESIAN_POINT('Ctrl Pts',(181.076655216884,503.893951128991,-38.1896754883366)) ;
#57530=CARTESIAN_POINT('Ctrl Pts',(181.033964008986,503.897819475564,-38.2332894065256)) ;
#57531=CARTESIAN_POINT('Ctrl Pts',(180.988914761083,503.901637447854,-38.2745527568117)) ;
#57532=CARTESIAN_POINT('Ctrl Pts',(180.94178849477,503.905451918346,-38.3131923884192)) ;
#57533=CARTESIAN_POINT('Ctrl Pts',(180.893075149975,503.909394849345,-38.3531332928131)) ;
#57534=CARTESIAN_POINT('Ctrl Pts',(180.842142081548,503.913334469124,-38.3902700821888)) ;
#57535=CARTESIAN_POINT('Ctrl Pts',(180.789339977226,503.917340157934,-38.4243323963118)) ;
#57536=CARTESIAN_POINT('Ctrl Pts',(180.743396128359,503.920825563746,-38.453970491843)) ;
#57537=CARTESIAN_POINT('Ctrl Pts',(180.696036557341,503.924361639824,-38.4812815026592)) ;
#57538=CARTESIAN_POINT('Ctrl Pts',(180.647522868314,503.927999005388,-38.5061118036851)) ;
#57539=CARTESIAN_POINT('Ctrl Pts',(180.640308509786,503.928539909611,-38.5098042603412)) ;
#57540=CARTESIAN_POINT('Ctrl Pts',(180.633068590654,503.929083053748,-38.5134419444454)) ;
#57541=CARTESIAN_POINT('Ctrl Pts',(180.625803928338,503.92962860426,-38.5170244397967)) ;
#57542=CARTESIAN_POINT('Ctrl Pts',(180.625776227412,503.929630684501,-38.5170381002305)) ;
#57543=CARTESIAN_POINT('Ctrl Pts',(180.625748526126,503.929632764778,-38.5170517598619)) ;
#57544=CARTESIAN_POINT('Ctrl Pts',(180.625720824481,503.92963484509,-38.5170654186909)) ;
#57545=CARTESIAN_POINT('Ctrl Pts',(180.575999633131,503.933368759793,-38.5415814082224)) ;
#57546=CARTESIAN_POINT('Ctrl Pts',(180.524937783754,503.937225215228,-38.563592697846)) ;
#57547=CARTESIAN_POINT('Ctrl Pts',(180.472822234143,503.941140992713,-38.582987229563)) ;
#57548=CARTESIAN_POINT('Ctrl Pts',(180.467990408081,503.941504038979,-38.5847853685928)) ;
#57549=CARTESIAN_POINT('Ctrl Pts',(180.463149560691,503.941867595168,-38.586561022526)) ;
#57550=CARTESIAN_POINT('Ctrl Pts',(180.458299942609,503.942231610897,-38.5883141075688)) ;
#57551=CARTESIAN_POINT('Ctrl Pts',(180.40043283571,503.946575156459,-38.6092324474977)) ;
#57552=CARTESIAN_POINT('Ctrl Pts',(180.341311015314,503.950983464914,-38.6269365125238)) ;
#57553=CARTESIAN_POINT('Ctrl Pts',(180.281328632211,503.955385157311,-38.6413236454677)) ;
#57554=CARTESIAN_POINT('Ctrl Pts',(180.222247370112,503.959720722668,-38.6554946391551)) ;
#57555=CARTESIAN_POINT('Ctrl Pts',(180.162331216653,503.96404958664,-38.6664480600204)) ;
#57556=CARTESIAN_POINT('Ctrl Pts',(180.101957983656,503.968324092576,-38.6741248465967)) ;
#57557=CARTESIAN_POINT('Ctrl Pts',(180.041622242767,503.97259594402,-38.6817968658464)) ;
#57558=CARTESIAN_POINT('Ctrl Pts',(179.980829976647,503.976813370938,-38.686196445756)) ;
#57559=CARTESIAN_POINT('Ctrl Pts',(179.919959587964,503.980952576775,-38.6872998714748)) ;
#57560=CARTESIAN_POINT('Ctrl Pts',(179.859104293839,503.985090756178,-38.6884030235676)) ;
#57561=CARTESIAN_POINT('Ctrl Pts',(179.798170937088,503.989150751186,-38.6862116238091)) ;
#57562=CARTESIAN_POINT('Ctrl Pts',(179.737538894785,503.993133537007,-38.6807365485424)) ;
#57563=CARTESIAN_POINT('Ctrl Pts',(179.675211763591,503.997227669498,-38.6751084066972)) ;
#57564=CARTESIAN_POINT('Ctrl Pts',(179.613203102409,504.001240224082,-38.6660100621272)) ;
#57565=CARTESIAN_POINT('Ctrl Pts',(179.551925650776,504.005198583097,-38.6534930410653)) ;
#57566=CARTESIAN_POINT('Ctrl Pts',(179.49223897753,504.009054182095,-38.6413009650862)) ;
#57567=CARTESIAN_POINT('Ctrl Pts',(179.433246182249,504.012858731079,-38.6258652821553)) ;
#57568=CARTESIAN_POINT('Ctrl Pts',(179.375327730127,504.016659006697,-38.6072738104232)) ;
#57569=CARTESIAN_POINT('Ctrl Pts',(179.315093800773,504.02061121061,-38.5879390845484)) ;
#57570=CARTESIAN_POINT('Ctrl Pts',(179.256022189819,504.024559211105,-38.5651903779576)) ;
#57571=CARTESIAN_POINT('Ctrl Pts',(179.198536157218,504.02857361947,-38.5391783218387)) ;
#57572=CARTESIAN_POINT('Ctrl Pts',(179.14880772746,504.032046293012,-38.5166765305859)) ;
#57573=CARTESIAN_POINT('Ctrl Pts',(179.100264884407,504.035569318995,-38.4917324825779)) ;
#57574=CARTESIAN_POINT('Ctrl Pts',(179.0531776563,504.039193368418,-38.4644828027308)) ;
#57575=CARTESIAN_POINT('Ctrl Pts',(179.045858000477,504.039756722761,-38.4602468711253)) ;
#57576=CARTESIAN_POINT('Ctrl Pts',(179.038573417292,504.04032251827,-38.4559552409651)) ;
#57577=CARTESIAN_POINT('Ctrl Pts',(179.031324808433,504.040890945281,-38.4516084395122)) ;
#57578=CARTESIAN_POINT('Ctrl Pts',(179.031299138759,504.040892958265,-38.451593046079)) ;
#57579=CARTESIAN_POINT('Ctrl Pts',(179.031273469536,504.040894971282,-38.4515776519539)) ;
#57580=CARTESIAN_POINT('Ctrl Pts',(179.031247800765,504.040896984333,-38.4515622571369)) ;
#57581=CARTESIAN_POINT('Ctrl Pts',(178.983709945429,504.044625097892,-38.4230514819521)) ;
#57582=CARTESIAN_POINT('Ctrl Pts',(178.937552118394,504.048476294638,-38.3920576524867)) ;
#57583=CARTESIAN_POINT('Ctrl Pts',(178.893023657722,504.052387432178,-38.3587614226577)) ;
#57584=CARTESIAN_POINT('Ctrl Pts',(178.888860064263,504.052753139558,-38.3556480887891)) ;
#57585=CARTESIAN_POINT('Ctrl Pts',(178.884710729245,504.053119371001,-38.3525146603628)) ;
#57586=CARTESIAN_POINT('Ctrl Pts',(178.880575863895,504.053486074888,-38.3493613070806)) ;
#57587=CARTESIAN_POINT('Ctrl Pts',(178.831649049199,504.05782518913,-38.3120484761493)) ;
#57588=CARTESIAN_POINT('Ctrl Pts',(178.784745748647,504.06222978468,-38.2719403856926)) ;
#57589=CARTESIAN_POINT('Ctrl Pts',(178.740165376907,504.066628466276,-38.2293129576102)) ;
#57590=CARTESIAN_POINT('Ctrl Pts',(178.696226804807,504.070963822419,-38.1872992136885)) ;
#57591=CARTESIAN_POINT('Ctrl Pts',(178.654544388054,504.075293146648,-38.1428383973493)) ;
#57592=CARTESIAN_POINT('Ctrl Pts',(178.615372496037,504.07956861893,-38.0962167323261)) ;
#57593=CARTESIAN_POINT('Ctrl Pts',(178.576224659597,504.083841465632,-38.0496236978077)) ;
#57594=CARTESIAN_POINT('Ctrl Pts',(178.539584148741,504.088060391233,-38.0008725250665)) ;
#57595=CARTESIAN_POINT('Ctrl Pts',(178.50567587558,504.092201451286,-37.950269012115)) ;
#57596=CARTESIAN_POINT('Ctrl Pts',(178.471775817483,504.096341508071,-37.8996777590359)) ;
#57597=CARTESIAN_POINT('Ctrl Pts',(178.440606709769,504.100403734332,-37.8472350625964)) ;
#57598=CARTESIAN_POINT('Ctrl Pts',(178.412364887662,504.104388987196,-37.7932662174788)) ;
#57599=CARTESIAN_POINT('Ctrl Pts',(178.38336594261,504.108481079002,-37.7378505446471)) ;
#57600=CARTESIAN_POINT('Ctrl Pts',(178.357453670579,504.112492027932,-37.6808256691424)) ;
#57601=CARTESIAN_POINT('Ctrl Pts',(178.33480771692,504.116449022292,-37.622565670781)) ;
#57602=CARTESIAN_POINT('Ctrl Pts',(178.312724852657,504.120307626379,-37.5657543015131)) ;
#57603=CARTESIAN_POINT('Ctrl Pts',(178.293748080204,504.124115289283,-37.5077685123963)) ;
#57604=CARTESIAN_POINT('Ctrl Pts',(178.27800969468,504.127918723497,-37.4489760990798)) ;
#57605=CARTESIAN_POINT('Ctrl Pts',(178.261669341185,504.131867632962,-37.3879349703697)) ;
#57606=CARTESIAN_POINT('Ctrl Pts',(178.248820705576,504.135812404332,-37.3260241937824)) ;
#57607=CARTESIAN_POINT('Ctrl Pts',(178.23956602147,504.139823266144,-37.2636794060451)) ;
#57608=CARTESIAN_POINT('Ctrl Pts',(178.231544361973,504.14329975085,-37.2096409696274)) ;
#57609=CARTESIAN_POINT('Ctrl Pts',(178.22622250326,504.146826543878,-37.1552755703853)) ;
#57610=CARTESIAN_POINT('Ctrl Pts',(178.223631999662,504.15045438272,-37.1008847160766)) ;
#57611=CARTESIAN_POINT('Ctrl Pts',(178.223235216675,504.151010052563,-37.0925537623512)) ;
#57612=CARTESIAN_POINT('Ctrl Pts',(178.222902446833,504.151568092995,-37.0842221367079)) ;
#57613=CARTESIAN_POINT('Ctrl Pts',(178.222633734156,504.152128686334,-37.0758908393388)) ;
#57614=CARTESIAN_POINT('Ctrl Pts',(178.222632780434,504.152130676006,-37.0758612696975)) ;
#57615=CARTESIAN_POINT('Ctrl Pts',(178.22263182752,504.152132665709,-37.0758317000604)) ;
#57616=CARTESIAN_POINT('Ctrl Pts',(178.222630875412,504.152134655445,-37.0758021304273)) ;
#57617=CARTESIAN_POINT('Ctrl Pts',(178.220846087648,504.155864544243,-37.0203719331003)) ;
#57618=CARTESIAN_POINT('Ctrl Pts',(178.221898634255,504.159717283414,-36.9647570884874)) ;
#57619=CARTESIAN_POINT('Ctrl Pts',(178.225771600282,504.163629724937,-36.909265371742)) ;
#57620=CARTESIAN_POINT('Ctrl Pts',(178.226132585354,504.163994389377,-36.9040931907217)) ;
#57621=CARTESIAN_POINT('Ctrl Pts',(178.226518050009,504.164359572476,-36.8989221091583)) ;
#57622=CARTESIAN_POINT('Ctrl Pts',(178.2269279662,504.164725223103,-36.893752394232)) ;
#57623=CARTESIAN_POINT('Ctrl Pts',(178.231791448608,504.169063513302,-36.8324159108179)) ;
#57624=CARTESIAN_POINT('Ctrl Pts',(178.240100224105,504.173466950864,-36.7712667789477)) ;
#57625=CARTESIAN_POINT('Ctrl Pts',(178.251784480751,504.177864274275,-36.710705959758)) ;
#57626=CARTESIAN_POINT('Ctrl Pts',(178.263303322816,504.182199344568,-36.6510025029893)) ;
#57627=CARTESIAN_POINT('Ctrl Pts',(178.278102341194,504.18652818541,-36.5918706425448)) ;
#57628=CARTESIAN_POINT('Ctrl Pts',(178.296078632547,504.190803066331,-36.5336793420849)) ;
#57629=CARTESIAN_POINT('Ctrl Pts',(178.314043956525,504.195075339138,-36.4755235442623)) ;
#57630=CARTESIAN_POINT('Ctrl Pts',(178.335182566682,504.199293582935,-36.4183070920453)) ;
#57631=CARTESIAN_POINT('Ctrl Pts',(178.359359152784,504.203433949214,-36.3623847921564)) ;
#57632=CARTESIAN_POINT('Ctrl Pts',(178.383529968864,504.207573327346,-36.3064758387721)) ;
#57633=CARTESIAN_POINT('Ctrl Pts',(178.410737331575,504.211634862792,-36.2518604502738)) ;
#57634=CARTESIAN_POINT('Ctrl Pts',(178.440814060322,504.215619510201,-36.1988799748682)) ;
#57635=CARTESIAN_POINT('Ctrl Pts',(178.471683800588,504.219709217948,-36.1445026012948)) ;
#57636=CARTESIAN_POINT('Ctrl Pts',(178.50557649632,504.223717945013,-36.0918476971024)) ;
#57637=CARTESIAN_POINT('Ctrl Pts',(178.542275190797,504.227672939551,-36.041268561789)) ;
#57638=CARTESIAN_POINT('Ctrl Pts',(178.578077018835,504.231531279374,-35.9919255121081)) ;
#57639=CARTESIAN_POINT('Ctrl Pts',(178.616549439427,504.235338843381,-35.9445581959155)) ;
#57640=CARTESIAN_POINT('Ctrl Pts',(178.65745484286,504.239142415311,-35.8994771634488)) ;
#57641=CARTESIAN_POINT('Ctrl Pts',(178.69989731935,504.243088911341,-35.8527021533026)) ;
#57642=CARTESIAN_POINT('Ctrl Pts',(178.744959640762,504.2470315321,-35.808389125236)) ;
#57643=CARTESIAN_POINT('Ctrl Pts',(178.792331462551,504.251040416332,-35.7668594981143)) ;
#57644=CARTESIAN_POINT('Ctrl Pts',(178.833406729212,504.254516448764,-35.7308498948544)) ;
#57645=CARTESIAN_POINT('Ctrl Pts',(178.876218948242,504.258042955032,-35.696932219074)) ;
#57646=CARTESIAN_POINT('Ctrl Pts',(178.92053188491,504.261670629236,-35.6652962359978)) ;
#57647=CARTESIAN_POINT('Ctrl Pts',(178.927300464559,504.262224738344,-35.6604639976644)) ;
#57648=CARTESIAN_POINT('Ctrl Pts',(178.934104084428,504.262781207804,-35.6556848982313)) ;
#57649=CARTESIAN_POINT('Ctrl Pts',(178.940941934694,504.263340218276,-35.6509595114309)) ;
#57650=CARTESIAN_POINT('Ctrl Pts',(178.940966471226,504.263342224195,-35.6509425551364)) ;
#57651=CARTESIAN_POINT('Ctrl Pts',(178.940991008198,504.263344230148,-35.6509255995334)) ;
#57652=CARTESIAN_POINT('Ctrl Pts',(178.941015545612,504.263346236133,-35.650908644622)) ;
#57653=CARTESIAN_POINT('Ctrl Pts',(178.986944662912,504.267101037983,-35.6191724502927)) ;
#57654=CARTESIAN_POINT('Ctrl Pts',(179.034583862883,504.2709801353,-35.5897545977169)) ;
#57655=CARTESIAN_POINT('Ctrl Pts',(179.083663645032,504.274919333971,-35.5628072016248)) ;
#57656=CARTESIAN_POINT('Ctrl Pts',(179.088570639873,504.275313174911,-35.5601130019402)) ;
#57657=CARTESIAN_POINT('Ctrl Pts',(179.09349199182,504.275707616624,-35.5574434950931)) ;
#57658=CARTESIAN_POINT('Ctrl Pts',(179.098427403031,504.276102594954,-35.5547988311475)) ;
#57659=CARTESIAN_POINT('Ctrl Pts',(179.152635977017,504.280440878255,-35.5257509048351)) ;
#57660=CARTESIAN_POINT('Ctrl Pts',(179.208546689207,504.284843266207,-35.499699719582)) ;
#57661=CARTESIAN_POINT('Ctrl Pts',(179.265791140492,504.289239112474,-35.4768014184793)) ;
#57662=CARTESIAN_POINT('Ctrl Pts',(179.322947672265,504.293628207333,-35.4539382859812)) ;
#57663=CARTESIAN_POINT('Ctrl Pts',(179.381433839323,504.298010444336,-35.4342179835861)) ;
#57664=CARTESIAN_POINT('Ctrl Pts',(179.440876471456,504.302336984258,-35.4177585037803)) ;
#57665=CARTESIAN_POINT('Ctrl Pts',(179.500265672515,504.306659635192,-35.4013138188721)) ;
#57666=CARTESIAN_POINT('Ctrl Pts',(179.560609664863,504.310926549102,-35.388123959882)) ;
#57667=CARTESIAN_POINT('Ctrl Pts',(179.621529458883,504.315113966885,-35.3782729958669)) ;
#57668=CARTESIAN_POINT('Ctrl Pts',(179.682417740684,504.319299218626,-35.3684271274981)) ;
#57669=CARTESIAN_POINT('Ctrl Pts',(179.743881263251,504.323405051185,-35.3619167450483)) ;
#57670=CARTESIAN_POINT('Ctrl Pts',(179.805534178045,504.327433730372,-35.3587928477403)) ;
#57671=CARTESIAN_POINT('Ctrl Pts',(179.833460793808,504.32925858125,-35.3573778314333)) ;
#57672=CARTESIAN_POINT('Ctrl Pts',(179.861426164107,504.331067955713,-35.3566571930793)) ;
#57673=CARTESIAN_POINT('Ctrl Pts',(179.889393904536,504.332863786117,-35.3566333596088)) ;
#57674=CARTESIAN_POINT('Ctrl Pts',(179.889376469388,504.333136041102,-35.356160388007)) ;
#57675=CARTESIAN_POINT('Ctrl Pts',(179.962317757491,504.3377604451,-35.3561975523419)) ;
#57676=CARTESIAN_POINT('Ctrl Pts',(180.035181643089,504.342252983734,-35.3610248634196)) ;
#57677=CARTESIAN_POINT('Ctrl Pts',(180.211581870764,504.353134911495,-35.3844131273454)) ;
#57678=CARTESIAN_POINT('Ctrl Pts',(180.314114978436,504.359460830589,-35.4080194385543)) ;
#57679=CARTESIAN_POINT('Ctrl Pts',(180.430608289387,504.367296800496,-35.4467171416852)) ;
#57680=CARTESIAN_POINT('Ctrl Pts',(180.447390450651,504.36844237917,-35.4525919563438)) ;
#57681=CARTESIAN_POINT('Ctrl Pts',(180.464073435314,504.369601015799,-35.4587334799406)) ;
#57682=CARTESIAN_POINT('Origin',(179.888527625422,620.256490441073,-37.0221601717597)) ;
#57683=CARTESIAN_POINT('',(181.517739097406,616.918146095397,-35.7700948611419)) ;
#57684=CARTESIAN_POINT('',(181.517739074368,616.85992786049,-35.7700948311641)) ;
#57685=CARTESIAN_POINT('',(181.517739089189,620.256490441073,-35.7700948504488)) ;
#57686=CARTESIAN_POINT('',(179.065295445318,616.710565160536,-35.1395326620963)) ;
#57687=CARTESIAN_POINT('Ctrl Pts',(181.517739074368,616.85992786049,-35.7700948311641)) ;
#57688=CARTESIAN_POINT('Ctrl Pts',(181.506609107836,616.858866348378,-35.7556123051225)) ;
#57689=CARTESIAN_POINT('Ctrl Pts',(181.495285009743,616.857799228944,-35.741276854028)) ;
#57690=CARTESIAN_POINT('Ctrl Pts',(181.39714883938,616.848663946389,-35.6203944242632)) ;
#57691=CARTESIAN_POINT('Ctrl Pts',(181.300047612677,616.840327777811,-35.5226622490848)) ;
#57692=CARTESIAN_POINT('Ctrl Pts',(181.155040681315,616.829340879517,-35.4033714355429)) ;
#57693=CARTESIAN_POINT('Ctrl Pts',(181.114994883078,616.826441830741,-35.3728236061938)) ;
#57694=CARTESIAN_POINT('Ctrl Pts',(181.049444651431,616.82195796045,-35.3265296152158)) ;
#57695=CARTESIAN_POINT('Ctrl Pts',(181.024650646624,616.820319711129,-35.3098178704186)) ;
#57696=CARTESIAN_POINT('Ctrl Pts',(180.964094489759,616.816462006346,-35.270896475894)) ;
#57697=CARTESIAN_POINT('Ctrl Pts',(180.927999232584,616.814274192439,-35.2492338086848)) ;
#57698=CARTESIAN_POINT('Ctrl Pts',(180.794503903944,616.806491824449,-35.1745960578176)) ;
#57699=CARTESIAN_POINT('Ctrl Pts',(180.693519165775,616.801177658522,-35.1284129259982)) ;
#57700=CARTESIAN_POINT('Ctrl Pts',(180.468180350198,616.789637118546,-35.0466602879336)) ;
#57701=CARTESIAN_POINT('Ctrl Pts',(180.343212053813,616.783417505349,-35.0142120406523)) ;
#57702=CARTESIAN_POINT('Ctrl Pts',(180.157277050943,616.773810250216,-34.9841921653847)) ;
#57703=CARTESIAN_POINT('Ctrl Pts',(180.098140669292,616.770707818637,-34.9772637601659)) ;
#57704=CARTESIAN_POINT('Ctrl Pts',(179.983239558847,616.764551176367,-34.9688385471496)) ;
#57705=CARTESIAN_POINT('Ctrl Pts',(179.92755007429,616.761509321861,-34.9670259885493)) ;
#57706=CARTESIAN_POINT('Ctrl Pts',(179.813152576433,616.755131963,-34.9679540391312)) ;
#57707=CARTESIAN_POINT('Ctrl Pts',(179.754497305784,616.751792334337,-34.9709460657023)) ;
#57708=CARTESIAN_POINT('Ctrl Pts',(179.511442039914,616.737693994545,-34.9938142339676)) ;
#57709=CARTESIAN_POINT('Ctrl Pts',(179.330042150489,616.726468516774,-35.0360909204514)) ;
#57710=CARTESIAN_POINT('Ctrl Pts',(179.125992098987,616.714177429145,-35.1138565302351)) ;
#57711=CARTESIAN_POINT('Ctrl Pts',(179.095487977552,616.712351867416,-35.1263301225568)) ;
#57712=CARTESIAN_POINT('Ctrl Pts',(179.065295445318,616.710565160536,-35.1395326620961)) ;
#57713=CARTESIAN_POINT('',(178.234449048513,616.711852647397,-35.799415550035)) ;
#57714=CARTESIAN_POINT('Origin',(179.888527625422,616.710565160536,-37.0221601717597)) ;
#57715=CARTESIAN_POINT('Ctrl Pts',(178.236389517568,616.713140134259,-35.8005066877149)) ;
#57716=CARTESIAN_POINT('Ctrl Pts',(178.246281071676,616.714039061134,-35.7871295609758)) ;
#57717=CARTESIAN_POINT('Ctrl Pts',(178.25633508351,616.714927007289,-35.773872585346)) ;
#57718=CARTESIAN_POINT('Ctrl Pts',(178.280148287692,616.716974845351,-35.743252763817)) ;
#57719=CARTESIAN_POINT('Ctrl Pts',(178.294029590926,616.718127209171,-35.7259872121017)) ;
#57720=CARTESIAN_POINT('Ctrl Pts',(178.386281286779,616.725546033727,-35.6149700240209)) ;
#57721=CARTESIAN_POINT('Ctrl Pts',(178.47260906756,616.731403820701,-35.5281360333275)) ;
#57722=CARTESIAN_POINT('Ctrl Pts',(178.657151287698,616.743100547166,-35.3729644679706)) ;
#57723=CARTESIAN_POINT('Ctrl Pts',(178.754617781303,616.748917689103,-35.3044933824928)) ;
#57724=CARTESIAN_POINT('Ctrl Pts',(178.903393629093,616.757792529321,-35.2181840499202)) ;
#57725=CARTESIAN_POINT('Ctrl Pts',(178.950350783986,616.760590155878,-35.1933238278685)) ;
#57726=CARTESIAN_POINT('Ctrl Pts',(179.045990364134,616.766311283977,-35.1473432456521)) ;
#57727=CARTESIAN_POINT('Ctrl Pts',(179.09463247113,616.76923234295,-35.1262336713056)) ;
#57728=CARTESIAN_POINT('Ctrl Pts',(179.247680335172,616.778473618264,-35.0667373362296)) ;
#57729=CARTESIAN_POINT('Ctrl Pts',(179.35441431837,616.785000864595,-35.0349306516471)) ;
#57730=CARTESIAN_POINT('Ctrl Pts',(179.556339881529,616.797329737497,-34.9922056682046)) ;
#57731=CARTESIAN_POINT('Ctrl Pts',(179.650752835576,616.803082489123,-34.9789941339355)) ;
#57732=CARTESIAN_POINT('Ctrl Pts',(179.787019112059,616.811142508186,-34.9695019825114)) ;
#57733=CARTESIAN_POINT('Ctrl Pts',(179.828375835261,616.813555838922,-34.9678739828228)) ;
#57734=CARTESIAN_POINT('Ctrl Pts',(179.904154121519,616.817886019535,-34.967181646926)) ;
#57735=CARTESIAN_POINT('Ctrl Pts',(179.938557529514,616.81981724856,-34.9677312374899)) ;
#57736=CARTESIAN_POINT('Ctrl Pts',(180.003949330139,616.823401331865,-34.9704196844264)) ;
#57737=CARTESIAN_POINT('Ctrl Pts',(180.034932991873,616.825060691311,-34.9723975660884)) ;
#57738=CARTESIAN_POINT('Ctrl Pts',(180.137813650187,616.830473422,-34.9813098338369)) ;
#57739=CARTESIAN_POINT('Ctrl Pts',(180.209394385912,616.83408306858,-34.9913327653996)) ;
#57740=CARTESIAN_POINT('Ctrl Pts',(180.444109653757,616.845813294523,-35.0369219662064)) ;
#57741=CARTESIAN_POINT('Ctrl Pts',(180.603423779144,616.853656347961,-35.0885710813705)) ;
#57742=CARTESIAN_POINT('Ctrl Pts',(180.809038231136,616.865140915143,-35.1841604138706)) ;
#57743=CARTESIAN_POINT('Ctrl Pts',(180.862201693352,616.868239308291,-35.2117622080527)) ;
#57744=CARTESIAN_POINT('Ctrl Pts',(180.957293248508,616.874070777027,-35.2665336812578)) ;
#57745=CARTESIAN_POINT('Ctrl Pts',(180.999581890234,616.876776150802,-35.2929863389798)) ;
#57746=CARTESIAN_POINT('Ctrl Pts',(181.101309196086,616.883583339896,-35.36189261198)) ;
#57747=CARTESIAN_POINT('Ctrl Pts',(181.159523288404,616.887747072433,-35.40602412492)) ;
#57748=CARTESIAN_POINT('Ctrl Pts',(181.327103008902,616.900548417978,-35.5477277959752)) ;
#57749=CARTESIAN_POINT('Ctrl Pts',(181.428501854798,616.909465413451,-35.6539776441301)) ;
#57750=CARTESIAN_POINT('Ctrl Pts',(181.517739097406,616.918146095397,-35.7700948611417)) ;
#57751=CARTESIAN_POINT('Origin',(179.888527625422,620.256490441073,-37.0221601717597)) ;
#57752=CARTESIAN_POINT('',(181.517739089193,617.617803659368,-35.7700948504542)) ;
#57753=CARTESIAN_POINT('',(181.517739089189,617.559637408341,-35.7700948504488)) ;
#57754=CARTESIAN_POINT('',(181.517739089189,620.256490441073,-35.7700948504488)) ;
#57755=CARTESIAN_POINT('',(179.887993154238,617.107857237813,-39.0769101022477)) ;
#57756=CARTESIAN_POINT('Ctrl Pts',(181.517739089189,617.559637408341,-35.7700948504488)) ;
#57757=CARTESIAN_POINT('Ctrl Pts',(181.502586585041,617.55838496062,-35.7503781207849)) ;
#57758=CARTESIAN_POINT('Ctrl Pts',(181.48707049028,617.557121165613,-35.7309290693371)) ;
#57759=CARTESIAN_POINT('Ctrl Pts',(181.436305398982,617.553037290777,-35.6696163119889)) ;
#57760=CARTESIAN_POINT('Ctrl Pts',(181.399746698261,617.550170829413,-35.6288880856673)) ;
#57761=CARTESIAN_POINT('Ctrl Pts',(181.325493689432,617.544453120502,-35.5525310944956)) ;
#57762=CARTESIAN_POINT('Ctrl Pts',(181.287989926459,617.541611310833,-35.5167746163965)) ;
#57763=CARTESIAN_POINT('Ctrl Pts',(181.177330663977,617.533335783561,-35.4189828374422)) ;
#57764=CARTESIAN_POINT('Ctrl Pts',(181.101136387809,617.527758860662,-35.3606045772991)) ;
#57765=CARTESIAN_POINT('Ctrl Pts',(180.906988104656,617.513927774877,-35.2323394139)) ;
#57766=CARTESIAN_POINT('Ctrl Pts',(180.785577864741,617.505568757037,-35.1685096301611)) ;
#57767=CARTESIAN_POINT('Ctrl Pts',(180.615481219117,617.494837194308,-35.0997367396894)) ;
#57768=CARTESIAN_POINT('Ctrl Pts',(180.571650207537,617.492156157517,-35.0837284404162)) ;
#57769=CARTESIAN_POINT('Ctrl Pts',(180.499593955378,617.487926256182,-35.0601597089916)) ;
#57770=CARTESIAN_POINT('Ctrl Pts',(180.471689702302,617.486332214729,-35.0516855779554)) ;
#57771=CARTESIAN_POINT('Ctrl Pts',(180.401718114024,617.482444319193,-35.0320531077093)) ;
#57772=CARTESIAN_POINT('Ctrl Pts',(180.359460892321,617.480188632512,-35.021631990952)) ;
#57773=CARTESIAN_POINT('Ctrl Pts',(180.258835714518,617.474966558407,-35.0001823398716)) ;
#57774=CARTESIAN_POINT('Ctrl Pts',(180.200257315445,617.472042845602,-34.9903265749881)) ;
#57775=CARTESIAN_POINT('Ctrl Pts',(179.973804732676,617.460923544124,-34.9622519189994)) ;
#57776=CARTESIAN_POINT('Ctrl Pts',(179.804369589251,617.45292613096,-34.9622063400165)) ;
#57777=CARTESIAN_POINT('Ctrl Pts',(179.583141569119,617.441467885864,-34.9895106669195)) ;
#57778=CARTESIAN_POINT('Ctrl Pts',(179.529732889551,617.438628030699,-34.9982554623742)) ;
#57779=CARTESIAN_POINT('Ctrl Pts',(179.425547790386,617.43291024879,-35.0195676161912)) ;
#57780=CARTESIAN_POINT('Ctrl Pts',(179.374782905162,617.430039126328,-35.0319860777773)) ;
#57781=CARTESIAN_POINT('Ctrl Pts',(179.225930602873,617.421349339453,-35.074474157384)) ;
#57782=CARTESIAN_POINT('Ctrl Pts',(179.129569871467,617.415359318058,-35.1099640084541)) ;
#57783=CARTESIAN_POINT('Ctrl Pts',(178.913668042379,617.401211382308,-35.208379310482)) ;
#57784=CARTESIAN_POINT('Ctrl Pts',(178.796860832817,617.392988049764,-35.2761886918068)) ;
#57785=CARTESIAN_POINT('Ctrl Pts',(178.652736433403,617.382655276666,-35.3800101413563)) ;
#57786=CARTESIAN_POINT('Ctrl Pts',(178.618731176535,617.380204483273,-35.4061607562826)) ;
#57787=CARTESIAN_POINT('Ctrl Pts',(178.562969642741,617.376198015675,-35.4518902364823)) ;
#57788=CARTESIAN_POINT('Ctrl Pts',(178.540772050863,617.374608824275,-35.4709004560454)) ;
#57789=CARTESIAN_POINT('Ctrl Pts',(178.48346343048,617.370514785968,-35.5221393584425)) ;
#57790=CARTESIAN_POINT('Ctrl Pts',(178.449055899489,617.368061368419,-35.555125866284)) ;
#57791=CARTESIAN_POINT('Ctrl Pts',(178.367703064376,617.362181236546,-35.6387397730613)) ;
#57792=CARTESIAN_POINT('Ctrl Pts',(178.322101522062,617.358813994491,-35.6905935922773)) ;
#57793=CARTESIAN_POINT('Ctrl Pts',(178.184923953435,617.348112886578,-35.863401454723)) ;
#57794=CARTESIAN_POINT('Ctrl Pts',(178.104095651772,617.340851873848,-35.9922153202804)) ;
#57795=CARTESIAN_POINT('Ctrl Pts',(178.014722026189,617.330280878681,-36.1773173992612)) ;
#57796=CARTESIAN_POINT('Ctrl Pts',(177.993193309615,617.32744851166,-36.2267899102247)) ;
#57797=CARTESIAN_POINT('Ctrl Pts',(177.954682671024,617.321736369837,-36.3257599657668)) ;
#57798=CARTESIAN_POINT('Ctrl Pts',(177.937595561359,617.318862922739,-36.3751725948307)) ;
#57799=CARTESIAN_POINT('Ctrl Pts',(177.89237840864,617.310122572018,-36.5240923650791)) ;
#57800=CARTESIAN_POINT('Ctrl Pts',(177.869855803236,617.304080325146,-36.6251178418996)) ;
#57801=CARTESIAN_POINT('Ctrl Pts',(177.835704709839,617.289874665742,-36.8607182836646)) ;
#57802=CARTESIAN_POINT('Ctrl Pts',(177.829537230187,617.281649080268,-36.9956152099634)) ;
#57803=CARTESIAN_POINT('Ctrl Pts',(177.83885503347,617.271335960438,-37.1726698259194)) ;
#57804=CARTESIAN_POINT('Ctrl Pts',(177.842414513726,617.268902649459,-37.215117567384)) ;
#57805=CARTESIAN_POINT('Ctrl Pts',(177.850628220982,617.264917443303,-37.2863818727768)) ;
#57806=CARTESIAN_POINT('Ctrl Pts',(177.854580792064,617.263332645549,-37.3152600224801)) ;
#57807=CARTESIAN_POINT('Ctrl Pts',(177.866599212484,617.259247174458,-37.3910312637793)) ;
#57808=CARTESIAN_POINT('Ctrl Pts',(177.87568104503,617.256797951674,-37.4377437402562)) ;
#57809=CARTESIAN_POINT('Ctrl Pts',(177.901856227057,617.250930052497,-37.5511923359043)) ;
#57810=CARTESIAN_POINT('Ctrl Pts',(177.920698726028,617.247570693924,-37.6174656764953)) ;
#57811=CARTESIAN_POINT('Ctrl Pts',(177.991623658939,617.236871778689,-37.8263922486861)) ;
#57812=CARTESIAN_POINT('Ctrl Pts',(178.056181857435,617.229606466954,-37.9642533268478)) ;
#57813=CARTESIAN_POINT('Ctrl Pts',(178.163348689015,617.21903941333,-38.1395864694115)) ;
#57814=CARTESIAN_POINT('Ctrl Pts',(178.193152007248,617.216218448627,-38.1843067631357)) ;
#57815=CARTESIAN_POINT('Ctrl Pts',(178.25514324928,617.210536265199,-38.2698580442139)) ;
#57816=CARTESIAN_POINT('Ctrl Pts',(178.287195954441,617.207681646063,-38.3107371694879)) ;
#57817=CARTESIAN_POINT('Ctrl Pts',(178.385731225683,617.199121661689,-38.4270455827215)) ;
#57818=CARTESIAN_POINT('Ctrl Pts',(178.456233181178,617.193252179432,-38.4988552214778)) ;
#57819=CARTESIAN_POINT('Ctrl Pts',(178.634009548446,617.17912993173,-38.6551768238592)) ;
#57820=CARTESIAN_POINT('Ctrl Pts',(178.745013702691,617.170795664895,-38.7347415664399)) ;
#57821=CARTESIAN_POINT('Ctrl Pts',(178.90137574635,617.160263973947,-38.8247921923812)) ;
#57822=CARTESIAN_POINT('Ctrl Pts',(178.940380988712,617.157729746914,-38.8456100819122)) ;
#57823=CARTESIAN_POINT('Ctrl Pts',(179.006275570121,617.153637511541,-38.8780925730419)) ;
#57824=CARTESIAN_POINT('Ctrl Pts',(179.03279211868,617.152042008275,-38.8904670711412)) ;
#57825=CARTESIAN_POINT('Ctrl Pts',(179.101975382736,617.148004095038,-38.9209706044151)) ;
#57826=CARTESIAN_POINT('Ctrl Pts',(179.145005717671,617.145608388341,-38.9382293992682)) ;
#57827=CARTESIAN_POINT('Ctrl Pts',(179.250361721806,617.139936310134,-38.976401472423)) ;
#57828=CARTESIAN_POINT('Ctrl Pts',(179.313178811052,617.136712612141,-38.9958089206235)) ;
#57829=CARTESIAN_POINT('Ctrl Pts',(179.4980724366,617.127415336166,-39.0433520007103)) ;
#57830=CARTESIAN_POINT('Ctrl Pts',(179.621914097063,617.121407885486,-39.0633822627132)) ;
#57831=CARTESIAN_POINT('Ctrl Pts',(179.79380202668,617.112726932359,-39.0752660378272)) ;
#57832=CARTESIAN_POINT('Ctrl Pts',(179.84089165485,617.110316209617,-39.0768978504434)) ;
#57833=CARTESIAN_POINT('Ctrl Pts',(179.887993154238,617.107857237813,-39.0769101022477)) ;
#57834=CARTESIAN_POINT('Ctrl Pts',(179.887994300553,617.107857177969,-39.0769101025456)) ;
#57835=CARTESIAN_POINT('Ctrl Pts',(179.931748483178,617.105572954829,-39.076921459253)) ;
#57836=CARTESIAN_POINT('Ctrl Pts',(179.97548999554,617.10324833753,-39.075535261176)) ;
#57837=CARTESIAN_POINT('Ctrl Pts',(180.071561238632,617.098035449014,-39.0694154273536)) ;
#57838=CARTESIAN_POINT('Ctrl Pts',(180.12381888014,617.095129323125,-39.0640692522285)) ;
#57839=CARTESIAN_POINT('Ctrl Pts',(180.342482870469,617.082651282919,-39.0331936076929)) ;
#57840=CARTESIAN_POINT('Ctrl Pts',(180.505609754287,617.072491440771,-38.9892704948936)) ;
#57841=CARTESIAN_POINT('Ctrl Pts',(180.742998106722,617.057100438195,-38.8928847970312)) ;
#57842=CARTESIAN_POINT('Ctrl Pts',(180.822274454612,617.05186350609,-38.8546038648334)) ;
#57843=CARTESIAN_POINT('Ctrl Pts',(180.926988113091,617.045023143873,-38.7954737114887)) ;
#57844=CARTESIAN_POINT('Ctrl Pts',(180.954741046925,617.043218570973,-38.7789272071751)) ;
#57845=CARTESIAN_POINT('Ctrl Pts',(181.010632278967,617.039619800362,-38.7437916482847)) ;
#57846=CARTESIAN_POINT('Ctrl Pts',(181.038725918926,617.037828987409,-38.7251510622714)) ;
#57847=CARTESIAN_POINT('Ctrl Pts',(181.170747514585,617.029437403796,-38.6327942940199)) ;
#57848=CARTESIAN_POINT('Ctrl Pts',(181.268137532102,617.023307596862,-38.550202539998)) ;
#57849=CARTESIAN_POINT('Ctrl Pts',(181.442290554182,617.011209674755,-38.3721984430523)) ;
#57850=CARTESIAN_POINT('Ctrl Pts',(181.51943714825,617.005266341215,-38.2779122576196)) ;
#57851=CARTESIAN_POINT('Ctrl Pts',(181.618062377617,616.996214627546,-38.1328384535756)) ;
#57852=CARTESIAN_POINT('Ctrl Pts',(181.646569915149,616.993378284313,-38.0871405969377)) ;
#57853=CARTESIAN_POINT('Ctrl Pts',(181.699819310156,616.987582234548,-37.9938057004965)) ;
#57854=CARTESIAN_POINT('Ctrl Pts',(181.7245548971,616.984625351876,-37.9462141191694)) ;
#57855=CARTESIAN_POINT('Ctrl Pts',(181.7956346867,616.975227139334,-37.7953057049953)) ;
#57856=CARTESIAN_POINT('Ctrl Pts',(181.835318675884,616.968568838972,-37.6891010116894)) ;
#57857=CARTESIAN_POINT('Ctrl Pts',(181.891898060409,616.95609510919,-37.488594272575)) ;
#57858=CARTESIAN_POINT('Ctrl Pts',(181.911348701779,616.950333216952,-37.3953211495107)) ;
#57859=CARTESIAN_POINT('Ctrl Pts',(181.931962597854,616.941354485208,-37.2448434608005)) ;
#57860=CARTESIAN_POINT('Ctrl Pts',(181.937331067427,616.938055335606,-37.1883522907547)) ;
#57861=CARTESIAN_POINT('Ctrl Pts',(181.941925447787,616.933207546444,-37.1022991223444)) ;
#57862=CARTESIAN_POINT('Ctrl Pts',(181.942863276539,616.931580674787,-37.0728577866721)) ;
#57863=CARTESIAN_POINT('Ctrl Pts',(181.94352433511,616.928130907502,-37.0089203794651)) ;
#57864=CARTESIAN_POINT('Ctrl Pts',(181.943012734418,616.926321035078,-36.9744314866176)) ;
#57865=CARTESIAN_POINT('Ctrl Pts',(181.937111839773,616.918742220634,-36.8270282926864)) ;
#57866=CARTESIAN_POINT('Ctrl Pts',(181.923278371657,616.913349797256,-36.7146404094036)) ;
#57867=CARTESIAN_POINT('Ctrl Pts',(181.87195147715,616.901331556798,-36.4677386305984)) ;
#57868=CARTESIAN_POINT('Ctrl Pts',(181.829877489038,616.894721323105,-36.3347662570377)) ;
#57869=CARTESIAN_POINT('Ctrl Pts',(181.752604770617,616.884830986749,-36.1559531550421)) ;
#57870=CARTESIAN_POINT('Ctrl Pts',(181.728448913669,616.881939946307,-36.1057612086665)) ;
#57871=CARTESIAN_POINT('Ctrl Pts',(181.678827079011,616.876315230185,-36.0125475253731)) ;
#57872=CARTESIAN_POINT('Ctrl Pts',(181.653771474374,616.873598235882,-35.9693528025679)) ;
#57873=CARTESIAN_POINT('Ctrl Pts',(181.593143507417,616.867275496381,-35.8730915803318)) ;
#57874=CARTESIAN_POINT('Ctrl Pts',(181.556626176123,616.86363668831,-35.8206954742303)) ;
#57875=CARTESIAN_POINT('Ctrl Pts',(181.517739074368,616.85992786049,-35.7700948311641)) ;
#57876=CARTESIAN_POINT('Ctrl Pts',(181.517739097406,616.918146095397,-35.7700948611415)) ;
#57877=CARTESIAN_POINT('Ctrl Pts',(181.550328721279,616.921316298233,-35.8125011067506)) ;
#57878=CARTESIAN_POINT('Ctrl Pts',(181.581246855276,616.924445264569,-35.8561583268598)) ;
#57879=CARTESIAN_POINT('Ctrl Pts',(181.625374003287,616.929048745201,-35.9239288915403)) ;
#57880=CARTESIAN_POINT('Ctrl Pts',(181.639855178756,616.930584660759,-35.9471721511206)) ;
#57881=CARTESIAN_POINT('Ctrl Pts',(181.669022937296,616.933721059168,-35.9961430811549)) ;
#57882=CARTESIAN_POINT('Ctrl Pts',(181.683625433427,616.935313808053,-36.0219109388662)) ;
#57883=CARTESIAN_POINT('Ctrl Pts',(181.725712386179,616.939994159661,-36.1000706894596)) ;
#57884=CARTESIAN_POINT('Ctrl Pts',(181.751498255502,616.942989324102,-36.1533457943525)) ;
#57885=CARTESIAN_POINT('Ctrl Pts',(181.828273701453,616.952592025105,-36.3311623217492)) ;
#57886=CARTESIAN_POINT('Ctrl Pts',(181.869341509308,616.958937602289,-36.4596016858192)) ;
#57887=CARTESIAN_POINT('Ctrl Pts',(181.911581610771,616.968819666931,-36.6564866040734)) ;
#57888=CARTESIAN_POINT('Ctrl Pts',(181.922404077584,616.972152671785,-36.7224766318149)) ;
#57889=CARTESIAN_POINT('Ctrl Pts',(181.936140540446,616.978357020819,-36.8426826702027)) ;
#57890=CARTESIAN_POINT('Ctrl Pts',(181.940159278133,616.981193203918,-36.8967103196874)) ;
#57891=CARTESIAN_POINT('Ctrl Pts',(181.943812903979,616.986839931187,-37.0018948196659)) ;
#57892=CARTESIAN_POINT('Ctrl Pts',(181.943681213294,616.989640781737,-37.0530037165148)) ;
#57893=CARTESIAN_POINT('Ctrl Pts',(181.937965970889,616.997669395724,-37.1962917900183)) ;
#57894=CARTESIAN_POINT('Ctrl Pts',(181.928075488364,617.003027668162,-37.2881684388466)) ;
#57895=CARTESIAN_POINT('Ctrl Pts',(181.891815335774,617.015414513837,-37.4937526547962)) ;
#57896=CARTESIAN_POINT('Ctrl Pts',(181.861872978786,617.022495958312,-37.6065127691157)) ;
#57897=CARTESIAN_POINT('Ctrl Pts',(181.807352682194,617.032082323236,-37.7584551703357)) ;
#57898=CARTESIAN_POINT('Ctrl Pts',(181.790778012824,617.034723677821,-37.8002757302703)) ;
#57899=CARTESIAN_POINT('Ctrl Pts',(181.75835588775,617.039398589554,-37.8748381738567)) ;
#57900=CARTESIAN_POINT('Ctrl Pts',(181.74298624706,617.041450542541,-37.9077679224054)) ;
#57901=CARTESIAN_POINT('Ctrl Pts',(181.713350732643,617.045101232571,-37.9671032943191)) ;
#57902=CARTESIAN_POINT('Ctrl Pts',(181.699365616808,617.046713767382,-37.9936346613234)) ;
#57903=CARTESIAN_POINT('Ctrl Pts',(181.655548903705,617.051471129102,-38.0725237332439)) ;
#57904=CARTESIAN_POINT('Ctrl Pts',(181.623988462496,617.054520402284,-38.1238882091899)) ;
#57905=CARTESIAN_POINT('Ctrl Pts',(181.514803487523,617.064177585205,-38.2852228144751)) ;
#57906=CARTESIAN_POINT('Ctrl Pts',(181.428630086657,617.070534384318,-38.3889767072537)) ;
#57907=CARTESIAN_POINT('Ctrl Pts',(181.285202348625,617.080453946922,-38.5307357513301)) ;
#57908=CARTESIAN_POINT('Ctrl Pts',(181.235196313883,617.083809486818,-38.575538116578)) ;
#57909=CARTESIAN_POINT('Ctrl Pts',(181.141472499279,617.090016628892,-38.6515769026892)) ;
#57910=CARTESIAN_POINT('Ctrl Pts',(181.098552023683,617.092830864496,-38.6836986141816)) ;
#57911=CARTESIAN_POINT('Ctrl Pts',(181.011669320262,617.098505144396,-38.7435685195111)) ;
#57912=CARTESIAN_POINT('Ctrl Pts',(180.967812709095,617.101358936485,-38.7713991426981)) ;
#57913=CARTESIAN_POINT('Ctrl Pts',(180.764235053408,617.114584965928,-38.8900137399832)) ;
#57914=CARTESIAN_POINT('Ctrl Pts',(180.593854302493,617.12569994237,-38.9607759619112)) ;
#57915=CARTESIAN_POINT('Ctrl Pts',(180.339716258798,617.141442511417,-39.0283307669638)) ;
#57916=CARTESIAN_POINT('Ctrl Pts',(180.261920739583,617.146139457245,-39.0442559505548)) ;
#57917=CARTESIAN_POINT('Ctrl Pts',(180.152085707938,617.152437967904,-39.0601826164286)) ;
#57918=CARTESIAN_POINT('Ctrl Pts',(180.120674440741,617.154201376314,-39.06399918876)) ;
#57919=CARTESIAN_POINT('Ctrl Pts',(180.055803867352,617.157748126157,-39.0703645630655)) ;
#57920=CARTESIAN_POINT('Ctrl Pts',(180.022345689361,617.159526796168,-39.0728224026525)) ;
#57921=CARTESIAN_POINT('Ctrl Pts',(179.860120920872,617.167969660526,-39.0807516487854)) ;
#57922=CARTESIAN_POINT('Ctrl Pts',(179.731080963116,617.174146901798,-39.0749201346289)) ;
#57923=CARTESIAN_POINT('Ctrl Pts',(179.488784219288,617.185993759301,-39.0409726421341)) ;
#57924=CARTESIAN_POINT('Ctrl Pts',(179.375709988295,617.19163197621,-39.0152516759678)) ;
#57925=CARTESIAN_POINT('Ctrl Pts',(179.212980670018,617.200381079083,-38.963464160089)) ;
#57926=CARTESIAN_POINT('Ctrl Pts',(179.16124581863,617.203259535436,-38.9446807292251)) ;
#57927=CARTESIAN_POINT('Ctrl Pts',(179.062983908672,617.208951568143,-38.9044704939683)) ;
#57928=CARTESIAN_POINT('Ctrl Pts',(179.016381441385,617.211753400817,-38.8833358608337)) ;
#57929=CARTESIAN_POINT('Ctrl Pts',(178.890154857852,617.219645758608,-38.8203086692027)) ;
#57930=CARTESIAN_POINT('Ctrl Pts',(178.812424763463,617.224856612693,-38.7748967759229)) ;
#57931=CARTESIAN_POINT('Ctrl Pts',(178.638774692763,617.237274261633,-38.6575307720814)) ;
#57932=CARTESIAN_POINT('Ctrl Pts',(178.545672381528,617.244554470164,-38.581986293298)) ;
#57933=CARTESIAN_POINT('Ctrl Pts',(178.42699329747,617.254367707815,-38.4671457367803)) ;
#57934=CARTESIAN_POINT('Ctrl Pts',(178.39536794152,617.25704084133,-38.4344421826375)) ;
#57935=CARTESIAN_POINT('Ctrl Pts',(178.340288451284,617.261764274289,-38.3735644535104)) ;
#57936=CARTESIAN_POINT('Ctrl Pts',(178.316452712281,617.263833496823,-38.3457609079863)) ;
#57937=CARTESIAN_POINT('Ctrl Pts',(178.274480773444,617.267500663887,-38.294067585386)) ;
#57938=CARTESIAN_POINT('Ctrl Pts',(178.256101949607,617.269113165125,-38.2703917847557)) ;
#57939=CARTESIAN_POINT('Ctrl Pts',(178.202693929471,617.27384209283,-38.198392916288)) ;
#57940=CARTESIAN_POINT('Ctrl Pts',(178.16924287227,617.276865347643,-38.1489342417559)) ;
#57941=CARTESIAN_POINT('Ctrl Pts',(178.067393037271,617.286517747301,-37.9832239347606)) ;
#57942=CARTESIAN_POINT('Ctrl Pts',(178.00827069366,617.292890850926,-37.8616905795828)) ;
#57943=CARTESIAN_POINT('Ctrl Pts',(177.938178140203,617.302830009259,-37.6722696361415)) ;
#57944=CARTESIAN_POINT('Ctrl Pts',(177.917979420572,617.306188529697,-37.6082013287826)) ;
#57945=CARTESIAN_POINT('Ctrl Pts',(177.887361106619,617.312399699006,-37.4914178531219)) ;
#57946=CARTESIAN_POINT('Ctrl Pts',(177.875803074765,617.315214936164,-37.4390647065857)) ;
#57947=CARTESIAN_POINT('Ctrl Pts',(177.85709408481,617.32089339154,-37.3351722068065)) ;
#57948=CARTESIAN_POINT('Ctrl Pts',(177.849827592242,617.323750457439,-37.2836945667341)) ;
#57949=CARTESIAN_POINT('Ctrl Pts',(177.825750344344,617.336988634995,-37.0491628894965)) ;
#57950=CARTESIAN_POINT('Ctrl Pts',(177.831600636578,617.348113475758,-36.8646577856199)) ;
#57951=CARTESIAN_POINT('Ctrl Pts',(177.875001283232,617.363881152821,-36.6049837039085)) ;
#57952=CARTESIAN_POINT('Ctrl Pts',(177.892659450038,617.368592317796,-36.5273502126785)) ;
#57953=CARTESIAN_POINT('Ctrl Pts',(177.923569987055,617.374904156855,-36.4205460128189)) ;
#57954=CARTESIAN_POINT('Ctrl Pts',(177.933064938416,617.376667845483,-36.390365775814)) ;
#57955=CARTESIAN_POINT('Ctrl Pts',(177.954013658771,617.380208142601,-36.3287847580082)) ;
#57956=CARTESIAN_POINT('Ctrl Pts',(177.965543906333,617.381980372035,-36.2974204563991)) ;
#57957=CARTESIAN_POINT('Ctrl Pts',(178.025788869192,617.390496766316,-36.1451209349666)) ;
#57958=CARTESIAN_POINT('Ctrl Pts',(178.085176990798,617.396739705751,-36.0287180031394)) ;
#57959=CARTESIAN_POINT('Ctrl Pts',(178.221447380879,617.409025717228,-35.8146595134732)) ;
#57960=CARTESIAN_POINT('Ctrl Pts',(178.296924316347,617.415041127856,-35.716782978665)) ;
#57961=CARTESIAN_POINT('Ctrl Pts',(178.416625919415,617.424129027223,-35.5874835335559)) ;
#57962=CARTESIAN_POINT('Ctrl Pts',(178.454016748612,617.426912338358,-35.5500971448259)) ;
#57963=CARTESIAN_POINT('Ctrl Pts',(178.5314303225,617.432598339232,-35.4784456753361)) ;
#57964=CARTESIAN_POINT('Ctrl Pts',(178.571411863573,617.435498321972,-35.4441953811801)) ;
#57965=CARTESIAN_POINT('Ctrl Pts',(178.742559221263,617.44778745189,-35.3086213109438)) ;
#57966=CARTESIAN_POINT('Ctrl Pts',(178.884410445348,617.457750667779,-35.2218295169491)) ;
#57967=CARTESIAN_POINT('Ctrl Pts',(179.093063813471,617.471527796875,-35.1265616067474)) ;
#57968=CARTESIAN_POINT('Ctrl Pts',(179.152221259439,617.475336158369,-35.102808649532)) ;
#57969=CARTESIAN_POINT('Ctrl Pts',(179.255237150789,617.481707829895,-35.0669109214474)) ;
#57970=CARTESIAN_POINT('Ctrl Pts',(179.298571368106,617.484311967162,-35.0534020130791)) ;
#57971=CARTESIAN_POINT('Ctrl Pts',(179.370234483952,617.488455684473,-35.0336410680502)) ;
#57972=CARTESIAN_POINT('Ctrl Pts',(179.3983069954,617.490036948082,-35.0265349636113)) ;
#57973=CARTESIAN_POINT('Ctrl Pts',(179.469271466407,617.493930359723,-35.010159584666)) ;
#57974=CARTESIAN_POINT('Ctrl Pts',(179.51232564288,617.49620276916,-35.0016664927409)) ;
#57975=CARTESIAN_POINT('Ctrl Pts',(179.689278683189,617.50529705332,-34.9726131001116)) ;
#57976=CARTESIAN_POINT('Ctrl Pts',(179.824787120053,617.511711385577,-34.9639361846214)) ;
#57977=CARTESIAN_POINT('Ctrl Pts',(180.060497655407,617.523197141869,-34.9721598209715)) ;
#57978=CARTESIAN_POINT('Ctrl Pts',(180.160424619279,617.528167077317,-34.9830073038409)) ;
#57979=CARTESIAN_POINT('Ctrl Pts',(180.310169803791,617.536049256118,-35.0104678971105)) ;
#57980=CARTESIAN_POINT('Ctrl Pts',(180.360811777393,617.538790535241,-35.0217514721223)) ;
#57981=CARTESIAN_POINT('Ctrl Pts',(180.462961472524,617.544502227499,-35.0486067082229)) ;
#57982=CARTESIAN_POINT('Ctrl Pts',(180.51439266739,617.547475161923,-35.0643093872556)) ;
#57983=CARTESIAN_POINT('Ctrl Pts',(180.725161334104,617.560086329988,-35.1378139503805)) ;
#57984=CARTESIAN_POINT('Ctrl Pts',(180.877638419302,617.570319822621,-35.2131939400467)) ;
#57985=CARTESIAN_POINT('Ctrl Pts',(181.089730278994,617.585552146686,-35.3529496062667)) ;
#57986=CARTESIAN_POINT('Ctrl Pts',(181.157423117762,617.590576635154,-35.403809668987)) ;
#57987=CARTESIAN_POINT('Ctrl Pts',(181.246109728965,617.597199768885,-35.4794386347682)) ;
#57988=CARTESIAN_POINT('Ctrl Pts',(181.269941834904,617.598983521114,-35.5007417472021)) ;
#57989=CARTESIAN_POINT('Ctrl Pts',(181.317382422261,617.602524754099,-35.5451824379964)) ;
#57990=CARTESIAN_POINT('Ctrl Pts',(181.340948958807,617.604279378033,-35.568350759617)) ;
#57991=CARTESIAN_POINT('Ctrl Pts',(181.418564822408,617.610084953589,-35.6484273383273)) ;
#57992=CARTESIAN_POINT('Ctrl Pts',(181.469913375323,617.613972930346,-35.7078631122422)) ;
#57993=CARTESIAN_POINT('Ctrl Pts',(181.517739089197,617.617803659368,-35.7700948504595)) ;
#57994=CARTESIAN_POINT('Origin',(179.888527625422,620.256490441073,-37.0221601717597)) ;
#57995=CARTESIAN_POINT('',(181.51728805297,618.315593727817,-35.7705118777721)) ;
#57996=CARTESIAN_POINT('',(181.517739089185,618.256600448669,-35.770094850444)) ;
#57997=CARTESIAN_POINT('',(181.517739089189,620.256490441073,-35.7700948504488)) ;
#57998=CARTESIAN_POINT('',(179.888164616977,618.564640754081,-39.0769101396937)) ;
#57999=CARTESIAN_POINT('Ctrl Pts',(179.888125504502,618.563693523877,-39.0763631698524)) ;
#58000=CARTESIAN_POINT('Ctrl Pts',(179.959056146154,618.559621057654,-39.0762415227883)) ;
#58001=CARTESIAN_POINT('Ctrl Pts',(180.030027539004,618.555603825935,-39.0724738662884)) ;
#58002=CARTESIAN_POINT('Ctrl Pts',(180.100642834529,618.551671173244,-39.0650869459768)) ;
#58003=CARTESIAN_POINT('Ctrl Pts',(180.171240300517,618.547739513502,-39.0577018907762)) ;
#58004=CARTESIAN_POINT('Ctrl Pts',(180.241481827655,618.543892420134,-39.0466994145418)) ;
#58005=CARTESIAN_POINT('Ctrl Pts',(180.310975081654,618.540134620763,-39.0321407020133)) ;
#58006=CARTESIAN_POINT('Ctrl Pts',(180.380474576421,618.536376483926,-39.0175806820547)) ;
#58007=CARTESIAN_POINT('Ctrl Pts',(180.449225593483,618.532707584397,-38.9994636931089)) ;
#58008=CARTESIAN_POINT('Ctrl Pts',(180.516840591467,618.529108370222,-38.9778860130638)) ;
#58009=CARTESIAN_POINT('Ctrl Pts',(180.584533976828,618.525504983408,-38.9562833175963)) ;
#58010=CARTESIAN_POINT('Ctrl Pts',(180.651088576284,618.521971257736,-38.9312116960932)) ;
#58011=CARTESIAN_POINT('Ctrl Pts',(180.71612189975,618.51846514406,-38.9028051720917)) ;
#58012=CARTESIAN_POINT('Ctrl Pts',(180.781195676329,618.514956849453,-38.8743809781904)) ;
#58013=CARTESIAN_POINT('Ctrl Pts',(180.844746048432,618.511475855401,-38.8426174166942)) ;
#58014=CARTESIAN_POINT('Ctrl Pts',(180.90639890197,618.507961534938,-38.8076901049773)) ;
#58015=CARTESIAN_POINT('Ctrl Pts',(180.964471862557,618.504651274634,-38.7747908589512)) ;
#58016=CARTESIAN_POINT('Ctrl Pts',(181.020861449749,618.501310953758,-38.7390842018661)) ;
#58017=CARTESIAN_POINT('Ctrl Pts',(181.075265040859,618.497880064485,-38.7007560774233)) ;
#58018=CARTESIAN_POINT('Ctrl Pts',(181.078727888333,618.497661684668,-38.6983164508069)) ;
#58019=CARTESIAN_POINT('Ctrl Pts',(181.082182707133,618.497442937917,-38.6958662022202)) ;
#58020=CARTESIAN_POINT('Ctrl Pts',(181.085629426356,618.497223808628,-38.6934053789544)) ;
#58021=CARTESIAN_POINT('Ctrl Pts',(181.122314421018,618.494891516302,-38.6672137217535)) ;
#58022=CARTESIAN_POINT('Ctrl Pts',(181.158079903752,618.492515656591,-38.6398252694906)) ;
#58023=CARTESIAN_POINT('Ctrl Pts',(181.192836848114,618.490076781835,-38.6113088574816)) ;
#58024=CARTESIAN_POINT('Ctrl Pts',(181.192864076843,618.49007487121,-38.6112865176113)) ;
#58025=CARTESIAN_POINT('Ctrl Pts',(181.192891304952,618.490072960548,-38.6112641770488)) ;
#58026=CARTESIAN_POINT('Ctrl Pts',(181.192918532444,618.490071049846,-38.6112418357942)) ;
#58027=CARTESIAN_POINT('Ctrl Pts',(181.242673139758,618.486579497818,-38.5704161744067)) ;
#58028=CARTESIAN_POINT('Ctrl Pts',(181.290541683293,618.482949500952,-38.52712164623)) ;
#58029=CARTESIAN_POINT('Ctrl Pts',(181.336294377515,618.47924615687,-38.4815793682111)) ;
#58030=CARTESIAN_POINT('Ctrl Pts',(181.340932471314,618.47887073729,-38.4769626049605)) ;
#58031=CARTESIAN_POINT('Ctrl Pts',(181.345548813078,618.478494563957,-38.4723227860285)) ;
#58032=CARTESIAN_POINT('Ctrl Pts',(181.350143158393,618.478117704687,-38.4676601711489)) ;
#58033=CARTESIAN_POINT('Ctrl Pts',(181.39998204525,618.47402958217,-38.4170807045429)) ;
#58034=CARTESIAN_POINT('Ctrl Pts',(181.447234070826,618.4698613568,-38.3638129387118)) ;
#58035=CARTESIAN_POINT('Ctrl Pts',(181.491635364602,618.465687402768,-38.3081764046326)) ;
#58036=CARTESIAN_POINT('Ctrl Pts',(181.535981829134,618.461518602973,-38.252608573711)) ;
#58037=CARTESIAN_POINT('Ctrl Pts',(181.577484930695,618.45734444223,-38.1946780085854)) ;
#58038=CARTESIAN_POINT('Ctrl Pts',(181.615918052772,618.453219658054,-38.1347204485888)) ;
#58039=CARTESIAN_POINT('Ctrl Pts',(181.654325510364,618.449097628284,-38.0748029264502)) ;
#58040=CARTESIAN_POINT('Ctrl Pts',(181.689667249886,618.445025077976,-38.0128611802261)) ;
#58041=CARTESIAN_POINT('Ctrl Pts',(181.721749657168,618.441033439463,-37.9492458730777)) ;
#58042=CARTESIAN_POINT('Ctrl Pts',(181.753821421396,618.437043125141,-37.8856516697398)) ;
#58043=CARTESIAN_POINT('Ctrl Pts',(181.78263603063,618.433133709202,-37.8203850336934)) ;
#58044=CARTESIAN_POINT('Ctrl Pts',(181.80803130034,618.42931187499,-37.7538112969984)) ;
#58045=CARTESIAN_POINT('Ctrl Pts',(181.833426678707,618.425490024426,-37.6872372754576)) ;
#58046=CARTESIAN_POINT('Ctrl Pts',(181.85540257914,618.421755691541,-37.619356141093)) ;
#58047=CARTESIAN_POINT('Ctrl Pts',(181.873828778154,618.418091025479,-37.550548137017)) ;
#58048=CARTESIAN_POINT('Ctrl Pts',(181.892273434705,618.414422688518,-37.4816712079157)) ;
#58049=CARTESIAN_POINT('Ctrl Pts',(181.907161034768,618.410823979583,-37.4118655412063)) ;
#58050=CARTESIAN_POINT('Ctrl Pts',(181.91839560142,618.407254203748,-37.3415275613066)) ;
#58051=CARTESIAN_POINT('Ctrl Pts',(181.929636220517,618.403682504752,-37.2711516879324)) ;
#58052=CARTESIAN_POINT('Ctrl Pts',(181.937219477996,618.400139432256,-37.2002429455114)) ;
#58053=CARTESIAN_POINT('Ctrl Pts',(181.941088598904,618.39656524962,-37.1292134404523)) ;
#58054=CARTESIAN_POINT('Ctrl Pts',(181.944752203609,618.393180916943,-37.0619568116149)) ;
#58055=CARTESIAN_POINT('Ctrl Pts',(181.94508548051,618.389768200429,-36.9945915705661)) ;
#58056=CARTESIAN_POINT('Ctrl Pts',(181.942079051817,618.386265885841,-36.92748080267)) ;
#58057=CARTESIAN_POINT('Ctrl Pts',(181.94190493884,618.386063054349,-36.9235941794562)) ;
#58058=CARTESIAN_POINT('Ctrl Pts',(181.94171963135,618.385859922347,-36.9197083968835)) ;
#58059=CARTESIAN_POINT('Ctrl Pts',(181.941523129918,618.385656477945,-36.915823520671)) ;
#58060=CARTESIAN_POINT('Ctrl Pts',(181.93935010503,618.383406673734,-36.8728623442949)) ;
#58061=CARTESIAN_POINT('Ctrl Pts',(181.935808169022,618.381118446845,-36.8300140550891)) ;
#58062=CARTESIAN_POINT('Ctrl Pts',(181.930904882405,618.378775043707,-36.7873756177613)) ;
#58063=CARTESIAN_POINT('Ctrl Pts',(181.930900988185,618.378773182562,-36.7873417540572)) ;
#58064=CARTESIAN_POINT('Ctrl Pts',(181.930897093107,618.378771321383,-36.7873078904849)) ;
#58065=CARTESIAN_POINT('Ctrl Pts',(181.93089319717,618.378769460168,-36.7872740270446)) ;
#58066=CARTESIAN_POINT('Ctrl Pts',(181.923496304728,618.37523572605,-36.7229803128489)) ;
#58067=CARTESIAN_POINT('Ctrl Pts',(181.912971962119,618.371567819245,-36.6589431336752)) ;
#58068=CARTESIAN_POINT('Ctrl Pts',(181.899383298866,618.367830687328,-36.595478813972)) ;
#58069=CARTESIAN_POINT('Ctrl Pts',(181.898055332695,618.367465472246,-36.5892766976896)) ;
#58070=CARTESIAN_POINT('Ctrl Pts',(181.896698130639,618.367099596038,-36.5830800809786)) ;
#58071=CARTESIAN_POINT('Ctrl Pts',(181.89531177119,618.366733119321,-36.5768892771111)) ;
#58072=CARTESIAN_POINT('Ctrl Pts',(181.87984539817,618.362644666207,-36.5078240126944)) ;
#58073=CARTESIAN_POINT('Ctrl Pts',(181.860746264821,618.358482213079,-36.4394783858795)) ;
#58074=CARTESIAN_POINT('Ctrl Pts',(181.83813916127,618.35431735719,-36.3722398226686)) ;
#58075=CARTESIAN_POINT('Ctrl Pts',(181.836937952426,618.354096061184,-36.3686671599152)) ;
#58076=CARTESIAN_POINT('Ctrl Pts',(181.835726847168,618.353874758394,-36.3650976323868)) ;
#58077=CARTESIAN_POINT('Ctrl Pts',(181.8345058668,618.353653459561,-36.3615313014004)) ;
#58078=CARTESIAN_POINT('Ctrl Pts',(181.811430103808,618.349471050443,-36.2941298830263)) ;
#58079=CARTESIAN_POINT('Ctrl Pts',(181.784824745324,618.345290261806,-36.2278660420256)) ;
#58080=CARTESIAN_POINT('Ctrl Pts',(181.75485184391,618.341163559267,-36.1631118241443)) ;
#58081=CARTESIAN_POINT('Ctrl Pts',(181.724898856605,618.337039598525,-36.0984006292118)) ;
#58082=CARTESIAN_POINT('Ctrl Pts',(181.691582932313,618.332969810021,-36.0351969575839)) ;
#58083=CARTESIAN_POINT('Ctrl Pts',(181.655096405581,618.328983264932,-35.9738533116335)) ;
#58084=CARTESIAN_POINT('Ctrl Pts',(181.618619862224,618.324997810633,-35.9125264504166)) ;
#58085=CARTESIAN_POINT('Ctrl Pts',(181.578974467337,618.321095586499,-35.853058600381)) ;
#58086=CARTESIAN_POINT('Ctrl Pts',(181.536381933975,618.317280962604,-35.7957838575602)) ;
#58087=CARTESIAN_POINT('Ctrl Pts',(181.53008148432,618.316716688918,-35.7873115595969)) ;
#58088=CARTESIAN_POINT('Ctrl Pts',(181.523716599731,618.316154287881,-35.7788872173185)) ;
#58089=CARTESIAN_POINT('Ctrl Pts',(181.51728805297,618.315593727817,-35.7705118777721)) ;
#58090=CARTESIAN_POINT('',(177.90335329975,618.710565160536,-37.552330388949)) ;
#58091=CARTESIAN_POINT('Ctrl Pts',(177.90335329975,618.710565160536,-37.552330388949)) ;
#58092=CARTESIAN_POINT('Ctrl Pts',(177.922083606511,618.706629227194,-37.6224643249733)) ;
#58093=CARTESIAN_POINT('Ctrl Pts',(177.944552733151,618.702693293853,-37.6916719620047)) ;
#58094=CARTESIAN_POINT('Ctrl Pts',(177.970646133763,618.698757360511,-37.7595394137045)) ;
#58095=CARTESIAN_POINT('Ctrl Pts',(177.996718458269,618.694824606293,-37.8273520476528)) ;
#58096=CARTESIAN_POINT('Ctrl Pts',(178.026409071389,618.690891852074,-37.8938262197478)) ;
#58097=CARTESIAN_POINT('Ctrl Pts',(178.059554051881,618.686959097856,-37.9585645874841)) ;
#58098=CARTESIAN_POINT('Ctrl Pts',(178.092688887672,618.683027547338,-38.0232831407163)) ;
#58099=CARTESIAN_POINT('Ctrl Pts',(178.129275785989,618.67909599682,-38.086266532727)) ;
#58100=CARTESIAN_POINT('Ctrl Pts',(178.169103756104,618.675164446301,-38.1471397805177)) ;
#58101=CARTESIAN_POINT('Ctrl Pts',(178.208927037003,618.671233358671,-38.2080058612881)) ;
#58102=CARTESIAN_POINT('Ctrl Pts',(178.251990379354,618.667302271041,-38.2667619058341)) ;
#58103=CARTESIAN_POINT('Ctrl Pts',(178.29803893613,618.663371183411,-38.3230611256129)) ;
#58104=CARTESIAN_POINT('Ctrl Pts',(178.344095108192,618.659439445677,-38.3793696558808)) ;
#58105=CARTESIAN_POINT('Ctrl Pts',(178.39313718377,618.655507707943,-38.4332201974016)) ;
#58106=CARTESIAN_POINT('Ctrl Pts',(178.444870336052,618.651575970209,-38.484299424139)) ;
#58107=CARTESIAN_POINT('Ctrl Pts',(178.496626691879,618.647642468997,-38.535401561121)) ;
#58108=CARTESIAN_POINT('Ctrl Pts',(178.551076195138,618.643708967785,-38.5837295897)) ;
#58109=CARTESIAN_POINT('Ctrl Pts',(178.607888558719,618.639775466573,-38.6290083734684)) ;
#58110=CARTESIAN_POINT('Ctrl Pts',(178.664784842608,618.635836154995,-38.6743540407325)) ;
#58111=CARTESIAN_POINT('Ctrl Pts',(178.724050592454,618.631896843418,-38.7166411852367)) ;
#58112=CARTESIAN_POINT('Ctrl Pts',(178.785324331511,618.62795753184,-38.7556364637246)) ;
#58113=CARTESIAN_POINT('Ctrl Pts',(178.846648938566,618.624014949939,-38.7946641151639)) ;
#58114=CARTESIAN_POINT('Ctrl Pts',(178.909984453703,618.620072368038,-38.8303942316352)) ;
#58115=CARTESIAN_POINT('Ctrl Pts',(178.974944743423,618.616129786138,-38.8626394246227)) ;
#58116=CARTESIAN_POINT('Ctrl Pts',(179.040028692326,618.612179699091,-38.8949459999443)) ;
#58117=CARTESIAN_POINT('Ctrl Pts',(179.106743168932,618.608229612045,-38.9237542227441)) ;
#58118=CARTESIAN_POINT('Ctrl Pts',(179.174682422129,618.604279524998,-38.948924970129)) ;
#58119=CARTESIAN_POINT('Ctrl Pts',(179.202984719819,618.602633988225,-38.9594106606842)) ;
#58120=CARTESIAN_POINT('Ctrl Pts',(179.231499396579,618.600988451452,-38.9692657018397)) ;
#58121=CARTESIAN_POINT('Ctrl Pts',(179.26019651201,618.599342914678,-38.9784826335278)) ;
#58122=CARTESIAN_POINT('Ctrl Pts',(179.339550661574,618.594792625589,-39.0039695775893)) ;
#58123=CARTESIAN_POINT('Ctrl Pts',(179.420542892379,618.5902423365,-39.024651836472)) ;
#58124=CARTESIAN_POINT('Ctrl Pts',(179.50263213996,618.585692047411,-39.0403480314002)) ;
#58125=CARTESIAN_POINT('Ctrl Pts',(179.583845704284,618.581190298321,-39.0558767878938)) ;
#58126=CARTESIAN_POINT('Ctrl Pts',(179.666132889144,618.576688549231,-39.0665252057191)) ;
#58127=CARTESIAN_POINT('Ctrl Pts',(179.748948669339,618.572186800141,-39.0721638979804)) ;
#58128=CARTESIAN_POINT('Ctrl Pts',(179.795221919972,618.569671451454,-39.0753145127502)) ;
#58129=CARTESIAN_POINT('Ctrl Pts',(179.841659828985,618.567156102768,-39.0769019237886)) ;
#58130=CARTESIAN_POINT('Ctrl Pts',(179.888164616977,618.564640754081,-39.0769101396937)) ;
#58131=CARTESIAN_POINT('',(177.901919214914,618.709347838499,-36.4891859383096)) ;
#58132=CARTESIAN_POINT('Origin',(179.888527625422,618.710565160536,-37.0221601717597)) ;
#58133=CARTESIAN_POINT('Ctrl Pts',(177.903934811095,618.708121040096,-36.4898173087268)) ;
#58134=CARTESIAN_POINT('Ctrl Pts',(177.89961331501,618.70721870862,-36.5059279972954)) ;
#58135=CARTESIAN_POINT('Ctrl Pts',(177.895488008535,618.706327482754,-36.522091261017)) ;
#58136=CARTESIAN_POINT('Ctrl Pts',(177.886633355003,618.704340332833,-36.558636087596)) ;
#58137=CARTESIAN_POINT('Ctrl Pts',(177.882017504782,618.70325007211,-36.5790434341295)) ;
#58138=CARTESIAN_POINT('Ctrl Pts',(177.847956110036,618.694720105473,-36.7410982126199)) ;
#58139=CARTESIAN_POINT('Ctrl Pts',(177.833231202522,618.687867576172,-36.8854382773337)) ;
#58140=CARTESIAN_POINT('Ctrl Pts',(177.834192659606,618.67580505919,-37.1330268029234)) ;
#58141=CARTESIAN_POINT('Ctrl Pts',(177.842319395807,618.67071454387,-37.2357312845398)) ;
#58142=CARTESIAN_POINT('Ctrl Pts',(177.866104838432,618.662686387422,-37.3889365830538)) ;
#58143=CARTESIAN_POINT('Ctrl Pts',(177.876067460293,618.659929360742,-37.4401581341412)) ;
#58144=CARTESIAN_POINT('Ctrl Pts',(177.900297135361,618.654186813558,-37.5435599297601)) ;
#58145=CARTESIAN_POINT('Ctrl Pts',(177.914696888043,618.651198863856,-37.5956666098326)) ;
#58146=CARTESIAN_POINT('Ctrl Pts',(177.981046279874,618.638880335466,-37.8034677918017)) ;
#58147=CARTESIAN_POINT('Ctrl Pts',(178.049501899252,618.629007724035,-37.9532323266272)) ;
#58148=CARTESIAN_POINT('Ctrl Pts',(178.17967765215,618.614064101347,-38.1663497344923)) ;
#58149=CARTESIAN_POINT('Ctrl Pts',(178.228871061269,618.608981376482,-38.2366067359811)) ;
#58150=CARTESIAN_POINT('Ctrl Pts',(178.302289575914,618.602299660776,-38.328633536338)) ;
#58151=CARTESIAN_POINT('Ctrl Pts',(178.322852354449,618.600513368516,-38.3532067691423)) ;
#58152=CARTESIAN_POINT('Ctrl Pts',(178.36575584161,618.596972252822,-38.4021071171549)) ;
#58153=CARTESIAN_POINT('Ctrl Pts',(178.388125183866,618.595220293271,-38.4263967150322)) ;
#58154=CARTESIAN_POINT('Ctrl Pts',(178.505050836438,618.58646734713,-38.5473737279596)) ;
#58155=CARTESIAN_POINT('Ctrl Pts',(178.608410297247,618.580012766468,-38.6351053656314)) ;
#58156=CARTESIAN_POINT('Ctrl Pts',(178.787843049251,618.569455660769,-38.7592168399994)) ;
#58157=CARTESIAN_POINT('Ctrl Pts',(178.858824452271,618.565422800512,-38.8022115113597)) ;
#58158=CARTESIAN_POINT('Ctrl Pts',(178.990564734723,618.55796187353,-38.871486449181)) ;
#58159=CARTESIAN_POINT('Ctrl Pts',(179.050362128865,618.554584290457,-38.8993448978869)) ;
#58160=CARTESIAN_POINT('Ctrl Pts',(179.157258933908,618.54849327467,-38.9430190012259)) ;
#58161=CARTESIAN_POINT('Ctrl Pts',(179.20378586791,618.545825814901,-38.9600922339088)) ;
#58162=CARTESIAN_POINT('Ctrl Pts',(179.312169929997,618.539556043029,-38.9954736023798)) ;
#58163=CARTESIAN_POINT('Ctrl Pts',(179.374360329489,618.535917063841,-39.0125834421195)) ;
#58164=CARTESIAN_POINT('Ctrl Pts',(179.5802153312,618.523740225149,-39.0589264262495)) ;
#58165=CARTESIAN_POINT('Ctrl Pts',(179.726206525767,618.514864335276,-39.0757221602284)) ;
#58166=CARTESIAN_POINT('Ctrl Pts',(179.948302534723,618.501608568692,-39.0774308612065)) ;
#58167=CARTESIAN_POINT('Ctrl Pts',(180.023866402557,618.497150861992,-39.0738414215875)) ;
#58168=CARTESIAN_POINT('Ctrl Pts',(180.130322055668,618.491088932512,-39.0628758123629)) ;
#58169=CARTESIAN_POINT('Ctrl Pts',(180.161502796812,618.48934047946,-39.0589394319344)) ;
#58170=CARTESIAN_POINT('Ctrl Pts',(180.225712322454,618.485813081276,-39.0493321260682)) ;
#58171=CARTESIAN_POINT('Ctrl Pts',(180.258717135631,618.484039559066,-39.0435655412924)) ;
#58172=CARTESIAN_POINT('Ctrl Pts',(180.330747227359,618.480227518069,-39.0291568835457)) ;
#58173=CARTESIAN_POINT('Ctrl Pts',(180.369691397373,618.4782045599,-39.020178123827)) ;
#58174=CARTESIAN_POINT('Ctrl Pts',(180.493796374131,618.471811475084,-38.9877256030707)) ;
#58175=CARTESIAN_POINT('Ctrl Pts',(180.577716191718,618.467567438777,-38.9598955044967)) ;
#58176=CARTESIAN_POINT('Ctrl Pts',(180.774970011025,618.457285290354,-38.8800386740116)) ;
#58177=CARTESIAN_POINT('Ctrl Pts',(180.885861987713,618.451232463878,-38.8229414252176)) ;
#58178=CARTESIAN_POINT('Ctrl Pts',(181.035385943492,618.442112491024,-38.7278836789447)) ;
#58179=CARTESIAN_POINT('Ctrl Pts',(181.07876619861,618.439342195626,-38.697901246832)) ;
#58180=CARTESIAN_POINT('Ctrl Pts',(181.162137476564,618.433736417945,-38.6354071935382)) ;
#58181=CARTESIAN_POINT('Ctrl Pts',(181.202153551803,618.430906022112,-38.602993575127)) ;
#58182=CARTESIAN_POINT('Ctrl Pts',(181.317403243452,618.422310838689,-38.5022397837769)) ;
#58183=CARTESIAN_POINT('Ctrl Pts',(181.388823549767,618.416376584277,-38.4297925276021)) ;
#58184=CARTESIAN_POINT('Ctrl Pts',(181.541737413827,618.40229258387,-38.2497665914924)) ;
#58185=CARTESIAN_POINT('Ctrl Pts',(181.618593258647,618.394074008006,-38.1388488094641)) ;
#58186=CARTESIAN_POINT('Ctrl Pts',(181.704910577153,618.383739431602,-37.9837170132153)) ;
#58187=CARTESIAN_POINT('Ctrl Pts',(181.724594738408,618.381285270113,-37.9455759404892)) ;
#58188=CARTESIAN_POINT('Ctrl Pts',(181.755437896193,618.377301698849,-37.8809200770703)) ;
#58189=CARTESIAN_POINT('Ctrl Pts',(181.767258746696,618.375737504471,-37.8547417504993)) ;
#58190=CARTESIAN_POINT('Ctrl Pts',(181.796316346807,618.371787103676,-37.7866176271214)) ;
#58191=CARTESIAN_POINT('Ctrl Pts',(181.812720084319,618.369445895648,-37.7443353452659)) ;
#58192=CARTESIAN_POINT('Ctrl Pts',(181.848797120666,618.363929626167,-37.6413593251634)) ;
#58193=CARTESIAN_POINT('Ctrl Pts',(181.867069807588,618.360804865118,-37.5802244572526)) ;
#58194=CARTESIAN_POINT('Ctrl Pts',(181.922437871714,618.349665604171,-37.357721203799)) ;
#58195=CARTESIAN_POINT('Ctrl Pts',(181.942850800634,618.341788867134,-37.1928801363761)) ;
#58196=CARTESIAN_POINT('Ctrl Pts',(181.943404022786,618.330546555151,-36.9749850571563)) ;
#58197=CARTESIAN_POINT('Ctrl Pts',(181.941533167896,618.327787165639,-36.9226107820929)) ;
#58198=CARTESIAN_POINT('Ctrl Pts',(181.93379970047,618.322143924147,-36.8182119053593)) ;
#58199=CARTESIAN_POINT('Ctrl Pts',(181.927946609171,618.319262393995,-36.7662260929597)) ;
#58200=CARTESIAN_POINT('Ctrl Pts',(181.90300970013,618.309889593059,-36.6015463543813)) ;
#58201=CARTESIAN_POINT('Ctrl Pts',(181.876510221542,618.303170319916,-36.4902080197683)) ;
#58202=CARTESIAN_POINT('Ctrl Pts',(181.797194748318,618.287933050784,-36.2484378800886)) ;
#58203=CARTESIAN_POINT('Ctrl Pts',(181.739966540451,618.279386662566,-36.1200328535147)) ;
#58204=CARTESIAN_POINT('Ctrl Pts',(181.653501196833,618.269481012114,-35.9695554823476)) ;
#58205=CARTESIAN_POINT('Ctrl Pts',(181.63619477641,618.267612317719,-35.941064356618)) ;
#58206=CARTESIAN_POINT('Ctrl Pts',(181.604025215241,618.264352052203,-35.8908974682713)) ;
#58207=CARTESIAN_POINT('Ctrl Pts',(181.589425771995,618.262944376528,-35.8690630999813)) ;
#58208=CARTESIAN_POINT('Ctrl Pts',(181.556124742666,618.259874760947,-35.8212685712881)) ;
#58209=CARTESIAN_POINT('Ctrl Pts',(181.537232829484,618.258225086448,-35.7954604800369)) ;
#58210=CARTESIAN_POINT('Ctrl Pts',(181.517739089185,618.256600448668,-35.770094850444)) ;
#58211=CARTESIAN_POINT('Origin',(29.8885276254223,620.2564904411,-37.0221601717529)) ;
#58212=CARTESIAN_POINT('',(31.5177255283109,616.918093972863,-35.7700772049646)) ;
#58213=CARTESIAN_POINT('',(31.5177255072015,616.859929736371,-35.7700771774972)) ;
#58214=CARTESIAN_POINT('',(31.5177255210695,620.2564904411,-35.7700771955414)) ;
#58215=CARTESIAN_POINT('',(29.0652954453167,616.710565160562,-35.13953266209)) ;
#58216=CARTESIAN_POINT('Ctrl Pts',(31.5177255072015,616.859929736371,-35.7700771774972)) ;
#58217=CARTESIAN_POINT('Ctrl Pts',(31.5070758016168,616.858913289289,-35.7562198869983)) ;
#58218=CARTESIAN_POINT('Ctrl Pts',(31.4962483273789,616.857891707172,-35.7424972042907)) ;
#58219=CARTESIAN_POINT('Ctrl Pts',(31.3993198244515,616.848852906981,-35.622823695312)) ;
#58220=CARTESIAN_POINT('Ctrl Pts',(31.3030407494217,616.84056895853,-35.5255688104259)) ;
#58221=CARTESIAN_POINT('Ctrl Pts',(31.1577709294923,616.829521299164,-35.4054595155509)) ;
#58222=CARTESIAN_POINT('Ctrl Pts',(31.1164640319347,616.826523350537,-35.3738663346817)) ;
#58223=CARTESIAN_POINT('Ctrl Pts',(31.0496272070208,616.821948325107,-35.3266555931457)) ;
#58224=CARTESIAN_POINT('Ctrl Pts',(31.0248811535925,616.820312007831,-35.3099717983299)) ;
#58225=CARTESIAN_POINT('Ctrl Pts',(30.9647529495311,616.816478629932,-35.2713117111252)) ;
#58226=CARTESIAN_POINT('Ctrl Pts',(30.9290507794141,616.814312021376,-35.2498612881938)) ;
#58227=CARTESIAN_POINT('Ctrl Pts',(30.7974219010079,616.80662762584,-35.1761265851227)) ;
#58228=CARTESIAN_POINT('Ctrl Pts',(30.6980120090074,616.801384371956,-35.1304235094043)) ;
#58229=CARTESIAN_POINT('Ctrl Pts',(30.471555861231,616.78977377737,-35.0474497055228)) ;
#58230=CARTESIAN_POINT('Ctrl Pts',(30.3436058340661,616.783413451447,-35.0141005035696)) ;
#58231=CARTESIAN_POINT('Ctrl Pts',(30.1546124015791,616.773647561923,-34.9838435558175)) ;
#58232=CARTESIAN_POINT('Ctrl Pts',(30.0955014531932,616.770546090958,-34.9769959522721)) ;
#58233=CARTESIAN_POINT('Ctrl Pts',(29.9804744645932,616.764381935861,-34.9687087925195)) ;
#58234=CARTESIAN_POINT('Ctrl Pts',(29.9246323255411,616.761331149433,-34.9669685864957)) ;
#58235=CARTESIAN_POINT('Ctrl Pts',(29.8098147855787,616.754928891967,-34.9680714506353)) ;
#58236=CARTESIAN_POINT('Ctrl Pts',(29.7508931735155,616.751573047756,-34.971176959048)) ;
#58237=CARTESIAN_POINT('Ctrl Pts',(29.5090659293153,616.737541431677,-34.9943905089217)) ;
#58238=CARTESIAN_POINT('Ctrl Pts',(29.3291426086356,616.726413364237,-35.0364799321757)) ;
#58239=CARTESIAN_POINT('Ctrl Pts',(29.1262892653866,616.714195092401,-35.1137350351922)) ;
#58240=CARTESIAN_POINT('Ctrl Pts',(29.0956350468344,616.712360570578,-35.1262658123426)) ;
#58241=CARTESIAN_POINT('Ctrl Pts',(29.0652954453167,616.710565160562,-35.13953266209)) ;
#58242=CARTESIAN_POINT('',(28.2344189562597,616.711828241264,-35.79952680519)) ;
#58243=CARTESIAN_POINT('Origin',(29.8885276254216,616.710565160562,-37.0221601717529)) ;
#58244=CARTESIAN_POINT('Ctrl Pts',(28.2363225441489,616.713091321964,-35.8005972663254)) ;
#58245=CARTESIAN_POINT('Ctrl Pts',(28.2461879736039,616.713987411299,-35.787253939836)) ;
#58246=CARTESIAN_POINT('Ctrl Pts',(28.2562150344361,616.714872582277,-35.7740301393109)) ;
#58247=CARTESIAN_POINT('Ctrl Pts',(28.2799467919758,616.716912631926,-35.7435076644347)) ;
#58248=CARTESIAN_POINT('Ctrl Pts',(28.2937722969416,616.718060065299,-35.7263052242832)) ;
#58249=CARTESIAN_POINT('Ctrl Pts',(28.3869420455029,616.725551514342,-35.6141284741815)) ;
#58250=CARTESIAN_POINT('Ctrl Pts',(28.4744573232012,616.731475828916,-35.5262580427306)) ;
#58251=CARTESIAN_POINT('Ctrl Pts',(28.6596557087188,616.743190129311,-35.3711777069199)) ;
#58252=CARTESIAN_POINT('Ctrl Pts',(28.7562840888164,616.748954333741,-35.3034715834117)) ;
#58253=CARTESIAN_POINT('Ctrl Pts',(28.9040598591426,616.757766104653,-35.217822661049)) ;
#58254=CARTESIAN_POINT('Ctrl Pts',(28.9509573279974,616.760559292809,-35.1930150451144)) ;
#58255=CARTESIAN_POINT('Ctrl Pts',(29.0464682789855,616.766271136086,-35.1471308166295)) ;
#58256=CARTESIAN_POINT('Ctrl Pts',(29.0950415055828,616.769187351072,-35.1260646905364)) ;
#58257=CARTESIAN_POINT('Ctrl Pts',(29.2473293032392,616.778380676497,-35.0668947150754)) ;
#58258=CARTESIAN_POINT('Ctrl Pts',(29.3533330904979,616.784861443889,-35.0352631740274)) ;
#58259=CARTESIAN_POINT('Ctrl Pts',(29.5549607882299,616.797170951437,-34.9924091893092)) ;
#58260=CARTESIAN_POINT('Ctrl Pts',(29.6498446545391,616.802952864566,-34.9790775434269)) ;
#58261=CARTESIAN_POINT('Ctrl Pts',(29.7866736101263,616.811046505724,-34.9695173861438)) ;
#58262=CARTESIAN_POINT('Ctrl Pts',(29.8281148978698,616.813464912003,-34.9678799296528)) ;
#58263=CARTESIAN_POINT('Ctrl Pts',(29.9040235380157,616.817802751366,-34.9671798941917)) ;
#58264=CARTESIAN_POINT('Ctrl Pts',(29.9384725971119,616.819736644985,-34.9677284066378)) ;
#58265=CARTESIAN_POINT('Ctrl Pts',(30.003914294452,616.823323617532,-34.9704176490453)) ;
#58266=CARTESIAN_POINT('Ctrl Pts',(30.0349022557098,616.824983304555,-34.9723953062286)) ;
#58267=CARTESIAN_POINT('Ctrl Pts',(30.1377297047151,616.830393633256,-34.9813016263603)) ;
#58268=CARTESIAN_POINT('Ctrl Pts',(30.2092536173663,616.834000962602,-34.9913125852556)) ;
#58269=CARTESIAN_POINT('Ctrl Pts',(30.4436538618571,616.845717434096,-35.03681693915)) ;
#58270=CARTESIAN_POINT('Ctrl Pts',(30.6027257030683,616.853550066324,-35.088336202994)) ;
#58271=CARTESIAN_POINT('Ctrl Pts',(30.8081311364695,616.865020887423,-35.1837068592273)) ;
#58272=CARTESIAN_POINT('Ctrl Pts',(30.8612957951291,616.868118609061,-35.2112757521316)) ;
#58273=CARTESIAN_POINT('Ctrl Pts',(30.9563653462243,616.873947110266,-35.265970372132)) ;
#58274=CARTESIAN_POINT('Ctrl Pts',(30.9986314399163,616.876650128572,-35.2923772591693)) ;
#58275=CARTESIAN_POINT('Ctrl Pts',(31.1002082138946,616.883444628465,-35.3610970904895)) ;
#58276=CARTESIAN_POINT('Ctrl Pts',(31.1583049759041,616.887597582255,-35.4050751128561)) ;
#58277=CARTESIAN_POINT('Ctrl Pts',(31.3262979694729,616.900421320143,-35.5468859946604)) ;
#58278=CARTESIAN_POINT('Ctrl Pts',(31.4281461657989,616.909377068406,-35.6535162573635)) ;
#58279=CARTESIAN_POINT('Ctrl Pts',(31.5177316112097,616.918094564784,-35.7700851200118)) ;
#58280=CARTESIAN_POINT('Origin',(29.8885276254223,620.2564904411,-37.0221601717529)) ;
#58281=CARTESIAN_POINT('',(31.5177255210722,617.617782467769,-35.7700771955454)) ;
#58282=CARTESIAN_POINT('',(31.5177255210691,617.559653386529,-35.7700771955414)) ;
#58283=CARTESIAN_POINT('',(31.5177255210695,620.2564904411,-35.7700771955414)) ;
#58284=CARTESIAN_POINT('',(29.8879638322405,617.107918393054,-39.0769100944046)) ;
#58285=CARTESIAN_POINT('Ctrl Pts',(31.5177255210691,617.559653386529,-35.7700771955414)) ;
#58286=CARTESIAN_POINT('Ctrl Pts',(31.502991126039,617.558435449222,-35.7509049475094)) ;
#58287=CARTESIAN_POINT('Ctrl Pts',(31.4879129621458,617.557206784429,-35.7319858330172)) ;
#58288=CARTESIAN_POINT('Ctrl Pts',(31.4375483698562,617.553152210874,-35.6710337459098)) ;
#58289=CARTESIAN_POINT('Ctrl Pts',(31.4009221260746,617.550278991236,-35.6301580101145)) ;
#58290=CARTESIAN_POINT('Ctrl Pts',(31.3267030075278,617.544561639328,-35.5537187131028)) ;
#58291=CARTESIAN_POINT('Ctrl Pts',(31.289316142577,617.54172762946,-35.5180127086929)) ;
#58292=CARTESIAN_POINT('Ctrl Pts',(31.1799902393308,617.533548717352,-35.4212159312012)) ;
#58293=CARTESIAN_POINT('Ctrl Pts',(31.1051401783234,617.528066766664,-35.3636221502404)) ;
#58294=CARTESIAN_POINT('Ctrl Pts',(30.9123588128159,617.514315078443,-35.2353764267797)) ;
#58295=CARTESIAN_POINT('Ctrl Pts',(30.7907893302688,617.505931073154,-35.1710120597553)) ;
#58296=CARTESIAN_POINT('Ctrl Pts',(30.6195492721135,617.495100987945,-35.1012543683798)) ;
#58297=CARTESIAN_POINT('Ctrl Pts',(30.5747682416913,617.492356018127,-35.0848046893483)) ;
#58298=CARTESIAN_POINT('Ctrl Pts',(30.5017221218475,617.48806195108,-35.0608234065258)) ;
#58299=CARTESIAN_POINT('Ctrl Pts',(30.4738016783234,617.486464449153,-35.0523114567785)) ;
#58300=CARTESIAN_POINT('Ctrl Pts',(30.4046469229523,617.482616540755,-35.0328291440998)) ;
#58301=CARTESIAN_POINT('Ctrl Pts',(30.3632362678253,617.480401567754,-35.0225428867216)) ;
#58302=CARTESIAN_POINT('Ctrl Pts',(30.2653072842815,617.475308431126,-35.0014318743699)) ;
#58303=CARTESIAN_POINT('Ctrl Pts',(30.2085947381004,617.472469910751,-34.9916766096514)) ;
#58304=CARTESIAN_POINT('Ctrl Pts',(29.9731022906157,617.460882721466,-34.9612824677208)) ;
#58305=CARTESIAN_POINT('Ctrl Pts',(29.7924221408081,617.452382551702,-34.9617883859521)) ;
#58306=CARTESIAN_POINT('Ctrl Pts',(29.562198858248,617.44036749658,-34.9928126447981)) ;
#58307=CARTESIAN_POINT('Ctrl Pts',(29.510572338815,617.437601327174,-35.0017911498368)) ;
#58308=CARTESIAN_POINT('Ctrl Pts',(29.4066479320116,617.431858312386,-35.0239876255355)) ;
#58309=CARTESIAN_POINT('Ctrl Pts',(29.3544149773128,617.428879919666,-35.0373114459427)) ;
#58310=CARTESIAN_POINT('Ctrl Pts',(29.2383412229445,617.422041677258,-35.0718336985198)) ;
#58311=CARTESIAN_POINT('Ctrl Pts',(29.1748976216132,617.418149535632,-35.0941439369834)) ;
#58312=CARTESIAN_POINT('Ctrl Pts',(28.9873492175115,617.406210048386,-35.1706228033579)) ;
#58313=CARTESIAN_POINT('Ctrl Pts',(28.8673968171397,617.397956733476,-35.233976201964)) ;
#58314=CARTESIAN_POINT('Ctrl Pts',(28.7050266674759,617.386422592202,-35.3414313445753)) ;
#58315=CARTESIAN_POINT('Ctrl Pts',(28.6569455556233,617.382960385271,-35.3763379866491)) ;
#58316=CARTESIAN_POINT('Ctrl Pts',(28.5871134581726,617.377937531909,-35.4318123188885)) ;
#58317=CARTESIAN_POINT('Ctrl Pts',(28.5641899467216,617.376290411072,-35.4508501289309)) ;
#58318=CARTESIAN_POINT('Ctrl Pts',(28.5137153392614,617.372679274582,-35.4946588149386)) ;
#58319=CARTESIAN_POINT('Ctrl Pts',(28.486404875669,617.370732966615,-35.5196884152189)) ;
#58320=CARTESIAN_POINT('Ctrl Pts',(28.4265927164114,617.36644823922,-35.5775575195833)) ;
#58321=CARTESIAN_POINT('Ctrl Pts',(28.3944915102253,617.364132782466,-35.6107824627978)) ;
#58322=CARTESIAN_POINT('Ctrl Pts',(28.2803180623839,617.355715753428,-35.7372176454534)) ;
#58323=CARTESIAN_POINT('Ctrl Pts',(28.2056236270247,617.349824927486,-35.8367272637574)) ;
#58324=CARTESIAN_POINT('Ctrl Pts',(28.0952268731418,617.339508001895,-36.0154581225617)) ;
#58325=CARTESIAN_POINT('Ctrl Pts',(28.0547164842007,617.335204126619,-36.0912943017524)) ;
#58326=CARTESIAN_POINT('Ctrl Pts',(27.9980973707526,617.328102653095,-36.2154226000785)) ;
#58327=CARTESIAN_POINT('Ctrl Pts',(27.9788276283632,617.325417757679,-36.2621619029228)) ;
#58328=CARTESIAN_POINT('Ctrl Pts',(27.9418742575579,617.319629991556,-36.3621024476641)) ;
#58329=CARTESIAN_POINT('Ctrl Pts',(27.9246052753928,617.316515659955,-36.4154117360528)) ;
#58330=CARTESIAN_POINT('Ctrl Pts',(27.8928049523524,617.309799908756,-36.5292542321095)) ;
#58331=CARTESIAN_POINT('Ctrl Pts',(27.8788025471966,617.306185876264,-36.5898763071068)) ;
#58332=CARTESIAN_POINT('Ctrl Pts',(27.8417339647674,617.294067479475,-36.7917333186514)) ;
#58333=CARTESIAN_POINT('Ctrl Pts',(27.8306611104694,617.285318600139,-36.9347344745592)) ;
#58334=CARTESIAN_POINT('Ctrl Pts',(27.8359513091915,617.273794571544,-37.1303028387367)) ;
#58335=CARTESIAN_POINT('Ctrl Pts',(27.8393923308154,617.270748228964,-37.1828144292426)) ;
#58336=CARTESIAN_POINT('Ctrl Pts',(27.8478967474127,617.266146320857,-37.2644199927145)) ;
#58337=CARTESIAN_POINT('Ctrl Pts',(27.8515771213451,617.264526829675,-37.2936324753227)) ;
#58338=CARTESIAN_POINT('Ctrl Pts',(27.8616648490393,617.260817914198,-37.3618451048856)) ;
#58339=CARTESIAN_POINT('Ctrl Pts',(27.8685714178916,617.258753927448,-37.4007574734309)) ;
#58340=CARTESIAN_POINT('Ctrl Pts',(27.8990527993423,617.251075135044,-37.5477214915681)) ;
#58341=CARTESIAN_POINT('Ctrl Pts',(27.9302145641686,617.24575567078,-37.6540135586227)) ;
#58342=CARTESIAN_POINT('Ctrl Pts',(28.0157023503227,617.234196138655,-37.8771438990388)) ;
#58343=CARTESIAN_POINT('Ctrl Pts',(28.0727494026608,617.227959746302,-37.9924268047008)) ;
#58344=CARTESIAN_POINT('Ctrl Pts',(28.168040873026,617.218611856161,-38.146765489254)) ;
#58345=CARTESIAN_POINT('Ctrl Pts',(28.1976460384395,617.215820439363,-38.1908049243284)) ;
#58346=CARTESIAN_POINT('Ctrl Pts',(28.2598619851919,617.210134992398,-38.2760341031513)) ;
#58347=CARTESIAN_POINT('Ctrl Pts',(28.2924139222578,617.207244521475,-38.3172168987872)) ;
#58348=CARTESIAN_POINT('Ctrl Pts',(28.3984101666931,617.198064207035,-38.4412433327354)) ;
#58349=CARTESIAN_POINT('Ctrl Pts',(28.4769869049569,617.191563539166,-38.5194223987981)) ;
#58350=CARTESIAN_POINT('Ctrl Pts',(28.6718413347213,617.176279119739,-38.6842592156002)) ;
#58351=CARTESIAN_POINT('Ctrl Pts',(28.7917656033892,617.167437868424,-38.7657239882183)) ;
#58352=CARTESIAN_POINT('Ctrl Pts',(28.9492871742426,617.157217127079,-38.849996417456)) ;
#58353=CARTESIAN_POINT('Ctrl Pts',(28.9797206142325,617.155303028099,-38.8653172714772)) ;
#58354=CARTESIAN_POINT('Ctrl Pts',(29.039259880253,617.151694418015,-38.8934570856586)) ;
#58355=CARTESIAN_POINT('Ctrl Pts',(29.0683092671745,617.149995176269,-38.9063708426932)) ;
#58356=CARTESIAN_POINT('Ctrl Pts',(29.1692992035839,617.144259019019,-38.9484869463668)) ;
#58357=CARTESIAN_POINT('Ctrl Pts',(29.2425932038203,617.140388324798,-38.9742859911017)) ;
#58358=CARTESIAN_POINT('Ctrl Pts',(29.4630978199586,617.129131617353,-39.0381175533183)) ;
#58359=CARTESIAN_POINT('Ctrl Pts',(29.6132467134803,617.121925270207,-39.0640453542879)) ;
#58360=CARTESIAN_POINT('Ctrl Pts',(29.8058657166775,617.112166553026,-39.0756572525885)) ;
#58361=CARTESIAN_POINT('Ctrl Pts',(29.8469109682732,617.11006072416,-39.0768988301021)) ;
#58362=CARTESIAN_POINT('Ctrl Pts',(29.8879638322405,617.107918393054,-39.0769100944046)) ;
#58363=CARTESIAN_POINT('Ctrl Pts',(29.8879650432987,617.107918329855,-39.0769100947366)) ;
#58364=CARTESIAN_POINT('Ctrl Pts',(29.9315771889072,617.105642442673,-39.0769220355636)) ;
#58365=CARTESIAN_POINT('Ctrl Pts',(29.9751768076821,617.103326411558,-39.0755454802514)) ;
#58366=CARTESIAN_POINT('Ctrl Pts',(30.0708303228857,617.09813884521,-39.0694735329993)) ;
#58367=CARTESIAN_POINT('Ctrl Pts',(30.1228134801749,617.095249816721,-39.0641777290822)) ;
#58368=CARTESIAN_POINT('Ctrl Pts',(30.3382243479021,617.082966641511,-39.03389919662)) ;
#58369=CARTESIAN_POINT('Ctrl Pts',(30.4985175174765,617.073008081404,-38.9912251018306)) ;
#58370=CARTESIAN_POINT('Ctrl Pts',(30.7363796074016,617.057611673656,-38.8960377293712)) ;
#58371=CARTESIAN_POINT('Ctrl Pts',(30.8184930569696,617.052187039343,-38.856672950899)) ;
#58372=CARTESIAN_POINT('Ctrl Pts',(30.926001939634,617.045164364312,-38.796053574394)) ;
#58373=CARTESIAN_POINT('Ctrl Pts',(30.9538916559741,617.043350842893,-38.7794451825445)) ;
#58374=CARTESIAN_POINT('Ctrl Pts',(31.0098105175161,617.039750175778,-38.7443243603351)) ;
#58375=CARTESIAN_POINT('Ctrl Pts',(31.0378023568366,617.037965795252,-38.7257718348289)) ;
#58376=CARTESIAN_POINT('Ctrl Pts',(31.171043081828,617.029496975284,-38.6326825087456)) ;
#58377=CARTESIAN_POINT('Ctrl Pts',(31.2695811741949,617.02329746239,-38.5490283005279)) ;
#58378=CARTESIAN_POINT('Ctrl Pts',(31.4437645929501,617.011175323734,-38.3704025050064)) ;
#58379=CARTESIAN_POINT('Ctrl Pts',(31.5201380657735,617.005281005028,-38.276896562426)) ;
#58380=CARTESIAN_POINT('Ctrl Pts',(31.6180742208949,616.996289879995,-38.1328141854124)) ;
#58381=CARTESIAN_POINT('Ctrl Pts',(31.6465187571827,616.993459394362,-38.0872189692384)) ;
#58382=CARTESIAN_POINT('Ctrl Pts',(31.6996966574815,616.987671397294,-37.9940319069262)) ;
#58383=CARTESIAN_POINT('Ctrl Pts',(31.7244185946076,616.984716508215,-37.9464823676244)) ;
#58384=CARTESIAN_POINT('Ctrl Pts',(31.7953781938994,616.975336137687,-37.7958945905848)) ;
#58385=CARTESIAN_POINT('Ctrl Pts',(31.8349981783252,616.96869480133,-37.6899854309348)) ;
#58386=CARTESIAN_POINT('Ctrl Pts',(31.8917462987526,616.956207680718,-37.4893425415177)) ;
#58387=CARTESIAN_POINT('Ctrl Pts',(31.9113181040995,616.950414417912,-37.3956082111246)) ;
#58388=CARTESIAN_POINT('Ctrl Pts',(31.9320022987042,616.941395619489,-37.2445156793934)) ;
#58389=CARTESIAN_POINT('Ctrl Pts',(31.9373733476164,616.938086874235,-37.1878796874816)) ;
#58390=CARTESIAN_POINT('Ctrl Pts',(31.9419490093459,616.933230205193,-37.101689858339)) ;
#58391=CARTESIAN_POINT('Ctrl Pts',(31.9428778902427,616.931603421004,-37.0722570072935)) ;
#58392=CARTESIAN_POINT('Ctrl Pts',(31.9435203274071,616.928153804639,-37.0083387008325)) ;
#58393=CARTESIAN_POINT('Ctrl Pts',(31.942999213504,616.92634391122,-36.9738605568451)) ;
#58394=CARTESIAN_POINT('Ctrl Pts',(31.9370641261593,616.918769897551,-36.8266080748743)) ;
#58395=CARTESIAN_POINT('Ctrl Pts',(31.9232284056203,616.913380509238,-36.7143608993811)) ;
#58396=CARTESIAN_POINT('Ctrl Pts',(31.8720276180124,616.901387063719,-36.4681529992633)) ;
#58397=CARTESIAN_POINT('Ctrl Pts',(31.8301709992059,616.894798434857,-36.3357102627553)) ;
#58398=CARTESIAN_POINT('Ctrl Pts',(31.7532891834867,616.884937280678,-36.1574327091939)) ;
#58399=CARTESIAN_POINT('Ctrl Pts',(31.7292089626923,616.882049546242,-36.1072936903947)) ;
#58400=CARTESIAN_POINT('Ctrl Pts',(31.6797251012503,616.87642981557,-36.0141436132491)) ;
#58401=CARTESIAN_POINT('Ctrl Pts',(31.6547287678234,616.873714378485,-35.9709614851591)) ;
#58402=CARTESIAN_POINT('Ctrl Pts',(31.5938687678378,616.867356440517,-35.874132168649)) ;
#58403=CARTESIAN_POINT('Ctrl Pts',(31.5570063355971,616.863678843146,-35.8211889989262)) ;
#58404=CARTESIAN_POINT('Ctrl Pts',(31.5177255072015,616.859929736371,-35.7700771774972)) ;
#58405=CARTESIAN_POINT('Ctrl Pts',(31.5177255283109,616.918093972863,-35.7700772049646)) ;
#58406=CARTESIAN_POINT('Ctrl Pts',(31.5504703761168,616.92128033574,-35.812684475242)) ;
#58407=CARTESIAN_POINT('Ctrl Pts',(31.5815278351766,616.924425086327,-35.8565546524622)) ;
#58408=CARTESIAN_POINT('Ctrl Pts',(31.6257430902973,616.929040762863,-35.9245140082766)) ;
#58409=CARTESIAN_POINT('Ctrl Pts',(31.6401914556706,616.930574133232,-35.9477214087963)) ;
#58410=CARTESIAN_POINT('Ctrl Pts',(31.6695115632588,616.93372873491,-35.9969806283676)) ;
#58411=CARTESIAN_POINT('Ctrl Pts',(31.6842835650919,616.935341188256,-36.0230818316763)) ;
#58412=CARTESIAN_POINT('Ctrl Pts',(31.7268984222215,616.940085810236,-36.10238056251)) ;
#58413=CARTESIAN_POINT('Ctrl Pts',(31.7529882615877,616.9431230095,-36.1564873560444)) ;
#58414=CARTESIAN_POINT('Ctrl Pts',(31.8297213296731,616.952761267061,-36.335245781618)) ;
#58415=CARTESIAN_POINT('Ctrl Pts',(31.8705100498814,616.959108104695,-36.4637403265578)) ;
#58416=CARTESIAN_POINT('Ctrl Pts',(31.9123597814348,616.96900463626,-36.6607963977105)) ;
#58417=CARTESIAN_POINT('Ctrl Pts',(31.9230586170022,616.97234802105,-36.7269262624697)) ;
#58418=CARTESIAN_POINT('Ctrl Pts',(31.9364883062573,616.978544805199,-36.8468335709622)) ;
#58419=CARTESIAN_POINT('Ctrl Pts',(31.9403709603395,616.981361522084,-36.900420321945)) ;
#58420=CARTESIAN_POINT('Ctrl Pts',(31.9438520414071,616.987006424688,-37.0054489306091)) ;
#58421=CARTESIAN_POINT('Ctrl Pts',(31.9436271335698,616.98982675231,-37.0568452382634)) ;
#58422=CARTESIAN_POINT('Ctrl Pts',(31.9374503976631,616.998098742825,-37.2042659241374)) ;
#58423=CARTESIAN_POINT('Ctrl Pts',(31.9266836122089,617.003696372191,-37.2999430552917)) ;
#58424=CARTESIAN_POINT('Ctrl Pts',(31.888853368992,617.016112342874,-37.5052493637281)) ;
#58425=CARTESIAN_POINT('Ctrl Pts',(31.8593789487323,617.022957650745,-37.6141250879011)) ;
#58426=CARTESIAN_POINT('Ctrl Pts',(31.8060606756644,617.0322757838,-37.761777724535)) ;
#58427=CARTESIAN_POINT('Ctrl Pts',(31.7896382870827,617.034880784364,-37.8030223878796)) ;
#58428=CARTESIAN_POINT('Ctrl Pts',(31.7574948070252,617.039500564444,-37.8767102755709)) ;
#58429=CARTESIAN_POINT('Ctrl Pts',(31.742231314005,617.041533138547,-37.9093338835254)) ;
#58430=CARTESIAN_POINT('Ctrl Pts',(31.712653570239,617.045169952847,-37.9684516292274)) ;
#58431=CARTESIAN_POINT('Ctrl Pts',(31.6986006541938,617.046786975107,-37.995062353153)) ;
#58432=CARTESIAN_POINT('Ctrl Pts',(31.6541338665252,617.051604966576,-38.0749640872589)) ;
#58433=CARTESIAN_POINT('Ctrl Pts',(31.6219113062678,617.054706274737,-38.127213892491)) ;
#58434=CARTESIAN_POINT('Ctrl Pts',(31.5123835074203,617.064349323908,-38.2882066630305)) ;
#58435=CARTESIAN_POINT('Ctrl Pts',(31.4268140636884,617.070653774258,-38.3909037134841)) ;
#58436=CARTESIAN_POINT('Ctrl Pts',(31.2842042798917,617.080513330055,-38.5316547445731)) ;
#58437=CARTESIAN_POINT('Ctrl Pts',(31.2342442199837,617.08386525464,-38.5763587020572)) ;
#58438=CARTESIAN_POINT('Ctrl Pts',(31.140624725421,617.090065034447,-38.6522255057367)) ;
#58439=CARTESIAN_POINT('Ctrl Pts',(31.097760134777,617.092875582938,-38.6842721361552)) ;
#58440=CARTESIAN_POINT('Ctrl Pts',(31.0108498884887,617.098551729317,-38.7441056503696)) ;
#58441=CARTESIAN_POINT('Ctrl Pts',(30.9669019100713,617.101411522617,-38.7719635021546)) ;
#58442=CARTESIAN_POINT('Ctrl Pts',(30.7649452818898,617.114532418059,-38.8894805824347)) ;
#58443=CARTESIAN_POINT('Ctrl Pts',(30.5965423156839,617.125515560337,-38.9596033015113)) ;
#58444=CARTESIAN_POINT('Ctrl Pts',(30.343239904977,617.141223374881,-39.0275887881929)) ;
#58445=CARTESIAN_POINT('Ctrl Pts',(30.2641443442507,617.146004141819,-39.0438974097544)) ;
#58446=CARTESIAN_POINT('Ctrl Pts',(30.1528958369099,617.152386198162,-39.060079057168)) ;
#58447=CARTESIAN_POINT('Ctrl Pts',(30.1213984966922,617.1541551225,-39.0639181032308)) ;
#58448=CARTESIAN_POINT('Ctrl Pts',(30.0565752019225,617.157700480766,-39.0702992396898)) ;
#58449=CARTESIAN_POINT('Ctrl Pts',(30.0232512775326,617.159472735478,-39.0727609262248)) ;
#58450=CARTESIAN_POINT('Ctrl Pts',(29.8595380961235,617.167996642145,-39.0808460714569)) ;
#58451=CARTESIAN_POINT('Ctrl Pts',(29.7288648069245,617.174246301298,-39.0748518630524)) ;
#58452=CARTESIAN_POINT('Ctrl Pts',(29.4798107975362,617.186427593269,-39.0394838586637)) ;
#58453=CARTESIAN_POINT('Ctrl Pts',(29.3617340729236,617.192329162083,-39.011916288408)) ;
#58454=CARTESIAN_POINT('Ctrl Pts',(29.1960941755263,617.201307513484,-38.9574586002064)) ;
#58455=CARTESIAN_POINT('Ctrl Pts',(29.1460820623195,617.20411233534,-38.9388286312322)) ;
#58456=CARTESIAN_POINT('Ctrl Pts',(29.0486770461878,617.2097944305,-38.898159699867)) ;
#58457=CARTESIAN_POINT('Ctrl Pts',(29.0012875165223,617.212666733969,-38.8762172113009)) ;
#58458=CARTESIAN_POINT('Ctrl Pts',(28.7960472441117,617.225614690331,-38.771514516949)) ;
#58459=CARTESIAN_POINT('Ctrl Pts',(28.6485375963178,617.236378366049,-38.6702370148164)) ;
#58460=CARTESIAN_POINT('Ctrl Pts',(28.4540009811894,617.252051311751,-38.4956136231043)) ;
#58461=CARTESIAN_POINT('Ctrl Pts',(28.3954659820874,617.256994412151,-38.436268025622)) ;
#58462=CARTESIAN_POINT('Ctrl Pts',(28.3197243948614,617.263537183279,-38.3495147776606)) ;
#58463=CARTESIAN_POINT('Ctrl Pts',(28.2993182099413,617.265316107096,-38.3250138088617)) ;
#58464=CARTESIAN_POINT('Ctrl Pts',(28.2588900992197,617.268856730283,-38.2741090997091)) ;
#58465=CARTESIAN_POINT('Ctrl Pts',(28.2389201579336,617.27061522854,-38.2476764179967)) ;
#58466=CARTESIAN_POINT('Ctrl Pts',(28.1416362127798,617.279295145511,-38.1122194395653)) ;
#58467=CARTESIAN_POINT('Ctrl Pts',(28.0744433992065,617.285684147149,-37.996308591324)) ;
#58468=CARTESIAN_POINT('Ctrl Pts',(27.9687631401648,617.29802012389,-37.7645559045053)) ;
#58469=CARTESIAN_POINT('Ctrl Pts',(27.9283770598511,617.3039306574,-37.6502153177323)) ;
#58470=CARTESIAN_POINT('Ctrl Pts',(27.8851688249047,617.312896547507,-37.4818737544366)) ;
#58471=CARTESIAN_POINT('Ctrl Pts',(27.8740230286492,617.315676119635,-37.4302699809292)) ;
#58472=CARTESIAN_POINT('Ctrl Pts',(27.8557511023794,617.321359702055,-37.3264447772798)) ;
#58473=CARTESIAN_POINT('Ctrl Pts',(27.8486226890249,617.324261256862,-37.2742645895387)) ;
#58474=CARTESIAN_POINT('Ctrl Pts',(27.8338595758887,617.332812085135,-37.1230919061091)) ;
#58475=CARTESIAN_POINT('Ctrl Pts',(27.8313836469252,617.338615415119,-37.0237549811193)) ;
#58476=CARTESIAN_POINT('Ctrl Pts',(27.8411560044508,617.350896607055,-36.8180873847492)) ;
#58477=CARTESIAN_POINT('Ctrl Pts',(27.8545081233521,617.35737442525,-36.7120946622519)) ;
#58478=CARTESIAN_POINT('Ctrl Pts',(27.8881306274189,617.367254916963,-36.5488655668992)) ;
#58479=CARTESIAN_POINT('Ctrl Pts',(27.9028008764859,617.37075559266,-36.4906656854881)) ;
#58480=CARTESIAN_POINT('Ctrl Pts',(27.928591868237,617.37582674508,-36.4044642621942)) ;
#58481=CARTESIAN_POINT('Ctrl Pts',(27.9378138894227,617.377485457928,-36.3759305320441)) ;
#58482=CARTESIAN_POINT('Ctrl Pts',(27.9596413734839,617.381079730528,-36.3131272538345)) ;
#58483=CARTESIAN_POINT('Ctrl Pts',(27.9725415290632,617.382999550098,-36.2789727902339)) ;
#58484=CARTESIAN_POINT('Ctrl Pts',(28.0487700735364,617.393388233787,-36.092352601581)) ;
#58485=CARTESIAN_POINT('Ctrl Pts',(28.1293898941948,617.401109566302,-35.9475922514663)) ;
#58486=CARTESIAN_POINT('Ctrl Pts',(28.2794081723667,617.413602761734,-35.7412085190113)) ;
#58487=CARTESIAN_POINT('Ctrl Pts',(28.3370654608879,617.418096248167,-35.6719507544019)) ;
#58488=CARTESIAN_POINT('Ctrl Pts',(28.4343066963667,617.42542942223,-35.5696262346848)) ;
#58489=CARTESIAN_POINT('Ctrl Pts',(28.4709083876609,617.428141371419,-35.5338831756515)) ;
#58490=CARTESIAN_POINT('Ctrl Pts',(28.5495459472495,617.433896809562,-35.4626254266216)) ;
#58491=CARTESIAN_POINT('Ctrl Pts',(28.5917509012738,617.436947652639,-35.4273592883029)) ;
#58492=CARTESIAN_POINT('Ctrl Pts',(28.759647540145,617.448959362497,-35.2981410543486)) ;
#58493=CARTESIAN_POINT('Ctrl Pts',(28.8945142251436,617.458404099755,-35.2170186846993)) ;
#58494=CARTESIAN_POINT('Ctrl Pts',(29.0948463575378,617.471623183932,-35.1258295400905)) ;
#58495=CARTESIAN_POINT('Ctrl Pts',(29.1536077095088,617.475403672968,-35.1022921382166)) ;
#58496=CARTESIAN_POINT('Ctrl Pts',(29.2560353067579,617.481736148464,-35.0666570952842)) ;
#58497=CARTESIAN_POINT('Ctrl Pts',(29.2991882114397,617.484328380547,-35.053221757059)) ;
#58498=CARTESIAN_POINT('Ctrl Pts',(29.370662057624,617.488460067083,-35.0335297595935)) ;
#58499=CARTESIAN_POINT('Ctrl Pts',(29.398730250739,617.490040619739,-35.0264311268173)) ;
#58500=CARTESIAN_POINT('Ctrl Pts',(29.4698531621015,617.493941723509,-35.0100348535839)) ;
#58501=CARTESIAN_POINT('Ctrl Pts',(29.5130722666402,617.496221999972,-35.0015240268596)) ;
#58502=CARTESIAN_POINT('Ctrl Pts',(29.6903010573981,617.505326967233,-34.972507285805)) ;
#58503=CARTESIAN_POINT('Ctrl Pts',(29.8259155322748,617.511745300934,-34.9638949022875)) ;
#58504=CARTESIAN_POINT('Ctrl Pts',(30.0614098466465,617.523222240443,-34.9722518193884)) ;
#58505=CARTESIAN_POINT('Ctrl Pts',(30.1610210524882,617.528177819032,-34.9831022698607)) ;
#58506=CARTESIAN_POINT('Ctrl Pts',(30.3104304591404,617.536043138459,-35.0105231942293)) ;
#58507=CARTESIAN_POINT('Ctrl Pts',(30.3610465084739,617.538783291811,-35.0218075559155)) ;
#58508=CARTESIAN_POINT('Ctrl Pts',(30.4631846030945,617.544494843745,-35.0486712308223)) ;
#58509=CARTESIAN_POINT('Ctrl Pts',(30.5146293087276,617.547468865616,-35.0643846099378)) ;
#58510=CARTESIAN_POINT('Ctrl Pts',(30.7251790752793,617.560068356588,-35.1378432037574)) ;
#58511=CARTESIAN_POINT('Ctrl Pts',(30.8774438854176,617.570286891645,-35.2131098293127)) ;
#58512=CARTESIAN_POINT('Ctrl Pts',(31.0894716818041,617.585512951448,-35.352757225089)) ;
#58513=CARTESIAN_POINT('Ctrl Pts',(31.1572708861873,617.590545224624,-35.403683800898)) ;
#58514=CARTESIAN_POINT('Ctrl Pts',(31.2460584333802,617.597175873938,-35.4793934037561)) ;
#58515=CARTESIAN_POINT('Ctrl Pts',(31.2698945611658,617.598959928042,-35.500698731266)) ;
#58516=CARTESIAN_POINT('Ctrl Pts',(31.3173271751894,617.602500572974,-35.5451293765081)) ;
#58517=CARTESIAN_POINT('Ctrl Pts',(31.3408824356191,617.604254354984,-35.5682846927383)) ;
#58518=CARTESIAN_POINT('Ctrl Pts',(31.4185112090113,617.610060823034,-35.6483659421535)) ;
#58519=CARTESIAN_POINT('Ctrl Pts',(31.4698810713146,617.613950295082,-35.7078224741377)) ;
#58520=CARTESIAN_POINT('Ctrl Pts',(31.5177255210752,617.617782467769,-35.7700771955494)) ;
#58521=CARTESIAN_POINT('Origin',(29.8885276254223,620.2564904411,-37.0221601717529)) ;
#58522=CARTESIAN_POINT('',(31.5172546949865,618.315547812711,-35.7705124947133)) ;
#58523=CARTESIAN_POINT('',(31.5177255210653,618.256605597193,-35.7700771955364)) ;
#58524=CARTESIAN_POINT('',(31.5177255210695,620.2564904411,-35.7700771955414)) ;
#58525=CARTESIAN_POINT('',(29.8880104657039,618.564640757452,-39.076910106671)) ;
#58526=CARTESIAN_POINT('Ctrl Pts',(29.8879717390109,618.563699092458,-39.076366355844)) ;
#58527=CARTESIAN_POINT('Ctrl Pts',(29.958886902367,618.559625141501,-39.0762487268419)) ;
#58528=CARTESIAN_POINT('Ctrl Pts',(30.029843646248,618.555606320871,-39.0724866387931)) ;
#58529=CARTESIAN_POINT('Ctrl Pts',(30.1004452629841,618.551672025826,-39.0651066485485)) ;
#58530=CARTESIAN_POINT('Ctrl Pts',(30.1710285639294,618.547738751434,-39.0577285728543)) ;
#58531=CARTESIAN_POINT('Ctrl Pts',(30.2412569002453,618.543889988967,-39.0467344870698)) ;
#58532=CARTESIAN_POINT('Ctrl Pts',(30.3107380554495,618.540130523603,-39.032185393595)) ;
#58533=CARTESIAN_POINT('Ctrl Pts',(30.3802249924105,618.536370745402,-39.017635089442)) ;
#58534=CARTESIAN_POINT('Ctrl Pts',(30.4489645533068,618.532700206655,-38.9995290920226)) ;
#58535=CARTESIAN_POINT('Ctrl Pts',(30.5165692974033,618.529099417949,-38.9779635031361)) ;
#58536=CARTESIAN_POINT('Ctrl Pts',(30.5842518358638,618.525494485732,-38.9563730982209)) ;
#58537=CARTESIAN_POINT('Ctrl Pts',(30.6507968126384,618.521959278623,-38.9313149292811)) ;
#58538=CARTESIAN_POINT('Ctrl Pts',(30.7158218297607,618.518451812108,-38.9029228453313)) ;
#58539=CARTESIAN_POINT('Ctrl Pts',(30.7808869631807,618.514942181708,-38.8745132452724)) ;
#58540=CARTESIAN_POINT('Ctrl Pts',(30.8444300254264,618.511459980868,-38.8427653008565)) ;
#58541=CARTESIAN_POINT('Ctrl Pts',(30.9060769860698,618.507944643049,-38.8078544511538)) ;
#58542=CARTESIAN_POINT('Ctrl Pts',(30.9641619067275,618.504632425932,-38.7749607948581)) ;
#58543=CARTESIAN_POINT('Ctrl Pts',(31.0205636933408,618.501290298965,-38.7392587848989)) ;
#58544=CARTESIAN_POINT('Ctrl Pts',(31.0749795173423,618.497857737732,-38.7009343756282)) ;
#58545=CARTESIAN_POINT('Ctrl Pts',(31.0784253563871,618.497640373505,-38.6985075127026)) ;
#58546=CARTESIAN_POINT('Ctrl Pts',(31.081863249142,618.497422646641,-38.6960701328843)) ;
#58547=CARTESIAN_POINT('Ctrl Pts',(31.0852931257368,618.49720454177,-38.6936222827423)) ;
#58548=CARTESIAN_POINT('Ctrl Pts',(31.1220574975077,618.494866705896,-38.6673841163901)) ;
#58549=CARTESIAN_POINT('Ctrl Pts',(31.1578988857675,618.492485205559,-38.6399441114312)) ;
#58550=CARTESIAN_POINT('Ctrl Pts',(31.1927276901434,618.490040470431,-38.6113715191787)) ;
#58551=CARTESIAN_POINT('Ctrl Pts',(31.1927544277232,618.490038593642,-38.6113495844044)) ;
#58552=CARTESIAN_POINT('Ctrl Pts',(31.192781164707,618.490036716816,-38.6113276489626)) ;
#58553=CARTESIAN_POINT('Ctrl Pts',(31.1928079010947,618.490034839953,-38.6113057128533)) ;
#58554=CARTESIAN_POINT('Ctrl Pts',(31.2425623278416,618.486542137522,-38.5704842469339)) ;
#58555=CARTESIAN_POINT('Ctrl Pts',(31.2904310167438,618.482911067368,-38.5271940059014)) ;
#58556=CARTESIAN_POINT('Ctrl Pts',(31.3361841844741,618.47920671304,-38.4816560532498)) ;
#58557=CARTESIAN_POINT('Ctrl Pts',(31.3408223115385,618.478831192241,-38.4770397431421)) ;
#58558=CARTESIAN_POINT('Ctrl Pts',(31.3454386900853,618.478454918342,-38.4724003778938)) ;
#58559=CARTESIAN_POINT('Ctrl Pts',(31.3500330757116,618.478077959143,-38.4677382171815)) ;
#58560=CARTESIAN_POINT('Ctrl Pts',(31.3998725111635,618.473988743479,-38.4171635643799)) ;
#58561=CARTESIAN_POINT('Ctrl Pts',(31.4471254874043,618.469819499512,-38.363900657135)) ;
#58562=CARTESIAN_POINT('Ctrl Pts',(31.4915281287634,618.465644591886,-38.3082689663401)) ;
#58563=CARTESIAN_POINT('Ctrl Pts',(31.5358759040669,618.461474842977,-38.2527060167584)) ;
#58564=CARTESIAN_POINT('Ctrl Pts',(31.5773807165747,618.457299798004,-38.1947803216217)) ;
#58565=CARTESIAN_POINT('Ctrl Pts',(31.6158159408338,618.453174194508,-38.1348275695914)) ;
#58566=CARTESIAN_POINT('Ctrl Pts',(31.6542254806768,618.449051347955,-38.0749148811085)) ;
#58567=CARTESIAN_POINT('Ctrl Pts',(31.6895696959779,618.444978045726,-38.0129779087523)) ;
#58568=CARTESIAN_POINT('Ctrl Pts',(31.7216549625858,618.44098572889,-37.9493672717772)) ;
#58569=CARTESIAN_POINT('Ctrl Pts',(31.7537295713231,618.436994738195,-37.8857777645605)) ;
#58570=CARTESIAN_POINT('Ctrl Pts',(31.7825474111275,618.433084719467,-37.8205157226673)) ;
#58571=CARTESIAN_POINT('Ctrl Pts',(31.8079462877662,618.429262372097,-37.7539464378962)) ;
#58572=CARTESIAN_POINT('Ctrl Pts',(31.8333452633637,618.425440009834,-37.6873768937589)) ;
#58573=CARTESIAN_POINT('Ctrl Pts',(31.8553251400435,618.421705254944,-37.619500095794)) ;
#58574=CARTESIAN_POINT('Ctrl Pts',(31.873755684885,618.418040278261,-37.5506962471976)) ;
#58575=CARTESIAN_POINT('Ctrl Pts',(31.8922046876711,618.414371631152,-37.4818234924653)) ;
#58576=CARTESIAN_POINT('Ctrl Pts',(31.9070970059626,618.410772723826,-37.4120218194748)) ;
#58577=CARTESIAN_POINT('Ctrl Pts',(31.9183366521414,618.407202886512,-37.341687609629)) ;
#58578=CARTESIAN_POINT('Ctrl Pts',(31.9295823506379,618.403631126913,-37.2713155262622)) ;
#58579=CARTESIAN_POINT('Ctrl Pts',(31.9371710513632,618.400088131138,-37.2004103504049)) ;
#58580=CARTESIAN_POINT('Ctrl Pts',(31.9410459640722,618.396514187764,-37.1293841390509)) ;
#58581=CARTESIAN_POINT('Ctrl Pts',(31.9447155325314,618.393129639294,-37.0621218380576)) ;
#58582=CARTESIAN_POINT('Ctrl Pts',(31.945054214817,618.389716845712,-36.9947506530059)) ;
#58583=CARTESIAN_POINT('Ctrl Pts',(31.9420526097717,618.386214585767,-36.9276337594214)) ;
#58584=CARTESIAN_POINT('Ctrl Pts',(31.9418791901511,618.386012240495,-36.9237560386523)) ;
#58585=CARTESIAN_POINT('Ctrl Pts',(31.9416946273324,618.385809596582,-36.919879153918)) ;
#58586=CARTESIAN_POINT('Ctrl Pts',(31.9414989218786,618.385606642221,-36.916003170487)) ;
#58587=CARTESIAN_POINT('Ctrl Pts',(31.9393270093727,618.383354282328,-36.8729880336002)) ;
#58588=CARTESIAN_POINT('Ctrl Pts',(31.9357827578583,618.381063467541,-36.8300859542973)) ;
#58589=CARTESIAN_POINT('Ctrl Pts',(31.9308737538022,618.378717381752,-36.7873942606187)) ;
#58590=CARTESIAN_POINT('Ctrl Pts',(31.9308699800843,618.378715578236,-36.787361442066)) ;
#58591=CARTESIAN_POINT('Ctrl Pts',(31.9308662055602,618.378713774688,-36.7873286236371)) ;
#58592=CARTESIAN_POINT('Ctrl Pts',(31.93086243023,618.378711971107,-36.7872958053321)) ;
#58593=CARTESIAN_POINT('Ctrl Pts',(31.9234657916981,618.375178389614,-36.7229980818359)) ;
#58594=CARTESIAN_POINT('Ctrl Pts',(31.9129413273326,618.371510719047,-36.6589569896053)) ;
#58595=CARTESIAN_POINT('Ctrl Pts',(31.8993521999746,618.367773903285,-36.5954889062645)) ;
#58596=CARTESIAN_POINT('Ctrl Pts',(31.8980251491897,618.36740898329,-36.5892909093221)) ;
#58597=CARTESIAN_POINT('Ctrl Pts',(31.896668901543,618.367043403887,-36.5830984054195)) ;
#58598=CARTESIAN_POINT('Ctrl Pts',(31.8952835353884,618.366677225559,-36.5769117071961)) ;
#58599=CARTESIAN_POINT('Ctrl Pts',(31.8798168048714,618.36258907781,-36.5078411629959)) ;
#58600=CARTESIAN_POINT('Ctrl Pts',(31.8607167866845,618.358427016829,-36.4394904355047)) ;
#58601=CARTESIAN_POINT('Ctrl Pts',(31.8381083273044,618.3542626363,-36.3722470330963)) ;
#58602=CARTESIAN_POINT('Ctrl Pts',(31.8369080392276,618.354041548423,-36.3686770660853)) ;
#58603=CARTESIAN_POINT('Ctrl Pts',(31.8356978697627,618.353820454007,-36.3651102298551)) ;
#58604=CARTESIAN_POINT('Ctrl Pts',(31.8344778401687,618.353599363767,-36.3615465855829)) ;
#58605=CARTESIAN_POINT('Ctrl Pts',(31.8114027137413,618.349417755992,-36.2941453171842)) ;
#58606=CARTESIAN_POINT('Ctrl Pts',(31.7847980465032,618.345237848864,-36.2278817047819)) ;
#58607=CARTESIAN_POINT('Ctrl Pts',(31.7548259193759,618.341112089252,-36.1631277835381)) ;
#58608=CARTESIAN_POINT('Ctrl Pts',(31.7248736523755,618.336989063449,-36.0984167695291)) ;
#58609=CARTESIAN_POINT('Ctrl Pts',(31.6915585194135,618.332920271387,-36.035213352281)) ;
#58610=CARTESIAN_POINT('Ctrl Pts',(31.6550728830991,618.328934767944,-35.9738700195009)) ;
#58611=CARTESIAN_POINT('Ctrl Pts',(31.6185971393183,618.324950345112,-35.9125433190463)) ;
#58612=CARTESIAN_POINT('Ctrl Pts',(31.578952627417,618.321049198024,-35.8530756978182)) ;
#58613=CARTESIAN_POINT('Ctrl Pts',(31.5363610872593,618.317235683044,-35.7958012323473)) ;
#58614=CARTESIAN_POINT('Ctrl Pts',(31.5300565508543,618.316671194323,-35.7873232822356)) ;
#58615=CARTESIAN_POINT('Ctrl Pts',(31.5236874952941,618.316108581474,-35.7788933533313)) ;
#58616=CARTESIAN_POINT('Ctrl Pts',(31.5172546949865,618.315547812711,-35.7705124947133)) ;
#58617=CARTESIAN_POINT('',(27.9033532997491,618.710565160563,-37.5523303889371)) ;
#58618=CARTESIAN_POINT('Ctrl Pts',(27.9033532997491,618.710565160563,-37.5523303889371)) ;
#58619=CARTESIAN_POINT('Ctrl Pts',(27.9220878244754,618.70662834087,-37.6224801187498)) ;
#58620=CARTESIAN_POINT('Ctrl Pts',(27.9445626526125,618.702691521177,-37.6917023881676)) ;
#58621=CARTESIAN_POINT('Ctrl Pts',(27.9706629726565,618.698754701484,-37.75958320921)) ;
#58622=CARTESIAN_POINT('Ctrl Pts',(27.9967424465814,618.694821026098,-37.827409814378)) ;
#58623=CARTESIAN_POINT('Ctrl Pts',(28.0264414901395,618.690887350711,-37.8938966728783)) ;
#58624=CARTESIAN_POINT('Ctrl Pts',(28.0595959262627,618.686953675325,-37.9586463714965)) ;
#58625=CARTESIAN_POINT('Ctrl Pts',(28.0927405975631,618.683021158506,-38.0233769996852)) ;
#58626=CARTESIAN_POINT('Ctrl Pts',(28.1293384354892,618.679088641687,-38.0863710722528)) ;
#58627=CARTESIAN_POINT('Ctrl Pts',(28.1691782036139,618.675156124868,-38.1472535582005)) ;
#58628=CARTESIAN_POINT('Ctrl Pts',(28.2090135524799,618.671224044266,-38.2081292907088)) ;
#58629=CARTESIAN_POINT('Ctrl Pts',(28.252089864984,618.667291963665,-38.2668935165893)) ;
#58630=CARTESIAN_POINT('Ctrl Pts',(28.2981520624203,618.663359883063,-38.3231994221628)) ;
#58631=CARTESIAN_POINT('Ctrl Pts',(28.3442221609708,618.659427127986,-38.3795149859682)) ;
#58632=CARTESIAN_POINT('Ctrl Pts',(28.3932788704584,618.65549437291,-38.4333710351295)) ;
#58633=CARTESIAN_POINT('Ctrl Pts',(28.4450271473054,618.651561617833,-38.4844542366308)) ;
#58634=CARTESIAN_POINT('Ctrl Pts',(28.4967989193162,618.647627077175,-38.5355606313331)) ;
#58635=CARTESIAN_POINT('Ctrl Pts',(28.5512643595028,618.643692536518,-38.5838913532303)) ;
#58636=CARTESIAN_POINT('Ctrl Pts',(28.6080929788375,618.63975799586,-38.6291712726249)) ;
#58637=CARTESIAN_POINT('Ctrl Pts',(28.6650058778057,618.635817620086,-38.6745183443638)) ;
#58638=CARTESIAN_POINT('Ctrl Pts',(28.7242885905112,618.631877244311,-38.716805295332)) ;
#58639=CARTESIAN_POINT('Ctrl Pts',(28.7855794506329,618.627936868536,-38.7557987979462)) ;
#58640=CARTESIAN_POINT('Ctrl Pts',(28.846921413001,618.62399320741,-38.7948248120241)) ;
#58641=CARTESIAN_POINT('Ctrl Pts',(28.9102744564937,618.620049546283,-38.8305516828078)) ;
#58642=CARTESIAN_POINT('Ctrl Pts',(28.9752522709954,618.616105885156,-38.8627920440992)) ;
#58643=CARTESIAN_POINT('Ctrl Pts',(29.0403539253724,618.612154707887,-38.8950938516296)) ;
#58644=CARTESIAN_POINT('Ctrl Pts',(29.1070861114417,618.608203530619,-38.9238956989972)) ;
#58645=CARTESIAN_POINT('Ctrl Pts',(29.175042912625,618.604252353349,-38.9490584895437)) ;
#58646=CARTESIAN_POINT('Ctrl Pts',(29.2031889328429,618.602615873801,-38.9594802927941)) ;
#58647=CARTESIAN_POINT('Ctrl Pts',(29.2315448569522,618.600979394253,-38.9692784442526)) ;
#58648=CARTESIAN_POINT('Ctrl Pts',(29.260081250212,618.599342914705,-38.9784456100224)) ;
#58649=CARTESIAN_POINT('Ctrl Pts',(29.339438239858,618.594792021066,-39.0039386242396)) ;
#58650=CARTESIAN_POINT('Ctrl Pts',(29.4204345692865,618.590241127427,-39.024626781518)) ;
#58651=CARTESIAN_POINT('Ctrl Pts',(29.5025292142112,618.585690233788,-39.0403283483533)) ;
#58652=CARTESIAN_POINT('Ctrl Pts',(29.5837422767609,618.581188210421,-39.055861302186)) ;
#58653=CARTESIAN_POINT('Ctrl Pts',(29.6660300767945,618.576686187055,-39.0665141037531)) ;
#58654=CARTESIAN_POINT('Ctrl Pts',(29.748847668175,618.572184163688,-39.0721570185904)) ;
#58655=CARTESIAN_POINT('Ctrl Pts',(29.7951029245638,618.569669694942,-39.0753086976989)) ;
#58656=CARTESIAN_POINT('Ctrl Pts',(29.841523075707,618.567155226197,-39.0768984062664)) ;
#58657=CARTESIAN_POINT('Ctrl Pts',(29.8880104657039,618.564640757452,-39.076910106671)) ;
#58658=CARTESIAN_POINT('',(27.9019744556529,618.709370847142,-36.4891342933297)) ;
#58659=CARTESIAN_POINT('Origin',(29.888527625422,618.710565160562,-37.0221601717529)) ;
#58660=CARTESIAN_POINT('Ctrl Pts',(27.9039518707378,618.708167248319,-36.4897537138475)) ;
#58661=CARTESIAN_POINT('Ctrl Pts',(27.8958179074389,618.706470116412,-36.5200735308083)) ;
#58662=CARTESIAN_POINT('Ctrl Pts',(27.88837934808,618.704812394634,-36.5505776028213)) ;
#58663=CARTESIAN_POINT('Ctrl Pts',(27.8431917212744,618.693893956545,-36.7562537906378)) ;
#58664=CARTESIAN_POINT('Ctrl Pts',(27.8277943162262,618.685565557881,-36.9355616976458)) ;
#58665=CARTESIAN_POINT('Ctrl Pts',(27.8388765563881,618.673437805429,-37.1816200139386)) ;
#58666=CARTESIAN_POINT('Ctrl Pts',(27.8451738759113,618.670081227285,-37.2484375402449)) ;
#58667=CARTESIAN_POINT('Ctrl Pts',(27.8623906949846,618.663861917327,-37.3680818838262)) ;
#58668=CARTESIAN_POINT('Ctrl Pts',(27.8721429166722,618.661035685576,-37.4210144017641)) ;
#58669=CARTESIAN_POINT('Ctrl Pts',(27.8954255044598,618.655334774255,-37.5244209105406)) ;
#58670=CARTESIAN_POINT('Ctrl Pts',(27.9088257985101,618.652466219825,-37.5748824270022)) ;
#58671=CARTESIAN_POINT('Ctrl Pts',(27.975471419218,618.639712439912,-37.7921325404838)) ;
#58672=CARTESIAN_POINT('Ctrl Pts',(28.047981516357,618.629174682059,-37.9522201124276)) ;
#58673=CARTESIAN_POINT('Ctrl Pts',(28.1835046356398,618.613742648858,-38.1718545375616)) ;
#58674=CARTESIAN_POINT('Ctrl Pts',(28.2313858534902,618.60882149254,-38.2398563278635)) ;
#58675=CARTESIAN_POINT('Ctrl Pts',(28.3031600493299,618.602299103636,-38.3296860172536)) ;
#58676=CARTESIAN_POINT('Ctrl Pts',(28.3236417151513,618.600522194517,-38.3541311144503)) ;
#58677=CARTESIAN_POINT('Ctrl Pts',(28.3666148543829,618.596979225372,-38.4030596555268)) ;
#58678=CARTESIAN_POINT('Ctrl Pts',(28.3891479676044,618.595216809177,-38.4274938656349)) ;
#58679=CARTESIAN_POINT('Ctrl Pts',(28.5045482544813,618.586590899946,-38.5466931796163)) ;
#58680=CARTESIAN_POINT('Ctrl Pts',(28.605856823879,618.58024870474,-38.632862847615)) ;
#58681=CARTESIAN_POINT('Ctrl Pts',(28.7835397226048,618.569773646303,-38.756523992888)) ;
#58682=CARTESIAN_POINT('Ctrl Pts',(28.855162398266,618.565701365462,-38.800128514935)) ;
#58683=CARTESIAN_POINT('Ctrl Pts',(28.9878582775255,618.558183348016,-38.8701822298659)) ;
#58684=CARTESIAN_POINT('Ctrl Pts',(29.0479313401398,618.554789699881,-38.8982698529416)) ;
#58685=CARTESIAN_POINT('Ctrl Pts',(29.1550666372187,618.548684366271,-38.9421820553266)) ;
#58686=CARTESIAN_POINT('Ctrl Pts',(29.2015408390967,618.54601977539,-38.9592966206159)) ;
#58687=CARTESIAN_POINT('Ctrl Pts',(29.3094224135293,618.53977884292,-38.9946543935931)) ;
#58688=CARTESIAN_POINT('Ctrl Pts',(29.3711529176067,618.536167017023,-39.0117376272822)) ;
#58689=CARTESIAN_POINT('Ctrl Pts',(29.5767931540427,618.52400380586,-39.0584282827151)) ;
#58690=CARTESIAN_POINT('Ctrl Pts',(29.7230742455795,618.515108820438,-39.0754947541036)) ;
#58691=CARTESIAN_POINT('Ctrl Pts',(29.946364551797,618.501773289585,-39.0775188879853)) ;
#58692=CARTESIAN_POINT('Ctrl Pts',(30.0228129104608,618.497259917235,-39.0739432896319)) ;
#58693=CARTESIAN_POINT('Ctrl Pts',(30.130186690606,618.491143140938,-39.0628924800165)) ;
#58694=CARTESIAN_POINT('Ctrl Pts',(30.1614084544824,618.48939165761,-39.058952708263)) ;
#58695=CARTESIAN_POINT('Ctrl Pts',(30.225550993546,618.485866526515,-39.0493571541161)) ;
#58696=CARTESIAN_POINT('Ctrl Pts',(30.2584488989828,618.484097910884,-39.0436128409586)) ;
#58697=CARTESIAN_POINT('Ctrl Pts',(30.3993793160701,618.47663573984,-39.0154487994423)) ;
#58698=CARTESIAN_POINT('Ctrl Pts',(30.5056588163018,618.471293284236,-38.985148445248)) ;
#58699=CARTESIAN_POINT('Ctrl Pts',(30.7353702442326,618.459437023411,-38.8991426898609)) ;
#58700=CARTESIAN_POINT('Ctrl Pts',(30.8567623873737,618.452941103242,-38.8394999771351)) ;
#58701=CARTESIAN_POINT('Ctrl Pts',(31.0178742086254,618.443239053318,-38.7395886487558)) ;
#58702=CARTESIAN_POINT('Ctrl Pts',(31.0631484118104,618.440383012865,-38.7089469261163)) ;
#58703=CARTESIAN_POINT('Ctrl Pts',(31.1476668531352,618.434761371185,-38.6466905375196)) ;
#58704=CARTESIAN_POINT('Ctrl Pts',(31.1870754443988,618.432008503317,-38.6153655663368)) ;
#58705=CARTESIAN_POINT('Ctrl Pts',(31.2903263522578,618.424414368095,-38.5269163189289)) ;
#58706=CARTESIAN_POINT('Ctrl Pts',(31.3518070189032,618.419467094685,-38.4672004187941)) ;
#58707=CARTESIAN_POINT('Ctrl Pts',(31.5081110369865,618.405731835566,-38.2951512308979)) ;
#58708=CARTESIAN_POINT('Ctrl Pts',(31.5949044640117,618.396740376852,-38.1762104052946)) ;
#58709=CARTESIAN_POINT('Ctrl Pts',(31.6927471383449,618.385249498457,-38.0066328793852)) ;
#58710=CARTESIAN_POINT('Ctrl Pts',(31.7156934082364,618.382424981604,-37.9633617987878)) ;
#58711=CARTESIAN_POINT('Ctrl Pts',(31.7496755570405,618.378069848645,-37.8933427075535)) ;
#58712=CARTESIAN_POINT('Ctrl Pts',(31.7617294867282,618.376486041313,-37.867113266449)) ;
#58713=CARTESIAN_POINT('Ctrl Pts',(31.7892528263317,618.372776351983,-37.8037352263525)) ;
#58714=CARTESIAN_POINT('Ctrl Pts',(31.8041910090192,618.370679291382,-37.7663712314253)) ;
#58715=CARTESIAN_POINT('Ctrl Pts',(31.8559218303672,618.362997297284,-37.6250771314038)) ;
#58716=CARTESIAN_POINT('Ctrl Pts',(31.8854319324121,618.357697657238,-37.5186738273582)) ;
#58717=CARTESIAN_POINT('Ctrl Pts',(31.9302028257196,618.346233571352,-37.2859991857726)) ;
#58718=CARTESIAN_POINT('Ctrl Pts',(31.9425826302037,618.340072427152,-37.1596482204033)) ;
#58719=CARTESIAN_POINT('Ctrl Pts',(31.9435270491102,618.330824856966,-36.980163630891)) ;
#58720=CARTESIAN_POINT('Ctrl Pts',(31.9417689953612,618.328047330032,-36.9273680621678)) ;
#58721=CARTESIAN_POINT('Ctrl Pts',(31.9342531081693,618.322408310355,-36.8229084803561)) ;
#58722=CARTESIAN_POINT('Ctrl Pts',(31.9285648533262,618.31955107272,-36.771278926938)) ;
#58723=CARTESIAN_POINT('Ctrl Pts',(31.9053256584369,618.310672494464,-36.6150063341292)) ;
#58724=CARTESIAN_POINT('Ctrl Pts',(31.8816250186065,618.304462782732,-36.5114681674261)) ;
#58725=CARTESIAN_POINT('Ctrl Pts',(31.8054832463598,618.289193611457,-36.2673978465648)) ;
#58726=CARTESIAN_POINT('Ctrl Pts',(31.7454550690875,618.280040289192,-36.1298552521645)) ;
#58727=CARTESIAN_POINT('Ctrl Pts',(31.6543331744273,618.269578237659,-35.9709447421512)) ;
#58728=CARTESIAN_POINT('Ctrl Pts',(31.6369330476907,618.267695948273,-35.9422518920512)) ;
#58729=CARTESIAN_POINT('Ctrl Pts',(31.6045713756217,618.264411402832,-35.8917217301505)) ;
#58730=CARTESIAN_POINT('Ctrl Pts',(31.589876761326,618.262993049718,-35.8697243130972)) ;
#58731=CARTESIAN_POINT('Ctrl Pts',(31.5563615310839,618.259901609559,-35.8215917999241)) ;
#58732=CARTESIAN_POINT('Ctrl Pts',(31.5373483985618,618.258240915251,-35.7956102882554)) ;
#58733=CARTESIAN_POINT('Ctrl Pts',(31.5177255210653,618.256605597192,-35.7700771955364)) ;
#58734=CARTESIAN_POINT('Origin',(29.8885276254218,617.710565160562,-37.0221601717529)) ;
#58735=CARTESIAN_POINT('',(30.4641350798567,616.842375533648,-38.5858337721774)) ;
#58736=CARTESIAN_POINT('',(30.4640776578153,616.710565160562,-38.5855853091393)) ;
#58737=CARTESIAN_POINT('',(30.4640776578155,617.710565160562,-38.5855853091393)) ;
#58738=CARTESIAN_POINT('',(31.5536749489399,616.710572711416,-37.0981817538183)) ;
#58739=CARTESIAN_POINT('Origin',(29.8885276254216,616.710565160562,-37.0221601717529)) ;
#58740=CARTESIAN_POINT('Ctrl Pts',(31.5536749650872,616.710572711554,-37.0981817545555)) ;
#58741=CARTESIAN_POINT('Ctrl Pts',(31.5512370248751,616.714176385986,-37.1509048318303)) ;
#58742=CARTESIAN_POINT('Ctrl Pts',(31.5462328618462,616.717877019601,-37.2035994968077)) ;
#58743=CARTESIAN_POINT('Ctrl Pts',(31.538695327451,616.721620562842,-37.2559981327892)) ;
#58744=CARTESIAN_POINT('Ctrl Pts',(31.5300852276339,616.725896799511,-37.3158529158553)) ;
#58745=CARTESIAN_POINT('Ctrl Pts',(31.5181691960903,616.730228465095,-37.375322665228)) ;
#58746=CARTESIAN_POINT('Ctrl Pts',(31.5030344968599,616.734549424273,-37.434030310495)) ;
#58747=CARTESIAN_POINT('Ctrl Pts',(31.4879152270166,616.738865978358,-37.4926781050199)) ;
#58748=CARTESIAN_POINT('Ctrl Pts',(31.4695841279748,616.74317154987,-37.5505654863396)) ;
#58749=CARTESIAN_POINT('Ctrl Pts',(31.448162912522,616.747420965115,-37.6073326424816)) ;
#58750=CARTESIAN_POINT('Ctrl Pts',(31.4267554075257,616.75166766056,-37.6640634653153)) ;
#58751=CARTESIAN_POINT('Ctrl Pts',(31.4022618303736,616.755858153465,-37.719675546723)) ;
#58752=CARTESIAN_POINT('Ctrl Pts',(31.3748356773251,616.759971151056,-37.7738244111941)) ;
#58753=CARTESIAN_POINT('Ctrl Pts',(31.3474166723935,616.764083076671,-37.8279591627703)) ;
#58754=CARTESIAN_POINT('Ctrl Pts',(31.3170665926437,616.768117556839,-37.8806314084233)) ;
#58755=CARTESIAN_POINT('Ctrl Pts',(31.2839704058503,616.772077891308,-37.9315116012041)) ;
#58756=CARTESIAN_POINT('Ctrl Pts',(31.2508463402738,616.776041561791,-37.9824346532384)) ;
#58757=CARTESIAN_POINT('Ctrl Pts',(31.2149714186435,616.779931085611,-38.0315624785175)) ;
#58758=CARTESIAN_POINT('Ctrl Pts',(31.176563855066,616.783773406977,-38.0785809200733)) ;
#58759=CARTESIAN_POINT('Ctrl Pts',(31.1381418667361,616.787617171407,-38.1256170203741)) ;
#58760=CARTESIAN_POINT('Ctrl Pts',(31.0971851356059,616.791413971087,-38.1705418763009)) ;
#58761=CARTESIAN_POINT('Ctrl Pts',(31.053947309258,616.795211484728,-38.2130603820457)) ;
#58762=CARTESIAN_POINT('Ctrl Pts',(31.0106273634846,616.799016210796,-38.2556596410467)) ;
#58763=CARTESIAN_POINT('Ctrl Pts',(30.9650173952862,616.802822127504,-38.2958429243228)) ;
#58764=CARTESIAN_POINT('Ctrl Pts',(30.9174112921772,616.806692422931,-38.3333384864927)) ;
#58765=CARTESIAN_POINT('Ctrl Pts',(30.8746328984004,616.810170233779,-38.3670316438535)) ;
#58766=CARTESIAN_POINT('Ctrl Pts',(30.8302424171979,616.813700617628,-38.3985548429725)) ;
#58767=CARTESIAN_POINT('Ctrl Pts',(30.7844840289367,616.817333919169,-38.4277331502955)) ;
#58768=CARTESIAN_POINT('Ctrl Pts',(30.7803901276804,616.817658982579,-38.4303436685752)) ;
#58769=CARTESIAN_POINT('Ctrl Pts',(30.7762852659941,616.817984869793,-38.43293544994)) ;
#58770=CARTESIAN_POINT('Ctrl Pts',(30.7721696117842,616.818311616863,-38.435508388295)) ;
#58771=CARTESIAN_POINT('Ctrl Pts',(30.7721416414912,616.81831383746,-38.4355258741759)) ;
#58772=CARTESIAN_POINT('Ctrl Pts',(30.7721136706998,616.818316058097,-38.4355433591866)) ;
#58773=CARTESIAN_POINT('Ctrl Pts',(30.77208569941,616.818318278774,-38.435560843327)) ;
#58774=CARTESIAN_POINT('Ctrl Pts',(30.7243139528887,616.822110939553,-38.4654217445811)) ;
#58775=CARTESIAN_POINT('Ctrl Pts',(30.6749216910435,616.826028826852,-38.4928388875168)) ;
#58776=CARTESIAN_POINT('Ctrl Pts',(30.6241889147218,616.830006671409,-38.5176738823377)) ;
#58777=CARTESIAN_POINT('Ctrl Pts',(30.6187932154843,616.830429736229,-38.5203152154626)) ;
#58778=CARTESIAN_POINT('Ctrl Pts',(30.6133824015965,616.830853479251,-38.5229273434151)) ;
#58779=CARTESIAN_POINT('Ctrl Pts',(30.6079568443994,616.831277821956,-38.525510102549)) ;
#58780=CARTESIAN_POINT('Ctrl Pts',(30.5610484595922,616.834946612124,-38.5478401702115)) ;
#58781=CARTESIAN_POINT('Ctrl Pts',(30.5130337497002,616.83866013173,-38.5679758101255)) ;
#58782=CARTESIAN_POINT('Ctrl Pts',(30.4641350798567,616.842375533648,-38.5858337721774)) ;
#58783=CARTESIAN_POINT('Origin',(29.8885276254218,617.710565160562,-37.0221601717529)) ;
#58784=CARTESIAN_POINT('',(30.464077664741,617.544128797339,-38.5855853065898)) ;
#58785=CARTESIAN_POINT('',(30.4640668826956,617.349683543251,-38.5855644985231)) ;
#58786=CARTESIAN_POINT('',(30.4640776578155,617.710565160562,-38.5855853091393)) ;
#58787=CARTESIAN_POINT('',(29.5692971707939,616.710565160562,-38.6572894990045)) ;
#58788=CARTESIAN_POINT('Ctrl Pts',(30.4640668826956,617.349683543251,-38.5855644985231)) ;
#58789=CARTESIAN_POINT('Ctrl Pts',(30.521084074564,617.345357786454,-38.5644138620552)) ;
#58790=CARTESIAN_POINT('Ctrl Pts',(30.5769971533066,617.341054683646,-38.5401308190164)) ;
#58791=CARTESIAN_POINT('Ctrl Pts',(30.6314596324945,617.336815163341,-38.5128750276002)) ;
#58792=CARTESIAN_POINT('Ctrl Pts',(30.6858946674952,617.332577779371,-38.4856329706495)) ;
#58793=CARTESIAN_POINT('Ctrl Pts',(30.738880611153,617.328404005497,-38.4554212210874)) ;
#58794=CARTESIAN_POINT('Ctrl Pts',(30.790088868766,617.324310413416,-38.4224293693333)) ;
#58795=CARTESIAN_POINT('Ctrl Pts',(30.8412903621481,617.320217362068,-38.3894418755581)) ;
#58796=CARTESIAN_POINT('Ctrl Pts',(30.8907145741679,617.316204439522,-38.3536749709813)) ;
#58797=CARTESIAN_POINT('Ctrl Pts',(30.938050556099,617.312263488549,-38.3153482541213)) ;
#58798=CARTESIAN_POINT('Ctrl Pts',(30.9854321660804,617.308318738819,-38.2769845934124)) ;
#58799=CARTESIAN_POINT('Ctrl Pts',(31.0307213402496,617.304445949604,-38.2360560544996)) ;
#58800=CARTESIAN_POINT('Ctrl Pts',(31.073625597012,617.300613507346,-38.1928143189112)) ;
#58801=CARTESIAN_POINT('Ctrl Pts',(31.1165502658891,617.296779241766,-38.1495520106492)) ;
#58802=CARTESIAN_POINT('Ctrl Pts',(31.1570874286128,617.292985051796,-38.1039741089672)) ;
#58803=CARTESIAN_POINT('Ctrl Pts',(31.1949672362993,617.289179237764,-38.0563665633609)) ;
#58804=CARTESIAN_POINT('Ctrl Pts',(31.2329185155416,617.285366242928,-38.0086691919196)) ;
#58805=CARTESIAN_POINT('Ctrl Pts',(31.2682018582335,617.281541054248,-37.9589342907223)) ;
#58806=CARTESIAN_POINT('Ctrl Pts',(31.3005754213143,617.27763777361,-37.9074866807826)) ;
#58807=CARTESIAN_POINT('Ctrl Pts',(31.3266538243606,617.274493500445,-37.8660432503999)) ;
#58808=CARTESIAN_POINT('Ctrl Pts',(31.3508444137161,617.271298092349,-37.8234891432328)) ;
#58809=CARTESIAN_POINT('Ctrl Pts',(31.3730391559108,617.268014866734,-37.7800128089943)) ;
#58810=CARTESIAN_POINT('Ctrl Pts',(31.3730527461205,617.26801285636,-37.7799861877119)) ;
#58811=CARTESIAN_POINT('Ctrl Pts',(31.3730663355829,617.268010845954,-37.7799595660834)) ;
#58812=CARTESIAN_POINT('Ctrl Pts',(31.373079924298,617.268008835514,-37.7799329441086)) ;
#58813=CARTESIAN_POINT('Ctrl Pts',(31.3982667605873,617.264282463299,-37.7305888145781)) ;
#58814=CARTESIAN_POINT('Ctrl Pts',(31.4209704355625,617.260433120364,-37.6798714193184)) ;
#58815=CARTESIAN_POINT('Ctrl Pts',(31.4410752479256,617.256523934734,-37.6280657443909)) ;
#58816=CARTESIAN_POINT('Ctrl Pts',(31.4429546632665,617.256158500663,-37.6232229048535)) ;
#58817=CARTESIAN_POINT('Ctrl Pts',(31.444811375854,617.255792543645,-37.6183705919803)) ;
#58818=CARTESIAN_POINT('Ctrl Pts',(31.4466452965835,617.255426115251,-37.6135090611418)) ;
#58819=CARTESIAN_POINT('Ctrl Pts',(31.4683648172353,617.251086424368,-37.5559328978146)) ;
#58820=CARTESIAN_POINT('Ctrl Pts',(31.4868866525301,617.24668128716,-37.49705784101)) ;
#58821=CARTESIAN_POINT('Ctrl Pts',(31.5021029317602,617.242282244052,-37.4372768729893)) ;
#58822=CARTESIAN_POINT('Ctrl Pts',(31.5170903328867,617.237949369855,-37.3783951099837)) ;
#58823=CARTESIAN_POINT('Ctrl Pts',(31.5288713222752,617.233622692847,-37.3186344993347)) ;
#58824=CARTESIAN_POINT('Ctrl Pts',(31.5373819205906,617.229350066148,-37.2583721573177)) ;
#58825=CARTESIAN_POINT('Ctrl Pts',(31.5458873163396,617.225080051326,-37.1981466539369)) ;
#58826=CARTESIAN_POINT('Ctrl Pts',(31.5511264474828,617.220864156217,-37.1374200208457)) ;
#58827=CARTESIAN_POINT('Ctrl Pts',(31.5530707022731,617.216726391994,-37.0765703636333)) ;
#58828=CARTESIAN_POINT('Ctrl Pts',(31.5550144937777,617.212589613735,-37.0157352059442)) ;
#58829=CARTESIAN_POINT('Ctrl Pts',(31.5536649485285,617.208530932296,-36.9547771031583)) ;
#58830=CARTESIAN_POINT('Ctrl Pts',(31.5490280296545,617.204549585729,-36.8940755273518)) ;
#58831=CARTESIAN_POINT('Ctrl Pts',(31.5442614473403,617.200456907669,-36.8316765366528)) ;
#58832=CARTESIAN_POINT('Ctrl Pts',(31.5360207133408,617.19644594262,-36.769548687579)) ;
#58833=CARTESIAN_POINT('Ctrl Pts',(31.5243519731096,617.192489520133,-36.7081052790211)) ;
#58834=CARTESIAN_POINT('Ctrl Pts',(31.5129859546677,617.188635739,-36.6482558950284)) ;
#58835=CARTESIAN_POINT('Ctrl Pts',(31.4983673621653,617.184833340402,-36.5890560367305)) ;
#58836=CARTESIAN_POINT('Ctrl Pts',(31.4805789942823,617.181035702797,-36.5308871793491)) ;
#58837=CARTESIAN_POINT('Ctrl Pts',(31.4620799650653,617.177086346146,-36.4703944236729)) ;
#58838=CARTESIAN_POINT('Ctrl Pts',(31.4401520065572,617.173141723026,-36.4110170374954)) ;
#58839=CARTESIAN_POINT('Ctrl Pts',(31.4149400476954,617.169131324949,-36.3531800309747)) ;
#58840=CARTESIAN_POINT('Ctrl Pts',(31.3931141943669,617.165659545517,-36.3031108543509)) ;
#58841=CARTESIAN_POINT('Ctrl Pts',(31.3688269891719,617.162137815671,-36.2541951552217)) ;
#58842=CARTESIAN_POINT('Ctrl Pts',(31.3422116372834,617.15851533858,-36.2067052002401)) ;
#58843=CARTESIAN_POINT('Ctrl Pts',(31.3380974627472,617.157955379686,-36.1993642503878)) ;
#58844=CARTESIAN_POINT('Ctrl Pts',(31.3339276743812,617.15739301347,-36.1920572681479)) ;
#58845=CARTESIAN_POINT('Ctrl Pts',(31.3297027792135,617.156828052308,-36.1847851486677)) ;
#58846=CARTESIAN_POINT('Ctrl Pts',(31.3296873928244,617.156825994811,-36.1847586647773)) ;
#58847=CARTESIAN_POINT('Ctrl Pts',(31.3296720057043,617.156823937278,-36.1847321813494)) ;
#58848=CARTESIAN_POINT('Ctrl Pts',(31.3296566178535,617.156821879712,-36.1847056983838)) ;
#58849=CARTESIAN_POINT('Ctrl Pts',(31.3017663989003,617.153092575127,-36.1367057718919)) ;
#58850=CARTESIAN_POINT('Ctrl Pts',(31.2713681144063,617.149240376061,-36.090056891097)) ;
#58851=CARTESIAN_POINT('Ctrl Pts',(31.238639778123,617.145328386154,-36.0450113303155)) ;
#58852=CARTESIAN_POINT('Ctrl Pts',(31.2355817960872,617.144962868189,-36.0408024846696)) ;
#58853=CARTESIAN_POINT('Ctrl Pts',(31.2325035074693,617.144596828241,-36.0366076495894)) ;
#58854=CARTESIAN_POINT('Ctrl Pts',(31.2294050793384,617.144230317784,-36.0324270385321)) ;
#58855=CARTESIAN_POINT('Ctrl Pts',(31.1927794812004,617.139897906588,-35.9830092776272)) ;
#58856=CARTESIAN_POINT('Ctrl Pts',(31.1533343681168,617.135500412305,-35.9355765055245)) ;
#58857=CARTESIAN_POINT('Ctrl Pts',(31.1113410921262,617.131108789479,-35.890430876453)) ;
#58858=CARTESIAN_POINT('Ctrl Pts',(31.0698813712581,617.126772965416,-35.8458588554433)) ;
#58859=CARTESIAN_POINT('Ctrl Pts',(31.0259380743513,617.122443157015,-35.8035158665467)) ;
#58860=CARTESIAN_POINT('Ctrl Pts',(30.9797947503753,617.118167100219,-35.7636606684064)) ;
#58861=CARTESIAN_POINT('Ctrl Pts',(30.9336795843829,617.113893652795,-35.7238297910543)) ;
#58862=CARTESIAN_POINT('Ctrl Pts',(30.8853671327275,617.109674026449,-35.6864835511092)) ;
#58863=CARTESIAN_POINT('Ctrl Pts',(30.8351608804874,617.105532053112,-35.6518515018267)) ;
#58864=CARTESIAN_POINT('Ctrl Pts',(30.7849667375342,617.10139107878,-35.6172278054765)) ;
#58865=CARTESIAN_POINT('Ctrl Pts',(30.7328797036994,617.09732772183,-35.5853170260124)) ;
#58866=CARTESIAN_POINT('Ctrl Pts',(30.6792231421848,617.093340991862,-35.5563204134524)) ;
#58867=CARTESIAN_POINT('Ctrl Pts',(30.6242918057594,617.089259544991,-35.5266348981162)) ;
#58868=CARTESIAN_POINT('Ctrl Pts',(30.5677153525766,617.085258382378,-35.5000039746551)) ;
#58869=CARTESIAN_POINT('Ctrl Pts',(30.5098629151243,617.081310449078,-35.4766113274609)) ;
#58870=CARTESIAN_POINT('Ctrl Pts',(30.4532818035698,617.077449272881,-35.4537327412035)) ;
#58871=CARTESIAN_POINT('Ctrl Pts',(30.3954802001303,617.073638658514,-35.4339518764798)) ;
#58872=CARTESIAN_POINT('Ctrl Pts',(30.336824880697,617.069831848933,-35.4174066351672)) ;
#58873=CARTESIAN_POINT('Ctrl Pts',(30.2761926640822,617.06589673605,-35.4003037591639)) ;
#58874=CARTESIAN_POINT('Ctrl Pts',(30.2146480804883,617.061965258915,-35.3866591106143)) ;
#58875=CARTESIAN_POINT('Ctrl Pts',(30.1526206363921,617.057968154435,-35.3765801825369)) ;
#58876=CARTESIAN_POINT('Ctrl Pts',(30.0986360186937,617.054489336947,-35.3678081448204)) ;
#58877=CARTESIAN_POINT('Ctrl Pts',(30.0442847846414,617.050960158838,-35.3617368033136)) ;
#58878=CARTESIAN_POINT('Ctrl Pts',(29.9898683199497,617.04733002798,-35.3584023356605)) ;
#58879=CARTESIAN_POINT('Ctrl Pts',(29.9817940159459,617.046791389899,-35.3579075680258)) ;
#58880=CARTESIAN_POINT('Ctrl Pts',(29.9737182064909,617.046250529185,-35.3574729939872)) ;
#58881=CARTESIAN_POINT('Ctrl Pts',(29.9656418017626,617.045707280564,-35.3570986677741)) ;
#58882=CARTESIAN_POINT('Ctrl Pts',(29.9656089326697,617.045705069668,-35.3570971443533)) ;
#58883=CARTESIAN_POINT('Ctrl Pts',(29.9655760635669,617.045702858733,-35.3570956219304)) ;
#58884=CARTESIAN_POINT('Ctrl Pts',(29.9655431944543,617.045700647758,-35.3570941005052)) ;
#58885=CARTESIAN_POINT('Ctrl Pts',(29.9100643951679,617.041968808823,-35.3545261321799)) ;
#58886=CARTESIAN_POINT('Ctrl Pts',(29.8543607837217,617.038114620666,-35.3548001091035)) ;
#58887=CARTESIAN_POINT('Ctrl Pts',(29.7987417927496,617.034201555736,-35.357903173981)) ;
#58888=CARTESIAN_POINT('Ctrl Pts',(29.7936860654379,617.033845860876,-35.3581852404043)) ;
#58889=CARTESIAN_POINT('Ctrl Pts',(29.78863106613,617.033489679535,-35.3584906618042)) ;
#58890=CARTESIAN_POINT('Ctrl Pts',(29.7835770441503,617.033133059386,-35.3588194156066)) ;
#58891=CARTESIAN_POINT('Ctrl Pts',(29.7221734369149,617.028800319321,-35.3628135947849)) ;
#58892=CARTESIAN_POINT('Ctrl Pts',(29.6609090204286,617.024403469515,-35.3702550211247)) ;
#58893=CARTESIAN_POINT('Ctrl Pts',(29.6001859470569,617.02001353235,-35.381079378202)) ;
#58894=CARTESIAN_POINT('Ctrl Pts',(29.5403647077876,617.015688792726,-35.3917429763815)) ;
#58895=CARTESIAN_POINT('Ctrl Pts',(29.4810686797287,617.011371040941,-35.4056893581065)) ;
#58896=CARTESIAN_POINT('Ctrl Pts',(29.4226677322369,617.007107434284,-35.4228208822698)) ;
#58897=CARTESIAN_POINT('Ctrl Pts',(29.3643007018345,617.002846303771,-35.4399424570837)) ;
#58898=CARTESIAN_POINT('Ctrl Pts',(29.3068276492842,616.998639386775,-35.4602453669685)) ;
#58899=CARTESIAN_POINT('Ctrl Pts',(29.2506048261699,616.994509838509,-35.4835993866685)) ;
#58900=CARTESIAN_POINT('Ctrl Pts',(29.1943936706659,616.990381147224,-35.5069485598384)) ;
#58901=CARTESIAN_POINT('Ctrl Pts',(29.1394322573245,616.986329792316,-35.5333475998383)) ;
#58902=CARTESIAN_POINT('Ctrl Pts',(29.0860638811723,616.982354047787,-35.5626341994198)) ;
#58903=CARTESIAN_POINT('Ctrl Pts',(29.0312260496663,616.978268834327,-35.5927271819878)) ;
#58904=CARTESIAN_POINT('Ctrl Pts',(28.9780703963664,616.97426343898,-35.6258692258559)) ;
#58905=CARTESIAN_POINT('Ctrl Pts',(28.9269540427023,616.970309623841,-35.6618476287035)) ;
#58906=CARTESIAN_POINT('Ctrl Pts',(28.8771392174126,616.966456481036,-35.6969099467992)) ;
#58907=CARTESIAN_POINT('Ctrl Pts',(28.8292613449351,616.962651954101,-35.7346660907345)) ;
#58908=CARTESIAN_POINT('Ctrl Pts',(28.7836339573324,616.958848414507,-35.7748826535162)) ;
#58909=CARTESIAN_POINT('Ctrl Pts',(28.7362183870171,616.954895810413,-35.816675343403)) ;
#58910=CARTESIAN_POINT('Ctrl Pts',(28.6912338124573,616.950943843878,-35.8611256952804)) ;
#58911=CARTESIAN_POINT('Ctrl Pts',(28.649007039024,616.946921188459,-35.9079260438706)) ;
#58912=CARTESIAN_POINT('Ctrl Pts',(28.612563757972,616.943449486738,-35.9483164909338)) ;
#58913=CARTESIAN_POINT('Ctrl Pts',(28.5781738025082,616.939924470793,-35.9904578913708)) ;
#58914=CARTESIAN_POINT('Ctrl Pts',(28.5460281467764,616.936295530328,-36.0341183434806)) ;
#58915=CARTESIAN_POINT('Ctrl Pts',(28.540947446731,616.935721967352,-36.0410189854481)) ;
#58916=CARTESIAN_POINT('Ctrl Pts',(28.5359227081795,616.93514580828,-36.0479576011575)) ;
#58917=CARTESIAN_POINT('Ctrl Pts',(28.5309545704018,616.934566853292,-36.05493330865)) ;
#58918=CARTESIAN_POINT('Ctrl Pts',(28.5309342646271,616.934564486987,-36.0549618197645)) ;
#58919=CARTESIAN_POINT('Ctrl Pts',(28.5309139597978,616.934562120636,-36.0549903314986)) ;
#58920=CARTESIAN_POINT('Ctrl Pts',(28.530893655914,616.934559754237,-36.0550188438523)) ;
#58921=CARTESIAN_POINT('Ctrl Pts',(28.4989996356354,616.930842536283,-36.0998070033906)) ;
#58922=CARTESIAN_POINT('Ctrl Pts',(28.4693258899516,616.926999768579,-36.1462970726815)) ;
#58923=CARTESIAN_POINT('Ctrl Pts',(28.4420269705331,616.923094265841,-36.1942290788419)) ;
#58924=CARTESIAN_POINT('Ctrl Pts',(28.4393659813779,616.922713573101,-36.1989012985231)) ;
#58925=CARTESIAN_POINT('Ctrl Pts',(28.4367275537249,616.922332284279,-36.2035871781143)) ;
#58926=CARTESIAN_POINT('Ctrl Pts',(28.434111828081,616.921950457554,-36.208286450564)) ;
#58927=CARTESIAN_POINT('Ctrl Pts',(28.4041867740043,616.917582191555,-36.262048198287)) ;
#58928=CARTESIAN_POINT('Ctrl Pts',(28.3772331276111,616.913144219065,-36.3175689997004)) ;
#58929=CARTESIAN_POINT('Ctrl Pts',(28.3534166267093,616.908709835501,-36.3744743718786)) ;
#58930=CARTESIAN_POINT('Ctrl Pts',(28.3300446441918,616.904358216615,-36.4303176449596)) ;
#58931=CARTESIAN_POINT('Ctrl Pts',(28.3096933215118,616.900010337835,-36.4874941931902)) ;
#58932=CARTESIAN_POINT('Ctrl Pts',(28.2924806010451,616.895715230285,-36.5456427183914)) ;
#58933=CARTESIAN_POINT('Ctrl Pts',(28.2752787466916,616.891422834166,-36.6037545353646)) ;
#58934=CARTESIAN_POINT('Ctrl Pts',(28.2612113991684,616.887183285358,-36.6628370886462)) ;
#58935=CARTESIAN_POINT('Ctrl Pts',(28.2503615449872,616.883021951294,-36.7225229685776)) ;
#58936=CARTESIAN_POINT('Ctrl Pts',(28.2395144151561,616.878861662123,-36.7821938616503)) ;
#58937=CARTESIAN_POINT('Ctrl Pts',(28.2318831900086,616.874779559,-36.8424677555916)) ;
#58938=CARTESIAN_POINT('Ctrl Pts',(28.2275168206484,616.870776310009,-36.9029709682656)) ;
#58939=CARTESIAN_POINT('Ctrl Pts',(28.2229994847329,616.866634649294,-36.9655660703)) ;
#58940=CARTESIAN_POINT('Ctrl Pts',(28.2219770714696,616.862577421011,-37.0284066053647)) ;
#58941=CARTESIAN_POINT('Ctrl Pts',(28.2244639128333,616.858578369016,-37.0910719989216)) ;
#58942=CARTESIAN_POINT('Ctrl Pts',(28.2268707964393,616.854707895882,-37.1517225537264)) ;
#58943=CARTESIAN_POINT('Ctrl Pts',(28.2325649901524,616.85089153798,-37.2122089216034)) ;
#58944=CARTESIAN_POINT('Ctrl Pts',(28.2415198331724,616.847083689211,-37.2721447271132)) ;
#58945=CARTESIAN_POINT('Ctrl Pts',(28.2509209020711,616.843086092765,-37.3350671743111)) ;
#58946=CARTESIAN_POINT('Ctrl Pts',(28.2639166266811,616.839097499273,-37.3973826024798)) ;
#58947=CARTESIAN_POINT('Ctrl Pts',(28.2804231555915,616.835045936516,-37.4586406500308)) ;
#58948=CARTESIAN_POINT('Ctrl Pts',(28.2946495273849,616.83155404319,-37.5114367142142)) ;
#58949=CARTESIAN_POINT('Ctrl Pts',(28.3114838637982,616.828014712853,-37.5634483508293)) ;
#58950=CARTESIAN_POINT('Ctrl Pts',(28.3308327387374,616.82437615812,-37.6143849965462)) ;
#58951=CARTESIAN_POINT('Ctrl Pts',(28.3339272689223,616.823794231911,-37.6225314643995)) ;
#58952=CARTESIAN_POINT('Ctrl Pts',(28.3370860862066,616.823209767673,-37.6306505391174)) ;
#58953=CARTESIAN_POINT('Ctrl Pts',(28.3403087758142,616.822622553551,-37.6387411517518)) ;
#58954=CARTESIAN_POINT('Ctrl Pts',(28.3403156962882,616.822621292555,-37.6387585257097)) ;
#58955=CARTESIAN_POINT('Ctrl Pts',(28.3403226170566,616.822620031546,-37.6387758995365)) ;
#58956=CARTESIAN_POINT('Ctrl Pts',(28.3403295381196,616.822618770524,-37.6387932732319)) ;
#58957=CARTESIAN_POINT('Ctrl Pts',(28.3611300540204,616.818828904217,-37.6910080601294)) ;
#58958=CARTESIAN_POINT('Ctrl Pts',(28.3846714076599,616.814914584974,-37.7422176702767)) ;
#58959=CARTESIAN_POINT('Ctrl Pts',(28.4108107263033,616.810938157239,-37.7921428459409)) ;
#58960=CARTESIAN_POINT('Ctrl Pts',(28.4134417842094,616.810537909177,-37.7971680736424)) ;
#58961=CARTESIAN_POINT('Ctrl Pts',(28.416099125224,616.810137031865,-37.8021802670086)) ;
#58962=CARTESIAN_POINT('Ctrl Pts',(28.4187825777852,616.80973558888,-37.8071791277746)) ;
#58963=CARTESIAN_POINT('Ctrl Pts',(28.448063689259,616.805355151177,-37.8617253498502)) ;
#58964=CARTESIAN_POINT('Ctrl Pts',(28.480458763619,616.800907997258,-37.9146874851851)) ;
#58965=CARTESIAN_POINT('Ctrl Pts',(28.5157431936671,616.796463345162,-37.9657275419637)) ;
#58966=CARTESIAN_POINT('Ctrl Pts',(28.5509838970871,616.792024201152,-38.0167043467759)) ;
#58967=CARTESIAN_POINT('Ctrl Pts',(28.5891065722251,616.787587893215,-38.0657641391842)) ;
#58968=CARTESIAN_POINT('Ctrl Pts',(28.6298609711957,616.783202799171,-38.1125984677305)) ;
#58969=CARTESIAN_POINT('Ctrl Pts',(28.6705776712394,616.778821761458,-38.1593894732498)) ;
#58970=CARTESIAN_POINT('Ctrl Pts',(28.713921186153,616.774491979344,-38.2039592709164)) ;
#58971=CARTESIAN_POINT('Ctrl Pts',(28.7596174176482,616.770237644049,-38.2460251560201)) ;
#58972=CARTESIAN_POINT('Ctrl Pts',(28.8052857253946,616.765985908465,-38.2880653357831)) ;
#58973=CARTESIAN_POINT('Ctrl Pts',(28.8533039277465,616.761809520445,-38.3276046412806)) ;
#58974=CARTESIAN_POINT('Ctrl Pts',(28.903373768419,616.757707658521,-38.3643848801307)) ;
#58975=CARTESIAN_POINT('Ctrl Pts',(28.9534480750791,616.753605430732,-38.4011683996002)) ;
#58976=CARTESIAN_POINT('Ctrl Pts',(29.0055744969324,616.749577607991,-38.4351921860378)) ;
#58977=CARTESIAN_POINT('Ctrl Pts',(29.0594287737958,616.745599436479,-38.4662234489906)) ;
#58978=CARTESIAN_POINT('Ctrl Pts',(29.113280978284,616.741621418052,-38.4972535178244)) ;
#58979=CARTESIAN_POINT('Ctrl Pts',(29.1688610436538,616.73769275453,-38.5252909485167)) ;
#58980=CARTESIAN_POINT('Ctrl Pts',(29.225816917922,616.733767924342,-38.5501323001247)) ;
#58981=CARTESIAN_POINT('Ctrl Pts',(29.2828293655759,616.729839195681,-38.5749983262617)) ;
#58982=CARTESIAN_POINT('Ctrl Pts',(29.3412204591112,616.72591380392,-38.5966613468097)) ;
#58983=CARTESIAN_POINT('Ctrl Pts',(29.4006072854367,616.721931192345,-38.614953546914)) ;
#58984=CARTESIAN_POINT('Ctrl Pts',(29.4560806936032,616.718211023225,-38.6320403445327)) ;
#58985=CARTESIAN_POINT('Ctrl Pts',(29.5124225672536,616.714440274229,-38.6461857255948)) ;
#58986=CARTESIAN_POINT('Ctrl Pts',(29.5692971707936,616.710565160562,-38.6572894990042)) ;
#58987=CARTESIAN_POINT('Origin',(29.8885276254216,616.710565160562,-37.0221601717529)) ;
#58988=CARTESIAN_POINT('Ctrl Pts',(30.4640776716666,617.544128797339,-38.5855853040402)) ;
#58989=CARTESIAN_POINT('Ctrl Pts',(30.4870886073976,617.542498162509,-38.5771141947747)) ;
#58990=CARTESIAN_POINT('Ctrl Pts',(30.5099115798872,617.540850531879,-38.5681354130923)) ;
#58991=CARTESIAN_POINT('Ctrl Pts',(30.5976250051638,617.534394017862,-38.5313714471249)) ;
#58992=CARTESIAN_POINT('Ctrl Pts',(30.660911230605,617.529463405148,-38.4999825094059)) ;
#58993=CARTESIAN_POINT('Ctrl Pts',(30.8129108067211,617.51693396129,-38.4121577697486)) ;
#58994=CARTESIAN_POINT('Ctrl Pts',(30.8986404385462,617.509222910576,-38.3511624079992)) ;
#58995=CARTESIAN_POINT('Ctrl Pts',(31.0204908109826,617.49757869963,-38.2458277171379)) ;
#58996=CARTESIAN_POINT('Ctrl Pts',(31.0610538744134,617.493569625233,-38.2070172974096)) ;
#58997=CARTESIAN_POINT('Ctrl Pts',(31.120283128478,617.487597464982,-38.1443200794749)) ;
#58998=CARTESIAN_POINT('Ctrl Pts',(31.1403849618483,617.485549086919,-38.1218502411609)) ;
#58999=CARTESIAN_POINT('Ctrl Pts',(31.1872890121697,617.480729435838,-38.066466099345)) ;
#59000=CARTESIAN_POINT('Ctrl Pts',(31.2134640920881,617.477998173657,-38.0330509294253)) ;
#59001=CARTESIAN_POINT('Ctrl Pts',(31.2740490641244,617.471469895617,-37.9493055050781)) ;
#59002=CARTESIAN_POINT('Ctrl Pts',(31.3070285931238,617.467731322031,-37.8980163920712)) ;
#59003=CARTESIAN_POINT('Ctrl Pts',(31.3976063361618,617.456522781782,-37.738561859865)) ;
#59004=CARTESIAN_POINT('Ctrl Pts',(31.4461583310577,617.449102357673,-37.6257601040785)) ;
#59005=CARTESIAN_POINT('Ctrl Pts',(31.49695302564,617.437936044848,-37.4593979861534)) ;
#59006=CARTESIAN_POINT('Ctrl Pts',(31.5097002534967,617.434563236637,-37.4094682140154)) ;
#59007=CARTESIAN_POINT('Ctrl Pts',(31.5318042219605,617.42723820241,-37.3024112279107)) ;
#59008=CARTESIAN_POINT('Ctrl Pts',(31.5405380584223,617.423270257557,-37.2452268023006)) ;
#59009=CARTESIAN_POINT('Ctrl Pts',(31.5530848136482,617.414415644119,-37.1195881523293)) ;
#59010=CARTESIAN_POINT('Ctrl Pts',(31.5556816478247,617.409501703735,-37.0511186579818)) ;
#59011=CARTESIAN_POINT('Ctrl Pts',(31.551364639642,617.396283137486,-36.8689534061587)) ;
#59012=CARTESIAN_POINT('Ctrl Pts',(31.5370261938174,617.387906413662,-36.7557870216662)) ;
#59013=CARTESIAN_POINT('Ctrl Pts',(31.5040345977418,617.377735721192,-36.6138550900405)) ;
#59014=CARTESIAN_POINT('Ctrl Pts',(31.4959103809542,617.375544949996,-36.5829596299875)) ;
#59015=CARTESIAN_POINT('Ctrl Pts',(31.4765274013552,617.370944982721,-36.5170207832697)) ;
#59016=CARTESIAN_POINT('Ctrl Pts',(31.4649863835773,617.368550943906,-36.482079237073)) ;
#59017=CARTESIAN_POINT('Ctrl Pts',(31.4160475315186,617.359491463879,-36.348896047106)) ;
#59018=CARTESIAN_POINT('Ctrl Pts',(31.3705412875037,617.353157847879,-36.253888274902)) ;
#59019=CARTESIAN_POINT('Ctrl Pts',(31.2682944591186,617.341021908365,-36.083805167669)) ;
#59020=CARTESIAN_POINT('Ctrl Pts',(31.2135776528049,617.335260542601,-36.0080073074761)) ;
#59021=CARTESIAN_POINT('Ctrl Pts',(31.1199800046529,617.32600613038,-35.8989407106407)) ;
#59022=CARTESIAN_POINT('Ctrl Pts',(31.085436789944,617.322695776807,-35.8622013548397)) ;
#59023=CARTESIAN_POINT('Ctrl Pts',(31.0066504752701,617.315318776738,-35.785677373248)) ;
#59024=CARTESIAN_POINT('Ctrl Pts',(30.9618365196369,617.311227645608,-35.746583875975)) ;
#59025=CARTESIAN_POINT('Ctrl Pts',(30.8580545427131,617.301959437935,-35.6653966623566)) ;
#59026=CARTESIAN_POINT('Ctrl Pts',(30.7982369156724,617.296747847191,-35.6245848501746)) ;
#59027=CARTESIAN_POINT('Ctrl Pts',(30.6425297205435,617.283604867001,-35.5325918978048)) ;
#59028=CARTESIAN_POINT('Ctrl Pts',(30.5439205953216,617.275637758637,-35.4866484003713)) ;
#59029=CARTESIAN_POINT('Ctrl Pts',(30.412278357908,617.265930567536,-35.4403247633842)) ;
#59030=CARTESIAN_POINT('Ctrl Pts',(30.3827336529789,617.263811058756,-35.4308465257249)) ;
#59031=CARTESIAN_POINT('Ctrl Pts',(30.3155656254478,617.25914548512,-35.4113502077275)) ;
#59032=CARTESIAN_POINT('Ctrl Pts',(30.2778229749583,617.256624228392,-35.4018145475948)) ;
#59033=CARTESIAN_POINT('Ctrl Pts',(30.1884327320442,617.250811724477,-35.3825346584289)) ;
#59034=CARTESIAN_POINT('Ctrl Pts',(30.1365894251518,617.247562366096,-35.3738941068678)) ;
#59035=CARTESIAN_POINT('Ctrl Pts',(29.9487586834912,617.23595861954,-35.3516540917144)) ;
#59036=CARTESIAN_POINT('Ctrl Pts',(29.8116487772101,617.227755495534,-35.352338267726)) ;
#59037=CARTESIAN_POINT('Ctrl Pts',(29.6248758931455,617.215677846966,-35.3763419584364)) ;
#59038=CARTESIAN_POINT('Ctrl Pts',(29.5739286708588,617.212295000644,-35.385316760625)) ;
#59039=CARTESIAN_POINT('Ctrl Pts',(29.4675158041588,617.204992700149,-35.4092139180621)) ;
#59040=CARTESIAN_POINT('Ctrl Pts',(29.4122395552297,617.201059631714,-35.4246637422172)) ;
#59041=CARTESIAN_POINT('Ctrl Pts',(29.2939847461709,617.192319808958,-35.4643997058494)) ;
#59042=CARTESIAN_POINT('Ctrl Pts',(29.2314621985705,617.187487711256,-35.4897234637654)) ;
#59043=CARTESIAN_POINT('Ctrl Pts',(29.0648593524841,617.174104739204,-35.5692767664972)) ;
#59044=CARTESIAN_POINT('Ctrl Pts',(28.9646911415418,617.165465063662,-35.6308195405618)) ;
#59045=CARTESIAN_POINT('Ctrl Pts',(28.8467753484453,617.15508972846,-35.7216576232664)) ;
#59046=CARTESIAN_POINT('Ctrl Pts',(28.8222907732495,617.152925045025,-35.7416546882143)) ;
#59047=CARTESIAN_POINT('Ctrl Pts',(28.7699301968425,617.148296699119,-35.7869630925057)) ;
#59048=CARTESIAN_POINT('Ctrl Pts',(28.7423139543213,617.145851855969,-35.8125458436048)) ;
#59049=CARTESIAN_POINT('Ctrl Pts',(28.6802983183195,617.140285778908,-35.8740282239296)) ;
#59050=CARTESIAN_POINT('Ctrl Pts',(28.6465914251868,617.137201230933,-35.9105756221166)) ;
#59051=CARTESIAN_POINT('Ctrl Pts',(28.5176323076652,617.124896791614,-36.0636042640291)) ;
#59052=CARTESIAN_POINT('Ctrl Pts',(28.4367314832795,617.115900369978,-36.1912158425178)) ;
#59053=CARTESIAN_POINT('Ctrl Pts',(28.3530185123571,617.102925574984,-36.3738420434138)) ;
#59054=CARTESIAN_POINT('Ctrl Pts',(28.3340811954692,617.099599431862,-36.4206620424088)) ;
#59055=CARTESIAN_POINT('Ctrl Pts',(28.2967020748125,617.092024017412,-36.5266950412998)) ;
#59056=CARTESIAN_POINT('Ctrl Pts',(28.2793821606208,617.087741875056,-36.5862204813015)) ;
#59057=CARTESIAN_POINT('Ctrl Pts',(28.2289550007918,617.071942889591,-36.8041385018246)) ;
#59058=CARTESIAN_POINT('Ctrl Pts',(28.2156358069072,617.059870181053,-36.9661528427404)) ;
#59059=CARTESIAN_POINT('Ctrl Pts',(28.2281399435907,617.045929972079,-37.1634557467531)) ;
#59060=CARTESIAN_POINT('Ctrl Pts',(28.231580517554,617.043433705033,-37.1992999385523)) ;
#59061=CARTESIAN_POINT('Ctrl Pts',(28.2403058126092,617.038819791819,-37.2670348364461)) ;
#59062=CARTESIAN_POINT('Ctrl Pts',(28.2453618284591,617.036693075322,-37.2989364693367)) ;
#59063=CARTESIAN_POINT('Ctrl Pts',(28.2585259665357,617.032099508037,-37.3687946786095)) ;
#59064=CARTESIAN_POINT('Ctrl Pts',(28.2670395693494,617.029651298592,-37.4066570143532)) ;
#59065=CARTESIAN_POINT('Ctrl Pts',(28.3006255818359,617.021395066578,-37.5349161828583)) ;
#59066=CARTESIAN_POINT('Ctrl Pts',(28.3320023335011,617.015749891101,-37.6234771640302)) ;
#59067=CARTESIAN_POINT('Ctrl Pts',(28.4044325190586,617.004956760119,-37.7835583937137)) ;
#59068=CARTESIAN_POINT('Ctrl Pts',(28.4436523053243,616.999851902999,-37.8555858466508)) ;
#59069=CARTESIAN_POINT('Ctrl Pts',(28.5151216221253,616.991317092595,-37.966521728796)) ;
#59070=CARTESIAN_POINT('Ctrl Pts',(28.5441181483823,616.988013561413,-38.0073632187489)) ;
#59071=CARTESIAN_POINT('Ctrl Pts',(28.613441705303,616.980408985052,-38.0962352706777)) ;
#59072=CARTESIAN_POINT('Ctrl Pts',(28.6547275293901,616.97607115754,-38.1434170302327)) ;
#59073=CARTESIAN_POINT('Ctrl Pts',(28.779915770761,616.96341450797,-38.2711780970165)) ;
#59074=CARTESIAN_POINT('Ctrl Pts',(28.8697239072827,616.954876062616,-38.3454513757762)) ;
#59075=CARTESIAN_POINT('Ctrl Pts',(29.0150749100818,616.942224296778,-38.442031868612)) ;
#59076=CARTESIAN_POINT('Ctrl Pts',(29.0653010087839,616.938040557698,-38.4717306523879)) ;
#59077=CARTESIAN_POINT('Ctrl Pts',(29.1442432960397,616.931847911846,-38.5129796347347)) ;
#59078=CARTESIAN_POINT('Ctrl Pts',(29.1718933303721,616.929748206103,-38.5264665690584)) ;
#59079=CARTESIAN_POINT('Ctrl Pts',(29.2364771420603,616.925019053216,-38.5557830506843)) ;
#59080=CARTESIAN_POINT('Ctrl Pts',(29.2736396780909,616.922419203892,-38.5710573407325)) ;
#59081=CARTESIAN_POINT('Ctrl Pts',(29.3631528456667,616.916358122219,-38.6041179052323)) ;
#59082=CARTESIAN_POINT('Ctrl Pts',(29.4159079588574,616.912943380221,-38.6206721111095)) ;
#59083=CARTESIAN_POINT('Ctrl Pts',(29.6014600615896,616.901175595285,-38.6689051125641)) ;
#59084=CARTESIAN_POINT('Ctrl Pts',(29.7372310334632,616.892937798099,-38.6868770490437)) ;
#59085=CARTESIAN_POINT('Ctrl Pts',(29.9247134127121,616.880839787882,-38.6885491645884)) ;
#59086=CARTESIAN_POINT('Ctrl Pts',(29.9757459591647,616.877480072484,-38.6866582045623)) ;
#59087=CARTESIAN_POINT('Ctrl Pts',(30.0875067893749,616.869930109791,-38.6773634004201)) ;
#59088=CARTESIAN_POINT('Ctrl Pts',(30.1480740184896,616.86571182508,-38.668952337198)) ;
#59089=CARTESIAN_POINT('Ctrl Pts',(30.2951511863831,616.855140363488,-38.6402121081937)) ;
#59090=CARTESIAN_POINT('Ctrl Pts',(30.380757274049,616.848696268288,-38.6162559893195)) ;
#59091=CARTESIAN_POINT('Ctrl Pts',(30.4640381476845,616.84223029543,-38.585599853597)) ;
#59092=CARTESIAN_POINT('Origin',(29.8885276254218,617.710565160562,-37.0221601717529)) ;
#59093=CARTESIAN_POINT('',(30.4640776731091,618.242171074983,-38.5855853035092)) ;
#59094=CARTESIAN_POINT('',(30.4640776576043,618.051524931058,-38.5855853092171)) ;
#59095=CARTESIAN_POINT('',(30.4640776578155,617.710565160562,-38.5855853091393)) ;
#59096=CARTESIAN_POINT('',(29.8896085855951,618.281230024789,-38.6886301592882)) ;
#59097=CARTESIAN_POINT('Ctrl Pts',(29.889588780989,618.280960192427,-38.6881598338024)) ;
#59098=CARTESIAN_POINT('Ctrl Pts',(29.9346123899361,618.277705627339,-38.6881311560935)) ;
#59099=CARTESIAN_POINT('Ctrl Pts',(29.9796197792924,618.274477707997,-38.6862773372091)) ;
#59100=CARTESIAN_POINT('Ctrl Pts',(30.0545924905335,618.269194666625,-38.6801378871634)) ;
#59101=CARTESIAN_POINT('Ctrl Pts',(30.0846152551122,618.267104597096,-38.676855790806)) ;
#59102=CARTESIAN_POINT('Ctrl Pts',(30.1454735976508,618.262941509797,-38.6685228094867)) ;
#59103=CARTESIAN_POINT('Ctrl Pts',(30.1762873146518,618.260876176576,-38.6634175088081)) ;
#59104=CARTESIAN_POINT('Ctrl Pts',(30.2944515861005,618.253067360093,-38.6404092731344)) ;
#59105=CARTESIAN_POINT('Ctrl Pts',(30.3804395485023,618.247609791015,-38.6163753462388)) ;
#59106=CARTESIAN_POINT('Ctrl Pts',(30.4640776731659,618.242171075974,-38.5855853034883)) ;
#59107=CARTESIAN_POINT('',(30.9678862784725,618.710565160562,-35.7530892919022)) ;
#59108=CARTESIAN_POINT('Ctrl Pts',(29.8896085855951,618.281230024788,-38.6886301592882)) ;
#59109=CARTESIAN_POINT('Ctrl Pts',(29.8297449858523,618.285479107441,-38.6885353801434)) ;
#59110=CARTESIAN_POINT('Ctrl Pts',(29.7697812032065,618.289767378033,-38.6851881605191)) ;
#59111=CARTESIAN_POINT('Ctrl Pts',(29.7100945358446,618.294034879536,-38.678613355152)) ;
#59112=CARTESIAN_POINT('Ctrl Pts',(29.6504725284024,618.298297757958,-38.6720456724206)) ;
#59113=CARTESIAN_POINT('Ctrl Pts',(29.5911270001335,618.302539653761,-38.6622576307303)) ;
#59114=CARTESIAN_POINT('Ctrl Pts',(29.5324254623936,618.306721098468,-38.6493109448699)) ;
#59115=CARTESIAN_POINT('Ctrl Pts',(29.4737645016973,618.31089965278,-38.6363732083192)) ;
#59116=CARTESIAN_POINT('Ctrl Pts',(29.4157466608234,618.315017741293,-38.620281262818)) ;
#59117=CARTESIAN_POINT('Ctrl Pts',(29.3587302988432,618.319058873962,-38.601131373573)) ;
#59118=CARTESIAN_POINT('Ctrl Pts',(29.30173080255,618.323098811247,-38.5819871489481)) ;
#59119=CARTESIAN_POINT('Ctrl Pts',(29.2457322858195,618.327061860551,-38.559786746764)) ;
#59120=CARTESIAN_POINT('Ctrl Pts',(29.1910835605629,618.330954988191,-38.5346608511779)) ;
#59121=CARTESIAN_POINT('Ctrl Pts',(29.1363907934061,618.334851253337,-38.5095147064062)) ;
#59122=CARTESIAN_POINT('Ctrl Pts',(29.0830501679372,618.33867762189,-38.4814382115276)) ;
#59123=CARTESIAN_POINT('Ctrl Pts',(29.0314001022382,618.342463380071,-38.4505983134762)) ;
#59124=CARTESIAN_POINT('Ctrl Pts',(28.9797307970573,618.346250548434,-38.4197469276628)) ;
#59125=CARTESIAN_POINT('Ctrl Pts',(28.9297535935047,618.349997366089,-38.3861298563673)) ;
#59126=CARTESIAN_POINT('Ctrl Pts',(28.8817926756802,618.353752293416,-38.3499529169218)) ;
#59127=CARTESIAN_POINT('Ctrl Pts',(28.8337428817942,618.357514178974,-38.3137089382278)) ;
#59128=CARTESIAN_POINT('Ctrl Pts',(28.7877173256831,618.361284694683,-38.274895306099)) ;
#59129=CARTESIAN_POINT('Ctrl Pts',(28.7440217543737,618.365125980119,-38.2337617297627)) ;
#59130=CARTESIAN_POINT('Ctrl Pts',(28.7057698880118,618.368488708485,-38.197752678551)) ;
#59131=CARTESIAN_POINT('Ctrl Pts',(28.6693036492513,618.371906199368,-38.1599662778762)) ;
#59132=CARTESIAN_POINT('Ctrl Pts',(28.6348100298656,618.37542306303,-38.120599317061)) ;
#59133=CARTESIAN_POINT('Ctrl Pts',(28.6347883455892,618.375425273892,-38.120574569178)) ;
#59134=CARTESIAN_POINT('Ctrl Pts',(28.6347666620908,618.375427484794,-38.1205498206701)) ;
#59135=CARTESIAN_POINT('Ctrl Pts',(28.6347449793705,618.375429695735,-38.1205250715374)) ;
#59136=CARTESIAN_POINT('Ctrl Pts',(28.5981467952976,618.379161534733,-38.0787511013883)) ;
#59137=CARTESIAN_POINT('Ctrl Pts',(28.5636303654075,618.383015722911,-38.0350294420995)) ;
#59138=CARTESIAN_POINT('Ctrl Pts',(28.531378565565,618.386928787822,-37.9896100342397)) ;
#59139=CARTESIAN_POINT('Ctrl Pts',(28.5284469004474,618.387284482573,-37.9854814431429)) ;
#59140=CARTESIAN_POINT('Ctrl Pts',(28.5255339488775,618.387640663803,-37.9813388596409)) ;
#59141=CARTESIAN_POINT('Ctrl Pts',(28.5226398486572,618.38799728384,-37.977182492738)) ;
#59142=CARTESIAN_POINT('Ctrl Pts',(28.4874781000698,618.392330023944,-37.9266848883172)) ;
#59143=CARTESIAN_POINT('Ctrl Pts',(28.4550983019595,618.396726873743,-37.8741467840394)) ;
#59144=CARTESIAN_POINT('Ctrl Pts',(28.425700907645,618.401116810854,-37.8199226959434)) ;
#59145=CARTESIAN_POINT('Ctrl Pts',(28.396740112552,618.405441550244,-37.7665039239378)) ;
#59146=CARTESIAN_POINT('Ctrl Pts',(28.3706733647025,618.40975930175,-37.7114489965768)) ;
#59147=CARTESIAN_POINT('Ctrl Pts',(28.347654934977,618.414022908089,-37.6551079675871)) ;
#59148=CARTESIAN_POINT('Ctrl Pts',(28.324649873497,618.418284038284,-37.5987996593654)) ;
#59149=CARTESIAN_POINT('Ctrl Pts',(28.3046894658897,618.422490954923,-37.5412067612326)) ;
#59150=CARTESIAN_POINT('Ctrl Pts',(28.2878940171809,618.426620502795,-37.482688995998)) ;
#59151=CARTESIAN_POINT('Ctrl Pts',(28.2711020539386,618.430749193685,-37.4241833746311)) ;
#59152=CARTESIAN_POINT('Ctrl Pts',(28.2574737739795,618.434800548162,-37.364753280186)) ;
#59153=CARTESIAN_POINT('Ctrl Pts',(28.2470963213345,618.438776292223,-37.3047683084225)) ;
#59154=CARTESIAN_POINT('Ctrl Pts',(28.236433133094,618.4428615055,-37.2431316941786)) ;
#59155=CARTESIAN_POINT('Ctrl Pts',(28.229202618305,618.446866900611,-37.1809092011108)) ;
#59156=CARTESIAN_POINT('Ctrl Pts',(28.2254611411747,618.450820715466,-37.1185126557978)) ;
#59157=CARTESIAN_POINT('Ctrl Pts',(28.221814930076,618.454673857716,-37.0577048603424)) ;
#59158=CARTESIAN_POINT('Ctrl Pts',(28.221482507039,618.458478384057,-36.9967318626566)) ;
#59159=CARTESIAN_POINT('Ctrl Pts',(28.2244768711679,618.462281923013,-36.9359843188411)) ;
#59160=CARTESIAN_POINT('Ctrl Pts',(28.2275885877403,618.46623452687,-36.8728560115677)) ;
#59161=CARTESIAN_POINT('Ctrl Pts',(28.2342938498349,618.47018649312,-36.8099713082175)) ;
#59162=CARTESIAN_POINT('Ctrl Pts',(28.2445558748495,618.474209148222,-36.7477775418026)) ;
#59163=CARTESIAN_POINT('Ctrl Pts',(28.2534123844592,618.477680849325,-36.6941020061133)) ;
#59164=CARTESIAN_POINT('Ctrl Pts',(28.2649180720467,618.481205864618,-36.6409401234693)) ;
#59165=CARTESIAN_POINT('Ctrl Pts',(28.2790106999861,618.484834804392,-36.5885857918049)) ;
#59166=CARTESIAN_POINT('Ctrl Pts',(28.2812380762404,618.485408367698,-36.5803110544275)) ;
#59167=CARTESIAN_POINT('Ctrl Pts',(28.2835300330796,618.485984527103,-36.5720563932982)) ;
#59168=CARTESIAN_POINT('Ctrl Pts',(28.2858862795444,618.486563482427,-36.5638228581211)) ;
#59169=CARTESIAN_POINT('Ctrl Pts',(28.2858959098962,618.486565848709,-36.5637892063614)) ;
#59170=CARTESIAN_POINT('Ctrl Pts',(28.2859055413219,618.486568215038,-36.5637555549545)) ;
#59171=CARTESIAN_POINT('Ctrl Pts',(28.2859151738214,618.486570581413,-36.5637219039006)) ;
#59172=CARTESIAN_POINT('Ctrl Pts',(28.3010463718862,618.490287798736,-36.5108611940827)) ;
#59173=CARTESIAN_POINT('Ctrl Pts',(28.3188924951506,618.494130565774,-36.4586752415526)) ;
#59174=CARTESIAN_POINT('Ctrl Pts',(28.3393466499888,618.498036067807,-36.4074469701344)) ;
#59175=CARTESIAN_POINT('Ctrl Pts',(28.3413404373472,618.498416760172,-36.4024534477544)) ;
#59176=CARTESIAN_POINT('Ctrl Pts',(28.3433589712799,618.498798048617,-36.397469047839)) ;
#59177=CARTESIAN_POINT('Ctrl Pts',(28.3454021306024,618.499179874965,-36.3924940467439)) ;
#59178=CARTESIAN_POINT('Ctrl Pts',(28.3687767930042,618.503548140265,-36.3355777946607)) ;
#59179=CARTESIAN_POINT('Ctrl Pts',(28.3953793814839,618.507986112013,-36.2798879307798)) ;
#59180=CARTESIAN_POINT('Ctrl Pts',(28.4250204492715,618.512420494789,-36.2257875204666)) ;
#59181=CARTESIAN_POINT('Ctrl Pts',(28.4541082846005,618.516772112514,-36.1726968613278)) ;
#59182=CARTESIAN_POINT('Ctrl Pts',(28.4861218665686,618.521119990088,-36.1211365656175)) ;
#59183=CARTESIAN_POINT('Ctrl Pts',(28.5208522567435,618.525415096405,-36.071424110073)) ;
#59184=CARTESIAN_POINT('Ctrl Pts',(28.5555607222739,618.529707491302,-36.0217430370702)) ;
#59185=CARTESIAN_POINT('Ctrl Pts',(28.5929824726078,618.53394703886,-35.9739073758844)) ;
#59186=CARTESIAN_POINT('Ctrl Pts',(28.6328819965436,618.538108371662,-35.9282110840983)) ;
#59187=CARTESIAN_POINT('Ctrl Pts',(28.6727715019973,618.542268659583,-35.8825262663209)) ;
#59188=CARTESIAN_POINT('Ctrl Pts',(28.7151375358478,618.546350761444,-35.8389797790131)) ;
#59189=CARTESIAN_POINT('Ctrl Pts',(28.7597184621479,618.550354009176,-35.7978428806241)) ;
#59190=CARTESIAN_POINT('Ctrl Pts',(28.8058407739393,618.554495669195,-35.755283674006)) ;
#59191=CARTESIAN_POINT('Ctrl Pts',(28.854334021853,618.558552896762,-35.7153038834646)) ;
#59192=CARTESIAN_POINT('Ctrl Pts',(28.9048783231777,618.56255194805,-35.6781769381591)) ;
#59193=CARTESIAN_POINT('Ctrl Pts',(28.95379750039,618.566422419963,-35.6422437158344)) ;
#59194=CARTESIAN_POINT('Ctrl Pts',(29.0046379149652,618.570238776668,-35.6089829846873)) ;
#59195=CARTESIAN_POINT('Ctrl Pts',(29.0570808636889,618.574046624285,-35.5786148015285)) ;
#59196=CARTESIAN_POINT('Ctrl Pts',(29.1121370912538,618.57804422034,-35.5467333447566)) ;
#59197=CARTESIAN_POINT('Ctrl Pts',(29.168959963637,618.582032813487,-35.5180407741232)) ;
#59198=CARTESIAN_POINT('Ctrl Pts',(29.227145093238,618.586084376013,-35.4927523278367)) ;
#59199=CARTESIAN_POINT('Ctrl Pts',(29.277292708399,618.58957626818,-35.4709571495654)) ;
#59200=CARTESIAN_POINT('Ctrl Pts',(29.3284530721797,618.593115597418,-35.4516900420697)) ;
#59201=CARTESIAN_POINT('Ctrl Pts',(29.380340762874,618.596754151116,-35.4350591250646)) ;
#59202=CARTESIAN_POINT('Ctrl Pts',(29.3886393508534,618.597336078304,-35.4323992817357)) ;
#59203=CARTESIAN_POINT('Ctrl Pts',(29.3969566044291,618.597920543533,-35.4298067796712)) ;
#59204=CARTESIAN_POINT('Ctrl Pts',(29.4052914292488,618.598507758659,-35.4272819610661)) ;
#59205=CARTESIAN_POINT('Ctrl Pts',(29.4053093277901,618.598509019668,-35.4272765391681)) ;
#59206=CARTESIAN_POINT('Ctrl Pts',(29.4053272264123,618.598510280691,-35.4272711175822)) ;
#59207=CARTESIAN_POINT('Ctrl Pts',(29.4053451251156,618.598511541726,-35.4272656963085)) ;
#59208=CARTESIAN_POINT('Ctrl Pts',(29.4591371956578,618.602301407442,-35.410972809824)) ;
#59209=CARTESIAN_POINT('Ctrl Pts',(29.5138522715128,618.606215726214,-35.3974495137543)) ;
#59210=CARTESIAN_POINT('Ctrl Pts',(29.5691829405726,618.610192153612,-35.3867582200091)) ;
#59211=CARTESIAN_POINT('Ctrl Pts',(29.5747522698706,618.610592402406,-35.3856820838174)) ;
#59212=CARTESIAN_POINT('Ctrl Pts',(29.580327795787,618.610993280455,-35.3846346234691)) ;
#59213=CARTESIAN_POINT('Ctrl Pts',(29.5859091781601,618.611394724179,-35.3836158907974)) ;
#59214=CARTESIAN_POINT('Ctrl Pts',(29.6468116129468,618.615775162321,-35.3724997736849)) ;
#59215=CARTESIAN_POINT('Ctrl Pts',(29.7084170829286,618.620222316849,-35.3648059135374)) ;
#59216=CARTESIAN_POINT('Ctrl Pts',(29.7703212950613,618.624666969685,-35.3605694397996)) ;
#59217=CARTESIAN_POINT('Ctrl Pts',(29.8321487915922,618.629106114427,-35.356338216167)) ;
#59218=CARTESIAN_POINT('Ctrl Pts',(29.8942743873207,618.633542423227,-35.3555554472147)) ;
#59219=CARTESIAN_POINT('Ctrl Pts',(29.9563008980942,618.637927518225,-35.3582177975719)) ;
#59220=CARTESIAN_POINT('Ctrl Pts',(30.0182700325272,618.64230855688,-35.3608776851769)) ;
#59221=CARTESIAN_POINT('Ctrl Pts',(30.0801403488002,618.646638340028,-35.3669762005155)) ;
#59222=CARTESIAN_POINT('Ctrl Pts',(30.1415199219065,618.650892676407,-35.3764753083873)) ;
#59223=CARTESIAN_POINT('Ctrl Pts',(30.2028619874384,618.655144413065,-35.3859686115837)) ;
#59224=CARTESIAN_POINT('Ctrl Pts',(30.2637139257696,618.659320802209,-35.3988584066383)) ;
#59225=CARTESIAN_POINT('Ctrl Pts',(30.3236879141443,618.663422665272,-35.4150724876848)) ;
#59226=CARTESIAN_POINT('Ctrl Pts',(30.3836672515966,618.66752489418,-35.4312880148645)) ;
#59227=CARTESIAN_POINT('Ctrl Pts',(30.442768415426,618.671552718056,-35.4508286163203)) ;
#59228=CARTESIAN_POINT('Ctrl Pts',(30.5006072297424,618.675530890686,-35.4735859176792)) ;
#59229=CARTESIAN_POINT('Ctrl Pts',(30.5584438181912,618.679508910221,-35.4963423432467)) ;
#59230=CARTESIAN_POINT('Ctrl Pts',(30.6150179711524,618.683437574835,-35.5223155447779)) ;
#59231=CARTESIAN_POINT('Ctrl Pts',(30.6699511312009,618.687362406073,-35.551357120278)) ;
#59232=CARTESIAN_POINT('Ctrl Pts',(30.7249388551544,618.691291135759,-35.5804275421391)) ;
#59233=CARTESIAN_POINT('Ctrl Pts',(30.7782819396851,618.695216528502,-35.6125728745798)) ;
#59234=CARTESIAN_POINT('Ctrl Pts',(30.8296104393782,618.699199140992,-35.6475983749195)) ;
#59235=CARTESIAN_POINT('Ctrl Pts',(30.8775564809086,618.7029193063,-35.6803157561786)) ;
#59236=CARTESIAN_POINT('Ctrl Pts',(30.9237443136949,618.706690051297,-35.7155460684294)) ;
#59237=CARTESIAN_POINT('Ctrl Pts',(30.9678862784723,618.710565160562,-35.7530892919022)) ;
#59238=CARTESIAN_POINT('',(30.9861662751902,618.710557609671,-38.2766259197886)) ;
#59239=CARTESIAN_POINT('Origin',(29.888527625422,618.710565160562,-37.0221601717529)) ;
#59240=CARTESIAN_POINT('',(29.8893921427819,618.088263764204,-38.6876853814548)) ;
#59241=CARTESIAN_POINT('Ctrl Pts',(30.9861662858252,618.710557609533,-38.2766259319431)) ;
#59242=CARTESIAN_POINT('Ctrl Pts',(31.0258667566383,618.70695394026,-38.2418476139244)) ;
#59243=CARTESIAN_POINT('Ctrl Pts',(31.0639450042156,618.703253312121,-38.2050806626661)) ;
#59244=CARTESIAN_POINT('Ctrl Pts',(31.1002122807239,618.699509774449,-38.1665176179903)) ;
#59245=CARTESIAN_POINT('Ctrl Pts',(31.1416403247482,618.695233538173,-38.1224671221618)) ;
#59246=CARTESIAN_POINT('Ctrl Pts',(31.1807061224321,618.690901872949,-38.0760720093977)) ;
#59247=CARTESIAN_POINT('Ctrl Pts',(31.2171692764965,618.686580914103,-38.0276356050523)) ;
#59248=CARTESIAN_POINT('Ctrl Pts',(31.2535952574382,618.682264360348,-37.9792485802092)) ;
#59249=CARTESIAN_POINT('Ctrl Pts',(31.2874241804867,618.677958789138,-37.92882455607)) ;
#59250=CARTESIAN_POINT('Ctrl Pts',(31.3184506199994,618.673709374166,-37.8766830306392)) ;
#59251=CARTESIAN_POINT('Ctrl Pts',(31.3494572013223,618.669462678993,-37.8245748779165)) ;
#59252=CARTESIAN_POINT('Ctrl Pts',(31.3776649807041,618.66527218633,-37.7707514607234)) ;
#59253=CARTESIAN_POINT('Ctrl Pts',(31.4029003397019,618.661159188947,-37.7155475642533)) ;
#59254=CARTESIAN_POINT('Ctrl Pts',(31.4281291215752,618.65704726354,-37.6603580556468)) ;
#59255=CARTESIAN_POINT('Ctrl Pts',(31.4503869748622,618.653012783546,-37.6037887980431)) ;
#59256=CARTESIAN_POINT('Ctrl Pts',(31.4695315749085,618.649052449208,-37.5461898742506)) ;
#59257=CARTESIAN_POINT('Ctrl Pts',(31.4886923015302,618.645088778857,-37.4885424316393)) ;
#59258=CARTESIAN_POINT('Ctrl Pts',(31.5047343325093,618.641199255126,-37.4298635887972)) ;
#59259=CARTESIAN_POINT('Ctrl Pts',(31.5175481043101,618.637356933796,-37.3705198260656)) ;
#59260=CARTESIAN_POINT('Ctrl Pts',(31.5303666885878,618.633513169403,-37.311153775557)) ;
#59261=CARTESIAN_POINT('Ctrl Pts',(31.539954249111,618.629716369706,-37.2511223227426)) ;
#59262=CARTESIAN_POINT('Ctrl Pts',(31.5462382095542,618.625918855984,-37.1908077727697)) ;
#59263=CARTESIAN_POINT('Ctrl Pts',(31.5525341048052,618.622114129837,-37.1303786704265)) ;
#59264=CARTESIAN_POINT('Ctrl Pts',(31.5555133084016,618.618308212986,-37.0696654927814)) ;
#59265=CARTESIAN_POINT('Ctrl Pts',(31.555146597125,618.614437917341,-37.0090674408427)) ;
#59266=CARTESIAN_POINT('Ctrl Pts',(31.5548170738568,618.610960106454,-36.9546146072387)) ;
#59267=CARTESIAN_POINT('Ctrl Pts',(31.5517858889841,618.607429722511,-36.9002543398607)) ;
#59268=CARTESIAN_POINT('Ctrl Pts',(31.5460685179213,618.603796420824,-36.8462866158652)) ;
#59269=CARTESIAN_POINT('Ctrl Pts',(31.545556999344,618.603471358608,-36.8414582615226)) ;
#59270=CARTESIAN_POINT('Ctrl Pts',(31.5450239981011,618.603145472594,-36.8366330202235)) ;
#59271=CARTESIAN_POINT('Ctrl Pts',(31.5444695359318,618.60281872673,-36.8318110893893)) ;
#59272=CARTESIAN_POINT('Ctrl Pts',(31.5444657676938,618.602816506098,-36.831778318564)) ;
#59273=CARTESIAN_POINT('Ctrl Pts',(31.5444619984646,618.602814285427,-36.8317455478917)) ;
#59274=CARTESIAN_POINT('Ctrl Pts',(31.5444582282442,618.602812064716,-36.8317127773723)) ;
#59275=CARTESIAN_POINT('Ctrl Pts',(31.5381108427545,618.599073368529,-36.7765417002896)) ;
#59276=CARTESIAN_POINT('Ctrl Pts',(31.5289226744486,618.595212190571,-36.7216055721164)) ;
#59277=CARTESIAN_POINT('Ctrl Pts',(31.5169560025884,618.591291590598,-36.6672070009179)) ;
#59278=CARTESIAN_POINT('Ctrl Pts',(31.5158419372211,618.590926593153,-36.6621426384192)) ;
#59279=CARTESIAN_POINT('Ctrl Pts',(31.5147038169095,618.590561080691,-36.6570829610815)) ;
#59280=CARTESIAN_POINT('Ctrl Pts',(31.5135417086785,618.590195104094,-36.6520282286846)) ;
#59281=CARTESIAN_POINT('Ctrl Pts',(31.4997587502424,618.585854509907,-36.5920775591406)) ;
#59282=CARTESIAN_POINT('Ctrl Pts',(31.4825975136841,618.58144928703,-36.5328179968727)) ;
#59283=CARTESIAN_POINT('Ctrl Pts',(31.4621857936471,618.577050252619,-36.4746349590504)) ;
#59284=CARTESIAN_POINT('Ctrl Pts',(31.4420337111258,618.572707174019,-36.4171920107145)) ;
#59285=CARTESIAN_POINT('Ctrl Pts',(31.4187136805253,618.568370419492,-36.3607981428071)) ;
#59286=CARTESIAN_POINT('Ctrl Pts',(31.3923820323704,618.564087593537,-36.3058038966044)) ;
#59287=CARTESIAN_POINT('Ctrl Pts',(31.3660662969591,618.55980735578,-36.2508428845287)) ;
#59288=CARTESIAN_POINT('Ctrl Pts',(31.3367426822218,618.555581116504,-36.197279718318)) ;
#59289=CARTESIAN_POINT('Ctrl Pts',(31.3045974844214,618.551432583277,-36.1454461744282)) ;
#59290=CARTESIAN_POINT('Ctrl Pts',(31.2724598498184,618.547285026127,-36.0936248260561)) ;
#59291=CARTESIAN_POINT('Ctrl Pts',(31.2375019420153,618.543215140447,-36.0435323174582)) ;
#59292=CARTESIAN_POINT('Ctrl Pts',(31.1999396127379,618.539221816271,-35.9954824563047)) ;
#59293=CARTESIAN_POINT('Ctrl Pts',(31.1614845324218,618.535133581999,-35.9462905849436)) ;
#59294=CARTESIAN_POINT('Ctrl Pts',(31.1202995205151,618.531125564924,-35.8992398452946)) ;
#59295=CARTESIAN_POINT('Ctrl Pts',(31.0766494256803,618.527170583501,-35.8546462743732)) ;
#59296=CARTESIAN_POINT('Ctrl Pts',(31.0339583163552,618.523302492379,-35.8110324169781)) ;
#59297=CARTESIAN_POINT('Ctrl Pts',(30.9889091924407,618.519484778323,-35.7697691473266)) ;
#59298=CARTESIAN_POINT('Ctrl Pts',(30.9417830813077,618.515670566426,-35.7311296085355)) ;
#59299=CARTESIAN_POINT('Ctrl Pts',(30.8930690543857,618.511727834539,-35.6911881092758)) ;
#59300=CARTESIAN_POINT('Ctrl Pts',(30.8421352602933,618.50778841439,-35.6540508351474)) ;
#59301=CARTESIAN_POINT('Ctrl Pts',(30.7893324095246,618.503782920354,-35.6199881496201)) ;
#59302=CARTESIAN_POINT('Ctrl Pts',(30.7433891606403,618.500297778799,-35.5903505369521)) ;
#59303=CARTESIAN_POINT('Ctrl Pts',(30.6960302507629,618.496761965997,-35.5630399679191)) ;
#59304=CARTESIAN_POINT('Ctrl Pts',(30.6475172782936,618.493124863879,-35.5382100550777)) ;
#59305=CARTESIAN_POINT('Ctrl Pts',(30.640301374707,618.492583875008,-35.5345168108173)) ;
#59306=CARTESIAN_POINT('Ctrl Pts',(30.6330599000393,618.492040645201,-35.530878363005)) ;
#59307=CARTESIAN_POINT('Ctrl Pts',(30.6257936722541,618.491495007886,-35.5272951280833)) ;
#59308=CARTESIAN_POINT('Ctrl Pts',(30.6257661079495,618.491492938021,-35.5272815351459)) ;
#59309=CARTESIAN_POINT('Ctrl Pts',(30.6257385432886,618.491490868121,-35.5272679430031)) ;
#59310=CARTESIAN_POINT('Ctrl Pts',(30.6257109782715,618.491488798186,-35.5272543516547)) ;
#59311=CARTESIAN_POINT('Ctrl Pts',(30.5759895713561,618.487755077898,-35.5027384603596)) ;
#59312=CARTESIAN_POINT('Ctrl Pts',(30.5249275120125,618.483898811178,-35.4807273012484)) ;
#59313=CARTESIAN_POINT('Ctrl Pts',(30.4728117649734,618.479983217499,-35.461332928774)) ;
#59314=CARTESIAN_POINT('Ctrl Pts',(30.4679799255449,618.479620188645,-35.4595348063458)) ;
#59315=CARTESIAN_POINT('Ctrl Pts',(30.4631390649157,618.479256649827,-35.4577591692149)) ;
#59316=CARTESIAN_POINT('Ctrl Pts',(30.458289433724,618.478892651429,-35.4560061011717)) ;
#59317=CARTESIAN_POINT('Ctrl Pts',(30.4004223207642,618.474549323946,-35.4350880184408)) ;
#59318=CARTESIAN_POINT('Ctrl Pts',(30.3413005195102,618.470141228125,-35.4173842219975)) ;
#59319=CARTESIAN_POINT('Ctrl Pts',(30.281318183977,618.465739742904,-35.4029973618508)) ;
#59320=CARTESIAN_POINT('Ctrl Pts',(30.2222367147747,618.461404362975,-35.3888265759499)) ;
#59321=CARTESIAN_POINT('Ctrl Pts',(30.1623203746084,618.457075679211,-35.3778733946167)) ;
#59322=CARTESIAN_POINT('Ctrl Pts',(30.1019469813105,618.452801348568,-35.3701968730303)) ;
#59323=CARTESIAN_POINT('Ctrl Pts',(30.0416110635627,618.448529671129,-35.3625251164877)) ;
#59324=CARTESIAN_POINT('Ctrl Pts',(29.9808186466924,618.444312413336,-35.3581258264937)) ;
#59325=CARTESIAN_POINT('Ctrl Pts',(29.9199481378645,618.440173371419,-35.3570227113294)) ;
#59326=CARTESIAN_POINT('Ctrl Pts',(29.8590927072241,618.436035354782,-35.3559198694169)) ;
#59327=CARTESIAN_POINT('Ctrl Pts',(29.7981592444871,618.431975517372,-35.3581116017446)) ;
#59328=CARTESIAN_POINT('Ctrl Pts',(29.7375271299118,618.427992883047,-35.3635870253733)) ;
#59329=CARTESIAN_POINT('Ctrl Pts',(29.6752004343361,618.423898939782,-35.3692154792717)) ;
#59330=CARTESIAN_POINT('Ctrl Pts',(29.6131922391728,618.419886566595,-35.3783140957345)) ;
#59331=CARTESIAN_POINT('Ctrl Pts',(29.5519152757824,618.415928380366,-35.3908313429493)) ;
#59332=CARTESIAN_POINT('Ctrl Pts',(29.4922285529616,618.412072915747,-35.4030237464832)) ;
#59333=CARTESIAN_POINT('Ctrl Pts',(29.4332357413764,618.408268493894,-35.4184597707061)) ;
#59334=CARTESIAN_POINT('Ctrl Pts',(29.3753173076147,618.404468336497,-35.4370515913484)) ;
#59335=CARTESIAN_POINT('Ctrl Pts',(29.3150841821071,618.40051630702,-35.4563864281773)) ;
#59336=CARTESIAN_POINT('Ctrl Pts',(29.2560133821818,618.396568471163,-35.4791351648903)) ;
#59337=CARTESIAN_POINT('Ctrl Pts',(29.1985281518379,618.392554218511,-35.5051471697204)) ;
#59338=CARTESIAN_POINT('Ctrl Pts',(29.148800094153,618.389081657189,-35.5276490622754)) ;
#59339=CARTESIAN_POINT('Ctrl Pts',(29.1002576320191,618.385558736114,-35.5525931822916)) ;
#59340=CARTESIAN_POINT('Ctrl Pts',(29.0531707881797,618.381934784252,-35.5798429037858)) ;
#59341=CARTESIAN_POINT('Ctrl Pts',(29.0458515041979,618.381371469095,-35.5840786612454)) ;
#59342=CARTESIAN_POINT('Ctrl Pts',(29.0385672899433,618.380805712803,-35.5883701117772)) ;
#59343=CARTESIAN_POINT('Ctrl Pts',(29.031319046969,618.380237325065,-35.5927167281838)) ;
#59344=CARTESIAN_POINT('Ctrl Pts',(29.0312934173751,618.380235315261,-35.5927320977036)) ;
#59345=CARTESIAN_POINT('Ctrl Pts',(29.0312677882308,618.380233305424,-35.5927474679131)) ;
#59346=CARTESIAN_POINT('Ctrl Pts',(29.0312421595363,618.380231295554,-35.5927628388123)) ;
#59347=CARTESIAN_POINT('Ctrl Pts',(28.9837044478577,618.376503263034,-35.6212737476888)) ;
#59348=CARTESIAN_POINT('Ctrl Pts',(28.9375467752205,618.372652138925,-35.6522677068982)) ;
#59349=CARTESIAN_POINT('Ctrl Pts',(28.8930184784191,618.368741066252,-35.6855640604781)) ;
#59350=CARTESIAN_POINT('Ctrl Pts',(28.8888546870006,618.368375346205,-35.6886775654011)) ;
#59351=CARTESIAN_POINT('Ctrl Pts',(28.8847051555669,618.368009101972,-35.691811166888)) ;
#59352=CARTESIAN_POINT('Ctrl Pts',(28.8805700953766,618.367642385182,-35.6949646952095)) ;
#59353=CARTESIAN_POINT('Ctrl Pts',(28.8316436881913,618.363303358867,-35.7322775283065)) ;
#59354=CARTESIAN_POINT('Ctrl Pts',(28.7847407909223,618.358898842722,-35.7723855885088)) ;
#59355=CARTESIAN_POINT('Ctrl Pts',(28.7401608122143,618.354500231938,-35.8150129554806)) ;
#59356=CARTESIAN_POINT('Ctrl Pts',(28.6962222493042,618.350164908274,-35.8570270007912)) ;
#59357=CARTESIAN_POINT('Ctrl Pts',(28.6545398706444,618.34583560831,-35.9014881307113)) ;
#59358=CARTESIAN_POINT('Ctrl Pts',(28.6153680467039,618.341560153364,-35.9481101168694)) ;
#59359=CARTESIAN_POINT('Ctrl Pts',(28.5762202788798,618.337287324051,-35.9947034716336)) ;
#59360=CARTESIAN_POINT('Ctrl Pts',(28.539579866489,618.333068408917,-36.0434549721131)) ;
#59361=CARTESIAN_POINT('Ctrl Pts',(28.5056717224049,618.32892735311,-36.0940588161533)) ;
#59362=CARTESIAN_POINT('Ctrl Pts',(28.4717717941343,618.324787300665,-36.1446503990759)) ;
#59363=CARTESIAN_POINT('Ctrl Pts',(28.4406028467046,618.320725072517,-36.1970934286391)) ;
#59364=CARTESIAN_POINT('Ctrl Pts',(28.4123612160282,618.316739811669,-36.2510626063029)) ;
#59365=CARTESIAN_POINT('Ctrl Pts',(28.38336289804,618.312647772415,-36.3064777979177)) ;
#59366=CARTESIAN_POINT('Ctrl Pts',(28.3574511941756,618.30863686713,-36.3635021437826)) ;
#59367=CARTESIAN_POINT('Ctrl Pts',(28.3348057428245,618.30467990851,-36.4217615767189)) ;
#59368=CARTESIAN_POINT('Ctrl Pts',(28.3127230432915,618.30082128247,-36.478573230969)) ;
#59369=CARTESIAN_POINT('Ctrl Pts',(28.2937464644792,618.297013591652,-36.5365593056891)) ;
#59370=CARTESIAN_POINT('Ctrl Pts',(28.2780083026968,618.293210123154,-36.5953520015067)) ;
#59371=CARTESIAN_POINT('Ctrl Pts',(28.2616685378942,618.289261264225,-36.6563920921512)) ;
#59372=CARTESIAN_POINT('Ctrl Pts',(28.2488203709418,618.285316536279,-36.7183017893232)) ;
#59373=CARTESIAN_POINT('Ctrl Pts',(28.2395660305023,618.281305714831,-36.7806454803147)) ;
#59374=CARTESIAN_POINT('Ctrl Pts',(28.2315445039564,618.277829193633,-36.8346840771793)) ;
#59375=CARTESIAN_POINT('Ctrl Pts',(28.2262227954632,618.274302359799,-36.889049637097)) ;
#59376=CARTESIAN_POINT('Ctrl Pts',(28.2236324605726,618.270674475694,-36.9434406507769)) ;
#59377=CARTESIAN_POINT('Ctrl Pts',(28.223235763576,618.270118883158,-36.9517703659216)) ;
#59378=CARTESIAN_POINT('Ctrl Pts',(28.2229030607497,618.26956092065,-36.960100752751)) ;
#59379=CARTESIAN_POINT('Ctrl Pts',(28.2226343961012,618.26900040593,-36.9684308115211)) ;
#59380=CARTESIAN_POINT('Ctrl Pts',(28.2226334432837,618.268998418067,-36.9684603540242)) ;
#59381=CARTESIAN_POINT('Ctrl Pts',(28.2226324912715,618.268996430173,-36.9684898965232)) ;
#59382=CARTESIAN_POINT('Ctrl Pts',(28.2226315400648,618.268994442247,-36.9685194390181)) ;
#59383=CARTESIAN_POINT('Ctrl Pts',(28.2208468079136,618.26526453179,-37.0239494927733)) ;
#59384=CARTESIAN_POINT('Ctrl Pts',(28.2218993982417,618.261411768754,-37.0795641973424)) ;
#59385=CARTESIAN_POINT('Ctrl Pts',(28.2257723975202,618.257499301475,-37.1350557789974)) ;
#59386=CARTESIAN_POINT('Ctrl Pts',(28.2261333900683,618.257134630213,-37.1402280101343)) ;
#59387=CARTESIAN_POINT('Ctrl Pts',(28.2265188627023,618.256769440263,-37.1453991418306)) ;
#59388=CARTESIAN_POINT('Ctrl Pts',(28.2269287873742,618.256403782759,-37.1505689068973)) ;
#59389=CARTESIAN_POINT('Ctrl Pts',(28.2317923068705,618.252065467639,-37.2119051838194)) ;
#59390=CARTESIAN_POINT('Ctrl Pts',(28.2401011002908,618.247662003083,-37.2730541153256)) ;
#59391=CARTESIAN_POINT('Ctrl Pts',(28.2517853580537,618.24326465075,-37.3336147428047)) ;
#59392=CARTESIAN_POINT('Ctrl Pts',(28.2633042205175,618.238929544683,-37.3933181106021)) ;
#59393=CARTESIAN_POINT('Ctrl Pts',(28.2781032539723,618.234600666219,-37.4524498885658)) ;
#59394=CARTESIAN_POINT('Ctrl Pts',(28.2960795570283,618.230325746232,-37.51064111304)) ;
#59395=CARTESIAN_POINT('Ctrl Pts',(28.3140448906859,618.226053434863,-37.5687968283932)) ;
#59396=CARTESIAN_POINT('Ctrl Pts',(28.3351835064466,618.221835151049,-37.6260132048384)) ;
#59397=CARTESIAN_POINT('Ctrl Pts',(28.3593600959597,618.217694743611,-37.6819354353026)) ;
#59398=CARTESIAN_POINT('Ctrl Pts',(28.3835309127598,618.21355532479,-37.7378443130568)) ;
#59399=CARTESIAN_POINT('Ctrl Pts',(28.41073827333,618.209493747495,-37.7924596325546)) ;
#59400=CARTESIAN_POINT('Ctrl Pts',(28.4408149988073,618.205509057314,-37.8454400449)) ;
#59401=CARTESIAN_POINT('Ctrl Pts',(28.4716846556205,618.201419316279,-37.899817212659)) ;
#59402=CARTESIAN_POINT('Ctrl Pts',(28.5055772510173,618.197410554523,-37.9524719262378)) ;
#59403=CARTESIAN_POINT('Ctrl Pts',(28.5422758315809,618.193455524331,-38.003050887678)) ;
#59404=CARTESIAN_POINT('Ctrl Pts',(28.578077631573,618.189597140771,-38.0523938822431)) ;
#59405=CARTESIAN_POINT('Ctrl Pts',(28.6165500236072,618.185789532356,-38.0997611500694)) ;
#59406=CARTESIAN_POINT('Ctrl Pts',(28.6574553993652,618.181985915573,-38.1448421396957)) ;
#59407=CARTESIAN_POINT('Ctrl Pts',(28.6998977011823,618.178039386579,-38.1916169445344)) ;
#59408=CARTESIAN_POINT('Ctrl Pts',(28.744959830827,618.17409673234,-38.2359297901857)) ;
#59409=CARTESIAN_POINT('Ctrl Pts',(28.7923314482007,618.170087815097,-38.2774592594093)) ;
#59410=CARTESIAN_POINT('Ctrl Pts',(28.8334067265285,618.166611738056,-38.3134688913732)) ;
#59411=CARTESIAN_POINT('Ctrl Pts',(28.8762189636619,618.163085187076,-38.3473865949876)) ;
#59412=CARTESIAN_POINT('Ctrl Pts',(28.9205319247919,618.159457468053,-38.3790226032246)) ;
#59413=CARTESIAN_POINT('Ctrl Pts',(28.927300312747,618.158903368099,-38.383854705879)) ;
#59414=CARTESIAN_POINT('Ctrl Pts',(28.9341037390459,618.158346907925,-38.3886336726395)) ;
#59415=CARTESIAN_POINT('Ctrl Pts',(28.9409413939369,618.15778790689,-38.3933589298167)) ;
#59416=CARTESIAN_POINT('Ctrl Pts',(28.9409658904565,618.157785904218,-38.3933758584796)) ;
#59417=CARTESIAN_POINT('Ctrl Pts',(28.9409903874154,618.157783901514,-38.3933927864532)) ;
#59418=CARTESIAN_POINT('Ctrl Pts',(28.9410148848135,618.157781898776,-38.3934097137375)) ;
#59419=CARTESIAN_POINT('Ctrl Pts',(28.9869438604082,618.154027064591,-38.4251458524531)) ;
#59420=CARTESIAN_POINT('Ctrl Pts',(29.0345829173173,618.150147935566,-38.454563664042)) ;
#59421=CARTESIAN_POINT('Ctrl Pts',(29.0836625571254,618.146208705783,-38.4815110330523)) ;
#59422=CARTESIAN_POINT('Ctrl Pts',(29.088569528916,618.14581486244,-38.4842052251874)) ;
#59423=CARTESIAN_POINT('Ctrl Pts',(29.0934908577691,618.145420418332,-38.4868747247128)) ;
#59424=CARTESIAN_POINT('Ctrl Pts',(29.0984262458447,618.145025437615,-38.4895193815645)) ;
#59425=CARTESIAN_POINT('Ctrl Pts',(29.1526346499945,618.140687121352,-38.5185672751158)) ;
#59426=CARTESIAN_POINT('Ctrl Pts',(29.2085451927026,618.136284701166,-38.5446184457616)) ;
#59427=CARTESIAN_POINT('Ctrl Pts',(29.2657894773234,618.131888823386,-38.5675167492335)) ;
#59428=CARTESIAN_POINT('Ctrl Pts',(29.3229458365822,618.127499697532,-38.590379881655)) ;
#59429=CARTESIAN_POINT('Ctrl Pts',(29.3814318336443,618.123117430252,-38.6101002015592)) ;
#59430=CARTESIAN_POINT('Ctrl Pts',(29.4408743003571,618.118790860888,-38.6265597151448)) ;
#59431=CARTESIAN_POINT('Ctrl Pts',(29.5002633325708,618.114468180799,-38.6430044328125)) ;
#59432=CARTESIAN_POINT('Ctrl Pts',(29.5606071605186,618.110201238562,-38.6561943411892)) ;
#59433=CARTESIAN_POINT('Ctrl Pts',(29.621526796277,618.106013793532,-38.666045369854)) ;
#59434=CARTESIAN_POINT('Ctrl Pts',(29.6824149151413,618.101828514884,-38.6758913020695)) ;
#59435=CARTESIAN_POINT('Ctrl Pts',(29.7438782808071,618.097722656485,-38.6824017641329)) ;
#59436=CARTESIAN_POINT('Ctrl Pts',(29.8055310461891,618.093693952894,-38.6855257554669)) ;
#59437=CARTESIAN_POINT('Ctrl Pts',(29.8334581163121,618.091869056849,-38.6869408408163)) ;
#59438=CARTESIAN_POINT('Ctrl Pts',(29.8614239439526,618.090059638097,-38.6876615252047)) ;
#59439=CARTESIAN_POINT('Ctrl Pts',(29.8893921427819,618.088263764204,-38.6876853814548)) ;
#59440=CARTESIAN_POINT('Ctrl Pts',(29.8893746478611,618.087990585226,-38.6881599564327)) ;
#59441=CARTESIAN_POINT('Ctrl Pts',(29.9622844351597,618.083368135722,-38.6881228878649)) ;
#59442=CARTESIAN_POINT('Ctrl Pts',(30.0351169275643,618.07887743536,-38.683299808865)) ;
#59443=CARTESIAN_POINT('Ctrl Pts',(30.2114913540784,618.067997029309,-38.6599253324782)) ;
#59444=CARTESIAN_POINT('Ctrl Pts',(30.3140297828991,618.0616708931,-38.6363236340286)) ;
#59445=CARTESIAN_POINT('Ctrl Pts',(30.4305569294752,618.053832960999,-38.5976212057701)) ;
#59446=CARTESIAN_POINT('Ctrl Pts',(30.4473670450482,618.052685496838,-38.5917370547404)) ;
#59447=CARTESIAN_POINT('Ctrl Pts',(30.4640776573931,618.051524931058,-38.5855853092948)) ;
#59448=CARTESIAN_POINT('Origin',(179.888527625422,617.710565160536,-37.0221601717597)) ;
#59449=CARTESIAN_POINT('',(180.464123912022,616.842332842895,-38.5858650494033)) ;
#59450=CARTESIAN_POINT('',(180.464060715702,616.710565160536,-38.5855915460107)) ;
#59451=CARTESIAN_POINT('',(180.464060715702,617.710565160536,-38.5855915460107)) ;
#59452=CARTESIAN_POINT('',(181.553667127593,616.710572776564,-37.0987295421981)) ;
#59453=CARTESIAN_POINT('Origin',(179.888527625422,616.710565160536,-37.0221601717597)) ;
#59454=CARTESIAN_POINT('Ctrl Pts',(181.553667143704,616.710572776701,-37.0987295429389)) ;
#59455=CARTESIAN_POINT('Ctrl Pts',(181.551219015739,616.71416598167,-37.1513058672652)) ;
#59456=CARTESIAN_POINT('Ctrl Pts',(181.546218975108,616.717855507709,-37.2038530482861)) ;
#59457=CARTESIAN_POINT('Ctrl Pts',(181.538699664615,616.721587750684,-37.2561056544767)) ;
#59458=CARTESIAN_POINT('Ctrl Pts',(181.530086063372,616.725863149705,-37.3159626206176)) ;
#59459=CARTESIAN_POINT('Ctrl Pts',(181.518166274836,616.730194042225,-37.3754342915452)) ;
#59460=CARTESIAN_POINT('Ctrl Pts',(181.503027609458,616.734514285927,-37.4341435669554)) ;
#59461=CARTESIAN_POINT('Ctrl Pts',(181.487904369475,616.738830127558,-37.492793021121)) ;
#59462=CARTESIAN_POINT('Ctrl Pts',(181.469569088151,616.743135044131,-37.5506817707635)) ;
#59463=CARTESIAN_POINT('Ctrl Pts',(181.448143519656,616.747383864401,-37.6074499818234)) ;
#59464=CARTESIAN_POINT('Ctrl Pts',(181.426731654152,616.751629967285,-37.6641818860634)) ;
#59465=CARTESIAN_POINT('Ctrl Pts',(181.402233542896,616.755819927562,-37.7197947350221)) ;
#59466=CARTESIAN_POINT('Ctrl Pts',(181.374802719427,616.759932463143,-37.7739440349984)) ;
#59467=CARTESIAN_POINT('Ctrl Pts',(181.347379033597,616.76404392862,-37.8280792450522)) ;
#59468=CARTESIAN_POINT('Ctrl Pts',(181.317024134035,616.768078019286,-37.8807516162109)) ;
#59469=CARTESIAN_POINT('Ctrl Pts',(181.283923023809,616.772038052194,-37.9316315845311)) ;
#59470=CARTESIAN_POINT('Ctrl Pts',(181.250794021577,616.776001421948,-37.9825544258659)) ;
#59471=CARTESIAN_POINT('Ctrl Pts',(181.214914057745,616.779890733246,-38.0316816889812)) ;
#59472=CARTESIAN_POINT('Ctrl Pts',(181.176501382908,616.783732952265,-38.0786991995177)) ;
#59473=CARTESIAN_POINT('Ctrl Pts',(181.138074270226,616.787576615427,-38.1257343821257)) ;
#59474=CARTESIAN_POINT('Ctrl Pts',(181.097112343844,616.791373424309,-38.1706579499562)) ;
#59475=CARTESIAN_POINT('Ctrl Pts',(181.053869293275,616.795171081348,-38.2131747791317)) ;
#59476=CARTESIAN_POINT('Ctrl Pts',(181.010544127622,616.798975949833,-38.255772344356)) ;
#59477=CARTESIAN_POINT('Ctrl Pts',(180.964928911648,616.802782144032,-38.2959535452537)) ;
#59478=CARTESIAN_POINT('Ctrl Pts',(180.917317584923,616.806652873016,-38.3334466202017)) ;
#59479=CARTESIAN_POINT('Ctrl Pts',(180.874538611528,616.810130738969,-38.3671343026506)) ;
#59480=CARTESIAN_POINT('Ctrl Pts',(180.830147886244,616.813661294112,-38.3986521148746)) ;
#59481=CARTESIAN_POINT('Ctrl Pts',(180.784389550097,616.817294877271,-38.4278251727132)) ;
#59482=CARTESIAN_POINT('Ctrl Pts',(180.780328267656,616.817617376049,-38.4304144283009)) ;
#59483=CARTESIAN_POINT('Ctrl Pts',(180.776256201053,616.817940686425,-38.4329852454072)) ;
#59484=CARTESIAN_POINT('Ctrl Pts',(180.77217351419,616.818264843595,-38.4355375204749)) ;
#59485=CARTESIAN_POINT('Ctrl Pts',(180.772144653369,616.818267135086,-38.435555562699)) ;
#59486=CARTESIAN_POINT('Ctrl Pts',(180.772115792019,616.81826942662,-38.4355736039966)) ;
#59487=CARTESIAN_POINT('Ctrl Pts',(180.772086930137,616.818271718196,-38.4355916443677)) ;
#59488=CARTESIAN_POINT('Ctrl Pts',(180.724316691767,616.822064580185,-38.4654508490374)) ;
#59489=CARTESIAN_POINT('Ctrl Pts',(180.674926046349,616.825982750278,-38.4928664980066)) ;
#59490=CARTESIAN_POINT('Ctrl Pts',(180.624194942044,616.82996095168,-38.5177002140637)) ;
#59491=CARTESIAN_POINT('Ctrl Pts',(180.618794683314,616.83038442594,-38.5203437301822)) ;
#59492=CARTESIAN_POINT('Ctrl Pts',(180.61337928401,616.830808580434,-38.5229579922498)) ;
#59493=CARTESIAN_POINT('Ctrl Pts',(180.607949116393,616.831233336425,-38.5255428361978)) ;
#59494=CARTESIAN_POINT('Ctrl Pts',(180.561039635885,616.834902667516,-38.5478724759674)) ;
#59495=CARTESIAN_POINT('Ctrl Pts',(180.513023781992,616.838616789469,-38.5680076336995)) ;
#59496=CARTESIAN_POINT('Ctrl Pts',(180.464123912022,616.842332842895,-38.5858650494033)) ;
#59497=CARTESIAN_POINT('Origin',(179.888527625422,617.710565160536,-37.0221601717597)) ;
#59498=CARTESIAN_POINT('',(180.464060722638,617.544113575794,-38.5855915434574)) ;
#59499=CARTESIAN_POINT('',(180.464050813976,617.349688765578,-38.5855724216838)) ;
#59500=CARTESIAN_POINT('',(180.464060715702,617.710565160536,-38.5855915460107)) ;
#59501=CARTESIAN_POINT('',(179.569297170793,616.710565160536,-38.6572894990111)) ;
#59502=CARTESIAN_POINT('Ctrl Pts',(180.464050813976,617.349688765578,-38.5855724216838)) ;
#59503=CARTESIAN_POINT('Ctrl Pts',(180.521067355346,617.345363131574,-38.5644227170943)) ;
#59504=CARTESIAN_POINT('Ctrl Pts',(180.576979882282,617.341060163679,-38.5401406905439)) ;
#59505=CARTESIAN_POINT('Ctrl Pts',(180.63144191744,617.336820795064,-38.5128859853913)) ;
#59506=CARTESIAN_POINT('Ctrl Pts',(180.685876495539,617.332583563729,-38.4856450207099)) ;
#59507=CARTESIAN_POINT('Ctrl Pts',(180.73886209061,617.328409959241,-38.4554344345994)) ;
#59508=CARTESIAN_POINT('Ctrl Pts',(180.790070116881,617.324316560357,-38.4224438033602)) ;
#59509=CARTESIAN_POINT('Ctrl Pts',(180.841271368363,617.320223703028,-38.38945753676)) ;
#59510=CARTESIAN_POINT('Ctrl Pts',(180.890695456401,617.316210998305,-38.3536919176301)) ;
#59511=CARTESIAN_POINT('Ctrl Pts',(180.938031441646,617.31227029805,-38.3153665301434)) ;
#59512=CARTESIAN_POINT('Ctrl Pts',(180.985413050195,617.308325799675,-38.2770042039347)) ;
#59513=CARTESIAN_POINT('Ctrl Pts',(181.030702350892,617.304453294816,-38.2360770441486)) ;
#59514=CARTESIAN_POINT('Ctrl Pts',(181.073606872153,617.300621180435,-38.1928367164287)) ;
#59515=CARTESIAN_POINT('Ctrl Pts',(181.116531800229,617.296787243374,-38.1495758221731)) ;
#59516=CARTESIAN_POINT('Ctrl Pts',(181.157069360915,617.292993425576,-38.1039993639689)) ;
#59517=CARTESIAN_POINT('Ctrl Pts',(181.194949715568,617.289188038191,-38.0563932722058)) ;
#59518=CARTESIAN_POINT('Ctrl Pts',(181.232901550976,617.285375469987,-38.008697347087)) ;
#59519=CARTESIAN_POINT('Ctrl Pts',(181.268185598401,617.281550762776,-37.9589639018266)) ;
#59520=CARTESIAN_POINT('Ctrl Pts',(181.300560023502,617.27764802761,-37.9075177337117)) ;
#59521=CARTESIAN_POINT('Ctrl Pts',(181.326651139868,617.274502744968,-37.8660563655292)) ;
#59522=CARTESIAN_POINT('Ctrl Pts',(181.350852802808,617.271306321776,-37.8234832859932)) ;
#59523=CARTESIAN_POINT('Ctrl Pts',(181.373056836464,617.268022027636,-37.7799871945257)) ;
#59524=CARTESIAN_POINT('Ctrl Pts',(181.373070496917,617.268020007059,-37.7799604346884)) ;
#59525=CARTESIAN_POINT('Ctrl Pts',(181.373084156616,617.268017986449,-37.7799336745013)) ;
#59526=CARTESIAN_POINT('Ctrl Pts',(181.373097815559,617.268015965807,-37.7799069139645)) ;
#59527=CARTESIAN_POINT('Ctrl Pts',(181.398284435998,617.26428996986,-37.7305614064458)) ;
#59528=CARTESIAN_POINT('Ctrl Pts',(181.420987785486,617.26044103349,-37.6798426520705)) ;
#59529=CARTESIAN_POINT('Ctrl Pts',(181.441092167919,617.256532284097,-37.6280356574811)) ;
#59530=CARTESIAN_POINT('Ctrl Pts',(181.442970993693,617.256166997616,-37.6231941102701)) ;
#59531=CARTESIAN_POINT('Ctrl Pts',(181.444827129073,617.255801188755,-37.6183430956054)) ;
#59532=CARTESIAN_POINT('Ctrl Pts',(181.44666048504,617.255434909036,-37.6134828686495)) ;
#59533=CARTESIAN_POINT('Ctrl Pts',(181.468379666709,617.251095710374,-37.5559053146194)) ;
#59534=CARTESIAN_POINT('Ctrl Pts',(181.486901038978,617.246691099595,-37.4970289075518)) ;
#59535=CARTESIAN_POINT('Ctrl Pts',(181.50211674275,617.242292615532,-37.4372466548332)) ;
#59536=CARTESIAN_POINT('Ctrl Pts',(181.517103241382,617.237960389013,-37.378364945384)) ;
#59537=CARTESIAN_POINT('Ctrl Pts',(181.528883363017,617.233634390947,-37.3186044913533)) ;
#59538=CARTESIAN_POINT('Ctrl Pts',(181.53739314816,617.229362469258,-37.2583424046209)) ;
#59539=CARTESIAN_POINT('Ctrl Pts',(181.545897740001,617.225093154612,-37.1981170942769)) ;
#59540=CARTESIAN_POINT('Ctrl Pts',(181.55113611504,617.220877985803,-37.1373907518155)) ;
#59541=CARTESIAN_POINT('Ctrl Pts',(181.553079682457,617.216740970537,-37.0765414751807)) ;
#59542=CARTESIAN_POINT('Ctrl Pts',(181.555022788807,617.212604936685,-37.0157066336646)) ;
#59543=CARTESIAN_POINT('Ctrl Pts',(181.553672620198,617.208547022454,-36.9547489367615)) ;
#59544=CARTESIAN_POINT('Ctrl Pts',(181.549035161303,617.204566464328,-36.8940478445899)) ;
#59545=CARTESIAN_POINT('Ctrl Pts',(181.544267852721,617.200474449854,-36.8316471108539)) ;
#59546=CARTESIAN_POINT('Ctrl Pts',(181.536026230921,617.196464176835,-36.7695176204549)) ;
#59547=CARTESIAN_POINT('Ctrl Pts',(181.524356469931,617.1925084719,-36.7080726968388)) ;
#59548=CARTESIAN_POINT('Ctrl Pts',(181.512989833439,617.188655517234,-36.6482238180451)) ;
#59549=CARTESIAN_POINT('Ctrl Pts',(181.498370712369,617.18485396578,-36.5890245417342)) ;
#59550=CARTESIAN_POINT('Ctrl Pts',(181.480581926585,617.181057197148,-36.5308563210037)) ;
#59551=CARTESIAN_POINT('Ctrl Pts',(181.462081556055,617.177108550662,-36.4703612625095)) ;
#59552=CARTESIAN_POINT('Ctrl Pts',(181.440152039501,617.173164661938,-36.4109817420282)) ;
#59553=CARTESIAN_POINT('Ctrl Pts',(181.414938348395,617.169155014526,-36.3531427996677)) ;
#59554=CARTESIAN_POINT('Ctrl Pts',(181.393112096556,617.165684060042,-36.3030744730292)) ;
#59555=CARTESIAN_POINT('Ctrl Pts',(181.368824610677,617.162163172294,-36.2541596554739)) ;
#59556=CARTESIAN_POINT('Ctrl Pts',(181.34220910718,617.15854155645,-36.2066705884739)) ;
#59557=CARTESIAN_POINT('Ctrl Pts',(181.338093638701,617.157981557806,-36.1993275089659)) ;
#59558=CARTESIAN_POINT('Ctrl Pts',(181.333922525122,617.157419150812,-36.1920184182069)) ;
#59559=CARTESIAN_POINT('Ctrl Pts',(181.329696273981,617.156854147676,-36.184744212076)) ;
#59560=CARTESIAN_POINT('Ctrl Pts',(181.329680599364,617.156852052153,-36.184717232989)) ;
#59561=CARTESIAN_POINT('Ctrl Pts',(181.329664923988,617.156849956594,-36.1846902543819)) ;
#59562=CARTESIAN_POINT('Ctrl Pts',(181.329649247854,617.156847860999,-36.1846632762546)) ;
#59563=CARTESIAN_POINT('Ctrl Pts',(181.301756420849,617.153119131574,-36.1366606097866)) ;
#59564=CARTESIAN_POINT('Ctrl Pts',(181.271355310078,617.149267513494,-36.0900092851452)) ;
#59565=CARTESIAN_POINT('Ctrl Pts',(181.238623991347,617.145356115883,-36.0449615989856)) ;
#59566=CARTESIAN_POINT('Ctrl Pts',(181.235567339023,617.144990845461,-36.0407547683434)) ;
#59567=CARTESIAN_POINT('Ctrl Pts',(181.232490400108,617.144625053704,-36.0365619363146)) ;
#59568=CARTESIAN_POINT('Ctrl Pts',(181.229393341455,617.144258792007,-36.0323833160391)) ;
#59569=CARTESIAN_POINT('Ctrl Pts',(181.192767074204,617.139927327777,-35.9829663433142)) ;
#59570=CARTESIAN_POINT('Ctrl Pts',(181.153321467234,617.135530799576,-35.9355344739163)) ;
#59571=CARTESIAN_POINT('Ctrl Pts',(181.111327896403,617.131140147732,-35.8903898196592)) ;
#59572=CARTESIAN_POINT('Ctrl Pts',(181.069866774346,617.126805166248,-35.8458175676854)) ;
#59573=CARTESIAN_POINT('Ctrl Pts',(181.025922137155,617.1224762055,-35.8034745375498)) ;
#59574=CARTESIAN_POINT('Ctrl Pts',(180.979777570001,617.118200988637,-35.7636194641676)) ;
#59575=CARTESIAN_POINT('Ctrl Pts',(180.933661057763,617.113928371014,-35.7237886218225)) ;
#59576=CARTESIAN_POINT('Ctrl Pts',(180.885347346948,617.109709566932,-35.6864425937983)) ;
#59577=CARTESIAN_POINT('Ctrl Pts',(180.835139953425,617.105568392055,-35.6518109058117)) ;
#59578=CARTESIAN_POINT('Ctrl Pts',(180.784944556286,617.101428206656,-35.6171874926035)) ;
#59579=CARTESIAN_POINT('Ctrl Pts',(180.732856377519,617.097365615128,-35.5852771577545)) ;
#59580=CARTESIAN_POINT('Ctrl Pts',(180.67919880623,617.09337960808,-35.5562811206363)) ;
#59581=CARTESIAN_POINT('Ctrl Pts',(180.624269322871,617.089299115755,-35.5265977544294)) ;
#59582=CARTESIAN_POINT('Ctrl Pts',(180.567695037457,617.085298854405,-35.4999687958035)) ;
#59583=CARTESIAN_POINT('Ctrl Pts',(180.509845044716,617.081351751734,-35.4765778642259)) ;
#59584=CARTESIAN_POINT('Ctrl Pts',(180.453263041289,617.077491163924,-35.4536996285002)) ;
#59585=CARTESIAN_POINT('Ctrl Pts',(180.395460668928,617.073681076396,-35.4339192356413)) ;
#59586=CARTESIAN_POINT('Ctrl Pts',(180.336804723169,617.069874711177,-35.4173745540024)) ;
#59587=CARTESIAN_POINT('Ctrl Pts',(180.276177078602,617.065940396342,-35.4002737287596)) ;
#59588=CARTESIAN_POINT('Ctrl Pts',(180.214637376693,617.062009628139,-35.3866306287752)) ;
#59589=CARTESIAN_POINT('Ctrl Pts',(180.152615030787,617.058013140031,-35.3765526801095)) ;
#59590=CARTESIAN_POINT('Ctrl Pts',(180.098634181558,617.054534815907,-35.3677813861586)) ;
#59591=CARTESIAN_POINT('Ctrl Pts',(180.044286870739,617.051006059877,-35.3617104242035)) ;
#59592=CARTESIAN_POINT('Ctrl Pts',(179.989874428038,617.047376279796,-35.3583759379269)) ;
#59593=CARTESIAN_POINT('Ctrl Pts',(179.981802538768,617.046837815036,-35.3578812789361)) ;
#59594=CARTESIAN_POINT('Ctrl Pts',(179.973729146896,617.046297127075,-35.3574467776772)) ;
#59595=CARTESIAN_POINT('Ctrl Pts',(179.965655161798,617.04575405075,-35.3570724882378)) ;
#59596=CARTESIAN_POINT('Ctrl Pts',(179.965621251352,617.045751769849,-35.3570709162356)) ;
#59597=CARTESIAN_POINT('Ctrl Pts',(179.965587340896,617.045749488906,-35.3570693452956)) ;
#59598=CARTESIAN_POINT('Ctrl Pts',(179.965553430429,617.04574720792,-35.3570677754175)) ;
#59599=CARTESIAN_POINT('Ctrl Pts',(179.910075199561,617.042015468516,-35.3544994222692)) ;
#59600=CARTESIAN_POINT('Ctrl Pts',(179.854372203603,617.038161292594,-35.3547729571841)) ;
#59601=CARTESIAN_POINT('Ctrl Pts',(179.79875385633,617.034248155015,-35.3578755092052)) ;
#59602=CARTESIAN_POINT('Ctrl Pts',(179.793694805022,617.033892215568,-35.3581577176963)) ;
#59603=CARTESIAN_POINT('Ctrl Pts',(179.788636482925,617.033535788287,-35.3584633118414)) ;
#59604=CARTESIAN_POINT('Ctrl Pts',(179.783579139854,617.033178920942,-35.3587922690107)) ;
#59605=CARTESIAN_POINT('Ctrl Pts',(179.722178408227,617.028846227719,-35.362786107392)) ;
#59606=CARTESIAN_POINT('Ctrl Pts',(179.660916913678,617.024449330578,-35.3702268616423)) ;
#59607=CARTESIAN_POINT('Ctrl Pts',(179.600196733796,617.020059248428,-35.3810502102344)) ;
#59608=CARTESIAN_POINT('Ctrl Pts',(179.540372919564,617.015733973708,-35.3917137819958)) ;
#59609=CARTESIAN_POINT('Ctrl Pts',(179.481074384113,617.011415593643,-35.4056604068221)) ;
#59610=CARTESIAN_POINT('Ctrl Pts',(179.422671023473,617.007151276808,-35.4227924252981)) ;
#59611=CARTESIAN_POINT('Ctrl Pts',(179.364301587598,617.002889436988,-35.4399144922975)) ;
#59612=CARTESIAN_POINT('Ctrl Pts',(179.306826223232,616.998681728917,-35.460218144617)) ;
#59613=CARTESIAN_POINT('Ctrl Pts',(179.250601206137,616.994551313171,-35.4835731411944)) ;
#59614=CARTESIAN_POINT('Ctrl Pts',(179.194387866254,616.990421755259,-35.5069232872396)) ;
#59615=CARTESIAN_POINT('Ctrl Pts',(179.139424385703,616.986369457334,-35.5333235335825)) ;
#59616=CARTESIAN_POINT('Ctrl Pts',(179.086054084856,616.982392692462,-35.5626115586872)) ;
#59617=CARTESIAN_POINT('Ctrl Pts',(179.03122286064,616.978307070254,-35.5927012948489)) ;
#59618=CARTESIAN_POINT('Ctrl Pts',(178.978073437803,616.974301158905,-35.6258393683047)) ;
#59619=CARTESIAN_POINT('Ctrl Pts',(178.92696280325,616.970346727896,-35.6618131631219)) ;
#59620=CARTESIAN_POINT('Ctrl Pts',(178.877145801042,616.966492385252,-35.6968764455774)) ;
#59621=CARTESIAN_POINT('Ctrl Pts',(178.829265868988,616.962686579411,-35.7346337876853)) ;
#59622=CARTESIAN_POINT('Ctrl Pts',(178.783636576234,616.958881672114,-35.7748517693634)) ;
#59623=CARTESIAN_POINT('Ctrl Pts',(178.736229952656,616.954928557852,-35.8166363030122)) ;
#59624=CARTESIAN_POINT('Ctrl Pts',(178.691253370136,616.950975984402,-35.8610775107474)) ;
#59625=CARTESIAN_POINT('Ctrl Pts',(178.64903346043,616.946952659638,-35.9078679213963)) ;
#59626=CARTESIAN_POINT('Ctrl Pts',(178.612588289104,616.943479635624,-35.9482584514652)) ;
#59627=CARTESIAN_POINT('Ctrl Pts',(178.578196485834,616.939953228555,-35.9904000939721)) ;
#59628=CARTESIAN_POINT('Ctrl Pts',(178.546049053209,616.936322818761,-36.0340609455452)) ;
#59629=CARTESIAN_POINT('Ctrl Pts',(178.540976461048,616.935749970892,-36.0409502575478)) ;
#59630=CARTESIAN_POINT('Ctrl Pts',(178.535959647509,616.935174533547,-36.0478774219443)) ;
#59631=CARTESIAN_POINT('Ctrl Pts',(178.530999248853,616.934596307854,-36.0548415611402)) ;
#59632=CARTESIAN_POINT('Ctrl Pts',(178.530978547663,616.93459389475,-36.054870624524)) ;
#59633=CARTESIAN_POINT('Ctrl Pts',(178.530957847456,616.934591481597,-36.0548996885518)) ;
#59634=CARTESIAN_POINT('Ctrl Pts',(178.53093714823,616.934589068395,-36.0549287532235)) ;
#59635=CARTESIAN_POINT('Ctrl Pts',(178.499041670027,616.93087056117,-36.099714564886)) ;
#59636=CARTESIAN_POINT('Ctrl Pts',(178.469366274533,616.927026440125,-36.146202366481)) ;
#59637=CARTESIAN_POINT('Ctrl Pts',(178.442065521419,616.923119508642,-36.1941322661498)) ;
#59638=CARTESIAN_POINT('Ctrl Pts',(178.439400200466,616.922738082302,-36.1988115717106)) ;
#59639=CARTESIAN_POINT('Ctrl Pts',(178.436757509736,616.9223560573,-36.203504581388)) ;
#59640=CARTESIAN_POINT('Ctrl Pts',(178.4341375904,616.921973492075,-36.2082110269501)) ;
#59641=CARTESIAN_POINT('Ctrl Pts',(178.404212362585,616.917603757737,-36.2619689628102)) ;
#59642=CARTESIAN_POINT('Ctrl Pts',(178.377258123467,616.913164238395,-36.317485980025)) ;
#59643=CARTESIAN_POINT('Ctrl Pts',(178.353440625791,616.908728220843,-36.3743877416019)) ;
#59644=CARTESIAN_POINT('Ctrl Pts',(178.330063871458,616.904374291898,-36.4302365347711)) ;
#59645=CARTESIAN_POINT('Ctrl Pts',(178.309708369483,616.900024020985,-36.4874192037108)) ;
#59646=CARTESIAN_POINT('Ctrl Pts',(178.292492160655,616.895726470822,-36.5455744061963)) ;
#59647=CARTESIAN_POINT('Ctrl Pts',(178.275286911396,616.891431656411,-36.603692587987)) ;
#59648=CARTESIAN_POINT('Ctrl Pts',(178.261216825728,616.887189638468,-36.662782052018)) ;
#59649=CARTESIAN_POINT('Ctrl Pts',(178.250364993454,616.883025817115,-36.7224753350455)) ;
#59650=CARTESIAN_POINT('Ctrl Pts',(178.23951594627,616.878863064394,-36.7821532979702)) ;
#59651=CARTESIAN_POINT('Ctrl Pts',(178.231883527854,616.874778478766,-36.8424347474778)) ;
#59652=CARTESIAN_POINT('Ctrl Pts',(178.2275167976,616.870772761268,-36.9029459335317)) ;
#59653=CARTESIAN_POINT('Ctrl Pts',(178.223000286466,616.866629645796,-36.9655326814236)) ;
#59654=CARTESIAN_POINT('Ctrl Pts',(178.221977733339,616.862570931832,-37.0283651792618)) ;
#59655=CARTESIAN_POINT('Ctrl Pts',(178.224463587513,616.858570423963,-37.0910230850861)) ;
#59656=CARTESIAN_POINT('Ctrl Pts',(178.226870116644,616.854697574613,-37.1516815409108)) ;
#59657=CARTESIAN_POINT('Ctrl Pts',(178.23256480618,616.850878896739,-37.212176243007)) ;
#59658=CARTESIAN_POINT('Ctrl Pts',(178.241521117425,616.847068824741,-37.2721207145744)) ;
#59659=CARTESIAN_POINT('Ctrl Pts',(178.25092026132,616.843070368906,-37.3350290591588)) ;
#59660=CARTESIAN_POINT('Ctrl Pts',(178.263912478694,616.839081015093,-37.3973311977644)) ;
#59661=CARTESIAN_POINT('Ctrl Pts',(178.280414158202,616.835028919848,-37.4585771180169)) ;
#59662=CARTESIAN_POINT('Ctrl Pts',(178.294643595531,616.83153478852,-37.5113896201309)) ;
#59663=CARTESIAN_POINT('Ctrl Pts',(178.311482658404,616.827993342589,-37.5634177529276)) ;
#59664=CARTESIAN_POINT('Ctrl Pts',(178.330837982447,616.824352802783,-37.6143707302497)) ;
#59665=CARTESIAN_POINT('Ctrl Pts',(178.333922252396,616.823772682941,-37.6224900847196)) ;
#59666=CARTESIAN_POINT('Ctrl Pts',(178.337070385027,616.823190046867,-37.6305822413713)) ;
#59667=CARTESIAN_POINT('Ctrl Pts',(178.340281970335,616.822604685048,-37.6386461419468)) ;
#59668=CARTESIAN_POINT('Ctrl Pts',(178.340288743505,616.822603450531,-37.6386631485557)) ;
#59669=CARTESIAN_POINT('Ctrl Pts',(178.340295516958,616.822602216003,-37.6386801550389)) ;
#59670=CARTESIAN_POINT('Ctrl Pts',(178.340302290693,616.822600981462,-37.6386971613965)) ;
#59671=CARTESIAN_POINT('Ctrl Pts',(178.361103043185,616.818809959359,-37.6909202003039)) ;
#59672=CARTESIAN_POINT('Ctrl Pts',(178.384645358417,616.81489472151,-37.7421380766257)) ;
#59673=CARTESIAN_POINT('Ctrl Pts',(178.410786328454,616.810917637055,-37.7920713750955)) ;
#59674=CARTESIAN_POINT('Ctrl Pts',(178.413407689976,616.810518823387,-37.7970785812978)) ;
#59675=CARTESIAN_POINT('Ctrl Pts',(178.416055144893,616.81011938781,-37.8020728492216)) ;
#59676=CARTESIAN_POINT('Ctrl Pts',(178.418728523548,616.809719393216,-37.8070538837687)) ;
#59677=CARTESIAN_POINT('Ctrl Pts',(178.447999575829,616.805339818079,-37.8615916584148)) ;
#59678=CARTESIAN_POINT('Ctrl Pts',(178.480383390813,616.800893861143,-37.9145463535274)) ;
#59679=CARTESIAN_POINT('Ctrl Pts',(178.515655526665,616.796450665732,-37.965580102408)) ;
#59680=CARTESIAN_POINT('Ctrl Pts',(178.550884077367,616.792012960698,-38.0165507897931)) ;
#59681=CARTESIAN_POINT('Ctrl Pts',(178.588993588597,616.787578349975,-38.0656055793173)) ;
#59682=CARTESIAN_POINT('Ctrl Pts',(178.62973396628,616.783195130616,-38.1124361119914)) ;
#59683=CARTESIAN_POINT('Ctrl Pts',(178.670436832959,616.778815947031,-38.1592235262559)) ;
#59684=CARTESIAN_POINT('Ctrl Pts',(178.713765681151,616.774488196203,-38.203790917384)) ;
#59685=CARTESIAN_POINT('Ctrl Pts',(178.759446552293,616.770235991496,-38.2458556574152)) ;
#59686=CARTESIAN_POINT('Ctrl Pts',(178.80509973814,616.765986363875,-38.287894903739)) ;
#59687=CARTESIAN_POINT('Ctrl Pts',(178.853102149004,616.761812183564,-38.3274345100296)) ;
#59688=CARTESIAN_POINT('Ctrl Pts',(178.903155657434,616.757712558082,-38.3642163568452)) ;
#59689=CARTESIAN_POINT('Ctrl Pts',(178.953214146788,616.753612524639,-38.4010018638952)) ;
#59690=CARTESIAN_POINT('Ctrl Pts',(179.005324252406,616.749586926448,-38.4350288880954)) ;
#59691=CARTESIAN_POINT('Ctrl Pts',(179.059161832729,616.745610946358,-38.4660647118646)) ;
#59692=CARTESIAN_POINT('Ctrl Pts',(179.112997641711,616.741635097085,-38.4970995145057)) ;
#59693=CARTESIAN_POINT('Ctrl Pts',(179.168560950204,616.737708570083,-38.5251429685137)) ;
#59694=CARTESIAN_POINT('Ctrl Pts',(179.225499824143,616.733785788633,-38.5499917127387)) ;
#59695=CARTESIAN_POINT('Ctrl Pts',(179.282495967825,616.729859061606,-38.5748654501032)) ;
#59696=CARTESIAN_POINT('Ctrl Pts',(179.340870547703,616.725935583558,-38.5965374738112)) ;
#59697=CARTESIAN_POINT('Ctrl Pts',(179.40024076439,616.721954749816,-38.6148400532057)) ;
#59698=CARTESIAN_POINT('Ctrl Pts',(179.455832998681,616.718227233657,-38.6319779607059)) ;
#59699=CARTESIAN_POINT('Ctrl Pts',(179.512297835651,616.714448772708,-38.6461613739341)) ;
#59700=CARTESIAN_POINT('Ctrl Pts',(179.569297170793,616.710565160536,-38.6572894990112)) ;
#59701=CARTESIAN_POINT('Origin',(179.888527625422,616.710565160536,-37.0221601717597)) ;
#59702=CARTESIAN_POINT('Ctrl Pts',(180.464060729575,617.544113575794,-38.585591540904)) ;
#59703=CARTESIAN_POINT('Ctrl Pts',(180.487228259808,617.54247185516,-38.5770630689456)) ;
#59704=CARTESIAN_POINT('Ctrl Pts',(180.510205228593,617.54081290889,-38.5680200076004)) ;
#59705=CARTESIAN_POINT('Ctrl Pts',(180.598264253176,617.534329295097,-38.5310812183154)) ;
#59706=CARTESIAN_POINT('Ctrl Pts',(180.661732357622,617.529382284152,-38.4995635541931)) ;
#59707=CARTESIAN_POINT('Ctrl Pts',(180.814529967429,617.516779470276,-38.4111381976683)) ;
#59708=CARTESIAN_POINT('Ctrl Pts',(180.900808349455,617.509009249844,-38.3495731762099)) ;
#59709=CARTESIAN_POINT('Ctrl Pts',(181.02252012136,617.49736285427,-38.2439169440387)) ;
#59710=CARTESIAN_POINT('Ctrl Pts',(181.062544230677,617.4934042498,-38.2055091790602)) ;
#59711=CARTESIAN_POINT('Ctrl Pts',(181.121210631552,617.487486759853,-38.1432991555566)) ;
#59712=CARTESIAN_POINT('Ctrl Pts',(181.141244782052,617.485444870038,-38.1208686359069)) ;
#59713=CARTESIAN_POINT('Ctrl Pts',(181.188402366363,617.480597787042,-38.0651016607649)) ;
#59714=CARTESIAN_POINT('Ctrl Pts',(181.214863737876,617.477834830551,-38.0312362765351)) ;
#59715=CARTESIAN_POINT('Ctrl Pts',(181.27640650444,617.471193517949,-37.9458628722803)) ;
#59716=CARTESIAN_POINT('Ctrl Pts',(181.309965329618,617.46737642322,-37.893337728381)) ;
#59717=CARTESIAN_POINT('Ctrl Pts',(181.398989250749,617.456283390246,-37.7351031546239)) ;
#59718=CARTESIAN_POINT('Ctrl Pts',(181.44613467645,617.449045828247,-37.6251848230472)) ;
#59719=CARTESIAN_POINT('Ctrl Pts',(181.496308291822,617.438080488535,-37.4617822287019)) ;
#59720=CARTESIAN_POINT('Ctrl Pts',(181.50916818018,617.434699240502,-37.4117104832382)) ;
#59721=CARTESIAN_POINT('Ctrl Pts',(181.531369068561,617.42739201278,-37.3048767218375)) ;
#59722=CARTESIAN_POINT('Ctrl Pts',(181.540139374621,617.423452018443,-37.2480669562751)) ;
#59723=CARTESIAN_POINT('Ctrl Pts',(181.552805283756,617.414690183658,-37.1236745399862)) ;
#59724=CARTESIAN_POINT('Ctrl Pts',(181.555552878684,617.409842640143,-37.0560780101603)) ;
#59725=CARTESIAN_POINT('Ctrl Pts',(181.55183161418,617.396485359588,-36.8718907693089)) ;
#59726=CARTESIAN_POINT('Ctrl Pts',(181.537235299013,617.387889720624,-36.7558388670058)) ;
#59727=CARTESIAN_POINT('Ctrl Pts',(181.503417768927,617.377549023494,-36.6114444148363)) ;
#59728=CARTESIAN_POINT('Ctrl Pts',(181.495323354846,617.375380372175,-36.5808374754927)) ;
#59729=CARTESIAN_POINT('Ctrl Pts',(181.475778917983,617.370764665774,-36.5146307816251)) ;
#59730=CARTESIAN_POINT('Ctrl Pts',(181.463993473597,617.368335480354,-36.4791494249022)) ;
#59731=CARTESIAN_POINT('Ctrl Pts',(181.413956652883,617.359140256472,-36.3439020594885)) ;
#59732=CARTESIAN_POINT('Ctrl Pts',(181.367336133876,617.35271142634,-36.2475003903021)) ;
#59733=CARTESIAN_POINT('Ctrl Pts',(181.264639212964,617.340621636482,-36.0787061870358)) ;
#59734=CARTESIAN_POINT('Ctrl Pts',(181.211231081331,617.335011868706,-36.0051836672477)) ;
#59735=CARTESIAN_POINT('Ctrl Pts',(181.119272786496,617.325924136133,-35.8981670026294)) ;
#59736=CARTESIAN_POINT('Ctrl Pts',(181.084724634698,617.322614635726,-35.8614680953434)) ;
#59737=CARTESIAN_POINT('Ctrl Pts',(181.005758281013,617.315223312717,-35.7848609089031)) ;
#59738=CARTESIAN_POINT('Ctrl Pts',(180.960752412362,617.31111621247,-35.7456625238566)) ;
#59739=CARTESIAN_POINT('Ctrl Pts',(180.85632288467,617.301794342589,-35.6641337814623)) ;
#59740=CARTESIAN_POINT('Ctrl Pts',(180.796025743465,617.296544107431,-35.6231217188557)) ;
#59741=CARTESIAN_POINT('Ctrl Pts',(180.640921235174,617.283464816743,-35.5318806821652)) ;
#59742=CARTESIAN_POINT('Ctrl Pts',(180.543569190138,617.27560524913,-35.4865973621708)) ;
#59743=CARTESIAN_POINT('Ctrl Pts',(180.413194050154,617.265986146595,-35.4406263574173)) ;
#59744=CARTESIAN_POINT('Ctrl Pts',(180.383562890426,617.263859232689,-35.431102416498)) ;
#59745=CARTESIAN_POINT('Ctrl Pts',(180.316529223903,617.259200903316,-35.4116114343015)) ;
#59746=CARTESIAN_POINT('Ctrl Pts',(180.279012906293,617.25669325476,-35.4021063274235)) ;
#59747=CARTESIAN_POINT('Ctrl Pts',(180.190361868786,617.250925295162,-35.3829050293004)) ;
#59748=CARTESIAN_POINT('Ctrl Pts',(180.13903628989,617.247705932207,-35.3742804706709)) ;
#59749=CARTESIAN_POINT('Ctrl Pts',(179.95021003229,617.236034891206,-35.3515791153275)) ;
#59750=CARTESIAN_POINT('Ctrl Pts',(179.811526663085,617.227744455219,-35.3522158946241)) ;
#59751=CARTESIAN_POINT('Ctrl Pts',(179.623314558065,617.215567638189,-35.376595360912)) ;
#59752=CARTESIAN_POINT('Ctrl Pts',(179.572454955257,617.212188742156,-35.3856032325347)) ;
#59753=CARTESIAN_POINT('Ctrl Pts',(179.465904619507,617.204873098296,-35.4096266942594)) ;
#59754=CARTESIAN_POINT('Ctrl Pts',(179.410411295285,617.200921696622,-35.4252012566082)) ;
#59755=CARTESIAN_POINT('Ctrl Pts',(179.291449808206,617.192121917137,-35.4653453175336)) ;
#59756=CARTESIAN_POINT('Ctrl Pts',(179.228454648776,617.187247210815,-35.4909918645347)) ;
#59757=CARTESIAN_POINT('Ctrl Pts',(179.06323587317,617.173956964152,-35.5703497614573)) ;
#59758=CARTESIAN_POINT('Ctrl Pts',(178.964727400564,617.165461933159,-35.6309534828837)) ;
#59759=CARTESIAN_POINT('Ctrl Pts',(178.848055629101,617.155198408885,-35.7206283528762)) ;
#59760=CARTESIAN_POINT('Ctrl Pts',(178.823401220682,617.153018832484,-35.7407260444342)) ;
#59761=CARTESIAN_POINT('Ctrl Pts',(178.771131236274,617.148398800956,-35.7858873849874)) ;
#59762=CARTESIAN_POINT('Ctrl Pts',(178.743751859662,617.145975444034,-35.8111960524104)) ;
#59763=CARTESIAN_POINT('Ctrl Pts',(178.641725376111,617.136823836361,-35.912062543586)) ;
#59764=CARTESIAN_POINT('Ctrl Pts',(178.573512241876,617.130429170258,-35.9937771284451)) ;
#59765=CARTESIAN_POINT('Ctrl Pts',(178.462018006044,617.118346099454,-36.1567404778624)) ;
#59766=CARTESIAN_POINT('Ctrl Pts',(178.416776960854,617.112705913602,-36.236139802998)) ;
#59767=CARTESIAN_POINT('Ctrl Pts',(178.357004338013,617.103586191004,-36.3644910274877)) ;
#59768=CARTESIAN_POINT('Ctrl Pts',(178.337826770242,617.100277869931,-36.411080612624)) ;
#59769=CARTESIAN_POINT('Ctrl Pts',(178.300632149563,617.092892382787,-36.5145252269169)) ;
#59770=CARTESIAN_POINT('Ctrl Pts',(178.28349857953,617.088790104647,-36.5716210725207)) ;
#59771=CARTESIAN_POINT('Ctrl Pts',(178.252336116539,617.079486436461,-36.7001160867461)) ;
#59772=CARTESIAN_POINT('Ctrl Pts',(178.239850899794,617.074249916677,-36.7717641053334)) ;
#59773=CARTESIAN_POINT('Ctrl Pts',(178.220532786075,617.061117841501,-36.9513657376716)) ;
#59774=CARTESIAN_POINT('Ctrl Pts',(178.219450268508,617.053188866332,-37.0596161349644)) ;
#59775=CARTESIAN_POINT('Ctrl Pts',(178.231557357831,617.043513198459,-37.1981407962776)) ;
#59776=CARTESIAN_POINT('Ctrl Pts',(178.235124343208,617.041391167387,-37.2289882729264)) ;
#59777=CARTESIAN_POINT('Ctrl Pts',(178.245062069491,617.036740668009,-37.2979679740585)) ;
#59778=CARTESIAN_POINT('Ctrl Pts',(178.251901199839,617.034236020005,-37.3360128886887)) ;
#59779=CARTESIAN_POINT('Ctrl Pts',(178.271021189482,617.028475398674,-37.4245616654215)) ;
#59780=CARTESIAN_POINT('Ctrl Pts',(178.2843535863,617.025260287678,-37.4747973884619)) ;
#59781=CARTESIAN_POINT('Ctrl Pts',(178.341537898242,617.013617805404,-37.6556882475495)) ;
#59782=CARTESIAN_POINT('Ctrl Pts',(178.399190595616,617.005351022861,-37.7813752338753)) ;
#59783=CARTESIAN_POINT('Ctrl Pts',(178.498673764095,616.993216947292,-37.9422148638106)) ;
#59784=CARTESIAN_POINT('Ctrl Pts',(178.52769655212,616.98985543118,-37.9846217154074)) ;
#59785=CARTESIAN_POINT('Ctrl Pts',(178.592964375516,616.982597822027,-38.0711222828626)) ;
#59786=CARTESIAN_POINT('Ctrl Pts',(178.629608481935,616.978688092588,-38.1148297682013)) ;
#59787=CARTESIAN_POINT('Ctrl Pts',(178.713874978571,616.970014753276,-38.205462398813)) ;
#59788=CARTESIAN_POINT('Ctrl Pts',(178.762226758882,616.965226466012,-38.2515737338429)) ;
#59789=CARTESIAN_POINT('Ctrl Pts',(178.905026198199,616.951662503466,-38.3722458681657)) ;
#59790=CARTESIAN_POINT('Ctrl Pts',(179.004974215103,616.94278270056,-38.4396730858431)) ;
#59791=CARTESIAN_POINT('Ctrl Pts',(179.139025842964,616.932217469467,-38.5103754587916)) ;
#59792=CARTESIAN_POINT('Ctrl Pts',(179.16714957219,616.930071729297,-38.5242094426074)) ;
#59793=CARTESIAN_POINT('Ctrl Pts',(179.230670040116,616.925402451974,-38.5532585032686)) ;
#59794=CARTESIAN_POINT('Ctrl Pts',(179.266236107803,616.922901044047,-38.5680555656971)) ;
#59795=CARTESIAN_POINT('Ctrl Pts',(179.350445356438,616.91716668458,-38.5997122333386)) ;
#59796=CARTESIAN_POINT('Ctrl Pts',(179.399420487653,616.913973055928,-38.615577250843)) ;
#59797=CARTESIAN_POINT('Ctrl Pts',(179.58278955523,616.902274090356,-38.6657242579006)) ;
#59798=CARTESIAN_POINT('Ctrl Pts',(179.720553916021,616.893934831471,-38.6854583440229)) ;
#59799=CARTESIAN_POINT('Ctrl Pts',(179.910889613995,616.881693872816,-38.6888130582876)) ;
#59800=CARTESIAN_POINT('Ctrl Pts',(179.962619718989,616.878301359716,-38.687315207343)) ;
#59801=CARTESIAN_POINT('Ctrl Pts',(180.072718072115,616.870891710868,-38.6789868878036)) ;
#59802=CARTESIAN_POINT('Ctrl Pts',(180.130961974825,616.866856791597,-38.6714706279383)) ;
#59803=CARTESIAN_POINT('Ctrl Pts',(180.282456566663,616.85603692188,-38.6437225766261)) ;
#59804=CARTESIAN_POINT('Ctrl Pts',(180.374572525789,616.849118914138,-38.6185312683209)) ;
#59805=CARTESIAN_POINT('Ctrl Pts',(180.464017215185,616.842172979815,-38.58560755881)) ;
#59806=CARTESIAN_POINT('Origin',(179.888527625422,617.710565160536,-37.0221601717597)) ;
#59807=CARTESIAN_POINT('',(180.464060715702,618.242141445689,-38.5855915460107)) ;
#59808=CARTESIAN_POINT('',(180.464060715494,618.051541226924,-38.5855915460876)) ;
#59809=CARTESIAN_POINT('',(180.464060715702,617.710565160536,-38.5855915460107)) ;
#59810=CARTESIAN_POINT('',(179.889570327489,618.281200386648,-38.688647256677)) ;
#59811=CARTESIAN_POINT('Ctrl Pts',(179.889549821694,618.280920770248,-38.6881598581687)) ;
#59812=CARTESIAN_POINT('Ctrl Pts',(179.935372015437,618.277609385829,-38.6881317433521)) ;
#59813=CARTESIAN_POINT('Ctrl Pts',(179.981177137719,618.274325601274,-38.6862131676218)) ;
#59814=CARTESIAN_POINT('Ctrl Pts',(180.057497874022,618.268952524589,-38.6798546522522)) ;
#59815=CARTESIAN_POINT('Ctrl Pts',(180.088073891955,618.266826693261,-38.6764526338771)) ;
#59816=CARTESIAN_POINT('Ctrl Pts',(180.150064623838,618.262594201886,-38.6678112488637)) ;
#59817=CARTESIAN_POINT('Ctrl Pts',(180.181456640678,618.260495094555,-38.6625143410322)) ;
#59818=CARTESIAN_POINT('Ctrl Pts',(180.298227785343,618.252793862451,-38.6393516539469)) ;
#59819=CARTESIAN_POINT('Ctrl Pts',(180.382278599981,618.247457897413,-38.6156973214008)) ;
#59820=CARTESIAN_POINT('Ctrl Pts',(180.464060715702,618.242141445689,-38.5855915460107)) ;
#59821=CARTESIAN_POINT('',(180.967886278469,618.710565160535,-35.7530892919062)) ;
#59822=CARTESIAN_POINT('Ctrl Pts',(179.889570327489,618.281200386648,-38.688647256677)) ;
#59823=CARTESIAN_POINT('Ctrl Pts',(179.829704746323,618.285448698176,-38.6885516393912)) ;
#59824=CARTESIAN_POINT('Ctrl Pts',(179.769739180832,618.289736185626,-38.6852034082082)) ;
#59825=CARTESIAN_POINT('Ctrl Pts',(179.710050946309,618.294002899686,-38.6786274687905)) ;
#59826=CARTESIAN_POINT('Ctrl Pts',(179.650427244363,618.298265000742,-38.6720586390204)) ;
#59827=CARTESIAN_POINT('Ctrl Pts',(179.591080237905,618.302506114863,-38.6622693141872)) ;
#59828=CARTESIAN_POINT('Ctrl Pts',(179.532377447291,618.306686786384,-38.6493212577048)) ;
#59829=CARTESIAN_POINT('Ctrl Pts',(179.47371511148,618.310864576811,-38.6363821243258)) ;
#59830=CARTESIAN_POINT('Ctrl Pts',(179.415696123102,618.314981909742,-38.6202886814295)) ;
#59831=CARTESIAN_POINT('Ctrl Pts',(179.358678843421,618.319022312191,-38.6011372402441)) ;
#59832=CARTESIAN_POINT('Ctrl Pts',(179.301678310872,618.323061527892,-38.5819914242253)) ;
#59833=CARTESIAN_POINT('Ctrl Pts',(179.24567899163,618.327023880714,-38.5597893633856)) ;
#59834=CARTESIAN_POINT('Ctrl Pts',(179.191029694323,618.330916357404,-38.5346617854854)) ;
#59835=CARTESIAN_POINT('Ctrl Pts',(179.136336185405,618.334811983132,-38.5095138792235)) ;
#59836=CARTESIAN_POINT('Ctrl Pts',(179.082995057282,618.338637757528,-38.481435580952)) ;
#59837=CARTESIAN_POINT('Ctrl Pts',(179.031344721663,618.342422989758,-38.450593880277)) ;
#59838=CARTESIAN_POINT('Ctrl Pts',(178.979675054896,618.346209638685,-38.419740636492)) ;
#59839=CARTESIAN_POINT('Ctrl Pts',(178.929697728594,618.349956005156,-38.3861216980553)) ;
#59840=CARTESIAN_POINT('Ctrl Pts',(178.881736917209,618.353710573408,-38.3499429252659)) ;
#59841=CARTESIAN_POINT('Ctrl Pts',(178.833687107688,618.357472108798,-38.3136970175966)) ;
#59842=CARTESIAN_POINT('Ctrl Pts',(178.787661776309,618.361242367052,-38.2748814771352)) ;
#59843=CARTESIAN_POINT('Ctrl Pts',(178.743966658101,618.365083510243,-38.2337460600409)) ;
#59844=CARTESIAN_POINT('Ctrl Pts',(178.705730437837,618.368444773542,-38.1977497535161)) ;
#59845=CARTESIAN_POINT('Ctrl Pts',(178.669278595077,618.371860843973,-38.1599775677742)) ;
#59846=CARTESIAN_POINT('Ctrl Pts',(178.634797890773,618.375376290139,-38.1206260862659)) ;
#59847=CARTESIAN_POINT('Ctrl Pts',(178.634775519202,618.375378571011,-38.1206005544658)) ;
#59848=CARTESIAN_POINT('Ctrl Pts',(178.63475314846,618.375380851924,-38.1205750220006)) ;
#59849=CARTESIAN_POINT('Ctrl Pts',(178.634730778545,618.375383132879,-38.1205494888704)) ;
#59850=CARTESIAN_POINT('Ctrl Pts',(178.598132648023,618.379114872309,-38.078776203119)) ;
#59851=CARTESIAN_POINT('Ctrl Pts',(178.563616256322,618.38296904822,-38.0350553006912)) ;
#59852=CARTESIAN_POINT('Ctrl Pts',(178.531364456865,618.386882185751,-37.9896367159316)) ;
#59853=CARTESIAN_POINT('Ctrl Pts',(178.52843083029,618.387238125093,-37.9855054373826)) ;
#59854=CARTESIAN_POINT('Ctrl Pts',(178.525515942001,618.387594552267,-37.981360148246)) ;
#59855=CARTESIAN_POINT('Ctrl Pts',(178.522619930061,618.387951419504,-37.9772010579421)) ;
#59856=CARTESIAN_POINT('Ctrl Pts',(178.487459707981,618.392284112733,-37.9267059143508)) ;
#59857=CARTESIAN_POINT('Ctrl Pts',(178.455081206244,618.396681009839,-37.8741705136963)) ;
#59858=CARTESIAN_POINT('Ctrl Pts',(178.425684827552,618.401071091914,-37.8199493167374)) ;
#59859=CARTESIAN_POINT('Ctrl Pts',(178.396722406297,618.405396366388,-37.7665285480182)) ;
#59860=CARTESIAN_POINT('Ctrl Pts',(178.370654285138,618.409714746169,-37.7114715087366)) ;
#59861=CARTESIAN_POINT('Ctrl Pts',(178.347634737273,618.413979062684,-37.6551282848904)) ;
#59862=CARTESIAN_POINT('Ctrl Pts',(178.324628560771,618.418240902185,-37.5988177891295)) ;
#59863=CARTESIAN_POINT('Ctrl Pts',(178.304667292194,618.422448609902,-37.5412226206631)) ;
#59864=CARTESIAN_POINT('Ctrl Pts',(178.287871239278,618.426579025262,-37.4827025310582)) ;
#59865=CARTESIAN_POINT('Ctrl Pts',(178.271078674683,618.430708582788,-37.4241945953139)) ;
#59866=CARTESIAN_POINT('Ctrl Pts',(178.257450048961,618.434760880296,-37.3647621325426)) ;
#59867=CARTESIAN_POINT('Ctrl Pts',(178.247072510769,618.438737644718,-37.3047747672279)) ;
#59868=CARTESIAN_POINT('Ctrl Pts',(178.236410903974,618.442823266741,-37.2431453431988)) ;
#59869=CARTESIAN_POINT('Ctrl Pts',(178.229181169598,618.446829177861,-37.1809301971565)) ;
#59870=CARTESIAN_POINT('Ctrl Pts',(178.22543965551,618.450783608598,-37.1185409966365)) ;
#59871=CARTESIAN_POINT('Ctrl Pts',(178.221792841014,618.454637950716,-37.0577308979622)) ;
#59872=CARTESIAN_POINT('Ctrl Pts',(178.221460070539,618.458443755999,-36.9967555430253)) ;
#59873=CARTESIAN_POINT('Ctrl Pts',(178.224454356076,618.462248662701,-36.9360056250828)) ;
#59874=CARTESIAN_POINT('Ctrl Pts',(178.227565273931,618.46620177674,-36.8728893985096)) ;
#59875=CARTESIAN_POINT('Ctrl Pts',(178.234268369628,618.470154349927,-36.8100166453997)) ;
#59876=CARTESIAN_POINT('Ctrl Pts',(178.244526904074,618.474177674403,-36.7478344419943)) ;
#59877=CARTESIAN_POINT('Ctrl Pts',(178.253382299866,618.477650697846,-36.6941573767934)) ;
#59878=CARTESIAN_POINT('Ctrl Pts',(178.264887024461,618.481177104316,-36.6409938986677)) ;
#59879=CARTESIAN_POINT('Ctrl Pts',(178.278978856662,618.484807513478,-36.588637928831)) ;
#59880=CARTESIAN_POINT('Ctrl Pts',(178.281202429831,618.485380361657,-36.5803765950255)) ;
#59881=CARTESIAN_POINT('Ctrl Pts',(178.283490374685,618.485955799315,-36.5721352701504)) ;
#59882=CARTESIAN_POINT('Ctrl Pts',(178.285842401795,618.486534025323,-36.5639149988284)) ;
#59883=CARTESIAN_POINT('Ctrl Pts',(178.285852217406,618.486536438409,-36.5638806935319)) ;
#59884=CARTESIAN_POINT('Ctrl Pts',(178.285862034133,618.486538851542,-36.563846388602)) ;
#59885=CARTESIAN_POINT('Ctrl Pts',(178.285871851977,618.486541264725,-36.5638120840387)) ;
#59886=CARTESIAN_POINT('Ctrl Pts',(178.301000305292,618.49025977141,-36.5109516979469)) ;
#59887=CARTESIAN_POINT('Ctrl Pts',(178.318843626882,618.494103891889,-36.4587658691368)) ;
#59888=CARTESIAN_POINT('Ctrl Pts',(178.339294991459,618.498010822778,-36.4075374771681)) ;
#59889=CARTESIAN_POINT('Ctrl Pts',(178.341291618342,618.49839224883,-36.4025361490564)) ;
#59890=CARTESIAN_POINT('Ctrl Pts',(178.343313069218,618.498774273543,-36.3975439695781)) ;
#59891=CARTESIAN_POINT('Ctrl Pts',(178.345359222393,618.499156838477,-36.3925612163449)) ;
#59892=CARTESIAN_POINT('Ctrl Pts',(178.368730796001,618.503526572189,-36.3356472055365)) ;
#59893=CARTESIAN_POINT('Ctrl Pts',(178.395330056032,618.507966090875,-36.279959238087)) ;
#59894=CARTESIAN_POINT('Ctrl Pts',(178.424967679135,618.512402107738,-36.2258603000353)) ;
#59895=CARTESIAN_POINT('Ctrl Pts',(178.454056855601,618.516756035746,-36.1727624672529)) ;
#59896=CARTESIAN_POINT('Ctrl Pts',(178.486072617855,618.521106305691,-36.1211950867261)) ;
#59897=CARTESIAN_POINT('Ctrl Pts',(178.520806054384,618.525403854869,-36.0714757396111)) ;
#59898=CARTESIAN_POINT('Ctrl Pts',(178.555517380224,618.529698668303,-36.0217880429491)) ;
#59899=CARTESIAN_POINT('Ctrl Pts',(178.592942827306,618.533940685251,-35.9739459312664)) ;
#59900=CARTESIAN_POINT('Ctrl Pts',(178.632846906928,618.538104505605,-35.9282434763273)) ;
#59901=CARTESIAN_POINT('Ctrl Pts',(178.672740745377,618.542267257336,-35.8825527506836)) ;
#59902=CARTESIAN_POINT('Ctrl Pts',(178.71511194355,618.546351841969,-35.8390006188666)) ;
#59903=CARTESIAN_POINT('Ctrl Pts',(178.759698879925,618.55035755848,-35.7978584663417)) ;
#59904=CARTESIAN_POINT('Ctrl Pts',(178.805815173444,618.554500673334,-35.7553051147069)) ;
#59905=CARTESIAN_POINT('Ctrl Pts',(178.854302049302,618.558559386672,-35.7153302272149)) ;
#59906=CARTESIAN_POINT('Ctrl Pts',(178.904839879814,618.562559893931,-35.6782071797221)) ;
#59907=CARTESIAN_POINT('Ctrl Pts',(178.95376501449,618.566432742339,-35.6422687534043)) ;
#59908=CARTESIAN_POINT('Ctrl Pts',(179.004612255485,618.570251419296,-35.6090032130565)) ;
#59909=CARTESIAN_POINT('Ctrl Pts',(179.057062896466,618.574061490419,-35.5786307741719)) ;
#59910=CARTESIAN_POINT('Ctrl Pts',(179.112106895572,618.578059945874,-35.5467566070012)) ;
#59911=CARTESIAN_POINT('Ctrl Pts',(179.168917188531,618.582049299349,-35.5180695816817)) ;
#59912=CARTESIAN_POINT('Ctrl Pts',(179.227089810526,618.58610139435,-35.4927849063632)) ;
#59913=CARTESIAN_POINT('Ctrl Pts',(179.277252190683,618.589595524799,-35.4709818751094)) ;
#59914=CARTESIAN_POINT('Ctrl Pts',(179.328428400699,618.593136969904,-35.451708177045)) ;
#59915=CARTESIAN_POINT('Ctrl Pts',(179.380332883121,618.596777508938,-35.435072119092)) ;
#59916=CARTESIAN_POINT('Ctrl Pts',(179.388603871233,618.597357629453,-35.4324211604245)) ;
#59917=CARTESIAN_POINT('Ctrl Pts',(179.396893413007,618.597940266208,-35.4298370893434)) ;
#59918=CARTESIAN_POINT('Ctrl Pts',(179.405200425425,618.598525628718,-35.4273202451089)) ;
#59919=CARTESIAN_POINT('Ctrl Pts',(179.405217944885,618.598526863246,-35.4273149370932)) ;
#59920=CARTESIAN_POINT('Ctrl Pts',(179.405235464423,618.598528097785,-35.4273096293765)) ;
#59921=CARTESIAN_POINT('Ctrl Pts',(179.405252984039,618.598529332337,-35.4273043219588)) ;
#59922=CARTESIAN_POINT('Ctrl Pts',(179.459051654156,618.60232035397,-35.4110064750025)) ;
#59923=CARTESIAN_POINT('Ctrl Pts',(179.51377379274,618.606235591445,-35.3974787764822)) ;
#59924=CARTESIAN_POINT('Ctrl Pts',(179.569111842561,618.610212675629,-35.3867837090165)) ;
#59925=CARTESIAN_POINT('Ctrl Pts',(179.574661034334,618.610611489879,-35.3857112284976)) ;
#59926=CARTESIAN_POINT('Ctrl Pts',(179.580216379535,618.611010926041,-35.3846672155845)) ;
#59927=CARTESIAN_POINT('Ctrl Pts',(179.585777541669,618.611410921222,-35.383651721626)) ;
#59928=CARTESIAN_POINT('Ctrl Pts',(179.646667098476,618.615790496704,-35.3725330065825)) ;
#59929=CARTESIAN_POINT('Ctrl Pts',(179.70825972965,618.620236454121,-35.3648349819728)) ;
#59930=CARTESIAN_POINT('Ctrl Pts',(179.7701513431,618.624679650117,-35.3605928285274)) ;
#59931=CARTESIAN_POINT('Ctrl Pts',(179.831966478092,618.629117355727,-35.3563559170419)) ;
#59932=CARTESIAN_POINT('Ctrl Pts',(179.894079953235,618.63355196713,-35.3555659745547)) ;
#59933=CARTESIAN_POINT('Ctrl Pts',(179.956094752594,618.637935187241,-35.3582197283047)) ;
#59934=CARTESIAN_POINT('Ctrl Pts',(180.01805245278,618.642314371569,-35.3608710386517)) ;
#59935=CARTESIAN_POINT('Ctrl Pts',(180.079911741523,618.646642123212,-35.3669595863454)) ;
#59936=CARTESIAN_POINT('Ctrl Pts',(180.141280840958,618.650894328773,-35.3764473975845)) ;
#59937=CARTESIAN_POINT('Ctrl Pts',(180.202612746982,618.655143957238,-35.3859294586323)) ;
#59938=CARTESIAN_POINT('Ctrl Pts',(180.263455073361,618.659318138432,-35.3988067183323)) ;
#59939=CARTESIAN_POINT('Ctrl Pts',(180.323420134712,618.663417764808,-35.4150070260749)) ;
#59940=CARTESIAN_POINT('Ctrl Pts',(180.383391163055,618.66751779913,-35.4312089458747)) ;
#59941=CARTESIAN_POINT('Ctrl Pts',(180.442484684221,618.67154339821,-35.4507347702405)) ;
#59942=CARTESIAN_POINT('Ctrl Pts',(180.500316653274,618.675519379174,-35.4734761721196)) ;
#59943=CARTESIAN_POINT('Ctrl Pts',(180.558146719432,618.679495229314,-35.4962168257189)) ;
#59944=CARTESIAN_POINT('Ctrl Pts',(180.61471513308,618.683421757168,-35.5221731686129)) ;
#59945=CARTESIAN_POINT('Ctrl Pts',(180.669643472711,618.687344539433,-35.5511968412561)) ;
#59946=CARTESIAN_POINT('Ctrl Pts',(180.724627059594,618.691271267257,-35.580249706082)) ;
#59947=CARTESIAN_POINT('Ctrl Pts',(180.777966886512,618.695194746064,-35.6123765119138)) ;
#59948=CARTESIAN_POINT('Ctrl Pts',(180.82929314479,618.69917558051,-35.6473825524794)) ;
#59949=CARTESIAN_POINT('Ctrl Pts',(180.877353246692,618.702903093786,-35.6801609768813)) ;
#59950=CARTESIAN_POINT('Ctrl Pts',(180.923647493842,618.706681551705,-35.7154637220932)) ;
#59951=CARTESIAN_POINT('Ctrl Pts',(180.967886278469,618.710565160535,-35.7530892919061)) ;
#59952=CARTESIAN_POINT('',(180.986589642961,618.710557544484,-38.2762782920169)) ;
#59953=CARTESIAN_POINT('Origin',(179.888527625422,618.710565160536,-37.0221601717597)) ;
#59954=CARTESIAN_POINT('',(179.889399881814,618.088273794561,-38.6876911816457)) ;
#59955=CARTESIAN_POINT('Ctrl Pts',(180.986589653577,618.710557544348,-38.2762783041407)) ;
#59956=CARTESIAN_POINT('Ctrl Pts',(181.026169046573,618.706964343704,-38.2415835129224)) ;
#59957=CARTESIAN_POINT('Ctrl Pts',(181.064134566316,618.703274822254,-38.2049117313778)) ;
#59958=CARTESIAN_POINT('Ctrl Pts',(181.100299043188,618.699542583949,-38.1664539739033)) ;
#59959=CARTESIAN_POINT('Ctrl Pts',(181.141726611101,618.695267185291,-38.1223993795229)) ;
#59960=CARTESIAN_POINT('Ctrl Pts',(181.180791568861,618.690936293108,-38.076000131448)) ;
#59961=CARTESIAN_POINT('Ctrl Pts',(181.217253524757,618.68661604972,-38.0275596099569)) ;
#59962=CARTESIAN_POINT('Ctrl Pts',(181.253678328109,618.682300208401,-37.9791684464486)) ;
#59963=CARTESIAN_POINT('Ctrl Pts',(181.287505713534,618.677995292116,-37.9287402994145)) ;
#59964=CARTESIAN_POINT('Ctrl Pts',(181.318530263923,618.67374647211,-37.8765947129868)) ;
#59965=CARTESIAN_POINT('Ctrl Pts',(181.349534972181,618.669500369488,-37.8244824769068)) ;
#59966=CARTESIAN_POINT('Ctrl Pts',(181.377740524878,618.665310409449,-37.7706550363168)) ;
#59967=CARTESIAN_POINT('Ctrl Pts',(181.402973312593,618.661197874076,-37.7154472169003)) ;
#59968=CARTESIAN_POINT('Ctrl Pts',(181.428199534615,618.657086408805,-37.660253762824)) ;
#59969=CARTESIAN_POINT('Ctrl Pts',(181.450454481109,618.653052318317,-37.6036806587458)) ;
#59970=CARTESIAN_POINT('Ctrl Pts',(181.46959583614,618.649092285549,-37.5460780256657)) ;
#59971=CARTESIAN_POINT('Ctrl Pts',(181.488753320266,618.645128915935,-37.488426854835)) ;
#59972=CARTESIAN_POINT('Ctrl Pts',(181.504791768155,618.641239604739,-37.4297444203877)) ;
#59973=CARTESIAN_POINT('Ctrl Pts',(181.517601625427,618.637397385774,-37.3703972420371)) ;
#59974=CARTESIAN_POINT('Ctrl Pts',(181.530416297433,618.633553722667,-37.3110277573567)) ;
#59975=CARTESIAN_POINT('Ctrl Pts',(181.539999611886,618.629756913792,-37.2509930458803)) ;
#59976=CARTESIAN_POINT('Ctrl Pts',(181.546279004478,618.625959256704,-37.1906754568052)) ;
#59977=CARTESIAN_POINT('Ctrl Pts',(181.552570321133,618.622154388169,-37.1302433294688)) ;
#59978=CARTESIAN_POINT('Ctrl Pts',(181.555544624921,618.618348193862,-37.0695273473087)) ;
#59979=CARTESIAN_POINT('Ctrl Pts',(181.555172712382,618.614477464704,-37.0089267621576)) ;
#59980=CARTESIAN_POINT('Ctrl Pts',(181.554838547445,618.610999598739,-36.954476888776)) ;
#59981=CARTESIAN_POINT('Ctrl Pts',(181.551802998906,618.607469043536,-36.9001197890744)) ;
#59982=CARTESIAN_POINT('Ctrl Pts',(181.546081556269,618.603835460268,-36.8461553786571)) ;
#59983=CARTESIAN_POINT('Ctrl Pts',(181.545573751228,618.603512962602,-36.8413657825042)) ;
#59984=CARTESIAN_POINT('Ctrl Pts',(181.545044806735,618.603189653342,-36.8365792511381)) ;
#59985=CARTESIAN_POINT('Ctrl Pts',(181.544494744016,618.602865497294,-36.8317959772675)) ;
#59986=CARTESIAN_POINT('Ctrl Pts',(181.544490855517,618.602863205773,-36.8317621633852)) ;
#59987=CARTESIAN_POINT('Ctrl Pts',(181.544486965962,618.602860914209,-36.8317283496656)) ;
#59988=CARTESIAN_POINT('Ctrl Pts',(181.544483075352,618.602858622603,-36.8316945361088)) ;
#59989=CARTESIAN_POINT('Ctrl Pts',(181.538135447463,618.599119809511,-36.7765268651732)) ;
#59990=CARTESIAN_POINT('Ctrl Pts',(181.528947374573,618.595258438764,-36.7215940585193)) ;
#59991=CARTESIAN_POINT('Ctrl Pts',(181.516981104278,618.591337573943,-36.6671986732568)) ;
#59992=CARTESIAN_POINT('Ctrl Pts',(181.51586624176,618.590972278398,-36.66213081379)) ;
#59993=CARTESIAN_POINT('Ctrl Pts',(181.514727290899,618.590606466438,-36.6570676453316)) ;
#59994=CARTESIAN_POINT('Ctrl Pts',(181.513564318844,618.590240189063,-36.6520094282069)) ;
#59995=CARTESIAN_POINT('Ctrl Pts',(181.499781160261,618.585899191248,-36.5920611186054)) ;
#59996=CARTESIAN_POINT('Ctrl Pts',(181.482619962743,618.581493479981,-36.5328037999466)) ;
#59997=CARTESIAN_POINT('Ctrl Pts',(181.462208479127,618.577093884059,-36.4746228510559)) ;
#59998=CARTESIAN_POINT('Ctrl Pts',(181.44205587073,618.57275008743,-36.4171798007995)) ;
#59999=CARTESIAN_POINT('Ctrl Pts',(181.418735267596,618.56841254422,-36.3607857591996)) ;
#60000=CARTESIAN_POINT('Ctrl Pts',(181.392402973023,618.56412887647,-36.3057912769584)) ;
#60001=CARTESIAN_POINT('Ctrl Pts',(181.366086649505,618.559847806849,-36.2508301499537)) ;
#60002=CARTESIAN_POINT('Ctrl Pts',(181.336762385989,618.555620682448,-36.1972668002697)) ;
#60003=CARTESIAN_POINT('Ctrl Pts',(181.304616451639,618.551471225851,-36.1454330180176)) ;
#60004=CARTESIAN_POINT('Ctrl Pts',(181.272478151229,618.547322754656,-36.0936115451292)) ;
#60005=CARTESIAN_POINT('Ctrl Pts',(181.237519502145,618.543251916378,-36.0435188495208)) ;
#60006=CARTESIAN_POINT('Ctrl Pts',(181.199956330705,618.539257613532,-35.9954687581075)) ;
#60007=CARTESIAN_POINT('Ctrl Pts',(181.161502667911,618.535168619743,-35.9462795671642)) ;
#60008=CARTESIAN_POINT('Ctrl Pts',(181.120319291636,618.531159806111,-35.8992312085298)) ;
#60009=CARTESIAN_POINT('Ctrl Pts',(181.076670980546,618.527204007082,-35.8546396928581)) ;
#60010=CARTESIAN_POINT('Ctrl Pts',(181.033979319065,618.523334908169,-35.8110254992176)) ;
#60011=CARTESIAN_POINT('Ctrl Pts',(180.988929530562,618.519516171893,-35.76976183486)) ;
#60012=CARTESIAN_POINT('Ctrl Pts',(180.941802622243,618.51570093191,-35.7311218745408)) ;
#60013=CARTESIAN_POINT('Ctrl Pts',(180.893091659676,618.511757452089,-35.6911831277021)) ;
#60014=CARTESIAN_POINT('Ctrl Pts',(180.842161143015,618.507817277096,-35.6540481292493)) ;
#60015=CARTESIAN_POINT('Ctrl Pts',(180.789361683744,618.503811044041,-35.6199872221115)) ;
#60016=CARTESIAN_POINT('Ctrl Pts',(180.743416088697,618.50032485755,-35.590347739664)) ;
#60017=CARTESIAN_POINT('Ctrl Pts',(180.69605459303,618.49678800037,-35.5630354622988)) ;
#60018=CARTESIAN_POINT('Ctrl Pts',(180.647538816787,618.493149850119,-35.5382040513801)) ;
#60019=CARTESIAN_POINT('Ctrl Pts',(180.6403294513,618.492609226905,-35.5345141440816)) ;
#60020=CARTESIAN_POINT('Ctrl Pts',(180.633094559179,618.492066366991,-35.5308789322976)) ;
#60021=CARTESIAN_POINT('Ctrl Pts',(180.625834956093,618.49152110427,-35.5272988314416)) ;
#60022=CARTESIAN_POINT('Ctrl Pts',(180.625806860057,618.491518994001,-35.527284975775)) ;
#60023=CARTESIAN_POINT('Ctrl Pts',(180.625778763652,618.491516883695,-35.5272711209338)) ;
#60024=CARTESIAN_POINT('Ctrl Pts',(180.625750666876,618.491514773353,-35.5272572669181)) ;
#60025=CARTESIAN_POINT('Ctrl Pts',(180.576030268583,618.487780286783,-35.5027410308854)) ;
#60026=CARTESIAN_POINT('Ctrl Pts',(180.524969197056,618.483923273951,-35.480729384318)) ;
#60027=CARTESIAN_POINT('Ctrl Pts',(180.472854387436,618.48000695136,-35.4613343960481)) ;
#60028=CARTESIAN_POINT('Ctrl Pts',(180.468022513008,618.479643845765,-35.4595361711569)) ;
#60029=CARTESIAN_POINT('Ctrl Pts',(180.463181616492,618.479280230328,-35.4577604315961)) ;
#60030=CARTESIAN_POINT('Ctrl Pts',(180.45833194852,618.478916155434,-35.4560072611747)) ;
#60031=CARTESIAN_POINT('Ctrl Pts',(180.400464932603,618.474571955415,-35.4350881505736)) ;
#60032=CARTESIAN_POINT('Ctrl Pts',(180.341343124075,618.470163005833,-35.4173832741389)) ;
#60033=CARTESIAN_POINT('Ctrl Pts',(180.281360663462,618.465760686335,-35.4029953114805)) ;
#60034=CARTESIAN_POINT('Ctrl Pts',(180.222280077188,618.461424558502,-35.3888236809662)) ;
#60035=CARTESIAN_POINT('Ctrl Pts',(180.162364534116,618.457095145439,-35.3778695236006)) ;
#60036=CARTESIAN_POINT('Ctrl Pts',(180.10199182776,618.452820103473,-35.3701919206502)) ;
#60037=CARTESIAN_POINT('Ctrl Pts',(180.041656666309,618.448547720093,-35.362519092289)) ;
#60038=CARTESIAN_POINT('Ctrl Pts',(179.980864896819,618.444329774189,-35.3581186178058)) ;
#60039=CARTESIAN_POINT('Ctrl Pts',(179.91999490829,618.440190063795,-35.3570142327182)) ;
#60040=CARTESIAN_POINT('Ctrl Pts',(179.859140066554,618.436051383519,-35.355910122444)) ;
#60041=CARTESIAN_POINT('Ctrl Pts',(179.798207065939,618.431990901943,-35.3581004936399)) ;
#60042=CARTESIAN_POINT('Ctrl Pts',(179.737575273906,618.42800764707,-35.3635744907322)) ;
#60043=CARTESIAN_POINT('Ctrl Pts',(179.675246879113,618.4239129325,-35.3692016615684)) ;
#60044=CARTESIAN_POINT('Ctrl Pts',(179.613236858033,618.419899818461,-35.3782991522623)) ;
#60045=CARTESIAN_POINT('Ctrl Pts',(179.551957974696,618.415940925301,-35.3908154544142)) ;
#60046=CARTESIAN_POINT('Ctrl Pts',(179.492271481222,618.412084907731,-35.4030065085917)) ;
#60047=CARTESIAN_POINT('Ctrl Pts',(179.433278761062,618.40827996142,-35.4184411264926)) ;
#60048=CARTESIAN_POINT('Ctrl Pts',(179.375360275416,618.40447931491,-35.4370315093212)) ;
#60049=CARTESIAN_POINT('Ctrl Pts',(179.315123958615,618.400526570899,-35.4563658578809)) ;
#60050=CARTESIAN_POINT('Ctrl Pts',(179.256049933563,618.396578059386,-35.4791144283665)) ;
#60051=CARTESIAN_POINT('Ctrl Pts',(179.198561508483,618.392563166561,-35.5051265924183)) ;
#60052=CARTESIAN_POINT('Ctrl Pts',(179.148831933066,618.389090138464,-35.5276280589684)) ;
#60053=CARTESIAN_POINT('Ctrl Pts',(179.10028791631,618.385566779611,-35.5525718741155)) ;
#60054=CARTESIAN_POINT('Ctrl Pts',(179.053199503989,618.381942418963,-35.5798214164548)) ;
#60055=CARTESIAN_POINT('Ctrl Pts',(179.04587875353,618.381378946156,-35.5840578536113)) ;
#60056=CARTESIAN_POINT('Ctrl Pts',(179.038593084181,618.380813032099,-35.5883500054825)) ;
#60057=CARTESIAN_POINT('Ctrl Pts',(179.031343398033,618.380244486385,-35.5926973446195)) ;
#60058=CARTESIAN_POINT('Ctrl Pts',(179.031317627898,618.380242465401,-35.5927127979116)) ;
#60059=CARTESIAN_POINT('Ctrl Pts',(179.031291858218,618.380240444383,-35.592728251901)) ;
#60060=CARTESIAN_POINT('Ctrl Pts',(179.031266088992,618.380238423333,-35.5927437065876)) ;
#60061=CARTESIAN_POINT('Ctrl Pts',(178.983727870414,618.376510055907,-35.6212540030795)) ;
#60062=CARTESIAN_POINT('Ctrl Pts',(178.937569640057,618.372658630446,-35.6522473603323)) ;
#60063=CARTESIAN_POINT('Ctrl Pts',(178.893040739353,618.36874728734,-35.6855431319309)) ;
#60064=CARTESIAN_POINT('Ctrl Pts',(178.888877711047,618.368381613995,-35.6886559696035)) ;
#60065=CARTESIAN_POINT('Ctrl Pts',(178.884728936709,618.368015416941,-35.6917888961039)) ;
#60066=CARTESIAN_POINT('Ctrl Pts',(178.880594627477,618.367648747775,-35.6949417418113)) ;
#60067=CARTESIAN_POINT('Ctrl Pts',(178.831666573002,618.363309350806,-35.732254530445)) ;
#60068=CARTESIAN_POINT('Ctrl Pts',(178.784762041634,618.358904497748,-35.7723626795533)) ;
#60069=CARTESIAN_POINT('Ctrl Pts',(178.740180467144,618.354505584414,-35.8149902629322)) ;
#60070=CARTESIAN_POINT('Ctrl Pts',(178.696241885767,618.350170115922,-35.8570030353077)) ;
#60071=CARTESIAN_POINT('Ctrl Pts',(178.654559366142,618.345840703961,-35.9014628428434)) ;
#60072=CARTESIAN_POINT('Ctrl Pts',(178.615387274715,618.341565164946,-35.9480834766588)) ;
#60073=CARTESIAN_POINT('Ctrl Pts',(178.57623923858,618.337292251509,-35.9946754810876)) ;
#60074=CARTESIAN_POINT('Ctrl Pts',(178.539598431727,618.333073280143,-36.04342560137)) ;
#60075=CARTESIAN_POINT('Ctrl Pts',(178.50568976433,618.328932193516,-36.0940280527371)) ;
#60076=CARTESIAN_POINT('Ctrl Pts',(178.471789310876,618.324792110015,-36.1446182463039)) ;
#60077=CARTESIAN_POINT('Ctrl Pts',(178.440619709841,618.320729876237,-36.1970598741901)) ;
#60078=CARTESIAN_POINT('Ctrl Pts',(178.412377294774,618.31674463504,-36.2510276540207)) ;
#60079=CARTESIAN_POINT('Ctrl Pts',(178.383376399135,618.312652365886,-36.3064447968897)) ;
#60080=CARTESIAN_POINT('Ctrl Pts',(178.357462357362,618.308641267557,-36.363471294895)) ;
#60081=CARTESIAN_POINT('Ctrl Pts',(178.334814837055,618.304684149029,-36.4217330290475)) ;
#60082=CARTESIAN_POINT('Ctrl Pts',(178.312731460251,618.300825601236,-36.4785434794226)) ;
#60083=CARTESIAN_POINT('Ctrl Pts',(178.293754082553,618.297018013748,-36.5365283491731)) ;
#60084=CARTESIAN_POINT('Ctrl Pts',(178.278014995893,618.293214675688,-36.5953198544874)) ;
#60085=CARTESIAN_POINT('Ctrl Pts',(178.261672801505,618.289265597114,-36.6563641977219)) ;
#60086=CARTESIAN_POINT('Ctrl Pts',(178.248822697785,618.28532067976,-36.7182783197643)) ;
#60087=CARTESIAN_POINT('Ctrl Pts',(178.239566934482,618.281309682721,-36.7806265090767)) ;
#60088=CARTESIAN_POINT('Ctrl Pts',(178.231544843613,618.277833299233,-36.8346644985706)) ;
#60089=CARTESIAN_POINT('Ctrl Pts',(178.226222505982,618.274306621661,-36.8890294525564)) ;
#60090=CARTESIAN_POINT('Ctrl Pts',(178.22363147269,618.270678912868,-36.9434198669935)) ;
#60091=CARTESIAN_POINT('Ctrl Pts',(178.223234423111,618.27012300328,-36.9517546464896)) ;
#60092=CARTESIAN_POINT('Ctrl Pts',(178.222901445326,618.269564721232,-36.9600900986547)) ;
#60093=CARTESIAN_POINT('Ctrl Pts',(178.2226325834,618.269003884147,-36.9684252219111)) ;
#60094=CARTESIAN_POINT('Ctrl Pts',(178.222631627995,618.269001891203,-36.9684548409136)) ;
#60095=CARTESIAN_POINT('Ctrl Pts',(178.222630673399,618.268999898226,-36.9684844599119)) ;
#60096=CARTESIAN_POINT('Ctrl Pts',(178.222629719612,618.268997905217,-36.9685140789061)) ;
#60097=CARTESIAN_POINT('Ctrl Pts',(178.220844750902,618.265268077855,-37.0239447132894)) ;
#60098=CARTESIAN_POINT('Ctrl Pts',(178.221897153798,618.261415407973,-37.0795599854219)) ;
#60099=CARTESIAN_POINT('Ctrl Pts',(178.225770009133,618.25750304258,-37.1350521154175)) ;
#60100=CARTESIAN_POINT('Ctrl Pts',(178.226130966848,618.257138402451,-37.1402240907859)) ;
#60101=CARTESIAN_POINT('Ctrl Pts',(178.22651640212,618.25677324377,-37.1453949666777)) ;
#60102=CARTESIAN_POINT('Ctrl Pts',(178.226926286903,618.256407617662,-37.150564475947)) ;
#60103=CARTESIAN_POINT('Ctrl Pts',(178.231789640912,618.252069400506,-37.2119015997002)) ;
#60104=CARTESIAN_POINT('Ctrl Pts',(178.240098348827,618.247666043529,-37.2730513545185)) ;
#60105=CARTESIAN_POINT('Ctrl Pts',(178.251782591525,618.243268807749,-37.333612770775)) ;
#60106=CARTESIAN_POINT('Ctrl Pts',(178.263301349628,618.238933850269,-37.393316452245)) ;
#60107=CARTESIAN_POINT('Ctrl Pts',(178.278100296117,618.234605129,-37.4524485192166)) ;
#60108=CARTESIAN_POINT('Ctrl Pts',(178.296076521841,618.230330372981,-37.5106400083246)) ;
#60109=CARTESIAN_POINT('Ctrl Pts',(178.314041786601,618.226058223484,-37.5687960153033)) ;
#60110=CARTESIAN_POINT('Ctrl Pts',(178.335180346023,618.22184010836,-37.6260126581506)) ;
#60111=CARTESIAN_POINT('Ctrl Pts',(178.359356884229,618.217699875044,-37.6819351315033)) ;
#60112=CARTESIAN_POINT('Ctrl Pts',(178.38352766094,618.213560628384,-37.7378442780082)) ;
#60113=CARTESIAN_POINT('Ctrl Pts',(178.410734989242,618.209499228755,-37.792459841562)) ;
#60114=CARTESIAN_POINT('Ctrl Pts',(178.44081168331,618.205514720716,-37.8454404763845)) ;
#60115=CARTESIAN_POINT('Ctrl Pts',(178.471681683884,618.201425116813,-37.8998185348105)) ;
#60116=CARTESIAN_POINT('Ctrl Pts',(178.50557469763,618.197416498929,-37.9524740743393)) ;
#60117=CARTESIAN_POINT('Ctrl Pts',(178.542273756713,618.193461617409,-38.0030537894537)) ;
#60118=CARTESIAN_POINT('Ctrl Pts',(178.578075628569,618.189603421452,-38.0523969749278)) ;
#60119=CARTESIAN_POINT('Ctrl Pts',(178.616548090732,618.18579600404,-38.0997644085252)) ;
#60120=CARTESIAN_POINT('Ctrl Pts',(178.657453529299,618.181992580754,-38.1448455442407)) ;
#60121=CARTESIAN_POINT('Ctrl Pts',(178.699896590135,618.178046188011,-38.1916212653381)) ;
#60122=CARTESIAN_POINT('Ctrl Pts',(178.744959556691,618.174103672878,-38.2359349255075)) ;
#60123=CARTESIAN_POINT('Ctrl Pts',(178.792332068751,618.170094893156,-38.2774650993131)) ;
#60124=CARTESIAN_POINT('Ctrl Pts',(178.833407260991,618.166619008289,-38.313474586644)) ;
#60125=CARTESIAN_POINT('Ctrl Pts',(178.876219382718,618.163092650363,-38.3473921510311)) ;
#60126=CARTESIAN_POINT('Ctrl Pts',(178.920532199528,618.159465125344,-38.3790280332569)) ;
#60127=CARTESIAN_POINT('Ctrl Pts',(178.927301502472,618.158910978315,-38.3838607856317)) ;
#60128=CARTESIAN_POINT('Ctrl Pts',(178.934105852788,618.158354470436,-38.3886403877065)) ;
#60129=CARTESIAN_POINT('Ctrl Pts',(178.940944440391,618.157795420989,-38.3933662655828)) ;
#60130=CARTESIAN_POINT('Ctrl Pts',(178.940969073529,618.157793407248,-38.3933832885721)) ;
#60131=CARTESIAN_POINT('Ctrl Pts',(178.940993707112,618.157791393474,-38.3934003108644)) ;
#60132=CARTESIAN_POINT('Ctrl Pts',(178.941018341139,618.157789379668,-38.3934173324596)) ;
#60133=CARTESIAN_POINT('Ctrl Pts',(178.986947887101,618.154034685892,-38.4251536842743)) ;
#60134=CARTESIAN_POINT('Ctrl Pts',(179.034587519952,618.150155694842,-38.4545716490728)) ;
#60135=CARTESIAN_POINT('Ctrl Pts',(179.083667732432,618.146216600731,-38.4815191143161)) ;
#60136=CARTESIAN_POINT('Ctrl Pts',(179.088574774354,618.145822769918,-38.4842133231419)) ;
#60137=CARTESIAN_POINT('Ctrl Pts',(179.093496173381,618.145428338316,-38.486882838659)) ;
#60138=CARTESIAN_POINT('Ctrl Pts',(179.098431631662,618.145033370078,-38.4895275108052)) ;
#60139=CARTESIAN_POINT('Ctrl Pts',(179.152640696328,618.140695199735,-38.5185755130836)) ;
#60140=CARTESIAN_POINT('Ctrl Pts',(179.208551896439,618.136292922672,-38.5446267206134)) ;
#60141=CARTESIAN_POINT('Ctrl Pts',(179.265796825254,618.131897185162,-38.5675249941924)) ;
#60142=CARTESIAN_POINT('Ctrl Pts',(179.322953854601,618.127508197298,-38.5903881075203)) ;
#60143=CARTESIAN_POINT('Ctrl Pts',(179.381440509849,618.123126065173,-38.6101083388411)) ;
#60144=CARTESIAN_POINT('Ctrl Pts',(179.440883614391,618.118799627606,-38.6265677000373)) ;
#60145=CARTESIAN_POINT('Ctrl Pts',(179.500273299633,618.114477078047,-38.6430122698199)) ;
#60146=CARTESIAN_POINT('Ctrl Pts',(179.560617760819,618.110210263012,-38.6562019649169)) ;
#60147=CARTESIAN_POINT('Ctrl Pts',(179.621538003104,618.106022940803,-38.6660527208549)) ;
#60148=CARTESIAN_POINT('Ctrl Pts',(179.682426749525,618.101837783448,-38.6758983839358)) ;
#60149=CARTESIAN_POINT('Ctrl Pts',(179.743890716494,618.097732042013,-38.682408515153)) ;
#60150=CARTESIAN_POINT('Ctrl Pts',(179.805544051061,618.093703449542,-38.6855321198862)) ;
#60151=CARTESIAN_POINT('Ctrl Pts',(179.833469375583,618.091878734741,-38.6869469286142)) ;
#60152=CARTESIAN_POINT('Ctrl Pts',(179.861433445486,618.090069493796,-38.6876674245861)) ;
#60153=CARTESIAN_POINT('Ctrl Pts',(179.889399881814,618.088273794561,-38.6876911816457)) ;
#60154=CARTESIAN_POINT('Ctrl Pts',(179.889382603702,618.088003960412,-38.6881599523756)) ;
#60155=CARTESIAN_POINT('Ctrl Pts',(179.962423314324,618.083373402089,-38.6881224684444)) ;
#60156=CARTESIAN_POINT('Ctrl Pts',(180.035386280762,618.078875076633,-38.6832817710899)) ;
#60157=CARTESIAN_POINT('Ctrl Pts',(180.211867029433,618.067988436433,-38.6598500499037)) ;
#60158=CARTESIAN_POINT('Ctrl Pts',(180.314382464896,618.061663276376,-38.6362294483913)) ;
#60159=CARTESIAN_POINT('Ctrl Pts',(180.430769124812,618.053833524208,-38.5975468162584)) ;
#60160=CARTESIAN_POINT('Ctrl Pts',(180.447464000146,618.052693836644,-38.5917011579464)) ;
#60161=CARTESIAN_POINT('Ctrl Pts',(180.464060715285,618.051541226924,-38.5855915461645)) ;
#60162=CARTESIAN_POINT('Origin',(179.888527625422,617.710565160536,-37.0221601717597)) ;
#60163=CARTESIAN_POINT('Ctrl Pts',(180.464060715285,618.051541226924,-38.5855915461645)) ;
#60164=CARTESIAN_POINT('Ctrl Pts',(180.481897953674,618.050302465268,-38.5790252707955)) ;
#60165=CARTESIAN_POINT('Ctrl Pts',(180.499621809325,618.04904877561,-38.5721541087867)) ;
#60166=CARTESIAN_POINT('Ctrl Pts',(180.54651059363,618.045661037341,-38.5530470101377)) ;
#60167=CARTESIAN_POINT('Ctrl Pts',(180.575446202966,618.043493376976,-38.5402834717153)) ;
#60168=CARTESIAN_POINT('Ctrl Pts',(180.708426674847,618.033221401202,-38.4770461607259)) ;
#60169=CARTESIAN_POINT('Ctrl Pts',(180.807395110013,618.024703257508,-38.4166519385844)) ;
#60170=CARTESIAN_POINT('Ctrl Pts',(180.953122418519,618.0114092671,-38.3054283094891)) ;
#60171=CARTESIAN_POINT('Ctrl Pts',(181.004389048798,618.006551978326,-38.2611089786966)) ;
#60172=CARTESIAN_POINT('Ctrl Pts',(181.093844965957,617.997784965623,-38.1737051200831)) ;
#60173=CARTESIAN_POINT('Ctrl Pts',(181.13277581992,617.99384898638,-38.1315264288429)) ;
#60174=CARTESIAN_POINT('Ctrl Pts',(181.202199529866,617.986574524375,-38.0480472311912)) ;
#60175=CARTESIAN_POINT('Ctrl Pts',(181.23311165478,617.983220872074,-38.007184469839)) ;
#60176=CARTESIAN_POINT('Ctrl Pts',(181.341487075236,617.970925665975,-37.8492917778832)) ;
#60177=CARTESIAN_POINT('Ctrl Pts',(181.405950168592,617.962514325683,-37.7240642386614)) ;
#60178=CARTESIAN_POINT('Ctrl Pts',(181.471436080325,617.950761540825,-37.5442384131307)) ;
#60179=CARTESIAN_POINT('Ctrl Pts',(181.486696060997,617.947597142538,-37.4954695604202)) ;
#60180=CARTESIAN_POINT('Ctrl Pts',(181.509415473696,617.941915047848,-37.4091215745386)) ;
#60181=CARTESIAN_POINT('Ctrl Pts',(181.517864380543,617.939436579263,-37.3718424456813)) ;
#60182=CARTESIAN_POINT('Ctrl Pts',(181.530825902746,617.934818756473,-37.3038895239917)) ;
#60183=CARTESIAN_POINT('Ctrl Pts',(181.535777960001,617.932701947745,-37.2733190358721)) ;
#60184=CARTESIAN_POINT('Ctrl Pts',(181.55606650409,617.922033117617,-37.1213570598269)) ;
#60185=CARTESIAN_POINT('Ctrl Pts',(181.558848367516,617.913001116171,-36.9986751456239)) ;
#60186=CARTESIAN_POINT('Ctrl Pts',(181.542437192452,617.899377626793,-36.8112979469856)) ;
#60187=CARTESIAN_POINT('Ctrl Pts',(181.532826603064,617.89466940303,-36.7461851866537)) ;
#60188=CARTESIAN_POINT('Ctrl Pts',(181.507846104336,617.886112625852,-36.6264873322731)) ;
#60189=CARTESIAN_POINT('Ctrl Pts',(181.493493454421,617.882241218155,-36.5717876978933)) ;
#60190=CARTESIAN_POINT('Ctrl Pts',(181.460787725981,617.875011179151,-36.4687975027266)) ;
#60191=CARTESIAN_POINT('Ctrl Pts',(181.442917151037,617.871641128152,-36.4204241573451)) ;
#60192=CARTESIAN_POINT('Ctrl Pts',(181.370334565773,617.859700978261,-36.2488863271084)) ;
#60193=CARTESIAN_POINT('Ctrl Pts',(181.302986370131,617.851604417519,-36.1316471018976)) ;
#60194=CARTESIAN_POINT('Ctrl Pts',(181.190495127365,617.840091392759,-35.9813697762763)) ;
#60195=CARTESIAN_POINT('Ctrl Pts',(181.156736065954,617.836815544789,-35.9404898957237)) ;
#60196=CARTESIAN_POINT('Ctrl Pts',(181.094803513211,617.830967522098,-35.8723858724377)) ;
#60197=CARTESIAN_POINT('Ctrl Pts',(181.067511624564,617.828438114352,-35.8444171751952)) ;
#60198=CARTESIAN_POINT('Ctrl Pts',(181.017087578928,617.823789225325,-35.7962527466986)) ;
#60199=CARTESIAN_POINT('Ctrl Pts',(180.994333773178,617.821696055835,-35.7756896605593)) ;
#60200=CARTESIAN_POINT('Ctrl Pts',(180.8859585382,617.811787212068,-35.6830513970048)) ;
#60201=CARTESIAN_POINT('Ctrl Pts',(180.793784812806,617.803562281883,-35.6190969098238)) ;
#60202=CARTESIAN_POINT('Ctrl Pts',(180.633804794777,617.790276838319,-35.5304637832991)) ;
#60203=CARTESIAN_POINT('Ctrl Pts',(180.569563479209,617.785166760879,-35.5000602517913)) ;
#60204=CARTESIAN_POINT('Ctrl Pts',(180.448972575006,617.776046706314,-35.4521573034835)) ;
#60205=CARTESIAN_POINT('Ctrl Pts',(180.393258611658,617.772004446071,-35.4333695375535)) ;
#60206=CARTESIAN_POINT('Ctrl Pts',(180.288341428885,617.76469073467,-35.4040681191089)) ;
#60207=CARTESIAN_POINT('Ctrl Pts',(180.239432459861,617.761396353379,-35.3927616118759)) ;
#60208=CARTESIAN_POINT('Ctrl Pts',(180.097263404458,617.752089697059,-35.3665960179337)) ;
#60209=CARTESIAN_POINT('Ctrl Pts',(180.003155295399,617.746266518971,-35.3574299056535)) ;
#60210=CARTESIAN_POINT('Ctrl Pts',(179.803917019628,617.734083293749,-35.355009218212)) ;
#60211=CARTESIAN_POINT('Ctrl Pts',(179.699191733516,617.727761225642,-35.3636371751317)) ;
#60212=CARTESIAN_POINT('Ctrl Pts',(179.560424461082,617.718749503903,-35.388388748647)) ;
#60213=CARTESIAN_POINT('Ctrl Pts',(179.525083564929,617.716396234846,-35.3958857032905)) ;
#60214=CARTESIAN_POINT('Ctrl Pts',(179.458974965252,617.711835810747,-35.4121717697229)) ;
#60215=CARTESIAN_POINT('Ctrl Pts',(179.428163433488,617.709641588438,-35.4207100937302)) ;
#60216=CARTESIAN_POINT('Ctrl Pts',(179.36111135906,617.704741214122,-35.441385751569)) ;
#60217=CARTESIAN_POINT('Ctrl Pts',(179.325002435639,617.702020470419,-35.4538953285266)) ;
#60218=CARTESIAN_POINT('Ctrl Pts',(179.205029954759,617.692769006359,-35.5001369653809)) ;
#60219=CARTESIAN_POINT('Ctrl Pts',(179.12348652897,617.686133575331,-35.5394477233273)) ;
#60220=CARTESIAN_POINT('Ctrl Pts',(178.973590584431,617.673587492226,-35.6273830842508)) ;
#60221=CARTESIAN_POINT('Ctrl Pts',(178.904910537178,617.66767715157,-35.6749355785667)) ;
#60222=CARTESIAN_POINT('Ctrl Pts',(178.800941350191,617.658506359587,-35.7591290789971)) ;
#60223=CARTESIAN_POINT('Ctrl Pts',(178.763263218048,617.655126930392,-35.7925779590251)) ;
#60224=CARTESIAN_POINT('Ctrl Pts',(178.68373363466,617.647836855873,-35.8699036244448)) ;
#60225=CARTESIAN_POINT('Ctrl Pts',(178.64264363275,617.643963540511,-35.9144606854707)) ;
#60226=CARTESIAN_POINT('Ctrl Pts',(178.495167109237,617.629437107523,-36.0929978521746)) ;
#60227=CARTESIAN_POINT('Ctrl Pts',(178.407232128629,617.619482714398,-36.2407877980694)) ;
#60228=CARTESIAN_POINT('Ctrl Pts',(178.330962865376,617.606334115431,-36.4300103031779)) ;
#60229=CARTESIAN_POINT('Ctrl Pts',(178.319517726683,617.604162615672,-36.4610389239493)) ;
#60230=CARTESIAN_POINT('Ctrl Pts',(178.298025315358,617.599607077456,-36.5251185099032)) ;
#60231=CARTESIAN_POINT('Ctrl Pts',(178.288067709336,617.59722021884,-36.5581821585891)) ;
#60232=CARTESIAN_POINT('Ctrl Pts',(178.252184011448,617.587459129075,-36.6922886260786)) ;
#60233=CARTESIAN_POINT('Ctrl Pts',(178.234746540399,617.579793336494,-36.7953527166721)) ;
#60234=CARTESIAN_POINT('Ctrl Pts',(178.219806339448,617.565078570355,-36.9974984904036)) ;
#60235=CARTESIAN_POINT('Ctrl Pts',(178.221260917136,617.558048176043,-37.096096092647)) ;
#60236=CARTESIAN_POINT('Ctrl Pts',(178.236591290263,617.547836417959,-37.243930067945)) ;
#60237=CARTESIAN_POINT('Ctrl Pts',(178.244022889307,617.54445897066,-37.2936019992806)) ;
#60238=CARTESIAN_POINT('Ctrl Pts',(178.264971093302,617.537288777169,-37.4003877287565)) ;
#60239=CARTESIAN_POINT('Ctrl Pts',(178.279283479626,617.533526962457,-37.4572767621196)) ;
#60240=CARTESIAN_POINT('Ctrl Pts',(178.317408361774,617.525387688406,-37.5808535502216)) ;
#60241=CARTESIAN_POINT('Ctrl Pts',(178.342529754871,617.521052477997,-37.6470166490607)) ;
#60242=CARTESIAN_POINT('Ctrl Pts',(178.418383129549,617.509851591488,-37.8139436064132)) ;
#60243=CARTESIAN_POINT('Ctrl Pts',(178.475261176036,617.503047173335,-37.9114950001219)) ;
#60244=CARTESIAN_POINT('Ctrl Pts',(178.559547380461,617.493728927175,-38.0272993081169)) ;
#60245=CARTESIAN_POINT('Ctrl Pts',(178.578237443446,617.49169889003,-38.0515447945929)) ;
#60246=CARTESIAN_POINT('Ctrl Pts',(178.622388799909,617.486954332514,-38.1056673925264)) ;
#60247=CARTESIAN_POINT('Ctrl Pts',(178.648253970182,617.484216302292,-38.135181308198)) ;
#60248=CARTESIAN_POINT('Ctrl Pts',(178.711701551785,617.477648053624,-38.2026195335171)) ;
#60249=CARTESIAN_POINT('Ctrl Pts',(178.750113677462,617.47378401114,-38.2397056173296)) ;
#60250=CARTESIAN_POINT('Ctrl Pts',(178.89083544996,617.460172189489,-38.3630797396613)) ;
#60251=CARTESIAN_POINT('Ctrl Pts',(179.001713128486,617.45043168011,-38.438856263214)) ;
#60252=CARTESIAN_POINT('Ctrl Pts',(179.166289939739,617.437632975247,-38.524356562795)) ;
#60253=CARTESIAN_POINT('Ctrl Pts',(179.213188107954,617.434144599432,-38.5460167409303)) ;
#60254=CARTESIAN_POINT('Ctrl Pts',(179.313255941849,617.427001611517,-38.5867041908084)) ;
#60255=CARTESIAN_POINT('Ctrl Pts',(179.366538847938,617.423366244538,-38.6052787333947)) ;
#60256=CARTESIAN_POINT('Ctrl Pts',(179.483502705193,617.415661988358,-38.6395028159113)) ;
#60257=CARTESIAN_POINT('Ctrl Pts',(179.547371262191,617.411625001174,-38.6541698911928)) ;
#60258=CARTESIAN_POINT('Ctrl Pts',(179.733491680605,617.400071792041,-38.6855041671382)) ;
#60259=CARTESIAN_POINT('Ctrl Pts',(179.856919981988,617.392680955341,-38.6924120822337)) ;
#60260=CARTESIAN_POINT('Ctrl Pts',(180.010811444156,617.38266695113,-38.6839535939988)) ;
#60261=CARTESIAN_POINT('Ctrl Pts',(180.041608285039,617.380620620016,-38.6814000296106)) ;
#60262=CARTESIAN_POINT('Ctrl Pts',(180.110659331588,617.375906596588,-38.6737357262902)) ;
#60263=CARTESIAN_POINT('Ctrl Pts',(180.148839272739,617.373218078077,-38.6681497055414)) ;
#60264=CARTESIAN_POINT('Ctrl Pts',(180.281221338282,617.363685573126,-38.6440605424444)) ;
#60265=CARTESIAN_POINT('Ctrl Pts',(180.373989177562,617.356640793906,-38.6187486185409)) ;
#60266=CARTESIAN_POINT('Ctrl Pts',(180.464057359858,617.349676493477,-38.5855927813658)) ;
#60267=CARTESIAN_POINT('Ctrl Pts',(180.464060715702,618.242141445689,-38.5855915460107)) ;
#60268=CARTESIAN_POINT('Ctrl Pts',(180.490194428087,618.240442558113,-38.5759711581275)) ;
#60269=CARTESIAN_POINT('Ctrl Pts',(180.51609650473,618.238746139063,-38.5656919854818)) ;
#60270=CARTESIAN_POINT('Ctrl Pts',(180.604553925177,618.232876486745,-38.5279903063056)) ;
#60271=CARTESIAN_POINT('Ctrl Pts',(180.665657202885,618.228684944444,-38.4973844480904)) ;
#60272=CARTESIAN_POINT('Ctrl Pts',(180.774581177908,618.220751282732,-38.4341765186819)) ;
#60273=CARTESIAN_POINT('Ctrl Pts',(180.822913785187,618.217046656664,-38.4026681695486)) ;
#60274=CARTESIAN_POINT('Ctrl Pts',(180.910828907134,618.209872686146,-38.338621019691)) ;
#60275=CARTESIAN_POINT('Ctrl Pts',(180.950733997755,618.206428499142,-38.3066389331058)) ;
#60276=CARTESIAN_POINT('Ctrl Pts',(181.095794146144,618.19312813507,-38.1789924057104)) ;
#60277=CARTESIAN_POINT('Ctrl Pts',(181.190016720997,618.182763120211,-38.071857226188)) ;
#60278=CARTESIAN_POINT('Ctrl Pts',(181.29771299437,618.168776489805,-37.912272000729)) ;
#60279=CARTESIAN_POINT('Ctrl Pts',(181.324027984768,618.165131180131,-37.8691795562848)) ;
#60280=CARTESIAN_POINT('Ctrl Pts',(181.366644813164,618.158872424577,-37.7916843154949)) ;
#60281=CARTESIAN_POINT('Ctrl Pts',(181.38380119825,618.156228951123,-37.7577927976852)) ;
#60282=CARTESIAN_POINT('Ctrl Pts',(181.412962731757,618.151533023018,-37.6949408348441)) ;
#60283=CARTESIAN_POINT('Ctrl Pts',(181.425336677519,618.149462748053,-37.6661743641821)) ;
#60284=CARTESIAN_POINT('Ctrl Pts',(181.481202190975,618.139644580347,-37.5255040248104)) ;
#60285=CARTESIAN_POINT('Ctrl Pts',(181.513328644025,618.132436677686,-37.409454884974)) ;
#60286=CARTESIAN_POINT('Ctrl Pts',(181.543457971187,618.121017193802,-37.225152904422)) ;
#60287=CARTESIAN_POINT('Ctrl Pts',(181.550254256156,618.116913500324,-37.1587768240989)) ;
#60288=CARTESIAN_POINT('Ctrl Pts',(181.555453049174,618.109102948324,-37.035182985312)) ;
#60289=CARTESIAN_POINT('Ctrl Pts',(181.554921452956,618.105430084247,-36.9781105238886)) ;
#60290=CARTESIAN_POINT('Ctrl Pts',(181.548326608462,618.098240988607,-36.8695043256539)) ;
#60291=CARTESIAN_POINT('Ctrl Pts',(181.542781725836,618.09474582968,-36.8180063112746)) ;
#60292=CARTESIAN_POINT('Ctrl Pts',(181.514217595271,618.081890330671,-36.6338123856813)) ;
#60293=CARTESIAN_POINT('Ctrl Pts',(181.477537922047,618.072092912377,-36.5037827927049)) ;
#60294=CARTESIAN_POINT('Ctrl Pts',(181.4051474434,618.058446751,-36.330610455888)) ;
#60295=CARTESIAN_POINT('Ctrl Pts',(181.382331038764,618.054602807897,-36.2826138745859)) ;
#60296=CARTESIAN_POINT('Ctrl Pts',(181.33877039037,618.048059947729,-36.2012544218042)) ;
#60297=CARTESIAN_POINT('Ctrl Pts',(181.319067309146,618.04532760079,-36.1673811517677)) ;
#60298=CARTESIAN_POINT('Ctrl Pts',(181.281655611491,618.040562685271,-36.1079870961481)) ;
#60299=CARTESIAN_POINT('Ctrl Pts',(181.264395351703,618.038507677835,-36.082210112539)) ;
#60300=CARTESIAN_POINT('Ctrl Pts',(181.18324135259,618.029404533506,-35.9680419194571)) ;
#60301=CARTESIAN_POINT('Ctrl Pts',(181.111474053317,618.022802296828,-35.8855610055033)) ;
#60302=CARTESIAN_POINT('Ctrl Pts',(180.979684533357,618.011732999542,-35.7611534299474)) ;
#60303=CARTESIAN_POINT('Ctrl Pts',(180.924060478161,618.007314191531,-35.7150901261825)) ;
#60304=CARTESIAN_POINT('Ctrl Pts',(180.817543656596,617.9990439276,-35.6379601023475)) ;
#60305=CARTESIAN_POINT('Ctrl Pts',(180.767636494697,617.995237429849,-35.6057397172037)) ;
#60306=CARTESIAN_POINT('Ctrl Pts',(180.67230584161,617.98800298968,-35.5511753422206)) ;
#60307=CARTESIAN_POINT('Ctrl Pts',(180.627378452858,617.984607805762,-35.5281042324051)) ;
#60308=CARTESIAN_POINT('Ctrl Pts',(180.492855145002,617.97444604565,-35.4665763354144)) ;
#60309=CARTESIAN_POINT('Ctrl Pts',(180.400862332379,617.967489679353,-35.4339031853769)) ;
#60310=CARTESIAN_POINT('Ctrl Pts',(180.205307591823,617.952828631034,-35.3832133669089)) ;
#60311=CARTESIAN_POINT('Ctrl Pts',(180.101808264679,617.945138619823,-35.3665607107201)) ;
#60312=CARTESIAN_POINT('Ctrl Pts',(179.962411799729,617.935307397315,-35.3574294270901)) ;
#60313=CARTESIAN_POINT('Ctrl Pts',(179.927329284662,617.932878886535,-35.3562423325857)) ;
#60314=CARTESIAN_POINT('Ctrl Pts',(179.859148410935,617.928280646042,-35.3560907253344)) ;
#60315=CARTESIAN_POINT('Ctrl Pts',(179.826067574678,617.926106581649,-35.3570026463725)) ;
#60316=CARTESIAN_POINT('Ctrl Pts',(179.622054283409,617.912930531312,-35.3687158150226)) ;
#60317=CARTESIAN_POINT('Ctrl Pts',(179.453592199867,617.902959063726,-35.4048368675258)) ;
#60318=CARTESIAN_POINT('Ctrl Pts',(179.236807105958,617.888398989924,-35.4877188114953)) ;
#60319=CARTESIAN_POINT('Ctrl Pts',(179.181273563675,617.884512014318,-35.5125111275231)) ;
#60320=CARTESIAN_POINT('Ctrl Pts',(179.082117176405,617.877183776244,-35.5634519465076)) ;
#60321=CARTESIAN_POINT('Ctrl Pts',(179.038097834638,617.873779650298,-35.5886694350974)) ;
#60322=CARTESIAN_POINT('Ctrl Pts',(178.870350467298,617.860149939329,-35.6952154510869)) ;
#60323=CARTESIAN_POINT('Ctrl Pts',(178.756556325577,617.849354523522,-35.7908641331461)) ;
#60324=CARTESIAN_POINT('Ctrl Pts',(178.623170438448,617.834965240491,-35.9372923197068)) ;
#60325=CARTESIAN_POINT('Ctrl Pts',(178.591111446813,617.83134612524,-35.9758433125001)) ;
#60326=CARTESIAN_POINT('Ctrl Pts',(178.5379905656,617.825124128182,-36.0459244798413)) ;
#60327=CARTESIAN_POINT('Ctrl Pts',(178.516174348507,617.822491688664,-36.0768382457494)) ;
#60328=CARTESIAN_POINT('Ctrl Pts',(178.478181265355,617.817797384028,-36.1347662242504)) ;
#60329=CARTESIAN_POINT('Ctrl Pts',(178.461682738277,617.815718549283,-36.1615448824615)) ;
#60330=CARTESIAN_POINT('Ctrl Pts',(178.386570477318,617.805980574862,-36.2915631430463)) ;
#60331=CARTESIAN_POINT('Ctrl Pts',(178.338337018995,617.798845451376,-36.4004171944896)) ;
#60332=CARTESIAN_POINT('Ctrl Pts',(178.281630845691,617.787485780771,-36.5772719921208)) ;
#60333=CARTESIAN_POINT('Ctrl Pts',(178.265045721292,617.783362615903,-36.6422282488572)) ;
#60334=CARTESIAN_POINT('Ctrl Pts',(178.241632304904,617.775522841004,-36.7641637083477)) ;
#60335=CARTESIAN_POINT('Ctrl Pts',(178.233748462783,617.771840787283,-36.8208368324697)) ;
#60336=CARTESIAN_POINT('Ctrl Pts',(178.224306918,617.764641388769,-36.9293866685259)) ;
#60337=CARTESIAN_POINT('Ctrl Pts',(178.2222279399,617.761145566237,-36.981150417142)) ;
#60338=CARTESIAN_POINT('Ctrl Pts',(178.223436185084,617.748245595999,-37.1681850253089)) ;
#60339=CARTESIAN_POINT('Ctrl Pts',(178.240780196684,617.738399051056,-37.3028164182479)) ;
#60340=CARTESIAN_POINT('Ctrl Pts',(178.287279400566,617.724716188803,-37.4851555156929)) ;
#60341=CARTESIAN_POINT('Ctrl Pts',(178.30280591029,617.720883078943,-37.5358214309226)) ;
#60342=CARTESIAN_POINT('Ctrl Pts',(178.333947161654,617.714355432036,-37.6224640495473)) ;
#60343=CARTESIAN_POINT('Ctrl Pts',(178.348466762302,617.71162764015,-37.6587906234727)) ;
#60344=CARTESIAN_POINT('Ctrl Pts',(178.376753752475,617.706870023981,-37.7229133633042)) ;
#60345=CARTESIAN_POINT('Ctrl Pts',(178.390042208449,617.704817839497,-37.750896646296)) ;
#60346=CARTESIAN_POINT('Ctrl Pts',(178.453788972829,617.695692104082,-37.8760095192563)) ;
#60347=CARTESIAN_POINT('Ctrl Pts',(178.512969306994,617.68906890695,-37.9684052799323)) ;
#60348=CARTESIAN_POINT('Ctrl Pts',(178.625433370478,617.677983737327,-38.110893464217)) ;
#60349=CARTESIAN_POINT('Ctrl Pts',(178.673692213999,617.67357124519,-38.164491644234)) ;
#60350=CARTESIAN_POINT('Ctrl Pts',(178.76773664091,617.665310238577,-38.2562198768082)) ;
#60351=CARTESIAN_POINT('Ctrl Pts',(178.812385195234,617.661506511059,-38.2953419920857)) ;
#60352=CARTESIAN_POINT('Ctrl Pts',(178.898698805325,617.654276242552,-38.3631828414228)) ;
#60353=CARTESIAN_POINT('Ctrl Pts',(178.939768869025,617.650882377663,-38.392546522685)) ;
#60354=CARTESIAN_POINT('Ctrl Pts',(179.066737170712,617.640487596817,-38.4748786383695)) ;
#60355=CARTESIAN_POINT('Ctrl Pts',(179.156164820347,617.633277320209,-38.5219498022823)) ;
#60356=CARTESIAN_POINT('Ctrl Pts',(179.320072900304,617.620387193143,-38.5900541117436)) ;
#60357=CARTESIAN_POINT('Ctrl Pts',(179.392808387375,617.614775331473,-38.6145467771622)) ;
#60358=CARTESIAN_POINT('Ctrl Pts',(179.513421079715,617.605836683831,-38.6460924593733)) ;
#60359=CARTESIAN_POINT('Ctrl Pts',(179.560377762781,617.60244506509,-38.6562286103148)) ;
#60360=CARTESIAN_POINT('Ctrl Pts',(179.636914680734,617.597124331008,-38.6693167197998)) ;
#60361=CARTESIAN_POINT('Ctrl Pts',(179.666243421498,617.595137480711,-38.673530440253)) ;
#60362=CARTESIAN_POINT('Ctrl Pts',(179.749303130417,617.589644790209,-38.6832102881073)) ;
#60363=CARTESIAN_POINT('Ctrl Pts',(179.803208794525,617.586228243378,-38.6868502193651)) ;
#60364=CARTESIAN_POINT('Ctrl Pts',(179.966553087462,617.576069001618,-38.6899221444192)) ;
#60365=CARTESIAN_POINT('Ctrl Pts',(180.075843088827,617.569517619354,-38.6812058408644)) ;
#60366=CARTESIAN_POINT('Ctrl Pts',(180.254133677697,617.558300975726,-38.6491327420644)) ;
#60367=CARTESIAN_POINT('Ctrl Pts',(180.323870596851,617.553777851979,-38.6318750748062)) ;
#60368=CARTESIAN_POINT('Ctrl Pts',(180.416389474131,617.547459445753,-38.6025265992448)) ;
#60369=CARTESIAN_POINT('Ctrl Pts',(180.440325112796,617.545795552742,-38.5943291378804)) ;
#60370=CARTESIAN_POINT('Ctrl Pts',(180.464060729575,617.544113575794,-38.585591540904)) ;
#60371=CARTESIAN_POINT('Origin',(29.8885276254218,617.710565160562,-37.0221601717529)) ;
#60372=CARTESIAN_POINT('Ctrl Pts',(30.4640776573931,618.051524931058,-38.5855853092948)) ;
#60373=CARTESIAN_POINT('Ctrl Pts',(30.4818456719863,618.050290927823,-38.5790442980743)) ;
#60374=CARTESIAN_POINT('Ctrl Pts',(30.4995011921984,618.049042110479,-38.5722007556456)) ;
#60375=CARTESIAN_POINT('Ctrl Pts',(30.5462955678426,618.045661610561,-38.5531387759382)) ;
#60376=CARTESIAN_POINT('Ctrl Pts',(30.5752048818118,618.04349626312,-38.5403920002099)) ;
#60377=CARTESIAN_POINT('Ctrl Pts',(30.7084201927192,618.033207854487,-38.4770719684504)) ;
#60378=CARTESIAN_POINT('Ctrl Pts',(30.8076237962935,618.024668323971,-38.4165243395425)) ;
#60379=CARTESIAN_POINT('Ctrl Pts',(30.9534704852753,618.011360591802,-38.3051350959759)) ;
#60380=CARTESIAN_POINT('Ctrl Pts',(31.0046631393638,618.006509591305,-38.2608575267715)) ;
#60381=CARTESIAN_POINT('Ctrl Pts',(31.0940165469926,617.997751623709,-38.1735235524342)) ;
#60382=CARTESIAN_POINT('Ctrl Pts',(31.1329149943528,617.993818537425,-38.131368290329)) ;
#60383=CARTESIAN_POINT('Ctrl Pts',(31.2023047439392,617.986547018802,-38.0479124602167)) ;
#60384=CARTESIAN_POINT('Ctrl Pts',(31.2332123482895,617.983193540939,-38.0070469768964)) ;
#60385=CARTESIAN_POINT('Ctrl Pts',(31.3414893771724,617.970908134843,-37.849263170228)) ;
#60386=CARTESIAN_POINT('Ctrl Pts',(31.405888891316,617.962504936777,-37.7241677596789)) ;
#60387=CARTESIAN_POINT('Ctrl Pts',(31.4713684294433,617.950758747922,-37.5444477170903)) ;
#60388=CARTESIAN_POINT('Ctrl Pts',(31.4866471646106,617.947591831547,-37.4956393027532)) ;
#60389=CARTESIAN_POINT('Ctrl Pts',(31.5093891828534,617.941906059241,-37.4092334991467)) ;
#60390=CARTESIAN_POINT('Ctrl Pts',(31.5178445228336,617.939426510315,-37.3719369672922)) ;
#60391=CARTESIAN_POINT('Ctrl Pts',(31.5308101022122,617.93480854639,-37.3039801052054)) ;
#60392=CARTESIAN_POINT('Ctrl Pts',(31.5357617716007,617.9326927768,-37.2734234931605)) ;
#60393=CARTESIAN_POINT('Ctrl Pts',(31.5560746289672,617.922017345664,-37.1213625090232)) ;
#60394=CARTESIAN_POINT('Ctrl Pts',(31.5588552417217,617.912976513806,-36.9985643991712)) ;
#60395=CARTESIAN_POINT('Ctrl Pts',(31.5424119202767,617.899347648282,-36.8111112224762)) ;
#60396=CARTESIAN_POINT('Ctrl Pts',(31.5328000530154,617.894642212824,-36.7460357643791)) ;
#60397=CARTESIAN_POINT('Ctrl Pts',(31.5078226835382,617.886089580696,-36.6263942265101)) ;
#60398=CARTESIAN_POINT('Ctrl Pts',(31.4934720677684,617.882219584392,-36.5717138933188)) ;
#60399=CARTESIAN_POINT('Ctrl Pts',(31.4607696472319,617.874991198607,-36.468746469291)) ;
#60400=CARTESIAN_POINT('Ctrl Pts',(31.4428987856974,617.871621439277,-36.4203770229569)) ;
#60401=CARTESIAN_POINT('Ctrl Pts',(31.3703281803715,617.859684239035,-36.2488809902844)) ;
#60402=CARTESIAN_POINT('Ctrl Pts',(31.303000783241,617.85158996359,-36.1316759864843)) ;
#60403=CARTESIAN_POINT('Ctrl Pts',(31.1905334887416,617.840078860783,-35.9814172372909)) ;
#60404=CARTESIAN_POINT('Ctrl Pts',(31.1567691755805,617.836802427588,-35.9405282078948)) ;
#60405=CARTESIAN_POINT('Ctrl Pts',(31.094829049508,617.830953626428,-35.8724125513417)) ;
#60406=CARTESIAN_POINT('Ctrl Pts',(31.0675354311014,617.828424046375,-35.8444408971369)) ;
#60407=CARTESIAN_POINT('Ctrl Pts',(31.0171161273781,617.823775587866,-35.7962792455947)) ;
#60408=CARTESIAN_POINT('Ctrl Pts',(30.9943692913621,617.821683057149,-35.7757213844907)) ;
#60409=CARTESIAN_POINT('Ctrl Pts',(30.8859443273232,617.811769591665,-35.6830342742105)) ;
#60410=CARTESIAN_POINT('Ctrl Pts',(30.7937035328853,617.803538683679,-35.6190382322996)) ;
#60411=CARTESIAN_POINT('Ctrl Pts',(30.6336727989741,617.790249959462,-35.5303993200199)) ;
#60412=CARTESIAN_POINT('Ctrl Pts',(30.5694572331204,617.785142238358,-35.5000141661783)) ;
#60413=CARTESIAN_POINT('Ctrl Pts',(30.4489076266454,617.776025657702,-35.4521347194695)) ;
#60414=CARTESIAN_POINT('Ctrl Pts',(30.3932081870512,617.771984564492,-35.4333541118267)) ;
#60415=CARTESIAN_POINT('Ctrl Pts',(30.2883116761563,617.764672414124,-35.4040609573287)) ;
#60416=CARTESIAN_POINT('Ctrl Pts',(30.2394084863563,617.761378460968,-35.3927566374694)) ;
#60417=CARTESIAN_POINT('Ctrl Pts',(30.0972470102894,617.752072374018,-35.3665940584388)) ;
#60418=CARTESIAN_POINT('Ctrl Pts',(30.0031407018643,617.746249342071,-35.3574290077688)) ;
#60419=CARTESIAN_POINT('Ctrl Pts',(29.8039076173302,617.734066485181,-35.3550099045083)) ;
#60420=CARTESIAN_POINT('Ctrl Pts',(29.6991857058721,617.727744633259,-35.3636380733002)) ;
#60421=CARTESIAN_POINT('Ctrl Pts',(29.5604244046807,617.718733336085,-35.3883888196727)) ;
#60422=CARTESIAN_POINT('Ctrl Pts',(29.5250861460649,617.716380256525,-35.3958851863884)) ;
#60423=CARTESIAN_POINT('Ctrl Pts',(29.4589862350037,617.71182047343,-35.4121688880796)) ;
#60424=CARTESIAN_POINT('Ctrl Pts',(29.4281807049303,617.709626711706,-35.4207052546039)) ;
#60425=CARTESIAN_POINT('Ctrl Pts',(29.3611441736728,617.704727563542,-35.4413750519209)) ;
#60426=CARTESIAN_POINT('Ctrl Pts',(29.3250446726323,617.702007596982,-35.4538804024139)) ;
#60427=CARTESIAN_POINT('Ctrl Pts',(29.205128899131,617.692760763286,-35.5000956307671)) ;
#60428=CARTESIAN_POINT('Ctrl Pts',(29.1236295352537,617.686129251742,-35.5393771226264)) ;
#60429=CARTESIAN_POINT('Ctrl Pts',(28.9738555782342,617.673594072776,-35.6272153975295)) ;
#60430=CARTESIAN_POINT('Ctrl Pts',(28.9052495406499,617.667690568227,-35.6746944628909)) ;
#60431=CARTESIAN_POINT('Ctrl Pts',(28.8013261420252,617.658524957484,-35.7587974524013)) ;
#60432=CARTESIAN_POINT('Ctrl Pts',(28.7636306321819,617.655144428079,-35.7922414189451)) ;
#60433=CARTESIAN_POINT('Ctrl Pts',(28.684157823262,617.647860736573,-35.8694665821047)) ;
#60434=CARTESIAN_POINT('Ctrl Pts',(28.643131838263,617.643994449372,-35.9139184005192)) ;
#60435=CARTESIAN_POINT('Ctrl Pts',(28.5567277594694,617.635487501786,-36.0184118363563)) ;
#60436=CARTESIAN_POINT('Ctrl Pts',(28.5128168078336,617.630898412853,-36.0794925029505)) ;
#60437=CARTESIAN_POINT('Ctrl Pts',(28.4199550443869,617.620151354334,-36.2290458686609)) ;
#60438=CARTESIAN_POINT('Ctrl Pts',(28.3746356837195,617.614019268511,-36.3194073610899)) ;
#60439=CARTESIAN_POINT('Ctrl Pts',(28.3263148046611,617.605447153156,-36.442479280643)) ;
#60440=CARTESIAN_POINT('Ctrl Pts',(28.3156840190504,617.603375712698,-36.4719768539655)) ;
#60441=CARTESIAN_POINT('Ctrl Pts',(28.2942597075081,617.598730379822,-36.5371317734945)) ;
#60442=CARTESIAN_POINT('Ctrl Pts',(28.2838179719575,617.596141088353,-36.5728839674862)) ;
#60443=CARTESIAN_POINT('Ctrl Pts',(28.2481799774797,617.585982904501,-36.7120819264732)) ;
#60444=CARTESIAN_POINT('Ctrl Pts',(28.2317228367642,617.578145749688,-36.8175006276438)) ;
#60445=CARTESIAN_POINT('Ctrl Pts',(28.2200722279935,617.563857051982,-37.0144211210282)) ;
#60446=CARTESIAN_POINT('Ctrl Pts',(28.2221293580943,617.557391996336,-37.1053757923779)) ;
#60447=CARTESIAN_POINT('Ctrl Pts',(28.2368128262116,617.547712859347,-37.2455536526412)) ;
#60448=CARTESIAN_POINT('Ctrl Pts',(28.2442783419981,617.5443432134,-37.2951284196061)) ;
#60449=CARTESIAN_POINT('Ctrl Pts',(28.2653598088032,617.537162685162,-37.4020984579944)) ;
#60450=CARTESIAN_POINT('Ctrl Pts',(28.2798102019331,617.533384023455,-37.4592601579964)) ;
#60451=CARTESIAN_POINT('Ctrl Pts',(28.3184101836088,617.52518551653,-37.5837537888375)) ;
#60452=CARTESIAN_POINT('Ctrl Pts',(28.3439248318459,617.520809406309,-37.6505385477115)) ;
#60453=CARTESIAN_POINT('Ctrl Pts',(28.4196780636781,617.509691722744,-37.8160561374397)) ;
#60454=CARTESIAN_POINT('Ctrl Pts',(28.4756028865259,617.503003894171,-37.9117817467726)) ;
#60455=CARTESIAN_POINT('Ctrl Pts',(28.5586555933462,617.493816530612,-38.0261231713888)) ;
#60456=CARTESIAN_POINT('Ctrl Pts',(28.5774087359438,617.49177902755,-38.0504930315122)) ;
#60457=CARTESIAN_POINT('Ctrl Pts',(28.6213285451078,617.487058127052,-38.1044114277407)) ;
#60458=CARTESIAN_POINT('Ctrl Pts',(28.6468725582231,617.484352754573,-38.1336246865377)) ;
#60459=CARTESIAN_POINT('Ctrl Pts',(28.7092403974957,617.477890662774,-38.2001163093121)) ;
#60460=CARTESIAN_POINT('Ctrl Pts',(28.7468501226909,617.474101439079,-38.2366027750438)) ;
#60461=CARTESIAN_POINT('Ctrl Pts',(28.8885330197957,617.46036169212,-38.3616479536149)) ;
#60462=CARTESIAN_POINT('Ctrl Pts',(29.0017041054897,617.450409256473,-38.4391197454327)) ;
#60463=CARTESIAN_POINT('Ctrl Pts',(29.1687690805487,617.43743934702,-38.5255395688852)) ;
#60464=CARTESIAN_POINT('Ctrl Pts',(29.2155312610575,617.433966408222,-38.5470466895237)) ;
#60465=CARTESIAN_POINT('Ctrl Pts',(29.3158620762587,617.42681389369,-38.587674758124)) ;
#60466=CARTESIAN_POINT('Ctrl Pts',(29.3695650709878,617.423155481785,-38.6062879455168)) ;
#60467=CARTESIAN_POINT('Ctrl Pts',(29.4878944797641,617.415373055664,-38.64063445404)) ;
#60468=CARTESIAN_POINT('Ctrl Pts',(29.5527225575204,617.411282742807,-38.6553171937956)) ;
#60469=CARTESIAN_POINT('Ctrl Pts',(29.7366612888557,617.399877920146,-38.6855576059664)) ;
#60470=CARTESIAN_POINT('Ctrl Pts',(29.8568045362706,617.392671455821,-38.692172106418)) ;
#60471=CARTESIAN_POINT('Ctrl Pts',(30.0077543928523,617.382863710481,-38.6841813934836)) ;
#60472=CARTESIAN_POINT('Ctrl Pts',(30.0388585672411,617.380800388477,-38.681657096448)) ;
#60473=CARTESIAN_POINT('Ctrl Pts',(30.1074146886604,617.376126461875,-38.674150100114)) ;
#60474=CARTESIAN_POINT('Ctrl Pts',(30.1448019559705,617.373498443337,-38.6687643008992)) ;
#60475=CARTESIAN_POINT('Ctrl Pts',(30.2780697697598,617.36392042104,-38.6449182485453)) ;
#60476=CARTESIAN_POINT('Ctrl Pts',(30.3724668659848,617.356753594313,-38.6193101182596)) ;
#60477=CARTESIAN_POINT('Ctrl Pts',(30.4640740060252,617.349670188918,-38.5855866534828)) ;
#60478=CARTESIAN_POINT('Ctrl Pts',(30.4640776731659,618.242171075974,-38.5855853034883)) ;
#60479=CARTESIAN_POINT('Ctrl Pts',(30.478405831787,618.24123936245,-38.5803106202233)) ;
#60480=CARTESIAN_POINT('Ctrl Pts',(30.4926650383209,618.240308364873,-38.5748376596405)) ;
#60481=CARTESIAN_POINT('Ctrl Pts',(30.575751765421,618.234852090735,-38.541628719478)) ;
#60482=CARTESIAN_POINT('Ctrl Pts',(30.64273248298,618.230321559955,-38.5095188079244)) ;
#60483=CARTESIAN_POINT('Ctrl Pts',(30.7597095722704,618.221895633445,-38.4435022114046)) ;
#60484=CARTESIAN_POINT('Ctrl Pts',(30.8104287437074,618.218049965343,-38.411141148849)) ;
#60485=CARTESIAN_POINT('Ctrl Pts',(30.9002930855428,618.210781366303,-38.3467102479627)) ;
#60486=CARTESIAN_POINT('Ctrl Pts',(30.9399406736874,618.207394080935,-38.3154628759016)) ;
#60487=CARTESIAN_POINT('Ctrl Pts',(31.0901105503909,618.193779859586,-38.1856359376912)) ;
#60488=CARTESIAN_POINT('Ctrl Pts',(31.1886875255874,618.182979929582,-38.0743215218763)) ;
#60489=CARTESIAN_POINT('Ctrl Pts',(31.2991000518324,618.168601050621,-37.9100426161833)) ;
#60490=CARTESIAN_POINT('Ctrl Pts',(31.3250807476398,618.164994686982,-37.8673616701239)) ;
#60491=CARTESIAN_POINT('Ctrl Pts',(31.3672539176288,618.15879213722,-37.7905011188881)) ;
#60492=CARTESIAN_POINT('Ctrl Pts',(31.3842749784051,618.15616656847,-37.7568163467594)) ;
#60493=CARTESIAN_POINT('Ctrl Pts',(31.4133330058182,618.151483323579,-37.6941046929351)) ;
#60494=CARTESIAN_POINT('Ctrl Pts',(31.4257200000535,618.149408774511,-37.6652625159311)) ;
#60495=CARTESIAN_POINT('Ctrl Pts',(31.4750099867373,618.140734675637,-37.5409181177682)) ;
#60496=CARTESIAN_POINT('Ctrl Pts',(31.5038876224152,618.134517533878,-37.4424622096123)) ;
#60497=CARTESIAN_POINT('Ctrl Pts',(31.5378980340447,618.123703999771,-37.2685833891882)) ;
#60498=CARTESIAN_POINT('Ctrl Pts',(31.547294361471,618.119136678163,-37.1943201711079)) ;
#60499=CARTESIAN_POINT('Ctrl Pts',(31.5552085104096,618.110652375872,-37.0593504951988)) ;
#60500=CARTESIAN_POINT('Ctrl Pts',(31.5554604097298,618.106785992725,-36.998878804543)) ;
#60501=CARTESIAN_POINT('Ctrl Pts',(31.549879823527,618.099476058329,-36.8878451430808)) ;
#60502=CARTESIAN_POINT('Ctrl Pts',(31.5450178368784,618.09606831119,-36.8373065749465)) ;
#60503=CARTESIAN_POINT('Ctrl Pts',(31.5183605802869,618.083108479532,-36.6502839179391)) ;
#60504=CARTESIAN_POINT('Ctrl Pts',(31.4819251881433,618.073077486742,-36.5164757788996)) ;
#60505=CARTESIAN_POINT('Ctrl Pts',(31.4085455969428,618.059038998112,-36.3379722042353)) ;
#60506=CARTESIAN_POINT('Ctrl Pts',(31.3851831201593,618.055061839461,-36.2882726876611)) ;
#60507=CARTESIAN_POINT('Ctrl Pts',(31.340654505117,618.048330936388,-36.2045548300127)) ;
#60508=CARTESIAN_POINT('Ctrl Pts',(31.3206364270694,618.045541417183,-36.1699770867571)) ;
#60509=CARTESIAN_POINT('Ctrl Pts',(31.2830349939648,618.040736876678,-36.1101013706384)) ;
#60510=CARTESIAN_POINT('Ctrl Pts',(31.2659615111449,618.038696445318,-36.084515216137)) ;
#60511=CARTESIAN_POINT('Ctrl Pts',(31.1983867054137,618.031087428169,-35.9890815479631)) ;
#60512=CARTESIAN_POINT('Ctrl Pts',(31.1431987958555,618.025787189952,-35.9227119536607)) ;
#60513=CARTESIAN_POINT('Ctrl Pts',(31.0241135103691,618.015339944938,-35.8002084646993)) ;
#60514=CARTESIAN_POINT('Ctrl Pts',(30.9605738535416,618.010205023156,-35.7441001621896)) ;
#60515=CARTESIAN_POINT('Ctrl Pts',(30.8418513938379,618.000913950436,-35.6543707141084)) ;
#60516=CARTESIAN_POINT('Ctrl Pts',(30.7884684064382,617.996831089576,-35.6186719285698)) ;
#60517=CARTESIAN_POINT('Ctrl Pts',(30.6898354743301,617.989336436594,-35.5606579933332)) ;
#60518=CARTESIAN_POINT('Ctrl Pts',(30.6453799794246,617.985975435694,-35.5371495815042)) ;
#60519=CARTESIAN_POINT('Ctrl Pts',(30.5273010973506,617.977054153712,-35.4813887995339)) ;
#60520=CARTESIAN_POINT('Ctrl Pts',(30.4522940376825,617.97138790265,-35.4523920555794)) ;
#60521=CARTESIAN_POINT('Ctrl Pts',(30.2838439518898,617.958708337387,-35.4009056120791)) ;
#60522=CARTESIAN_POINT('Ctrl Pts',(30.1899471763949,617.951666351828,-35.3808537809)) ;
#60523=CARTESIAN_POINT('Ctrl Pts',(30.0560091198578,617.941943615365,-35.3641378474514)) ;
#60524=CARTESIAN_POINT('Ctrl Pts',(30.0170069283446,617.939152099863,-35.360660368693)) ;
#60525=CARTESIAN_POINT('Ctrl Pts',(29.9454843796962,617.934144009723,-35.3568173353109)) ;
#60526=CARTESIAN_POINT('Ctrl Pts',(29.9130044188139,617.931911667228,-35.3560232270462)) ;
#60527=CARTESIAN_POINT('Ctrl Pts',(29.8446125751714,617.927326629971,-35.3563520635515)) ;
#60528=CARTESIAN_POINT('Ctrl Pts',(29.8087191204132,617.924984799699,-35.3576853897329)) ;
#60529=CARTESIAN_POINT('Ctrl Pts',(29.6116020615684,617.912341183982,-35.3714000279462)) ;
#60530=CARTESIAN_POINT('Ctrl Pts',(29.4527894116313,617.902877757318,-35.4060408198108)) ;
#60531=CARTESIAN_POINT('Ctrl Pts',(29.2434699455966,617.888871839149,-35.4848593017614)) ;
#60532=CARTESIAN_POINT('Ctrl Pts',(29.1867661957619,617.884917842321,-35.5099026427465)) ;
#60533=CARTESIAN_POINT('Ctrl Pts',(29.0866160899477,617.877537851914,-35.5609815355461)) ;
#60534=CARTESIAN_POINT('Ctrl Pts',(29.0427101341918,617.874153834571,-35.5859509509979)) ;
#60535=CARTESIAN_POINT('Ctrl Pts',(28.8724525947701,617.86037050265,-35.6932938257871)) ;
#60536=CARTESIAN_POINT('Ctrl Pts',(28.7564275144876,617.849371175943,-35.7906471723882)) ;
#60537=CARTESIAN_POINT('Ctrl Pts',(28.6217341314801,617.834818458955,-35.9389913871157)) ;
#60538=CARTESIAN_POINT('Ctrl Pts',(28.5900205326611,617.831234689477,-35.9772198201013)) ;
#60539=CARTESIAN_POINT('Ctrl Pts',(28.5373671982883,617.82506361963,-36.0467958201318)) ;
#60540=CARTESIAN_POINT('Ctrl Pts',(28.5156939178457,617.82244737342,-36.0775447441099)) ;
#60541=CARTESIAN_POINT('Ctrl Pts',(28.4777961269415,617.817763697418,-36.1353756591398)) ;
#60542=CARTESIAN_POINT('Ctrl Pts',(28.4612660100266,617.815680211949,-36.162233108645)) ;
#60543=CARTESIAN_POINT('Ctrl Pts',(28.3866327544997,617.805999203518,-36.2915813352369)) ;
#60544=CARTESIAN_POINT('Ctrl Pts',(28.338738448464,617.798915398544,-36.3995889590225)) ;
#60545=CARTESIAN_POINT('Ctrl Pts',(28.2820367281247,617.787596668335,-36.5757694074248)) ;
#60546=CARTESIAN_POINT('Ctrl Pts',(28.265331217687,617.783458758455,-36.6409644953251)) ;
#60547=CARTESIAN_POINT('Ctrl Pts',(28.2417727246344,617.775597861706,-36.763245465266)) ;
#60548=CARTESIAN_POINT('Ctrl Pts',(28.2338443967964,617.771909955589,-36.8200198026846)) ;
#60549=CARTESIAN_POINT('Ctrl Pts',(28.224353135804,617.764709795088,-36.9286005588733)) ;
#60550=CARTESIAN_POINT('Ctrl Pts',(28.2222514882408,617.761219630867,-36.9802921882637)) ;
#60551=CARTESIAN_POINT('Ctrl Pts',(28.2233603958254,617.748264883254,-37.1681689594493)) ;
#60552=CARTESIAN_POINT('Ctrl Pts',(28.2408576916802,617.738349618598,-37.3037107583147)) ;
#60553=CARTESIAN_POINT('Ctrl Pts',(28.2876994686318,617.724625479872,-37.4865690028681)) ;
#60554=CARTESIAN_POINT('Ctrl Pts',(28.3031705176895,617.720816770115,-37.5369124109155)) ;
#60555=CARTESIAN_POINT('Ctrl Pts',(28.3341957218464,617.714323906873,-37.6230978954343)) ;
#60556=CARTESIAN_POINT('Ctrl Pts',(28.348674509093,617.711606926103,-37.6592840365282)) ;
#60557=CARTESIAN_POINT('Ctrl Pts',(28.3769324541012,617.706857621446,-37.7233003641909)) ;
#60558=CARTESIAN_POINT('Ctrl Pts',(28.3902440041931,617.704803511503,-37.7513129941224)) ;
#60559=CARTESIAN_POINT('Ctrl Pts',(28.4537487116756,617.695719699661,-37.8758585683142)) ;
#60560=CARTESIAN_POINT('Ctrl Pts',(28.5125486704521,617.689133728099,-37.9677182434717)) ;
#60561=CARTESIAN_POINT('Ctrl Pts',(28.6246247468857,617.678075055629,-38.1099696175061)) ;
#60562=CARTESIAN_POINT('Ctrl Pts',(28.6729992614358,617.673649685354,-38.1637685392274)) ;
#60563=CARTESIAN_POINT('Ctrl Pts',(28.7672250576991,617.665370428635,-38.2557592545631)) ;
#60564=CARTESIAN_POINT('Ctrl Pts',(28.8119242010044,617.661561811506,-38.2949562666162)) ;
#60565=CARTESIAN_POINT('Ctrl Pts',(28.8982534605353,617.654329529728,-38.3628524801289)) ;
#60566=CARTESIAN_POINT('Ctrl Pts',(28.939280250983,617.650938960327,-38.3922066114468)) ;
#60567=CARTESIAN_POINT('Ctrl Pts',(29.0606903072189,617.64099843398,-38.4710003153332)) ;
#60568=CARTESIAN_POINT('Ctrl Pts',(29.1440141330573,617.634275604268,-38.5155277819997)) ;
#60569=CARTESIAN_POINT('Ctrl Pts',(29.3052302844579,617.621552783197,-38.5848217212131)) ;
#60570=CARTESIAN_POINT('Ctrl Pts',(29.3820604664016,617.615602499589,-38.6113858330639)) ;
#60571=CARTESIAN_POINT('Ctrl Pts',(29.508270477064,617.606226831418,-38.6449360530594)) ;
#60572=CARTESIAN_POINT('Ctrl Pts',(29.5565657400658,617.602730967901,-38.6555001333034)) ;
#60573=CARTESIAN_POINT('Ctrl Pts',(29.6344098776543,617.5973121353,-38.6689312362371)) ;
#60574=CARTESIAN_POINT('Ctrl Pts',(29.6636824628802,617.595325881698,-38.6731827991571)) ;
#60575=CARTESIAN_POINT('Ctrl Pts',(29.7465698481081,617.589837088992,-38.6829754234697)) ;
#60576=CARTESIAN_POINT('Ctrl Pts',(29.8003615577277,617.586424048284,-38.6866983577146)) ;
#60577=CARTESIAN_POINT('Ctrl Pts',(29.9642624515506,617.57622300459,-38.6900718178251)) ;
#60578=CARTESIAN_POINT('Ctrl Pts',(30.0742358677732,617.569633292837,-38.6814308653686)) ;
#60579=CARTESIAN_POINT('Ctrl Pts',(30.2533719695118,617.558366428119,-38.6493112177922)) ;
#60580=CARTESIAN_POINT('Ctrl Pts',(30.3232813592806,617.553833519323,-38.6320418896756)) ;
#60581=CARTESIAN_POINT('Ctrl Pts',(30.4161161524597,617.547494864546,-38.6026203312522)) ;
#60582=CARTESIAN_POINT('Ctrl Pts',(30.4401981230646,617.545820985094,-38.5943761792912)) ;
#60583=CARTESIAN_POINT('Ctrl Pts',(30.4640776716666,617.544128797339,-38.5855853040402)) ;
#60584=CARTESIAN_POINT('Origin',(29.8885276254223,620.2564904411,-37.0221601717529)) ;
#60585=CARTESIAN_POINT('Ctrl Pts',(31.5177255210653,618.256605597192,-35.7700771955364)) ;
#60586=CARTESIAN_POINT('Ctrl Pts',(31.4358975948208,618.249786276961,-35.6636035130611)) ;
#60587=CARTESIAN_POINT('Ctrl Pts',(31.3438305866016,618.243420671915,-35.5654073397872)) ;
#60588=CARTESIAN_POINT('Ctrl Pts',(31.1659268453259,618.231906784935,-35.4094901911848)) ;
#60589=CARTESIAN_POINT('Ctrl Pts',(31.0841098667658,618.226850009824,-35.3479339294522)) ;
#60590=CARTESIAN_POINT('Ctrl Pts',(30.9541032131772,618.218854762731,-35.2645272696165)) ;
#60591=CARTESIAN_POINT('Ctrl Pts',(30.9090927907251,618.21609514327,-35.2380158855215)) ;
#60592=CARTESIAN_POINT('Ctrl Pts',(30.8154875863962,618.210345137083,-35.187583728142)) ;
#60593=CARTESIAN_POINT('Ctrl Pts',(30.7668596171457,618.207352245656,-35.1638120824583)) ;
#60594=CARTESIAN_POINT('Ctrl Pts',(30.5631220148783,618.194769322437,-35.0739995647562)) ;
#60595=CARTESIAN_POINT('Ctrl Pts',(30.4011298183337,618.184593215762,-35.0252553221851)) ;
#60596=CARTESIAN_POINT('Ctrl Pts',(30.1764578127107,618.170920420864,-34.9868158716723)) ;
#60597=CARTESIAN_POINT('Ctrl Pts',(30.1174626865178,618.167378316383,-34.9793386835085)) ;
#60598=CARTESIAN_POINT('Ctrl Pts',(30.0148354621986,618.16138019276,-34.9708339230574)) ;
#60599=CARTESIAN_POINT('Ctrl Pts',(29.9713403548589,618.158888849364,-34.9686179490241)) ;
#60600=CARTESIAN_POINT('Ctrl Pts',(29.8986584161905,618.154846009495,-34.9672283612392)) ;
#60601=CARTESIAN_POINT('Ctrl Pts',(29.8695057571334,618.153258829605,-34.9672913864728)) ;
#60602=CARTESIAN_POINT('Ctrl Pts',(29.7937955336326,618.149221228424,-34.9690667123986)) ;
#60603=CARTESIAN_POINT('Ctrl Pts',(29.747279033869,618.146818877027,-34.971741582058)) ;
#60604=CARTESIAN_POINT('Ctrl Pts',(29.5646466340215,618.137558997937,-34.9884893175988)) ;
#60605=CARTESIAN_POINT('Ctrl Pts',(29.4299833001195,618.131089343044,-35.0145600535208)) ;
#60606=CARTESIAN_POINT('Ctrl Pts',(29.2069408376618,618.119725902436,-35.0813734454084)) ;
#60607=CARTESIAN_POINT('Ctrl Pts',(29.1170285565647,618.114956535324,-35.1153302566464)) ;
#60608=CARTESIAN_POINT('Ctrl Pts',(28.9827665072291,618.107293831612,-35.1770917490866)) ;
#60609=CARTESIAN_POINT('Ctrl Pts',(28.9365464882667,618.1045520558,-35.2005092851128)) ;
#60610=CARTESIAN_POINT('Ctrl Pts',(28.8434668763486,618.098786513679,-35.252178809114)) ;
#60611=CARTESIAN_POINT('Ctrl Pts',(28.7967522536233,618.095757797261,-35.2806057745684)) ;
#60612=CARTESIAN_POINT('Ctrl Pts',(28.6159992991661,618.08347149598,-35.4007307871783)) ;
#60613=CARTESIAN_POINT('Ctrl Pts',(28.4919153680927,618.073683245127,-35.5063038391899)) ;
#60614=CARTESIAN_POINT('Ctrl Pts',(28.3213146111363,618.058617679057,-35.6903578754549)) ;
#60615=CARTESIAN_POINT('Ctrl Pts',(28.2653241296603,618.05333994272,-35.7592005477882)) ;
#60616=CARTESIAN_POINT('Ctrl Pts',(28.1952477771545,618.046463800495,-35.8577536017175)) ;
#60617=CARTESIAN_POINT('Ctrl Pts',(28.1771649606245,618.044661272511,-35.8844970129365)) ;
#60618=CARTESIAN_POINT('Ctrl Pts',(28.1418160754024,618.041096823548,-35.939527475035)) ;
#60619=CARTESIAN_POINT('Ctrl Pts',(28.1245891198471,618.039337256018,-35.9678281433063)) ;
#60620=CARTESIAN_POINT('Ctrl Pts',(28.0406662650907,618.030582618844,-36.1135173168416)) ;
#60621=CARTESIAN_POINT('Ctrl Pts',(27.9849650321949,618.024133348046,-36.2368697454498)) ;
#60622=CARTESIAN_POINT('Ctrl Pts',(27.915405734525,618.013602410858,-36.4428706121116)) ;
#60623=CARTESIAN_POINT('Ctrl Pts',(27.8937665689741,618.009590964145,-36.5224465309044)) ;
#60624=CARTESIAN_POINT('Ctrl Pts',(27.8635604156702,618.002160791058,-36.6674425830066)) ;
#60625=CARTESIAN_POINT('Ctrl Pts',(27.8532525194182,617.998791543164,-36.732382878791)) ;
#60626=CARTESIAN_POINT('Ctrl Pts',(27.8406308303826,617.992692065399,-36.847233566189)) ;
#60627=CARTESIAN_POINT('Ctrl Pts',(27.8369914157998,617.99000672271,-36.8969436513977)) ;
#60628=CARTESIAN_POINT('Ctrl Pts',(27.8327554744115,617.98365306082,-37.0122609985426)) ;
#60629=CARTESIAN_POINT('Ctrl Pts',(27.8334866667382,617.97994521523,-37.0778595938705)) ;
#60630=CARTESIAN_POINT('Ctrl Pts',(27.8460559423183,617.967614698141,-37.2906753371488)) ;
#60631=CARTESIAN_POINT('Ctrl Pts',(27.8706162737434,617.958649045103,-37.4366674794061)) ;
#60632=CARTESIAN_POINT('Ctrl Pts',(27.9309603652972,617.945331043468,-37.651111086265)) ;
#60633=CARTESIAN_POINT('Ctrl Pts',(27.9552813842903,617.940892200627,-37.7223099487288)) ;
#60634=CARTESIAN_POINT('Ctrl Pts',(27.9952319771609,617.934847575687,-37.8211705799566)) ;
#60635=CARTESIAN_POINT('Ctrl Pts',(28.0076803922372,617.933097230471,-37.8500491306183)) ;
#60636=CARTESIAN_POINT('Ctrl Pts',(28.0350613669596,617.92952734202,-37.9097597191898)) ;
#60637=CARTESIAN_POINT('Ctrl Pts',(28.0501114284404,617.92771457136,-37.9405262861034)) ;
#60638=CARTESIAN_POINT('Ctrl Pts',(28.1320656161547,617.918505662467,-38.097965968923)) ;
#60639=CARTESIAN_POINT('Ctrl Pts',(28.2113196451691,617.911707233053,-38.2177768922417)) ;
#60640=CARTESIAN_POINT('Ctrl Pts',(28.3513203719568,617.901020474753,-38.3877783254848)) ;
#60641=CARTESIAN_POINT('Ctrl Pts',(28.4035349621028,617.897254965393,-38.4443819938088)) ;
#60642=CARTESIAN_POINT('Ctrl Pts',(28.5042370854527,617.890193705942,-38.5419429858827)) ;
#60643=CARTESIAN_POINT('Ctrl Pts',(28.5516810214853,617.886937925585,-38.5838388270995)) ;
#60644=CARTESIAN_POINT('Ctrl Pts',(28.6398428414635,617.880949627062,-38.6547258645091)) ;
#60645=CARTESIAN_POINT('Ctrl Pts',(28.6798286065754,617.878254620663,-38.6845471616879)) ;
#60646=CARTESIAN_POINT('Ctrl Pts',(28.7771038448506,617.871727751243,-38.7517287382187)) ;
#60647=CARTESIAN_POINT('Ctrl Pts',(28.8352485933516,617.867848073146,-38.7877399621918)) ;
#60648=CARTESIAN_POINT('Ctrl Pts',(29.0256835504104,617.855216377419,-38.8929248440873)) ;
#60649=CARTESIAN_POINT('Ctrl Pts',(29.1637549042228,617.84613100121,-38.9506199250456)) ;
#60650=CARTESIAN_POINT('Ctrl Pts',(29.373239653949,617.83310852921,-39.0124541009729)) ;
#60651=CARTESIAN_POINT('Ctrl Pts',(29.4406005402208,617.829037462199,-39.0286881568952)) ;
#60652=CARTESIAN_POINT('Ctrl Pts',(29.5390805754258,617.823367767415,-39.0472139081433)) ;
#60653=CARTESIAN_POINT('Ctrl Pts',(29.5696320867122,617.821647890139,-39.0522493161275)) ;
#60654=CARTESIAN_POINT('Ctrl Pts',(29.6349849706317,617.818067302193,-39.0615085068973)) ;
#60655=CARTESIAN_POINT('Ctrl Pts',(29.6698029308128,617.816216386936,-39.0655361382003)) ;
#60656=CARTESIAN_POINT('Ctrl Pts',(29.841214681719,617.807308357833,-39.0809324168315)) ;
#60657=CARTESIAN_POINT('Ctrl Pts',(29.9786188482924,617.800784336763,-39.0795063047954)) ;
#60658=CARTESIAN_POINT('Ctrl Pts',(30.1933287323379,617.790310328148,-39.0557101414683)) ;
#60659=CARTESIAN_POINT('Ctrl Pts',(30.2712194056519,617.786454970081,-39.0425005435805)) ;
#60660=CARTESIAN_POINT('Ctrl Pts',(30.4107047848824,617.779258388538,-39.0104879362867)) ;
#60661=CARTESIAN_POINT('Ctrl Pts',(30.4725440640204,617.775960531024,-38.9932106564754)) ;
#60662=CARTESIAN_POINT('Ctrl Pts',(30.5807903085818,617.769931969393,-38.9574260083721)) ;
#60663=CARTESIAN_POINT('Ctrl Pts',(30.6275224364838,617.7672415241,-38.9400672455821)) ;
#60664=CARTESIAN_POINT('Ctrl Pts',(30.7356896889251,617.760786251495,-38.8953477587663)) ;
#60665=CARTESIAN_POINT('Ctrl Pts',(30.7965014227713,617.756977011846,-38.8666377186207)) ;
#60666=CARTESIAN_POINT('Ctrl Pts',(30.985519277444,617.744556563513,-38.7657848103514)) ;
#60667=CARTESIAN_POINT('Ctrl Pts',(31.1074334120279,617.735617258806,-38.6828462819815)) ;
#60668=CARTESIAN_POINT('Ctrl Pts',(31.2748917162738,617.722490179842,-38.5404783517974)) ;
#60669=CARTESIAN_POINT('Ctrl Pts',(31.3278069179047,617.718199385269,-38.4904150521286)) ;
#60670=CARTESIAN_POINT('Ctrl Pts',(31.3994862933326,617.712305016767,-38.4149911634673)) ;
#60671=CARTESIAN_POINT('Ctrl Pts',(31.4204979899222,617.710566447073,-38.3918468073721)) ;
#60672=CARTESIAN_POINT('Ctrl Pts',(31.463600068895,617.706993217141,-38.3421363360367)) ;
#60673=CARTESIAN_POINT('Ctrl Pts',(31.4855644910323,617.705166446979,-38.3154752292432)) ;
#60674=CARTESIAN_POINT('Ctrl Pts',(31.5937264732664,617.696067076666,-38.1772245693299)) ;
#60675=CARTESIAN_POINT('Ctrl Pts',(31.6689541465479,617.689368066327,-38.0575185047584)) ;
#60676=CARTESIAN_POINT('Ctrl Pts',(31.7800214613876,617.677186996813,-37.8323232483487)) ;
#60677=CARTESIAN_POINT('Ctrl Pts',(31.8206949480617,617.671782433778,-37.7298603194332)) ;
#60678=CARTESIAN_POINT('Ctrl Pts',(31.868547838031,617.66336608807,-37.5738320623766)) ;
#60679=CARTESIAN_POINT('Ctrl Pts',(31.8821524409297,617.660567822003,-37.5224414165118)) ;
#60680=CARTESIAN_POINT('Ctrl Pts',(31.9053145869008,617.654846192592,-37.4188670259445)) ;
#60681=CARTESIAN_POINT('Ctrl Pts',(31.9148740395048,617.65192538401,-37.3667257612899)) ;
#60682=CARTESIAN_POINT('Ctrl Pts',(31.9394633157647,617.642186555127,-37.1955212758493)) ;
#60683=CARTESIAN_POINT('Ctrl Pts',(31.9460838023301,617.635111722276,-37.0755161923445)) ;
#60684=CARTESIAN_POINT('Ctrl Pts',(31.9378084543984,617.619782006461,-36.8200534179514)) ;
#60685=CARTESIAN_POINT('Ctrl Pts',(31.9200009801735,617.611529753312,-36.6852345299975)) ;
#60686=CARTESIAN_POINT('Ctrl Pts',(31.8814869554307,617.60191314656,-36.520957650826)) ;
#60687=CARTESIAN_POINT('Ctrl Pts',(31.8731631764905,617.600062235772,-36.4889501979671)) ;
#60688=CARTESIAN_POINT('Ctrl Pts',(31.8551799581335,617.596490641857,-36.4260717544974)) ;
#60689=CARTESIAN_POINT('Ctrl Pts',(31.845557137723,617.594768955087,-36.3952004401708)) ;
#60690=CARTESIAN_POINT('Ctrl Pts',(31.8064878533971,617.588395574146,-36.2795430377554)) ;
#60691=CARTESIAN_POINT('Ctrl Pts',(31.7722239974252,617.583973963416,-36.19648308121)) ;
#60692=CARTESIAN_POINT('Ctrl Pts',(31.6725973313151,617.572986535961,-35.993752053494)) ;
#60693=CARTESIAN_POINT('Ctrl Pts',(31.6005982485012,617.566503602382,-35.8779103629146)) ;
#60694=CARTESIAN_POINT('Ctrl Pts',(31.5177255210691,617.559653386529,-35.7700771955414)) ;
#60695=CARTESIAN_POINT('Ctrl Pts',(31.5177255210752,617.617782467769,-35.7700771955494)) ;
#60696=CARTESIAN_POINT('Ctrl Pts',(31.5180340350894,617.61780717866,-35.7704786309113)) ;
#60697=CARTESIAN_POINT('Ctrl Pts',(31.5183424025187,617.6178318871,-35.7708801826247)) ;
#60698=CARTESIAN_POINT('Ctrl Pts',(31.6277791123126,617.626603994928,-35.913496210444)) ;
#60699=CARTESIAN_POINT('Ctrl Pts',(31.7178211712387,617.635075826489,-36.0693669297009)) ;
#60700=CARTESIAN_POINT('Ctrl Pts',(31.8064719691583,617.64704221832,-36.2831031261027)) ;
#60701=CARTESIAN_POINT('Ctrl Pts',(31.824605112006,617.64979460496,-36.3320013986807)) ;
#60702=CARTESIAN_POINT('Ctrl Pts',(31.8575018699649,617.655494926049,-36.4322553547147)) ;
#60703=CARTESIAN_POINT('Ctrl Pts',(31.8721612338588,617.658443792538,-36.4836026361227)) ;
#60704=CARTESIAN_POINT('Ctrl Pts',(31.9136213921269,617.668321364748,-36.6536576592669)) ;
#60705=CARTESIAN_POINT('Ctrl Pts',(31.9318804715396,617.67551337769,-36.7741664863849)) ;
#60706=CARTESIAN_POINT('Ctrl Pts',(31.9473606350084,617.690595886966,-37.0249490179732)) ;
#60707=CARTESIAN_POINT('Ctrl Pts',(31.9430861333298,617.698466249787,-37.1548032883533)) ;
#60708=CARTESIAN_POINT('Ctrl Pts',(31.9223487291596,617.707777324383,-37.3165908073956)) ;
#60709=CARTESIAN_POINT('Ctrl Pts',(31.9172829720951,617.709653944115,-37.3496807373195)) ;
#60710=CARTESIAN_POINT('Ctrl Pts',(31.9058656688665,617.713213906091,-37.4137515633074)) ;
#60711=CARTESIAN_POINT('Ctrl Pts',(31.8996031592225,617.714900683671,-37.4447379100561)) ;
#60712=CARTESIAN_POINT('Ctrl Pts',(31.8751872213228,617.720690602479,-37.5526582438874)) ;
#60713=CARTESIAN_POINT('Ctrl Pts',(31.8533112900984,617.724618758108,-37.6286846519606)) ;
#60714=CARTESIAN_POINT('Ctrl Pts',(31.7659917248468,617.737495969088,-37.8772151824743)) ;
#60715=CARTESIAN_POINT('Ctrl Pts',(31.6817493213936,617.74618521428,-38.0421334800298)) ;
#60716=CARTESIAN_POINT('Ctrl Pts',(31.5470254037552,617.758416264534,-38.2362773444608)) ;
#60717=CARTESIAN_POINT('Ctrl Pts',(31.5158079386885,617.761160536737,-38.2778088173608)) ;
#60718=CARTESIAN_POINT('Ctrl Pts',(31.4492087337778,617.766869307908,-38.3597518160478)) ;
#60719=CARTESIAN_POINT('Ctrl Pts',(31.4137494187332,617.769835906617,-38.4000479180391)) ;
#60720=CARTESIAN_POINT('Ctrl Pts',(31.3304755612378,617.776657183452,-38.4875232888393)) ;
#60721=CARTESIAN_POINT('Ctrl Pts',(31.2818445737556,617.780544443793,-38.5338378737254)) ;
#60722=CARTESIAN_POINT('Ctrl Pts',(31.1286329000272,617.792476275938,-38.6660685062465)) ;
#60723=CARTESIAN_POINT('Ctrl Pts',(31.0177580551296,617.800726936988,-38.7441158107718)) ;
#60724=CARTESIAN_POINT('Ctrl Pts',(30.8483644354746,617.812257679575,-38.839915099798)) ;
#60725=CARTESIAN_POINT('Ctrl Pts',(30.7954600204953,617.815718687625,-38.8668808714581)) ;
#60726=CARTESIAN_POINT('Ctrl Pts',(30.7142323980204,617.820748628273,-38.9039425083672)) ;
#60727=CARTESIAN_POINT('Ctrl Pts',(30.6867359131042,617.822403573995,-38.9157697089775)) ;
#60728=CARTESIAN_POINT('Ctrl Pts',(30.6249935488472,617.826002520568,-38.9407430068953)) ;
#60729=CARTESIAN_POINT('Ctrl Pts',(30.5906360310009,617.827930192851,-38.9535809690912)) ;
#60730=CARTESIAN_POINT('Ctrl Pts',(30.5128330442322,617.832167248719,-38.9803018334237)) ;
#60731=CARTESIAN_POINT('Ctrl Pts',(30.4692317208715,617.834454358745,-38.993672082564)) ;
#60732=CARTESIAN_POINT('Ctrl Pts',(30.3089052561877,617.842664824357,-39.0370546611192)) ;
#60733=CARTESIAN_POINT('Ctrl Pts',(30.1900458390625,617.848385983677,-39.0582362199247)) ;
#60734=CARTESIAN_POINT('Ctrl Pts',(29.9812567813018,617.858654048457,-39.0767497507778)) ;
#60735=CARTESIAN_POINT('Ctrl Pts',(29.8920914668346,617.863104435427,-39.0788376245131)) ;
#60736=CARTESIAN_POINT('Ctrl Pts',(29.7520591887535,617.870387400234,-39.0730090851948)) ;
#60737=CARTESIAN_POINT('Ctrl Pts',(29.7011416541196,617.87309574215,-39.0689847297956)) ;
#60738=CARTESIAN_POINT('Ctrl Pts',(29.5957084870295,617.87885413864,-39.0566846056944)) ;
#60739=CARTESIAN_POINT('Ctrl Pts',(29.5412704864294,617.881912031968,-39.0481030063165)) ;
#60740=CARTESIAN_POINT('Ctrl Pts',(29.3727972044363,617.891654219457,-39.0145551405766)) ;
#60741=CARTESIAN_POINT('Ctrl Pts',(29.2605111867686,617.898565782613,-38.9820593640228)) ;
#60742=CARTESIAN_POINT('Ctrl Pts',(29.0327082543802,617.913217783146,-38.8945365403378)) ;
#60743=CARTESIAN_POINT('Ctrl Pts',(28.9183125322229,617.920944464703,-38.8378987004513)) ;
#60744=CARTESIAN_POINT('Ctrl Pts',(28.7812622343372,617.930140187678,-38.7533714455176)) ;
#60745=CARTESIAN_POINT('Ctrl Pts',(28.7530672089189,617.932027196406,-38.7350113220697)) ;
#60746=CARTESIAN_POINT('Ctrl Pts',(28.6993872913163,617.935590656082,-38.6981475093762)) ;
#60747=CARTESIAN_POINT('Ctrl Pts',(28.6738526812261,617.937271193357,-38.6797346655057)) ;
#60748=CARTESIAN_POINT('Ctrl Pts',(28.5871926029027,617.942960327631,-38.6141662490702)) ;
#60749=CARTESIAN_POINT('Ctrl Pts',(28.5283026621049,617.946802630882,-38.5641544513786)) ;
#60750=CARTESIAN_POINT('Ctrl Pts',(28.3651729182075,617.957819087282,-38.4089816282746)) ;
#60751=CARTESIAN_POINT('Ctrl Pts',(28.2693112317538,617.964818442891,-38.2957463715584)) ;
#60752=CARTESIAN_POINT('Ctrl Pts',(28.1504925531068,617.975480884393,-38.120044093854)) ;
#60753=CARTESIAN_POINT('Ctrl Pts',(28.1170593858906,617.978776929684,-38.0652393763678)) ;
#60754=CARTESIAN_POINT('Ctrl Pts',(28.0624492446223,617.984787255473,-37.9655003438917)) ;
#60755=CARTESIAN_POINT('Ctrl Pts',(28.0402334305266,617.987460715738,-37.9211934899408)) ;
#60756=CARTESIAN_POINT('Ctrl Pts',(27.9921124174203,617.993842119472,-37.8158821245273)) ;
#60757=CARTESIAN_POINT('Ctrl Pts',(27.9675148339435,617.997592184172,-37.7543443252872)) ;
#60758=CARTESIAN_POINT('Ctrl Pts',(27.9186100081024,618.006282466616,-37.6124590119968)) ;
#60759=CARTESIAN_POINT('Ctrl Pts',(27.8961665822768,618.011267532517,-37.5315948613946)) ;
#60760=CARTESIAN_POINT('Ctrl Pts',(27.8515192470603,618.024146599155,-37.3216612272472)) ;
#60761=CARTESIAN_POINT('Ctrl Pts',(27.8365872739035,618.032089078202,-37.1914189904872)) ;
#60762=CARTESIAN_POINT('Ctrl Pts',(27.8335127814323,618.041457646263,-37.027258609981)) ;
#60763=CARTESIAN_POINT('Ctrl Pts',(27.8337011390787,618.043328702714,-36.9938686816973)) ;
#60764=CARTESIAN_POINT('Ctrl Pts',(27.8356557756322,618.046890095625,-36.928766286273)) ;
#60765=CARTESIAN_POINT('Ctrl Pts',(27.8373436346707,618.048583372588,-36.8970616310105)) ;
#60766=CARTESIAN_POINT('Ctrl Pts',(27.8459430115139,618.054479068767,-36.7846674820529)) ;
#60767=CARTESIAN_POINT('Ctrl Pts',(27.8568885788465,618.058497213992,-36.704355455598)) ;
#60768=CARTESIAN_POINT('Ctrl Pts',(27.9071682153037,618.071198047,-36.4492054111199)) ;
#60769=CARTESIAN_POINT('Ctrl Pts',(27.9646014670271,618.079654419607,-36.2788102552533)) ;
#60770=CARTESIAN_POINT('Ctrl Pts',(28.066479086708,618.091612202793,-36.0709035896473)) ;
#60771=CARTESIAN_POINT('Ctrl Pts',(28.0913585827081,618.094378294162,-36.024697025177)) ;
#60772=CARTESIAN_POINT('Ctrl Pts',(28.1448566010235,618.100067665725,-35.9338519664303)) ;
#60773=CARTESIAN_POINT('Ctrl Pts',(28.1734887009863,618.102990056983,-35.8892682357778)) ;
#60774=CARTESIAN_POINT('Ctrl Pts',(28.2719351544637,618.112681648458,-35.7482734849555)) ;
#60775=CARTESIAN_POINT('Ctrl Pts',(28.3483991152899,618.11970177772,-35.6568192324954)) ;
#60776=CARTESIAN_POINT('Ctrl Pts',(28.5280465940214,618.134976739336,-35.4763616215468)) ;
#60777=CARTESIAN_POINT('Ctrl Pts',(28.6330486402326,618.143231348471,-35.3899291418472)) ;
#60778=CARTESIAN_POINT('Ctrl Pts',(28.7731860236744,618.152843600943,-35.2961544183743)) ;
#60779=CARTESIAN_POINT('Ctrl Pts',(28.8010024513293,618.154688161838,-35.2784939105625)) ;
#60780=CARTESIAN_POINT('Ctrl Pts',(28.856567681903,618.158231014209,-35.2450631377593)) ;
#60781=CARTESIAN_POINT('Ctrl Pts',(28.8842826298613,618.159930958142,-35.2292554409532)) ;
#60782=CARTESIAN_POINT('Ctrl Pts',(28.9865275629576,618.166002003966,-35.1740534260238)) ;
#60783=CARTESIAN_POINT('Ctrl Pts',(29.0631005461686,618.170171579565,-35.138606241793)) ;
#60784=CARTESIAN_POINT('Ctrl Pts',(29.3058957098525,618.182873570332,-35.0438718466805)) ;
#60785=CARTESIAN_POINT('Ctrl Pts',(29.4777021296833,618.191215298445,-35.0011938116259)) ;
#60786=CARTESIAN_POINT('Ctrl Pts',(29.7045357200796,618.203016184373,-34.9750031743947)) ;
#60787=CARTESIAN_POINT('Ctrl Pts',(29.7564278281711,618.205761213353,-34.9710010402733)) ;
#60788=CARTESIAN_POINT('Ctrl Pts',(29.861217999348,618.211423558823,-34.9669121681846)) ;
#60789=CARTESIAN_POINT('Ctrl Pts',(29.9140788300582,618.214340776853,-34.9668897348822)) ;
#60790=CARTESIAN_POINT('Ctrl Pts',(30.0862446390824,618.224056975366,-34.9734594725751)) ;
#60791=CARTESIAN_POINT('Ctrl Pts',(30.204970376356,618.231110943419,-34.9884139630212)) ;
#60792=CARTESIAN_POINT('Ctrl Pts',(30.454214332906,618.246422379792,-35.0421677326057)) ;
#60793=CARTESIAN_POINT('Ctrl Pts',(30.5835714136637,618.254678187611,-35.0837872724778)) ;
#60794=CARTESIAN_POINT('Ctrl Pts',(30.7380873653048,618.26429119596,-35.1509760529953)) ;
#60795=CARTESIAN_POINT('Ctrl Pts',(30.7679653662581,618.266136373358,-35.1648310929445)) ;
#60796=CARTESIAN_POINT('Ctrl Pts',(30.8264487915323,618.269701792271,-35.1936789898314)) ;
#60797=CARTESIAN_POINT('Ctrl Pts',(30.8550595855715,618.271423278598,-35.2086398987449)) ;
#60798=CARTESIAN_POINT('Ctrl Pts',(30.9597720477065,618.277681566113,-35.2665777293345)) ;
#60799=CARTESIAN_POINT('Ctrl Pts',(31.0334669062337,618.282003747505,-35.3137248703129)) ;
#60800=CARTESIAN_POINT('Ctrl Pts',(31.2188041883793,618.293222620977,-35.4496919881979)) ;
#60801=CARTESIAN_POINT('Ctrl Pts',(31.3245872744644,618.300020038451,-35.5456699319762)) ;
#60802=CARTESIAN_POINT('Ctrl Pts',(31.453785607836,618.30983286356,-35.6900213807411)) ;
#60803=CARTESIAN_POINT('Ctrl Pts',(31.4865351379034,618.31247668497,-35.7294894016799)) ;
#60804=CARTESIAN_POINT('Ctrl Pts',(31.5177728528538,618.315179696467,-35.7701387855975)) ;
#60805=CARTESIAN_POINT('Origin',(179.888527625422,620.256490441073,-37.0221601717597)) ;
#60806=CARTESIAN_POINT('Ctrl Pts',(181.517739089186,618.256600448668,-35.7700948504444)) ;
#60807=CARTESIAN_POINT('Ctrl Pts',(181.437873718606,618.249944347976,-35.6661724950447)) ;
#60808=CARTESIAN_POINT('Ctrl Pts',(181.348249767962,618.243721061608,-35.570129746345)) ;
#60809=CARTESIAN_POINT('Ctrl Pts',(181.195083460485,618.233775904554,-35.4346147506586)) ;
#60810=CARTESIAN_POINT('Ctrl Pts',(181.137527457287,618.230168969855,-35.3889464336022)) ;
#60811=CARTESIAN_POINT('Ctrl Pts',(181.02740908538,618.223347923362,-35.3108032938592)) ;
#60812=CARTESIAN_POINT('Ctrl Pts',(180.975590249206,618.220167953579,-35.2774288967524)) ;
#60813=CARTESIAN_POINT('Ctrl Pts',(180.879136016606,618.214246816729,-35.2212733318131)) ;
#60814=CARTESIAN_POINT('Ctrl Pts',(180.835017433914,618.211538046367,-35.1977000263673)) ;
#60815=CARTESIAN_POINT('Ctrl Pts',(180.726321802718,618.204844827544,-35.1446262477408)) ;
#60816=CARTESIAN_POINT('Ctrl Pts',(180.660994372857,618.200804800214,-35.1168186941649)) ;
#60817=CARTESIAN_POINT('Ctrl Pts',(180.458058867961,618.188217198479,-35.0425903292061)) ;
#60818=CARTESIAN_POINT('Ctrl Pts',(180.316859792524,618.179377619175,-35.0073183715969)) ;
#60819=CARTESIAN_POINT('Ctrl Pts',(180.105276350539,618.166643278124,-34.9777253772246)) ;
#60820=CARTESIAN_POINT('Ctrl Pts',(180.036970588114,618.162615853314,-34.9716334337022)) ;
#60821=CARTESIAN_POINT('Ctrl Pts',(179.937609290037,618.156990888051,-34.9677641076903)) ;
#60822=CARTESIAN_POINT('Ctrl Pts',(179.906709234979,618.155274718387,-34.9672582147298)) ;
#60823=CARTESIAN_POINT('Ctrl Pts',(179.840630094085,618.151690790556,-34.9676673477673)) ;
#60824=CARTESIAN_POINT('Ctrl Pts',(179.805463482461,618.149833283473,-34.9687884054165)) ;
#60825=CARTESIAN_POINT('Ctrl Pts',(179.634630225367,618.140978746619,-34.9786308331627)) ;
#60826=CARTESIAN_POINT('Ctrl Pts',(179.500016396077,618.134503612775,-34.9998983833042)) ;
#60827=CARTESIAN_POINT('Ctrl Pts',(179.257342681304,618.122341237677,-35.0633850829905)) ;
#60828=CARTESIAN_POINT('Ctrl Pts',(179.148847608016,618.11670887439,-35.1017267899532)) ;
#60829=CARTESIAN_POINT('Ctrl Pts',(178.995979528623,618.108050729845,-35.1706350433054)) ;
#60830=CARTESIAN_POINT('Ctrl Pts',(178.948684856959,618.105266263961,-35.1941879897356)) ;
#60831=CARTESIAN_POINT('Ctrl Pts',(178.855566939141,618.099538155132,-35.2451306830427)) ;
#60832=CARTESIAN_POINT('Ctrl Pts',(178.809798989781,618.096595426967,-35.2725358238972)) ;
#60833=CARTESIAN_POINT('Ctrl Pts',(178.660690677841,618.086556154298,-35.3698955778976)) ;
#60834=CARTESIAN_POINT('Ctrl Pts',(178.562672736491,618.079177333738,-35.4474656185981)) ;
#60835=CARTESIAN_POINT('Ctrl Pts',(178.39206117652,618.065036370574,-35.6097678900672)) ;
#60836=CARTESIAN_POINT('Ctrl Pts',(178.318117621821,618.058326716948,-35.6924691697643)) ;
#60837=CARTESIAN_POINT('Ctrl Pts',(178.226263122883,618.049502861199,-35.8136165960414)) ;
#60838=CARTESIAN_POINT('Ctrl Pts',(178.202322847058,618.047149847546,-35.8472496264347)) ;
#60839=CARTESIAN_POINT('Ctrl Pts',(178.163153824184,618.043236621683,-35.9059431292964)) ;
#60840=CARTESIAN_POINT('Ctrl Pts',(178.147421604658,618.041647703269,-35.9306450870052)) ;
#60841=CARTESIAN_POINT('Ctrl Pts',(178.106421886834,618.037449095999,-35.9981644481978)) ;
#60842=CARTESIAN_POINT('Ctrl Pts',(178.082171713741,618.034897738397,-36.0415750563872)) ;
#60843=CARTESIAN_POINT('Ctrl Pts',(177.996868291576,618.025492041655,-36.2082043311838)) ;
#60844=CARTESIAN_POINT('Ctrl Pts',(177.94665568358,618.018997394029,-36.3365676894766)) ;
#60845=CARTESIAN_POINT('Ctrl Pts',(177.884915100193,618.007779020365,-36.5574362968693)) ;
#60846=CARTESIAN_POINT('Ctrl Pts',(177.866150899087,618.003201296153,-36.6474316265925)) ;
#60847=CARTESIAN_POINT('Ctrl Pts',(177.846352136007,617.995757740068,-36.7894110523277)) ;
#60848=CARTESIAN_POINT('Ctrl Pts',(177.841158103839,617.993026342084,-36.8406931434261)) ;
#60849=CARTESIAN_POINT('Ctrl Pts',(177.834399433318,617.987235725424,-36.9472666228647)) ;
#60850=CARTESIAN_POINT('Ctrl Pts',(177.833128477895,617.984169388746,-37.0025341873973)) ;
#60851=CARTESIAN_POINT('Ctrl Pts',(177.836799212377,617.972164379123,-37.2142370524895)) ;
#60852=CARTESIAN_POINT('Ctrl Pts',(177.85737511703,617.962745757134,-37.3698509347612)) ;
#60853=CARTESIAN_POINT('Ctrl Pts',(177.910842681946,617.949534056878,-37.5832279587215)) ;
#60854=CARTESIAN_POINT('Ctrl Pts',(177.92913802079,617.945736579996,-37.6441150812566)) ;
#60855=CARTESIAN_POINT('Ctrl Pts',(177.965278909125,617.939377232603,-37.7468457875381)) ;
#60856=CARTESIAN_POINT('Ctrl Pts',(177.981745267152,617.936774790996,-37.7891259613203)) ;
#60857=CARTESIAN_POINT('Ctrl Pts',(178.011067588354,617.932623106229,-37.8576184659271)) ;
#60858=CARTESIAN_POINT('Ctrl Pts',(178.023104254186,617.93103262878,-37.8841593730473)) ;
#60859=CARTESIAN_POINT('Ctrl Pts',(178.055016794302,617.927088698896,-37.9507243446462)) ;
#60860=CARTESIAN_POINT('Ctrl Pts',(178.075640008708,617.924777153273,-37.9903711277945)) ;
#60861=CARTESIAN_POINT('Ctrl Pts',(178.164190357098,617.915626338094,-38.1478367251896)) ;
#60862=CARTESIAN_POINT('Ctrl Pts',(178.242444116224,617.909190339745,-38.259456095989)) ;
#60863=CARTESIAN_POINT('Ctrl Pts',(178.395878966116,617.897729245373,-38.43773123747)) ;
#60864=CARTESIAN_POINT('Ctrl Pts',(178.465957254829,617.89281231411,-38.5081387441332)) ;
#60865=CARTESIAN_POINT('Ctrl Pts',(178.580118574358,617.884978478061,-38.6073323098885)) ;
#60866=CARTESIAN_POINT('Ctrl Pts',(178.620675195722,617.882226948479,-38.6399532712892)) ;
#60867=CARTESIAN_POINT('Ctrl Pts',(178.706046920997,617.876470022482,-38.7034371289031)) ;
#60868=CARTESIAN_POINT('Ctrl Pts',(178.75093685773,617.873461018884,-38.7341295842102)) ;
#60869=CARTESIAN_POINT('Ctrl Pts',(178.937250291898,617.861023947727,-38.8509513511697)) ;
#60870=CARTESIAN_POINT('Ctrl Pts',(179.087610563969,617.85103698966,-38.9216130500305)) ;
#60871=CARTESIAN_POINT('Ctrl Pts',(179.327263755383,617.83589498556,-39.000675757637)) ;
#60872=CARTESIAN_POINT('Ctrl Pts',(179.411394071568,617.830729134247,-39.0226319020823)) ;
#60873=CARTESIAN_POINT('Ctrl Pts',(179.528275146704,617.82396131699,-39.0453389732761)) ;
#60874=CARTESIAN_POINT('Ctrl Pts',(179.56002534863,617.822163787926,-39.0507362494448)) ;
#60875=CARTESIAN_POINT('Ctrl Pts',(179.62480548891,617.81859728985,-39.0601872975185)) ;
#60876=CARTESIAN_POINT('Ctrl Pts',(179.657833049303,617.816831163087,-39.064189610487)) ;
#60877=CARTESIAN_POINT('Ctrl Pts',(179.82387116428,617.808149224599,-39.080229970175)) ;
#60878=CARTESIAN_POINT('Ctrl Pts',(179.957747433404,617.80176492764,-39.0800834622948)) ;
#60879=CARTESIAN_POINT('Ctrl Pts',(180.173234897981,617.791278765631,-39.0587804834641)) ;
#60880=CARTESIAN_POINT('Ctrl Pts',(180.255222823787,617.787241673223,-39.0456260498202)) ;
#60881=CARTESIAN_POINT('Ctrl Pts',(180.400575981089,617.779773145553,-39.0131791288436)) ;
#60882=CARTESIAN_POINT('Ctrl Pts',(180.464229605377,617.776392225983,-38.9957143499616)) ;
#60883=CARTESIAN_POINT('Ctrl Pts',(180.574299998063,617.770280646188,-38.9597353443057)) ;
#60884=CARTESIAN_POINT('Ctrl Pts',(180.621088322488,617.767595627313,-38.9425339680021)) ;
#60885=CARTESIAN_POINT('Ctrl Pts',(180.727670551739,617.761255754453,-38.898887711218)) ;
#60886=CARTESIAN_POINT('Ctrl Pts',(180.786917531223,617.757562060431,-38.8712576097892)) ;
#60887=CARTESIAN_POINT('Ctrl Pts',(180.978456773859,617.745049833906,-38.7705519177621)) ;
#60888=CARTESIAN_POINT('Ctrl Pts',(181.104000237173,617.735864903547,-38.6857215822447)) ;
#60889=CARTESIAN_POINT('Ctrl Pts',(181.274650382973,617.722489422965,-38.5407044179735)) ;
#60890=CARTESIAN_POINT('Ctrl Pts',(181.327659326773,617.718191225634,-38.4905656560473)) ;
#60891=CARTESIAN_POINT('Ctrl Pts',(181.39943471103,617.712289046957,-38.4150474504193)) ;
#60892=CARTESIAN_POINT('Ctrl Pts',(181.420457131513,617.710549601624,-38.391892842992)) ;
#60893=CARTESIAN_POINT('Ctrl Pts',(181.463570710291,617.706975438668,-38.3421713948152)) ;
#60894=CARTESIAN_POINT('Ctrl Pts',(181.485536379775,617.705148581621,-38.3155099691309)) ;
#60895=CARTESIAN_POINT('Ctrl Pts',(181.593725727476,617.696047024736,-38.1772303833297)) ;
#60896=CARTESIAN_POINT('Ctrl Pts',(181.668973288057,617.689346319362,-38.05749084968)) ;
#60897=CARTESIAN_POINT('Ctrl Pts',(181.780046550597,617.677163736028,-37.8322636695395)) ;
#60898=CARTESIAN_POINT('Ctrl Pts',(181.820714272263,617.671759491951,-37.729806412972)) ;
#60899=CARTESIAN_POINT('Ctrl Pts',(181.868564944837,617.663342836343,-37.5737718847934)) ;
#60900=CARTESIAN_POINT('Ctrl Pts',(181.88217107972,617.660543875888,-37.5223684848638)) ;
#60901=CARTESIAN_POINT('Ctrl Pts',(181.905336639262,617.654820230289,-37.4187580074584)) ;
#60902=CARTESIAN_POINT('Ctrl Pts',(181.914897171684,617.651898076025,-37.3665932739173)) ;
#60903=CARTESIAN_POINT('Ctrl Pts',(181.939535636014,617.64213428699,-37.1949527141264)) ;
#60904=CARTESIAN_POINT('Ctrl Pts',(181.946133435778,617.635033634421,-37.07452804646)) ;
#60905=CARTESIAN_POINT('Ctrl Pts',(181.937691298984,617.619716274516,-36.8192952740957)) ;
#60906=CARTESIAN_POINT('Ctrl Pts',(181.919939188561,617.611504833389,-36.6851189235826)) ;
#60907=CARTESIAN_POINT('Ctrl Pts',(181.881597471068,617.601919569737,-36.5213930895733)) ;
#60908=CARTESIAN_POINT('Ctrl Pts',(181.873264142803,617.600064804971,-36.4893221787337)) ;
#60909=CARTESIAN_POINT('Ctrl Pts',(181.855284539896,617.596491511571,-36.4264191375629)) ;
#60910=CARTESIAN_POINT('Ctrl Pts',(181.845679736028,617.59477176136,-36.3955853820921)) ;
#60911=CARTESIAN_POINT('Ctrl Pts',(181.806946761933,617.588448244574,-36.2808415770441)) ;
#60912=CARTESIAN_POINT('Ctrl Pts',(181.773113145488,617.584069505766,-36.1986156242123)) ;
#60913=CARTESIAN_POINT('Ctrl Pts',(181.673742299194,617.573071562562,-35.9955974580883)) ;
#60914=CARTESIAN_POINT('Ctrl Pts',(181.601263946288,617.566541251821,-35.8787790000532)) ;
#60915=CARTESIAN_POINT('Ctrl Pts',(181.517739089189,617.559637408341,-35.7700948504488)) ;
#60916=CARTESIAN_POINT('Ctrl Pts',(181.517739089197,617.617803659368,-35.7700948504595)) ;
#60917=CARTESIAN_POINT('Ctrl Pts',(181.518095630332,617.617832217488,-35.7705587886382)) ;
#60918=CARTESIAN_POINT('Ctrl Pts',(181.518451975681,617.617860772335,-35.7710228822118)) ;
#60919=CARTESIAN_POINT('Ctrl Pts',(181.627854687921,617.626631318891,-35.9136317836402)) ;
#60920=CARTESIAN_POINT('Ctrl Pts',(181.717835755209,617.635098718416,-36.0694147208747)) ;
#60921=CARTESIAN_POINT('Ctrl Pts',(181.806455767298,617.647060039349,-36.2830603899659)) ;
#60922=CARTESIAN_POINT('Ctrl Pts',(181.824593293176,617.649812918917,-36.3319675041867)) ;
#60923=CARTESIAN_POINT('Ctrl Pts',(181.857496237792,617.655514064215,-36.4322360169524)) ;
#60924=CARTESIAN_POINT('Ctrl Pts',(181.872157667491,617.658463251945,-36.4835889102274)) ;
#60925=CARTESIAN_POINT('Ctrl Pts',(181.913623345838,617.668341972707,-36.6536636167769)) ;
#60926=CARTESIAN_POINT('Ctrl Pts',(181.931883817161,617.675534875931,-36.7741869567704)) ;
#60927=CARTESIAN_POINT('Ctrl Pts',(181.947359583335,617.690617298293,-37.0249679291579)) ;
#60928=CARTESIAN_POINT('Ctrl Pts',(181.943084944151,617.698486619465,-37.1548057823885)) ;
#60929=CARTESIAN_POINT('Ctrl Pts',(181.922350183053,617.70779701347,-37.3165812157369)) ;
#60930=CARTESIAN_POINT('Ctrl Pts',(181.917283948896,617.709673857797,-37.3496750927066)) ;
#60931=CARTESIAN_POINT('Ctrl Pts',(181.905865114521,617.713234307245,-37.4137548281389)) ;
#60932=CARTESIAN_POINT('Ctrl Pts',(181.899601512369,617.714921345098,-37.4447461266343)) ;
#60933=CARTESIAN_POINT('Ctrl Pts',(181.875175102307,617.72071353073,-37.5527094656252)) ;
#60934=CARTESIAN_POINT('Ctrl Pts',(181.853285634692,617.724643504571,-37.6287728636373)) ;
#60935=CARTESIAN_POINT('Ctrl Pts',(181.765951233217,617.737520269442,-37.8772949850392)) ;
#60936=CARTESIAN_POINT('Ctrl Pts',(181.681722843776,617.746207733743,-38.0421723956153)) ;
#60937=CARTESIAN_POINT('Ctrl Pts',(181.547016737167,617.758437027098,-38.2362896192365)) ;
#60938=CARTESIAN_POINT('Ctrl Pts',(181.515792733701,617.76118182434,-38.2778289439284)) ;
#60939=CARTESIAN_POINT('Ctrl Pts',(181.449178602575,617.766891745284,-38.3597874225629)) ;
#60940=CARTESIAN_POINT('Ctrl Pts',(181.413710833998,617.769858970664,-38.4000910647036)) ;
#60941=CARTESIAN_POINT('Ctrl Pts',(181.330424375225,617.776681063526,-38.4875737824711)) ;
#60942=CARTESIAN_POINT('Ctrl Pts',(181.281789720238,617.78056848916,-38.5338885539261)) ;
#60943=CARTESIAN_POINT('Ctrl Pts',(181.128524844758,617.792504024189,-38.666155026847)) ;
#60944=CARTESIAN_POINT('Ctrl Pts',(181.017593418918,617.800758404951,-38.7442285517428)) ;
#60945=CARTESIAN_POINT('Ctrl Pts',(180.848194792386,617.81228784728,-38.8400024129723)) ;
#60946=CARTESIAN_POINT('Ctrl Pts',(180.795349973558,617.815744547612,-38.8669327484932)) ;
#60947=CARTESIAN_POINT('Ctrl Pts',(180.714454502399,617.820753601928,-38.9038403353509)) ;
#60948=CARTESIAN_POINT('Ctrl Pts',(180.687233212605,617.822392376592,-38.9155553319779)) ;
#60949=CARTESIAN_POINT('Ctrl Pts',(180.625964320843,617.825965667593,-38.9403662220668)) ;
#60950=CARTESIAN_POINT('Ctrl Pts',(180.591803853648,617.827883621515,-38.9531522047013)) ;
#60951=CARTESIAN_POINT('Ctrl Pts',(180.514572273599,617.832092728787,-38.9797376190929)) ;
#60952=CARTESIAN_POINT('Ctrl Pts',(180.471349262852,617.834362103501,-38.9930383347324)) ;
#60953=CARTESIAN_POINT('Ctrl Pts',(180.313980242041,617.842428209806,-39.0358337325119)) ;
#60954=CARTESIAN_POINT('Ctrl Pts',(180.197787086735,617.848029108326,-39.0569209600502)) ;
#60955=CARTESIAN_POINT('Ctrl Pts',(179.989324054953,617.85827029962,-39.0764751043245)) ;
#60956=CARTESIAN_POINT('Ctrl Pts',(179.897763572593,617.86283109334,-39.0789251444881)) ;
#60957=CARTESIAN_POINT('Ctrl Pts',(179.755136767785,617.870241532697,-39.0732163393845)) ;
#60958=CARTESIAN_POINT('Ctrl Pts',(179.704022034082,617.872957554038,-39.0692511757925)) ;
#60959=CARTESIAN_POINT('Ctrl Pts',(179.598727673481,617.878702809099,-39.057107473486)) ;
#60960=CARTESIAN_POINT('Ctrl Pts',(179.544620161169,617.881738535767,-39.0486648901577)) ;
#60961=CARTESIAN_POINT('Ctrl Pts',(179.425183348615,617.888635827255,-39.0251076829347)) ;
#60962=CARTESIAN_POINT('Ctrl Pts',(179.360127861777,617.892526544909,-39.0089362167855)) ;
#60963=CARTESIAN_POINT('Ctrl Pts',(179.15568788159,617.905138467976,-38.9473644362442)) ;
#60964=CARTESIAN_POINT('Ctrl Pts',(179.020323518093,617.914106625274,-38.8902298605387)) ;
#60965=CARTESIAN_POINT('Ctrl Pts',(178.849011608638,617.925603804225,-38.7952482934308)) ;
#60966=CARTESIAN_POINT('Ctrl Pts',(178.806706640264,617.928452190648,-38.7697582791156)) ;
#60967=CARTESIAN_POINT('Ctrl Pts',(178.740981499184,617.932843638587,-38.726854536905)) ;
#60968=CARTESIAN_POINT('Ctrl Pts',(178.71694539454,617.934440598286,-38.7104256673135)) ;
#60969=CARTESIAN_POINT('Ctrl Pts',(178.660022721154,617.938196261291,-38.669716919506)) ;
#60970=CARTESIAN_POINT('Ctrl Pts',(178.627497185245,617.940324828458,-38.6449572106225)) ;
#60971=CARTESIAN_POINT('Ctrl Pts',(178.509826818459,617.948046921445,-38.5497059906233)) ;
#60972=CARTESIAN_POINT('Ctrl Pts',(178.429667506768,617.953357959992,-38.4733469483095)) ;
#60973=CARTESIAN_POINT('Ctrl Pts',(178.272427868787,617.964781052121,-38.2972962350808)) ;
#60974=CARTESIAN_POINT('Ctrl Pts',(178.197578377633,617.97088958731,-38.1962288902197)) ;
#60975=CARTESIAN_POINT('Ctrl Pts',(178.10484972858,617.980092729238,-38.0435861039979)) ;
#60976=CARTESIAN_POINT('Ctrl Pts',(178.079049440486,617.982886524483,-37.9971503194508)) ;
#60977=CARTESIAN_POINT('Ctrl Pts',(178.031411536465,617.988570269215,-37.9029925202018)) ;
#60978=CARTESIAN_POINT('Ctrl Pts',(178.009545665626,617.991456392188,-37.8553299455452)) ;
#60979=CARTESIAN_POINT('Ctrl Pts',(177.947311039176,618.000620288519,-37.7047250903747)) ;
#60980=CARTESIAN_POINT('Ctrl Pts',(177.913412898147,618.007106835018,-37.5993368503828)) ;
#60981=CARTESIAN_POINT('Ctrl Pts',(177.855407924417,618.022287572548,-37.3522439600267)) ;
#60982=CARTESIAN_POINT('Ctrl Pts',(177.837341483634,618.031034681777,-37.2096951201353)) ;
#60983=CARTESIAN_POINT('Ctrl Pts',(177.833519332619,618.041178766265,-37.0323067071832)) ;
#60984=CARTESIAN_POINT('Ctrl Pts',(177.833634184828,618.043095164956,-36.9981748902709)) ;
#60985=CARTESIAN_POINT('Ctrl Pts',(177.835482181044,618.046674985967,-36.9328458811284)) ;
#60986=CARTESIAN_POINT('Ctrl Pts',(177.837076574522,618.048344116495,-36.9016557064381)) ;
#60987=CARTESIAN_POINT('Ctrl Pts',(177.844823471743,618.053845811982,-36.7969750243422)) ;
#60988=CARTESIAN_POINT('Ctrl Pts',(177.854220836984,618.057528018489,-36.7237765142689)) ;
#60989=CARTESIAN_POINT('Ctrl Pts',(177.894080442057,618.068357128435,-36.5065999790718)) ;
#60990=CARTESIAN_POINT('Ctrl Pts',(177.93607485989,618.075308188106,-36.3652348839258)) ;
#60991=CARTESIAN_POINT('Ctrl Pts',(178.018347766972,618.085996525488,-36.1684556289195)) ;
#60992=CARTESIAN_POINT('Ctrl Pts',(178.046833262195,618.089388001467,-36.1086258958834)) ;
#60993=CARTESIAN_POINT('Ctrl Pts',(178.101571516978,618.095491478451,-36.006662181027)) ;
#60994=CARTESIAN_POINT('Ctrl Pts',(178.126554005481,618.098156361988,-35.963908465536)) ;
#60995=CARTESIAN_POINT('Ctrl Pts',(178.187329449229,618.104399400863,-35.8680280414585)) ;
#60996=CARTESIAN_POINT('Ctrl Pts',(178.224109770048,618.108013341282,-35.8155914268306)) ;
#60997=CARTESIAN_POINT('Ctrl Pts',(178.311505435181,618.116259575137,-35.7026101109687)) ;
#60998=CARTESIAN_POINT('Ctrl Pts',(178.363280506203,618.120928390997,-35.6430913293319)) ;
#60999=CARTESIAN_POINT('Ctrl Pts',(178.51429149906,618.1338774019,-35.4884275239333)) ;
#61000=CARTESIAN_POINT('Ctrl Pts',(178.619854154395,618.142250560222,-35.4000222785229)) ;
#61001=CARTESIAN_POINT('Ctrl Pts',(178.762315899289,618.152122669112,-35.3031887229354)) ;
#61002=CARTESIAN_POINT('Ctrl Pts',(178.79167809621,618.154087433079,-35.2843059970602)) ;
#61003=CARTESIAN_POINT('Ctrl Pts',(178.847667853496,618.157683606821,-35.2502839214104)) ;
#61004=CARTESIAN_POINT('Ctrl Pts',(178.874178700074,618.159323929544,-35.234975002494)) ;
#61005=CARTESIAN_POINT('Ctrl Pts',(178.959724829872,618.16444980428,-35.1880925940932)) ;
#61006=CARTESIAN_POINT('Ctrl Pts',(179.019969480134,618.167813730566,-35.1588065362308)) ;
#61007=CARTESIAN_POINT('Ctrl Pts',(179.207962434688,618.177887125873,-35.078522918502)) ;
#61008=CARTESIAN_POINT('Ctrl Pts',(179.339482349915,618.184384509566,-35.0373564701003)) ;
#61009=CARTESIAN_POINT('Ctrl Pts',(179.547903589878,618.194925984724,-34.9944407611673)) ;
#61010=CARTESIAN_POINT('Ctrl Pts',(179.622449604035,618.198737527365,-34.9833194004161)) ;
#61011=CARTESIAN_POINT('Ctrl Pts',(179.746970597257,618.205282495372,-34.9716883961272)) ;
#61012=CARTESIAN_POINT('Ctrl Pts',(179.796656018017,618.207939844539,-34.968862358626)) ;
#61013=CARTESIAN_POINT('Ctrl Pts',(179.90441661017,618.213824090264,-34.9666521229542)) ;
#61014=CARTESIAN_POINT('Ctrl Pts',(179.962460511373,618.217069714695,-34.9679209561088)) ;
#61015=CARTESIAN_POINT('Ctrl Pts',(180.086747750104,618.224189448023,-34.9759122177706)) ;
#61016=CARTESIAN_POINT('Ctrl Pts',(180.152875020548,618.228082282332,-34.9834004601559)) ;
#61017=CARTESIAN_POINT('Ctrl Pts',(180.353461336179,618.240157507464,-35.0160380716334)) ;
#61018=CARTESIAN_POINT('Ctrl Pts',(180.485870393457,618.2485227758,-35.0514066279319)) ;
#61019=CARTESIAN_POINT('Ctrl Pts',(180.660296817167,618.259483124503,-35.1172084034319)) ;
#61020=CARTESIAN_POINT('Ctrl Pts',(180.706161606558,618.262355662103,-35.1364389914603)) ;
#61021=CARTESIAN_POINT('Ctrl Pts',(180.777776895497,618.266775942372,-35.1695713839637)) ;
#61022=CARTESIAN_POINT('Ctrl Pts',(180.804002672154,618.268378666778,-35.1823897484777)) ;
#61023=CARTESIAN_POINT('Ctrl Pts',(180.866487035888,618.272155884006,-35.2145975842519)) ;
#61024=CARTESIAN_POINT('Ctrl Pts',(180.902452338712,618.274299968275,-35.2345236712379)) ;
#61025=CARTESIAN_POINT('Ctrl Pts',(181.033539577708,618.28209016693,-35.3123808916821)) ;
#61026=CARTESIAN_POINT('Ctrl Pts',(181.124507528037,618.287454254803,-35.3769383077405)) ;
#61027=CARTESIAN_POINT('Ctrl Pts',(181.284059731833,618.297571184532,-35.5109057772926)) ;
#61028=CARTESIAN_POINT('Ctrl Pts',(181.35380900263,618.302300739728,-35.5784328434861)) ;
#61029=CARTESIAN_POINT('Ctrl Pts',(181.453109681435,618.309836560498,-35.6892067446014)) ;
#61030=CARTESIAN_POINT('Ctrl Pts',(181.486218887169,618.312508604253,-35.7290770797887)) ;
#61031=CARTESIAN_POINT('Ctrl Pts',(181.517784450449,618.315241095141,-35.7701538776056)) ;
#61032=CARTESIAN_POINT('Origin',(179.888527625402,504.710565160536,-37.0221601717597)) ;
#61033=CARTESIAN_POINT('Ctrl Pts',(180.464073435314,504.369601015799,-35.4587334799406)) ;
#61034=CARTESIAN_POINT('Ctrl Pts',(180.481858241129,504.370836174127,-35.4652806180445)) ;
#61035=CARTESIAN_POINT('Ctrl Pts',(180.499530337435,504.372086174135,-35.4721308578578)) ;
#61036=CARTESIAN_POINT('Ctrl Pts',(180.546347805476,504.375468445644,-35.4912038536254)) ;
#61037=CARTESIAN_POINT('Ctrl Pts',(180.575263684777,504.377634369866,-35.5039547808052)) ;
#61038=CARTESIAN_POINT('Ctrl Pts',(180.708421118899,504.387918732243,-35.5672543707548)) ;
#61039=CARTESIAN_POINT('Ctrl Pts',(180.807566701039,504.396452987282,-35.6277640822013)) ;
#61040=CARTESIAN_POINT('Ctrl Pts',(180.95338416137,504.409757351566,-35.739112506369)) ;
#61041=CARTESIAN_POINT('Ctrl Pts',(181.004595257379,504.414609923142,-35.7834005229483)) ;
#61042=CARTESIAN_POINT('Ctrl Pts',(181.093974244796,504.423370154077,-35.8707520135229)) ;
#61043=CARTESIAN_POINT('Ctrl Pts',(181.13288079304,504.427303966535,-35.9129131777258)) ;
#61044=CARTESIAN_POINT('Ctrl Pts',(181.202279033618,504.434576227059,-35.9963749455418)) ;
#61045=CARTESIAN_POINT('Ctrl Pts',(181.233187769377,504.43792975164,-36.0372398000582)) ;
#61046=CARTESIAN_POINT('Ctrl Pts',(181.341488947989,504.450217569608,-36.1950503917734)) ;
#61047=CARTESIAN_POINT('Ctrl Pts',(181.405904049199,504.458622768934,-36.320178246905)) ;
#61048=CARTESIAN_POINT('Ctrl Pts',(181.471385110967,504.470370578089,-36.4999242282575)) ;
#61049=CARTESIAN_POINT('Ctrl Pts',(181.486659222833,504.473536874829,-36.5487228939999)) ;
#61050=CARTESIAN_POINT('Ctrl Pts',(181.509395675403,504.479221744144,-36.6351144775146)) ;
#61051=CARTESIAN_POINT('Ctrl Pts',(181.517849434592,504.481701029314,-36.672406748695)) ;
#61052=CARTESIAN_POINT('Ctrl Pts',(181.530814044339,504.486318972039,-36.7403628224682)) ;
#61053=CARTESIAN_POINT('Ctrl Pts',(181.535765828239,504.488435009197,-36.7709230099683)) ;
#61054=CARTESIAN_POINT('Ctrl Pts',(181.556072539052,504.499108764789,-36.922958848566)) ;
#61055=CARTESIAN_POINT('Ctrl Pts',(181.55885349808,504.50814735064,-37.0457273969157)) ;
#61056=CARTESIAN_POINT('Ctrl Pts',(181.542418390989,504.521774856124,-37.2331613357748)) ;
#61057=CARTESIAN_POINT('Ctrl Pts',(181.532806844696,504.526481007609,-37.2982463718979)) ;
#61058=CARTESIAN_POINT('Ctrl Pts',(181.507828654272,504.535034705643,-37.417902391721)) ;
#61059=CARTESIAN_POINT('Ctrl Pts',(181.493477503475,504.538905065808,-37.4725877020964)) ;
#61060=CARTESIAN_POINT('Ctrl Pts',(181.46077419599,504.546133880742,-37.5755610408141)) ;
#61061=CARTESIAN_POINT('Ctrl Pts',(181.44290338083,504.549503718074,-37.6239315340321)) ;
#61062=CARTESIAN_POINT('Ctrl Pts',(181.370329768133,504.5614416565,-37.7954380240948)) ;
#61063=CARTESIAN_POINT('Ctrl Pts',(181.302997205377,504.569536499776,-37.912651528029)) ;
#61064=CARTESIAN_POINT('Ctrl Pts',(181.190523936661,504.58104808268,-38.0629149270111)) ;
#61065=CARTESIAN_POINT('Ctrl Pts',(181.15676089823,504.584324373238,-38.1038017167691)) ;
#61066=CARTESIAN_POINT('Ctrl Pts',(181.094822590378,504.590172986603,-38.171914542327)) ;
#61067=CARTESIAN_POINT('Ctrl Pts',(181.067529369425,504.592702526645,-38.1998854886461)) ;
#61068=CARTESIAN_POINT('Ctrl Pts',(181.017108761082,504.597351103467,-38.2480479364742)) ;
#61069=CARTESIAN_POINT('Ctrl Pts',(180.994360096597,504.599443801643,-38.2686071725116)) ;
#61070=CARTESIAN_POINT('Ctrl Pts',(180.885948072353,504.609356063916,-38.3612815766562)) ;
#61071=CARTESIAN_POINT('Ctrl Pts',(180.793724748195,504.617585414284,-38.4252667992938)) ;
#61072=CARTESIAN_POINT('Ctrl Pts',(180.633707227214,504.630873282899,-38.5139042103486)) ;
#61073=CARTESIAN_POINT('Ctrl Pts',(180.56948495682,504.63598161717,-38.5442941518347)) ;
#61074=CARTESIAN_POINT('Ctrl Pts',(180.448924593769,504.64509910191,-38.592179724118)) ;
#61075=CARTESIAN_POINT('Ctrl Pts',(180.39322136868,504.649140498909,-38.6109621989148)) ;
#61076=CARTESIAN_POINT('Ctrl Pts',(180.288319456093,504.656453056308,-38.6402575138159)) ;
#61077=CARTESIAN_POINT('Ctrl Pts',(180.239414745928,504.65974712157,-38.6515624075983)) ;
#61078=CARTESIAN_POINT('Ctrl Pts',(180.09725129968,504.669053355141,-38.6777257711572)) ;
#61079=CARTESIAN_POINT('Ctrl Pts',(180.003144542073,504.674876422941,-38.686891098083)) ;
#61080=CARTESIAN_POINT('Ctrl Pts',(179.803910120013,504.687059372146,-38.6893106208155)) ;
#61081=CARTESIAN_POINT('Ctrl Pts',(179.699187324155,504.693381278864,-38.6806825099998)) ;
#61082=CARTESIAN_POINT('Ctrl Pts',(179.560424373139,504.702392689467,-38.6559315350542)) ;
#61083=CARTESIAN_POINT('Ctrl Pts',(179.525085339673,504.704745823462,-38.6484349945293)) ;
#61084=CARTESIAN_POINT('Ctrl Pts',(179.45898303548,504.709305781391,-38.6321506353186)) ;
#61085=CARTESIAN_POINT('Ctrl Pts',(179.428175899254,504.711499665684,-38.6236137411598)) ;
#61086=CARTESIAN_POINT('Ctrl Pts',(179.361135219858,504.716399139524,-38.6029423705984)) ;
#61087=CARTESIAN_POINT('Ctrl Pts',(179.325033208504,504.719119312238,-38.5904358887148)) ;
#61088=CARTESIAN_POINT('Ctrl Pts',(179.20510232603,504.728367376382,-38.5442136059551)) ;
#61089=CARTESIAN_POINT('Ctrl Pts',(179.123591223014,504.734999929496,-38.5049243036887)) ;
#61090=CARTESIAN_POINT('Ctrl Pts',(178.973786538971,504.747537859219,-38.4170611779224)) ;
#61091=CARTESIAN_POINT('Ctrl Pts',(178.905162392707,504.753443039656,-38.3695638406436)) ;
#61092=CARTESIAN_POINT('Ctrl Pts',(178.801228055316,504.762609901532,-38.2854383732187)) ;
#61093=CARTESIAN_POINT('Ctrl Pts',(178.763537028124,504.765990143768,-38.2519932022954)) ;
#61094=CARTESIAN_POINT('Ctrl Pts',(178.684049726041,504.773275459142,-38.1747424229036)) ;
#61095=CARTESIAN_POINT('Ctrl Pts',(178.643007357345,504.777143540881,-38.1302637216515)) ;
#61096=CARTESIAN_POINT('Ctrl Pts',(178.495864022097,504.791632256073,-37.9522676721351)) ;
#61097=CARTESIAN_POINT('Ctrl Pts',(178.408082403847,504.801558392518,-37.8050249291368)) ;
#61098=CARTESIAN_POINT('Ctrl Pts',(178.331650789944,504.814679505556,-37.6161327611039)) ;
#61099=CARTESIAN_POINT('Ctrl Pts',(178.320070429599,504.816868296652,-37.5848417560817)) ;
#61100=CARTESIAN_POINT('Ctrl Pts',(178.298541512778,504.821417232173,-37.5208270475406)) ;
#61101=CARTESIAN_POINT('Ctrl Pts',(178.288645824104,504.823778477856,-37.4881024983474)) ;
#61102=CARTESIAN_POINT('Ctrl Pts',(178.25282757581,504.833462184719,-37.3550053630662)) ;
#61103=CARTESIAN_POINT('Ctrl Pts',(178.235292629288,504.841076982294,-37.2526213268534)) ;
#61104=CARTESIAN_POINT('Ctrl Pts',(178.219768308788,504.855851642582,-37.0497541533174)) ;
#61105=CARTESIAN_POINT('Ctrl Pts',(178.221110629713,504.862987234671,-36.9497326292546)) ;
#61106=CARTESIAN_POINT('Ctrl Pts',(178.236577142803,504.873295703593,-36.800497027016)) ;
#61107=CARTESIAN_POINT('Ctrl Pts',(178.244004565297,504.876672748673,-36.7508304797807)) ;
#61108=CARTESIAN_POINT('Ctrl Pts',(178.264939968442,504.883841173954,-36.6440694655757)) ;
#61109=CARTESIAN_POINT('Ctrl Pts',(178.279242130992,504.887601676615,-36.5871993360155)) ;
#61110=CARTESIAN_POINT('Ctrl Pts',(178.31733388124,504.895736764827,-36.4636820923205)) ;
#61111=CARTESIAN_POINT('Ctrl Pts',(178.342428995667,504.900069186051,-36.3975582380914)) ;
#61112=CARTESIAN_POINT('Ctrl Pts',(178.418298193856,504.911276768654,-36.230511463264)) ;
#61113=CARTESIAN_POINT('Ctrl Pts',(178.475253640498,504.918090076071,-36.1328168640231)) ;
#61114=CARTESIAN_POINT('Ctrl Pts',(178.559638748932,504.927418211188,-36.0169006278278)) ;
#61115=CARTESIAN_POINT('Ctrl Pts',(178.578323145101,504.929447466619,-35.9926668476939)) ;
#61116=CARTESIAN_POINT('Ctrl Pts',(178.622485743589,504.934192868097,-35.9385388064811)) ;
#61117=CARTESIAN_POINT('Ctrl Pts',(178.648369637508,504.936932630799,-35.9090093099107)) ;
#61118=CARTESIAN_POINT('Ctrl Pts',(178.711879488288,504.943506582762,-35.8415209538879)) ;
#61119=CARTESIAN_POINT('Ctrl Pts',(178.750337606184,504.947374659445,-35.8044029719168)) ;
#61120=CARTESIAN_POINT('Ctrl Pts',(178.890976691694,504.960975631911,-35.6811555490257)) ;
#61121=CARTESIAN_POINT('Ctrl Pts',(179.001689524252,504.970700730576,-35.6054978313398)) ;
#61122=CARTESIAN_POINT('Ctrl Pts',(179.16608245433,504.983486431906,-35.52006329648)) ;
#61123=CARTESIAN_POINT('Ctrl Pts',(179.212984515209,504.986975423506,-35.4983935918746)) ;
#61124=CARTESIAN_POINT('Ctrl Pts',(179.313032025306,504.994117532734,-35.4576993606721)) ;
#61125=CARTESIAN_POINT('Ctrl Pts',(179.366289628779,504.997751507513,-35.4391246524085)) ;
#61126=CARTESIAN_POINT('Ctrl Pts',(179.48317199108,505.005451058986,-35.4049026082535)) ;
#61127=CARTESIAN_POINT('Ctrl Pts',(179.546983568035,505.009484837401,-35.390233749576)) ;
#61128=CARTESIAN_POINT('Ctrl Pts',(179.733261232255,505.021048411961,-35.3588211267165)) ;
#61129=CARTESIAN_POINT('Ctrl Pts',(179.856913734484,505.028451606098,-35.3518919182735)) ;
#61130=CARTESIAN_POINT('Ctrl Pts',(180.011004067251,505.038479399329,-35.3603813560293)) ;
#61131=CARTESIAN_POINT('Ctrl Pts',(180.04177803009,505.040524403632,-35.3629364047818)) ;
#61132=CARTESIAN_POINT('Ctrl Pts',(180.110841560923,505.045239624819,-35.3706082979794)) ;
#61133=CARTESIAN_POINT('Ctrl Pts',(180.149056365601,505.047930843947,-35.3762041444531)) ;
#61134=CARTESIAN_POINT('Ctrl Pts',(180.281390474302,505.057460813301,-35.4003055456713)) ;
#61135=CARTESIAN_POINT('Ctrl Pts',(180.374077836177,505.064499610795,-35.4256035430713)) ;
#61136=CARTESIAN_POINT('Ctrl Pts',(180.464069889026,505.071458111631,-35.4587321744464)) ;
#61137=CARTESIAN_POINT('Ctrl Pts',(180.464073435749,504.178966917533,-35.4587334801008)) ;
#61138=CARTESIAN_POINT('Ctrl Pts',(180.464397541983,504.178987991548,-35.4588527936485)) ;
#61139=CARTESIAN_POINT('Ctrl Pts',(180.464721613219,504.179009065212,-35.4589722087537)) ;
#61140=CARTESIAN_POINT('Ctrl Pts',(180.542007893517,504.184035291354,-35.4874782755891)) ;
#61141=CARTESIAN_POINT('Ctrl Pts',(180.616766377915,504.189013538016,-35.5215095031763)) ;
#61142=CARTESIAN_POINT('Ctrl Pts',(180.744111715052,504.198079427466,-35.5912438595097)) ;
#61143=CARTESIAN_POINT('Ctrl Pts',(180.797736273365,504.202099652675,-35.6247039981196)) ;
#61144=CARTESIAN_POINT('Ctrl Pts',(180.890184944929,504.20951228652,-35.6899665679881)) ;
#61145=CARTESIAN_POINT('Ctrl Pts',(180.929718254343,504.212856745465,-35.7206309484186)) ;
#61146=CARTESIAN_POINT('Ctrl Pts',(181.031217494982,504.221960738824,-35.8069465722094)) ;
#61147=CARTESIAN_POINT('Ctrl Pts',(181.09048547241,504.22784103648,-35.8655367559403)) ;
#61148=CARTESIAN_POINT('Ctrl Pts',(181.206383767911,504.240565513492,-35.9986773236304)) ;
#61149=CARTESIAN_POINT('Ctrl Pts',(181.261623646416,504.247419689051,-36.0740733575443)) ;
#61150=CARTESIAN_POINT('Ctrl Pts',(181.33044396571,504.256925330051,-36.1867367240614)) ;
#61151=CARTESIAN_POINT('Ctrl Pts',(181.349470664175,504.259685073744,-36.2204738574176)) ;
#61152=CARTESIAN_POINT('Ctrl Pts',(181.382160963986,504.264645208874,-36.283475009766)) ;
#61153=CARTESIAN_POINT('Ctrl Pts',(181.39618383512,504.266860849097,-36.3125337374002)) ;
#61154=CARTESIAN_POINT('Ctrl Pts',(181.424081059909,504.271439445078,-36.3749102183598)) ;
#61155=CARTESIAN_POINT('Ctrl Pts',(181.437734619378,504.273790409771,-36.4083075344695)) ;
#61156=CARTESIAN_POINT('Ctrl Pts',(181.506556796633,504.286431058303,-36.5936138726663)) ;
#61157=CARTESIAN_POINT('Ctrl Pts',(181.540485136173,504.295886806324,-36.7524949464847)) ;
#61158=CARTESIAN_POINT('Ctrl Pts',(181.55502809248,504.309883907322,-36.9755956979436)) ;
#61159=CARTESIAN_POINT('Ctrl Pts',(181.555606853691,504.313836537297,-37.0375701003839)) ;
#61160=CARTESIAN_POINT('Ctrl Pts',(181.550393409002,504.321214382679,-37.1498584706652)) ;
#61161=CARTESIAN_POINT('Ctrl Pts',(181.545761145486,504.324597636104,-37.2001512812365)) ;
#61162=CARTESIAN_POINT('Ctrl Pts',(181.518277621417,504.338348576201,-37.3990917244728)) ;
#61163=CARTESIAN_POINT('Ctrl Pts',(181.477636852574,504.349311778951,-37.5445347395339)) ;
#61164=CARTESIAN_POINT('Ctrl Pts',(181.398355636548,504.363835546107,-37.7281687492511)) ;
#61165=CARTESIAN_POINT('Ctrl Pts',(181.376609984472,504.367424777227,-37.7729199624627)) ;
#61166=CARTESIAN_POINT('Ctrl Pts',(181.334940390606,504.373603875988,-37.8497249432087)) ;
#61167=CARTESIAN_POINT('Ctrl Pts',(181.315868805024,504.376222749187,-37.8822014920658)) ;
#61168=CARTESIAN_POINT('Ctrl Pts',(181.27879310803,504.38091367585,-37.9407006800149)) ;
#61169=CARTESIAN_POINT('Ctrl Pts',(181.261118668403,504.383001687648,-37.966908152936)) ;
#61170=CARTESIAN_POINT('Ctrl Pts',(181.17440346602,504.392650976523,-38.0879133588464)) ;
#61171=CARTESIAN_POINT('Ctrl Pts',(181.096216522383,504.399705139639,-38.1757639646798)) ;
#61172=CARTESIAN_POINT('Ctrl Pts',(180.95958800213,504.411000265744,-38.3000202866712)) ;
#61173=CARTESIAN_POINT('Ctrl Pts',(180.907033714774,504.41514676577,-38.3422893903067)) ;
#61174=CARTESIAN_POINT('Ctrl Pts',(180.805275970627,504.423020531029,-38.4144311223862)) ;
#61175=CARTESIAN_POINT('Ctrl Pts',(180.75680742599,504.426712462012,-38.4451622452122)) ;
#61176=CARTESIAN_POINT('Ctrl Pts',(180.661807857348,504.433917033347,-38.4987333038483)) ;
#61177=CARTESIAN_POINT('Ctrl Pts',(180.615607305877,504.437407378656,-38.5220217087054)) ;
#61178=CARTESIAN_POINT('Ctrl Pts',(180.443722488701,504.450389216829,-38.5988548089519)) ;
#61179=CARTESIAN_POINT('Ctrl Pts',(180.312681905936,504.460334784631,-38.6390358048322)) ;
#61180=CARTESIAN_POINT('Ctrl Pts',(180.126490967855,504.47408234086,-38.6719150463779)) ;
#61181=CARTESIAN_POINT('Ctrl Pts',(180.074333077924,504.477885165741,-38.6786005447031)) ;
#61182=CARTESIAN_POINT('Ctrl Pts',(179.983144057023,504.484369812791,-38.6859266367473)) ;
#61183=CARTESIAN_POINT('Ctrl Pts',(179.944243066473,504.48708437079,-38.6876833726016)) ;
#61184=CARTESIAN_POINT('Ctrl Pts',(179.874292763182,504.491832202552,-38.6883881544817)) ;
#61185=CARTESIAN_POINT('Ctrl Pts',(179.843270351526,504.493887127312,-38.6878342748889)) ;
#61186=CARTESIAN_POINT('Ctrl Pts',(179.703842866005,504.502956098488,-38.6814463918579)) ;
#61187=CARTESIAN_POINT('Ctrl Pts',(179.59613540767,504.509528829693,-38.6658914873721)) ;
#61188=CARTESIAN_POINT('Ctrl Pts',(179.420462885489,504.520576584962,-38.6226920564744)) ;
#61189=CARTESIAN_POINT('Ctrl Pts',(179.351432812034,504.525004994953,-38.6008669429078)) ;
#61190=CARTESIAN_POINT('Ctrl Pts',(179.228664767574,504.533288239,-38.5530647086376)) ;
#61191=CARTESIAN_POINT('Ctrl Pts',(179.174486032451,504.537097696241,-38.5285568600258)) ;
#61192=CARTESIAN_POINT('Ctrl Pts',(179.076978581403,504.544330184364,-38.4780055800623)) ;
#61193=CARTESIAN_POINT('Ctrl Pts',(179.033301757414,504.54772004277,-38.4527843209506)) ;
#61194=CARTESIAN_POINT('Ctrl Pts',(178.912002547721,504.557609319271,-38.375198508149)) ;
#61195=CARTESIAN_POINT('Ctrl Pts',(178.837567588632,504.564277771763,-38.3182280124686)) ;
#61196=CARTESIAN_POINT('Ctrl Pts',(178.690540302175,504.578677649443,-38.1846676287889)) ;
#61197=CARTESIAN_POINT('Ctrl Pts',(178.619619798217,504.586408943609,-38.1068129682312)) ;
#61198=CARTESIAN_POINT('Ctrl Pts',(178.534475663348,504.596417829104,-37.9934708275068)) ;
#61199=CARTESIAN_POINT('Ctrl Pts',(178.513419489688,504.598964773972,-37.9634248877142)) ;
#61200=CARTESIAN_POINT('Ctrl Pts',(178.475880213643,504.603610417177,-37.9059063941441)) ;
#61201=CARTESIAN_POINT('Ctrl Pts',(178.459165135602,504.605721025403,-37.8786081533552)) ;
#61202=CARTESIAN_POINT('Ctrl Pts',(178.386961736296,504.615114106342,-37.7526804414239)) ;
#61203=CARTESIAN_POINT('Ctrl Pts',(178.340817151707,504.621933938469,-37.6490247083484)) ;
#61204=CARTESIAN_POINT('Ctrl Pts',(178.284137746364,504.633047924257,-37.4762540826236)) ;
#61205=CARTESIAN_POINT('Ctrl Pts',(178.266792826746,504.637265865347,-37.4097726105492)) ;
#61206=CARTESIAN_POINT('Ctrl Pts',(178.242469212816,504.645243797963,-37.2855983544642)) ;
#61207=CARTESIAN_POINT('Ctrl Pts',(178.234310246879,504.648965943941,-37.2282465556806)) ;
#61208=CARTESIAN_POINT('Ctrl Pts',(178.2245658586,504.656184142796,-37.1193098536697)) ;
#61209=CARTESIAN_POINT('Ctrl Pts',(178.222358868817,504.659655386995,-37.0678490207687)) ;
#61210=CARTESIAN_POINT('Ctrl Pts',(178.22302421881,504.672848961248,-36.8763052320636)) ;
#61211=CARTESIAN_POINT('Ctrl Pts',(178.241173435281,504.683057876188,-36.7368801978048)) ;
#61212=CARTESIAN_POINT('Ctrl Pts',(178.289492096273,504.696961405301,-36.5517631179949)) ;
#61213=CARTESIAN_POINT('Ctrl Pts',(178.304735847762,504.700669898913,-36.5027448502892)) ;
#61214=CARTESIAN_POINT('Ctrl Pts',(178.335290740104,504.707020036296,-36.4184358237774)) ;
#61215=CARTESIAN_POINT('Ctrl Pts',(178.349606417897,504.709692759533,-36.3828245552561)) ;
#61216=CARTESIAN_POINT('Ctrl Pts',(178.377783719757,504.714412846952,-36.3191777561543)) ;
#61217=CARTESIAN_POINT('Ctrl Pts',(178.391227475442,504.716479468642,-36.2909804335926)) ;
#61218=CARTESIAN_POINT('Ctrl Pts',(178.453430439315,504.725342171005,-36.1694345175893)) ;
#61219=CARTESIAN_POINT('Ctrl Pts',(178.510190745571,504.731728824381,-36.0804391382631)) ;
#61220=CARTESIAN_POINT('Ctrl Pts',(178.620236259792,504.742651695549,-35.9393833058967)) ;
#61221=CARTESIAN_POINT('Ctrl Pts',(178.669281124357,504.747151170526,-35.8844406563264)) ;
#61222=CARTESIAN_POINT('Ctrl Pts',(178.764584924159,504.75553769545,-35.7909403012174)) ;
#61223=CARTESIAN_POINT('Ctrl Pts',(178.8096062676,504.759376751538,-35.7513034015851)) ;
#61224=CARTESIAN_POINT('Ctrl Pts',(178.896607173533,504.766668763896,-35.6826682676852)) ;
#61225=CARTESIAN_POINT('Ctrl Pts',(178.937971197453,504.770088021529,-35.6530048726729)) ;
#61226=CARTESIAN_POINT('Ctrl Pts',(179.05693685158,504.779829784863,-35.5756828560351)) ;
#61227=CARTESIAN_POINT('Ctrl Pts',(179.137173942613,504.786306529392,-35.5324277339193)) ;
#61228=CARTESIAN_POINT('Ctrl Pts',(179.297212372072,504.798959401514,-35.4623816376404)) ;
#61229=CARTESIAN_POINT('Ctrl Pts',(179.376315704695,504.805097940736,-35.4346457977434)) ;
#61230=CARTESIAN_POINT('Ctrl Pts',(179.505610781237,504.814714457185,-35.3999869536163)) ;
#61231=CARTESIAN_POINT('Ctrl Pts',(179.554620108505,504.818265938231,-35.3891941194007)) ;
#61232=CARTESIAN_POINT('Ctrl Pts',(179.633179014945,504.823738140319,-35.3755796941561)) ;
#61233=CARTESIAN_POINT('Ctrl Pts',(179.662438845217,504.825725098908,-35.3713075567878)) ;
#61234=CARTESIAN_POINT('Ctrl Pts',(179.744420682284,504.831157517958,-35.3615588122423)) ;
#61235=CARTESIAN_POINT('Ctrl Pts',(179.797312268705,504.8345175028,-35.3578150417454)) ;
#61236=CARTESIAN_POINT('Ctrl Pts',(179.961213487743,504.844728458033,-35.3540530046583)) ;
#61237=CARTESIAN_POINT('Ctrl Pts',(180.072108380191,504.851369896765,-35.362592520638)) ;
#61238=CARTESIAN_POINT('Ctrl Pts',(180.252392080602,504.862705117642,-35.3947792286458)) ;
#61239=CARTESIAN_POINT('Ctrl Pts',(180.322541431123,504.867251806807,-35.4120682142025)) ;
#61240=CARTESIAN_POINT('Ctrl Pts',(180.415779168701,504.873616399834,-35.4415847181096)) ;
#61241=CARTESIAN_POINT('Ctrl Pts',(180.440028900372,504.87530171097,-35.4498819413305)) ;
#61242=CARTESIAN_POINT('Ctrl Pts',(180.464073449582,504.877005588434,-35.458733485193)) ;
#61243=CARTESIAN_POINT('Origin',(29.888527625402,504.710565160562,-37.0221601717529)) ;
#61244=CARTESIAN_POINT('Ctrl Pts',(30.4640904795472,504.369620557053,-35.4587397545496)) ;
#61245=CARTESIAN_POINT('Ctrl Pts',(30.4818072267917,504.370851028822,-35.4652620575066)) ;
#61246=CARTESIAN_POINT('Ctrl Pts',(30.4994121352201,504.372096230735,-35.4720851531116)) ;
#61247=CARTESIAN_POINT('Ctrl Pts',(30.5461349865861,504.375471236898,-35.4911130913441)) ;
#61248=CARTESIAN_POINT('Ctrl Pts',(30.5750232638434,504.377634739377,-35.503846723006)) ;
#61249=CARTESIAN_POINT('Ctrl Pts',(30.7084207921841,504.387935871951,-35.56723141876)) ;
#61250=CARTESIAN_POINT('Ctrl Pts',(30.807807336918,504.396492032086,-35.6278989566728)) ;
#61251=CARTESIAN_POINT('Ctrl Pts',(30.9537451828525,504.409810285808,-35.7394168085837)) ;
#61252=CARTESIAN_POINT('Ctrl Pts',(31.0048788466309,504.414656247058,-35.7836608378205)) ;
#61253=CARTESIAN_POINT('Ctrl Pts',(31.094150352441,504.423406943605,-35.8709384745049)) ;
#61254=CARTESIAN_POINT('Ctrl Pts',(31.1330228165377,504.42733768956,-35.9130746596511)) ;
#61255=CARTESIAN_POINT('Ctrl Pts',(31.2023854262371,504.434606817046,-35.9965112568204)) ;
#61256=CARTESIAN_POINT('Ctrl Pts',(31.2332894861913,504.437960144194,-36.0373787220969)) ;
#61257=CARTESIAN_POINT('Ctrl Pts',(31.3414899318344,504.450237873685,-36.1950772960683)) ;
#61258=CARTESIAN_POINT('Ctrl Pts',(31.4058400244181,504.458634702507,-36.3200695238254)) ;
#61259=CARTESIAN_POINT('Ctrl Pts',(31.4713149728053,504.470375743832,-36.4997073047313)) ;
#61260=CARTESIAN_POINT('Ctrl Pts',(31.4866085210478,504.47354464176,-36.548546939597)) ;
#61261=CARTESIAN_POINT('Ctrl Pts',(31.509368349094,504.479233295625,-36.6349981986934)) ;
#61262=CARTESIAN_POINT('Ctrl Pts',(31.5178287374945,504.481713681474,-36.6723082882773)) ;
#61263=CARTESIAN_POINT('Ctrl Pts',(31.5307973189628,504.486331667881,-36.740267060104)) ;
#61264=CARTESIAN_POINT('Ctrl Pts',(31.5357485560298,504.488446541567,-36.7708116897684)) ;
#61265=CARTESIAN_POINT('Ctrl Pts',(31.5560816371796,504.499127512867,-36.9229558446275)) ;
#61266=CARTESIAN_POINT('Ctrl Pts',(31.5588609984445,504.508175784895,-37.0458518849898)) ;
#61267=CARTESIAN_POINT('Ctrl Pts',(31.5423903234936,504.521809135464,-37.2333685292144)) ;
#61268=CARTESIAN_POINT('Ctrl Pts',(31.5327773935459,504.5265121807,-37.2984120089292)) ;
#61269=CARTESIAN_POINT('Ctrl Pts',(31.5078027914526,504.535061250799,-37.4180051352628)) ;
#61270=CARTESIAN_POINT('Ctrl Pts',(31.4934539865168,504.538930028759,-37.4726687920088)) ;
#61271=CARTESIAN_POINT('Ctrl Pts',(31.4607546069237,504.546156970532,-37.575616289686)) ;
#61272=CARTESIAN_POINT('Ctrl Pts',(31.4428836514145,504.549526461959,-37.62398212294)) ;
#61273=CARTESIAN_POINT('Ctrl Pts',(31.3703229305544,504.561461240068,-37.795443819484)) ;
#61274=CARTESIAN_POINT('Ctrl Pts',(31.3030123891598,504.5695536622,-37.9126210641733)) ;
#61275=CARTESIAN_POINT('Ctrl Pts',(31.1905646628836,504.58106319146,-38.0628645200647)) ;
#61276=CARTESIAN_POINT('Ctrl Pts',(31.1567962696498,504.584340083067,-38.1037607655317)) ;
#61277=CARTESIAN_POINT('Ctrl Pts',(31.0948503770259,504.59018948277,-38.171885498301)) ;
#61278=CARTESIAN_POINT('Ctrl Pts',(31.0675555457996,504.592719186309,-38.19985939045)) ;
#61279=CARTESIAN_POINT('Ctrl Pts',(31.0171408119758,504.597367231119,-38.2480181786567)) ;
#61280=CARTESIAN_POINT('Ctrl Pts',(30.9944001770837,504.599459194373,-38.2685713665322)) ;
#61281=CARTESIAN_POINT('Ctrl Pts',(30.8859316669576,504.609376711437,-38.3613012386849)) ;
#61282=CARTESIAN_POINT('Ctrl Pts',(30.7936320177673,504.617612868785,-38.4253337212463)) ;
#61283=CARTESIAN_POINT('Ctrl Pts',(30.6335567869241,504.63090447705,-38.5139776708744)) ;
#61284=CARTESIAN_POINT('Ctrl Pts',(30.5693638243277,504.636010132638,-38.5443466897619)) ;
#61285=CARTESIAN_POINT('Ctrl Pts',(30.4488504973312,504.64512366722,-38.5922054866997)) ;
#61286=CARTESIAN_POINT('Ctrl Pts',(30.3931638365256,504.64916373651,-38.6109797977536)) ;
#61287=CARTESIAN_POINT('Ctrl Pts',(30.2882856003111,504.656474513121,-38.6402656589938)) ;
#61288=CARTESIAN_POINT('Ctrl Pts',(30.2393875840542,504.659768086624,-38.6515680386249)) ;
#61289=CARTESIAN_POINT('Ctrl Pts',(30.0972327074653,504.669073686927,-38.6777280030521)) ;
#61290=CARTESIAN_POINT('Ctrl Pts',(30.0031278187236,504.674896606954,-38.6868921379273)) ;
#61291=CARTESIAN_POINT('Ctrl Pts',(29.8038991865405,504.687079164596,-38.6893098239551)) ;
#61292=CARTESIAN_POINT('Ctrl Pts',(29.6991802951144,504.693400835222,-38.6806814645055)) ;
#61293=CARTESIAN_POINT('Ctrl Pts',(29.5604248691055,504.702411739959,-38.655931551754)) ;
#61294=CARTESIAN_POINT('Ctrl Pts',(29.525089495292,504.704764620284,-38.6484358399948)) ;
#61295=CARTESIAN_POINT('Ctrl Pts',(29.458998099112,504.709323786646,-38.6321545039943)) ;
#61296=CARTESIAN_POINT('Ctrl Pts',(29.428198159912,504.71151712402,-38.6236199890625)) ;
#61297=CARTESIAN_POINT('Ctrl Pts',(29.3611760464376,504.716415145603,-38.6029556946343)) ;
#61298=CARTESIAN_POINT('Ctrl Pts',(29.3250852623283,504.719134399474,-38.5904542925922)) ;
#61299=CARTESIAN_POINT('Ctrl Pts',(29.2052220738143,504.728376962964,-38.5442636730996)) ;
#61300=CARTESIAN_POINT('Ctrl Pts',(29.1237635829594,504.735004858204,-38.5050094135889)) ;
#61301=CARTESIAN_POINT('Ctrl Pts',(28.9737358103163,504.747560678263,-38.4170461880854)) ;
#61302=CARTESIAN_POINT('Ctrl Pts',(28.904865239867,504.753487307483,-38.3693658628624)) ;
#61303=CARTESIAN_POINT('Ctrl Pts',(28.8007541930881,504.7626710157,-38.2850289639115)) ;
#61304=CARTESIAN_POINT('Ctrl Pts',(28.7631017392957,504.766048273813,-38.2515934381774)) ;
#61305=CARTESIAN_POINT('Ctrl Pts',(28.68358132078,504.773337771596,-38.1742588931823)) ;
#61306=CARTESIAN_POINT('Ctrl Pts',(28.6424787659963,504.777212502998,-38.1296757094903)) ;
#61307=CARTESIAN_POINT('Ctrl Pts',(28.4948701589087,504.791753563263,-37.9509186692316)) ;
#61308=CARTESIAN_POINT('Ctrl Pts',(28.4068720471786,504.801719284437,-37.8028989543274)) ;
#61309=CARTESIAN_POINT('Ctrl Pts',(28.3306713993951,504.814878844816,-37.6135360615046)) ;
#61310=CARTESIAN_POINT('Ctrl Pts',(28.3192823274698,504.817043101958,-37.5826156517476)) ;
#61311=CARTESIAN_POINT('Ctrl Pts',(28.2978098136908,504.82160031745,-37.5185207020309)) ;
#61312=CARTESIAN_POINT('Ctrl Pts',(28.2878305142513,504.823996765863,-37.485328839444)) ;
#61313=CARTESIAN_POINT('Ctrl Pts',(28.2519775242662,504.833773376532,-37.3510233524459)) ;
#61314=CARTESIAN_POINT('Ctrl Pts',(28.2345960258612,504.841443558282,-37.2478931395869)) ;
#61315=CARTESIAN_POINT('Ctrl Pts',(28.2198204393433,504.856129917374,-37.0460990796966)) ;
#61316=CARTESIAN_POINT('Ctrl Pts',(28.2212989741902,504.863128964229,-36.947922933889)) ;
#61317=CARTESIAN_POINT('Ctrl Pts',(28.236573932299,504.873310251979,-36.8005240993064)) ;
#61318=CARTESIAN_POINT('Ctrl Pts',(28.2439982782578,504.876686277838,-36.7508711585461)) ;
#61319=CARTESIAN_POINT('Ctrl Pts',(28.2649251132639,504.883852817423,-36.6441351704651)) ;
#61320=CARTESIAN_POINT('Ctrl Pts',(28.2792217584378,504.887612455738,-36.587276377783)) ;
#61321=CARTESIAN_POINT('Ctrl Pts',(28.3172965947635,504.89574519811,-36.4637897806799)) ;
#61322=CARTESIAN_POINT('Ctrl Pts',(28.3423789427392,504.900076169707,-36.3976846332995)) ;
#61323=CARTESIAN_POINT('Ctrl Pts',(28.4182598676669,504.911287323251,-36.2305700188501)) ;
#61324=CARTESIAN_POINT('Ctrl Pts',(28.4752587737452,504.918105330507,-36.1327974778647)) ;
#61325=CARTESIAN_POINT('Ctrl Pts',(28.5596979907462,504.927438555201,-36.0168226005408)) ;
#61326=CARTESIAN_POINT('Ctrl Pts',(28.5783780831064,504.929467190729,-35.992597208781)) ;
#61327=CARTESIAN_POINT('Ctrl Pts',(28.6225395090025,504.934212130542,-35.9384758727604)) ;
#61328=CARTESIAN_POINT('Ctrl Pts',(28.6484270923263,504.936952080011,-35.9089451857543)) ;
#61329=CARTESIAN_POINT('Ctrl Pts',(28.7119488890555,504.943526749772,-35.8414513926158)) ;
#61330=CARTESIAN_POINT('Ctrl Pts',(28.7504156532799,504.947395358522,-35.80432964191)) ;
#61331=CARTESIAN_POINT('Ctrl Pts',(28.8910109427986,504.96099076579,-35.6811378833544)) ;
#61332=CARTESIAN_POINT('Ctrl Pts',(29.0016582060664,504.97070963352,-35.6055248417994)) ;
#61333=CARTESIAN_POINT('Ctrl Pts',(29.1659717199386,504.983489504468,-35.5201167017051)) ;
#61334=CARTESIAN_POINT('Ctrl Pts',(29.2128684082581,504.986978200553,-35.498445211476)) ;
#61335=CARTESIAN_POINT('Ctrl Pts',(29.3128978300854,504.994119221994,-35.4577491620444)) ;
#61336=CARTESIAN_POINT('Ctrl Pts',(29.3661424689265,504.997752433225,-35.4391736330252)) ;
#61337=CARTESIAN_POINT('Ctrl Pts',(29.4829858156303,505.005449635377,-35.4049502997174)) ;
#61338=CARTESIAN_POINT('Ctrl Pts',(29.5467710357804,505.00948187133,-35.3902792518849)) ;
#61339=CARTESIAN_POINT('Ctrl Pts',(29.7331360403668,505.021050937422,-35.3588240280395)) ;
#61340=CARTESIAN_POINT('Ctrl Pts',(29.8569074724625,505.028460527986,-35.3518832920923)) ;
#61341=CARTESIAN_POINT('Ctrl Pts',(30.0111009000491,505.038495321206,-35.3603887638529)) ;
#61342=CARTESIAN_POINT('Ctrl Pts',(30.0418603211689,505.040539427872,-35.3629442760115)) ;
#61343=CARTESIAN_POINT('Ctrl Pts',(30.1109129553052,505.045254007532,-35.3706178213031)) ;
#61344=CARTESIAN_POINT('Ctrl Pts',(30.1491312633468,505.047945531556,-35.376215912461)) ;
#61345=CARTESIAN_POINT('Ctrl Pts',(30.2814475543236,505.057474417214,-35.4003205988776)) ;
#61346=CARTESIAN_POINT('Ctrl Pts',(30.3741140780086,505.064511658039,-35.4256158096493)) ;
#61347=CARTESIAN_POINT('Ctrl Pts',(30.4640863420645,505.071468680575,-35.458738231369)) ;
#61348=CARTESIAN_POINT('Ctrl Pts',(30.4640904799732,504.178934308784,-35.4587397547064)) ;
#61349=CARTESIAN_POINT('Ctrl Pts',(30.4907011144323,504.180665101958,-35.4685362832436)) ;
#61350=CARTESIAN_POINT('Ctrl Pts',(30.5170714890677,504.182393321346,-35.4790158374907)) ;
#61351=CARTESIAN_POINT('Ctrl Pts',(30.6056643235233,504.188277764651,-35.5168731914104)) ;
#61352=CARTESIAN_POINT('Ctrl Pts',(30.6664576028908,504.192452399163,-35.547372768982)) ;
#61353=CARTESIAN_POINT('Ctrl Pts',(30.7749430871822,504.200360350362,-35.6103774131304)) ;
#61354=CARTESIAN_POINT('Ctrl Pts',(30.8231369247307,504.204056835209,-35.6418097956032)) ;
#61355=CARTESIAN_POINT('Ctrl Pts',(30.910970371616,504.211227626555,-35.705806787347)) ;
#61356=CARTESIAN_POINT('Ctrl Pts',(30.9509197831789,504.214677510178,-35.7378326074416)) ;
#61357=CARTESIAN_POINT('Ctrl Pts',(31.0955111224068,504.227942923774,-35.865112990807)) ;
#61358=CARTESIAN_POINT('Ctrl Pts',(31.1893389281624,504.238260893217,-35.9717116928767)) ;
#61359=CARTESIAN_POINT('Ctrl Pts',(31.2970019770797,504.25222851145,-36.1309059329223)) ;
#61360=CARTESIAN_POINT('Ctrl Pts',(31.3235110651886,504.255898359007,-36.1742466747629)) ;
#61361=CARTESIAN_POINT('Ctrl Pts',(31.366375972885,504.262191723867,-36.2521133151798)) ;
#61362=CARTESIAN_POINT('Ctrl Pts',(31.3836028547328,504.264845741402,-36.2861176778182)) ;
#61363=CARTESIAN_POINT('Ctrl Pts',(31.4127861562838,504.269545294304,-36.3489846440859)) ;
#61364=CARTESIAN_POINT('Ctrl Pts',(31.4251251096603,504.271609424052,-36.3776466676352)) ;
#61365=CARTESIAN_POINT('Ctrl Pts',(31.4755645661525,504.280470034501,-36.5045093805009)) ;
#61366=CARTESIAN_POINT('Ctrl Pts',(31.5051137642256,504.28685660227,-36.6058622738222)) ;
#61367=CARTESIAN_POINT('Ctrl Pts',(31.5387147580193,504.297780284296,-36.7816289284403)) ;
#61368=CARTESIAN_POINT('Ctrl Pts',(31.5477281471907,504.302280659341,-36.8547520594954)) ;
#61369=CARTESIAN_POINT('Ctrl Pts',(31.5552580151837,504.310668340292,-36.9880900742235)) ;
#61370=CARTESIAN_POINT('Ctrl Pts',(31.55540420449,504.314507575305,-37.0480849560254)) ;
#61371=CARTESIAN_POINT('Ctrl Pts',(31.5496982404839,504.321797888635,-37.1587422788779)) ;
#61372=CARTESIAN_POINT('Ctrl Pts',(31.5447553096988,504.32521516324,-37.2093802441109)) ;
#61373=CARTESIAN_POINT('Ctrl Pts',(31.5245676218829,504.334934620541,-37.3495161243687)) ;
#61374=CARTESIAN_POINT('Ctrl Pts',(31.5043172307581,504.341389633905,-37.4381025199924)) ;
#61375=CARTESIAN_POINT('Ctrl Pts',(31.4448062630143,504.35567833131,-37.6262474020342)) ;
#61376=CARTESIAN_POINT('Ctrl Pts',(31.4029658153932,504.36352646484,-37.7245865547845)) ;
#61377=CARTESIAN_POINT('Ctrl Pts',(31.3341699895455,504.373701781066,-37.8510561122995)) ;
#61378=CARTESIAN_POINT('Ctrl Pts',(31.3152272053732,504.37629781547,-37.8832520369713)) ;
#61379=CARTESIAN_POINT('Ctrl Pts',(31.2782180182557,504.380974069887,-37.9415747326819)) ;
#61380=CARTESIAN_POINT('Ctrl Pts',(31.2604575940171,504.383068956177,-37.9678719856091)) ;
#61381=CARTESIAN_POINT('Ctrl Pts',(31.1743298119563,504.392637318802,-38.0878610062847)) ;
#61382=CARTESIAN_POINT('Ctrl Pts',(31.0970414817693,504.399618028477,-38.1747690329425)) ;
#61383=CARTESIAN_POINT('Ctrl Pts',(30.961272612537,504.410855710863,-38.2986269216421)) ;
#61384=CARTESIAN_POINT('Ctrl Pts',(30.9084663887144,504.415024194965,-38.3412026621245)) ;
#61385=CARTESIAN_POINT('Ctrl Pts',(30.8063211535929,504.42292979897,-38.4137490700687)) ;
#61386=CARTESIAN_POINT('Ctrl Pts',(30.7577365016669,504.426630812306,-38.4446014988423)) ;
#61387=CARTESIAN_POINT('Ctrl Pts',(30.6626998312883,504.433838277046,-38.4982628230963)) ;
#61388=CARTESIAN_POINT('Ctrl Pts',(30.6165908763741,504.43732162946,-38.5215415474714)) ;
#61389=CARTESIAN_POINT('Ctrl Pts',(30.4437705063967,504.450373728195,-38.5989397397799)) ;
#61390=CARTESIAN_POINT('Ctrl Pts',(30.3115842294009,504.460407264738,-38.6394225371948)) ;
#61391=CARTESIAN_POINT('Ctrl Pts',(30.1246126224308,504.474206594011,-38.6721714552532)) ;
#61392=CARTESIAN_POINT('Ctrl Pts',(30.0728688706349,504.477977406946,-38.6787507480919)) ;
#61393=CARTESIAN_POINT('Ctrl Pts',(29.9822867808964,504.484416414237,-38.685970735421)) ;
#61394=CARTESIAN_POINT('Ctrl Pts',(29.9435749109091,504.487116777064,-38.6877011601384)) ;
#61395=CARTESIAN_POINT('Ctrl Pts',(29.8737630129181,504.491853884982,-38.6883845013247)) ;
#61396=CARTESIAN_POINT('Ctrl Pts',(29.842689357502,504.493911516148,-38.6878193451084)) ;
#61397=CARTESIAN_POINT('Ctrl Pts',(29.7041100929686,504.502922643108,-38.6814176055466)) ;
#61398=CARTESIAN_POINT('Ctrl Pts',(29.5972914075657,504.509443756828,-38.6660375990937)) ;
#61399=CARTESIAN_POINT('Ctrl Pts',(29.4221165524651,504.520455775701,-38.6231897395625)) ;
#61400=CARTESIAN_POINT('Ctrl Pts',(29.3527489373109,504.524902935258,-38.6013293068749)) ;
#61401=CARTESIAN_POINT('Ctrl Pts',(29.2295202282037,504.53321287539,-38.5534382064981)) ;
#61402=CARTESIAN_POINT('Ctrl Pts',(29.1752099573159,504.537029566373,-38.5289049259005)) ;
#61403=CARTESIAN_POINT('Ctrl Pts',(29.0776176967347,504.544265183361,-38.4783596755257)) ;
#61404=CARTESIAN_POINT('Ctrl Pts',(29.0339792758185,504.54765031761,-38.453187099049)) ;
#61405=CARTESIAN_POINT('Ctrl Pts',(28.9148868609788,504.557354038443,-38.3770979212853)) ;
#61406=CARTESIAN_POINT('Ctrl Pts',(28.8423754253948,504.563828251882,-38.3219268716572)) ;
#61407=CARTESIAN_POINT('Ctrl Pts',(28.6954838152663,504.578135134068,-38.1898758427256)) ;
#61408=CARTESIAN_POINT('Ctrl Pts',(28.623247345394,504.585981263866,-38.111187502659)) ;
#61409=CARTESIAN_POINT('Ctrl Pts',(28.5365293980443,504.596153456221,-37.9963520285435)) ;
#61410=CARTESIAN_POINT('Ctrl Pts',(28.5150426212387,504.598748664611,-37.9658171489067)) ;
#61411=CARTESIAN_POINT('Ctrl Pts',(28.4772641271797,504.603419285255,-37.9081020703248)) ;
#61412=CARTESIAN_POINT('Ctrl Pts',(28.460688141321,504.605509544811,-37.8811318041395)) ;
#61413=CARTESIAN_POINT('Ctrl Pts',(28.386715734315,504.615112203666,-37.7527088308068)) ;
#61414=CARTESIAN_POINT('Ctrl Pts',(28.3392924273754,504.622124959081,-37.6458733421152)) ;
#61415=CARTESIAN_POINT('Ctrl Pts',(28.2825984776944,504.63338753655,-37.4706225938849)) ;
#61416=CARTESIAN_POINT('Ctrl Pts',(28.265724868551,504.637546213729,-37.4050925232578)) ;
#61417=CARTESIAN_POINT('Ctrl Pts',(28.2419642768403,504.645437098255,-37.2823237836898)) ;
#61418=CARTESIAN_POINT('Ctrl Pts',(28.2339743448999,504.64913349586,-37.2254043310153)) ;
#61419=CARTESIAN_POINT('Ctrl Pts',(28.2244145514327,504.656336197896,-37.1167604938927)) ;
#61420=CARTESIAN_POINT('Ctrl Pts',(28.2222827180057,504.659819652864,-37.0651534021609)) ;
#61421=CARTESIAN_POINT('Ctrl Pts',(28.2232610291204,504.672845454525,-36.8761851121111)) ;
#61422=CARTESIAN_POINT('Ctrl Pts',(28.2409551547823,504.682849220847,-36.7394719751709)) ;
#61423=CARTESIAN_POINT('Ctrl Pts',(28.2882394629522,504.696626913346,-36.5559401494667)) ;
#61424=CARTESIAN_POINT('Ctrl Pts',(28.3036402169593,504.700404727469,-36.5060052666149)) ;
#61425=CARTESIAN_POINT('Ctrl Pts',(28.3345189341348,504.706853537362,-36.4203990176483)) ;
#61426=CARTESIAN_POINT('Ctrl Pts',(28.3489463634585,504.709556820619,-36.3843908914333)) ;
#61427=CARTESIAN_POINT('Ctrl Pts',(28.3771711069419,504.714296043972,-36.3205033510563)) ;
#61428=CARTESIAN_POINT('Ctrl Pts',(28.3905154654764,504.716353027107,-36.2924475525481)) ;
#61429=CARTESIAN_POINT('Ctrl Pts',(28.4536846769671,504.725379129408,-36.1686838939503)) ;
#61430=CARTESIAN_POINT('Ctrl Pts',(28.5119579065753,504.731913573759,-36.0775658859773)) ;
#61431=CARTESIAN_POINT('Ctrl Pts',(28.6235012799821,504.742936127844,-35.9356360680403)) ;
#61432=CARTESIAN_POINT('Ctrl Pts',(28.6720405308344,504.747379793806,-35.8815531297736)) ;
#61433=CARTESIAN_POINT('Ctrl Pts',(28.7665271136365,504.755685187347,-35.789189751515)) ;
#61434=CARTESIAN_POINT('Ctrl Pts',(28.8113009889449,504.759500965598,-35.7498855707174)) ;
#61435=CARTESIAN_POINT('Ctrl Pts',(28.8976650580656,504.766737110976,-35.681904430462)) ;
#61436=CARTESIAN_POINT('Ctrl Pts',(28.9386405089888,504.770123808217,-35.6525589211314)) ;
#61437=CARTESIAN_POINT('Ctrl Pts',(29.0577673824255,504.779878415715,-35.5751630419295)) ;
#61438=CARTESIAN_POINT('Ctrl Pts',(29.138636417171,504.786405515967,-35.5316496523497)) ;
#61439=CARTESIAN_POINT('Ctrl Pts',(29.2988974047154,504.799071204943,-35.4617727015263)) ;
#61440=CARTESIAN_POINT('Ctrl Pts',(29.377515150584,504.805169540373,-35.4342876098999)) ;
#61441=CARTESIAN_POINT('Ctrl Pts',(29.5061494292016,504.814734545311,-35.3998648546688)) ;
#61442=CARTESIAN_POINT('Ctrl Pts',(29.555004743805,504.818274079265,-35.3891204419165)) ;
#61443=CARTESIAN_POINT('Ctrl Pts',(29.6333991237245,504.823734147088,-35.3755457240655)) ;
#61444=CARTESIAN_POINT('Ctrl Pts',(29.662651257049,504.825720307625,-35.3712786297883)) ;
#61445=CARTESIAN_POINT('Ctrl Pts',(29.7447474034344,504.831159707993,-35.3615265866565)) ;
#61446=CARTESIAN_POINT('Ctrl Pts',(29.7977620325855,504.834526901093,-35.3577865547951)) ;
#61447=CARTESIAN_POINT('Ctrl Pts',(29.9616519833074,504.84473567362,-35.3540811318244)) ;
#61448=CARTESIAN_POINT('Ctrl Pts',(30.072409488731,504.851369367733,-35.3626348727482)) ;
#61449=CARTESIAN_POINT('Ctrl Pts',(30.2525156761033,504.862693904126,-35.394808733771)) ;
#61450=CARTESIAN_POINT('Ctrl Pts',(30.322622955803,504.867238072286,-35.4120920768919)) ;
#61451=CARTESIAN_POINT('Ctrl Pts',(30.4158119787388,504.873599448271,-35.4415957968915)) ;
#61452=CARTESIAN_POINT('Ctrl Pts',(30.4400537646826,504.875284228122,-35.4498907971939)) ;
#61453=CARTESIAN_POINT('Ctrl Pts',(30.4640904938027,504.876987562729,-35.4587397597976)) ;
#61454=CARTESIAN_POINT('Origin',(29.8885276254015,502.164639880024,-37.0221601717529)) ;
#61455=CARTESIAN_POINT('',(29.8869092437844,504.615879743148,-34.9674106288422)) ;
#61456=CARTESIAN_POINT('Ctrl Pts',(31.5177152521424,504.164515898581,-38.2742565096501)) ;
#61457=CARTESIAN_POINT('Ctrl Pts',(31.5148235489527,504.164756875326,-38.2780191011651)) ;
#61458=CARTESIAN_POINT('Ctrl Pts',(31.5119187232967,504.164997289862,-38.281771789605)) ;
#61459=CARTESIAN_POINT('Ctrl Pts',(31.4250406485552,504.172139640842,-38.393208136478)) ;
#61460=CARTESIAN_POINT('Ctrl Pts',(31.3305490130783,504.178599631649,-38.4922704745298)) ;
#61461=CARTESIAN_POINT('Ctrl Pts',(31.1532930766517,504.18999601998,-38.6444370332624)) ;
#61462=CARTESIAN_POINT('Ctrl Pts',(31.0752852035322,504.194813416355,-38.7023440114372)) ;
#61463=CARTESIAN_POINT('Ctrl Pts',(30.949737991717,504.202532357627,-38.7824221956525)) ;
#61464=CARTESIAN_POINT('Ctrl Pts',(30.9049538153029,504.205278060223,-38.8086558989463)) ;
#61465=CARTESIAN_POINT('Ctrl Pts',(30.8111129902634,504.211042858654,-38.8589546317743)) ;
#61466=CARTESIAN_POINT('Ctrl Pts',(30.7619937126592,504.214066489737,-38.8828143119784)) ;
#61467=CARTESIAN_POINT('Ctrl Pts',(30.5800826690271,504.225303492967,-38.962386093982)) ;
#61468=CARTESIAN_POINT('Ctrl Pts',(30.4424977051433,504.233912094998,-39.0060530827161)) ;
#61469=CARTESIAN_POINT('Ctrl Pts',(30.197888625853,504.24893002881,-39.0562401098375)) ;
#61470=CARTESIAN_POINT('Ctrl Pts',(30.092779254595,504.255282823913,-39.0694681919765)) ;
#61471=CARTESIAN_POINT('Ctrl Pts',(29.9543132818391,504.263178631244,-39.0761192898812)) ;
#61472=CARTESIAN_POINT('Ctrl Pts',(29.9214791238713,504.265015593504,-39.0769084030974)) ;
#61473=CARTESIAN_POINT('Ctrl Pts',(29.8560888868276,504.268584680553,-39.0769119187796)) ;
#61474=CARTESIAN_POINT('Ctrl Pts',(29.8235422794873,504.27031687866,-39.0761402520766)) ;
#61475=CARTESIAN_POINT('Ctrl Pts',(29.6961630925704,504.276969907332,-39.0700890533033)) ;
#61476=CARTESIAN_POINT('Ctrl Pts',(29.6017171766313,504.281631194197,-39.0590106957116)) ;
#61477=CARTESIAN_POINT('Ctrl Pts',(29.3501804194694,504.294061759902,-39.0116551863151)) ;
#61478=CARTESIAN_POINT('Ctrl Pts',(29.1960529846797,504.301740650502,-38.963392708511)) ;
#61479=CARTESIAN_POINT('Ctrl Pts',(29.000576079914,504.312781599337,-38.8759051151238)) ;
#61480=CARTESIAN_POINT('Ctrl Pts',(28.9528795596217,504.315582142882,-38.8522941201617)) ;
#61481=CARTESIAN_POINT('Ctrl Pts',(28.8597230943665,504.321298516359,-38.8015852483557)) ;
#61482=CARTESIAN_POINT('Ctrl Pts',(28.8142868220569,504.324211328772,-38.7745295183716)) ;
#61483=CARTESIAN_POINT('Ctrl Pts',(28.672155293724,504.333748773588,-38.6822887597222)) ;
#61484=CARTESIAN_POINT('Ctrl Pts',(28.5799550021247,504.340612396311,-38.6106247733197)) ;
#61485=CARTESIAN_POINT('Ctrl Pts',(28.3906925171473,504.356054008684,-38.4358061889736)) ;
#61486=CARTESIAN_POINT('Ctrl Pts',(28.2971796642736,504.364653587044,-38.3296465469626)) ;
#61487=CARTESIAN_POINT('Ctrl Pts',(28.1963986426728,504.374535187488,-38.1882456950988)) ;
#61488=CARTESIAN_POINT('Ctrl Pts',(28.1781470982285,504.376353560173,-38.1613066476604)) ;
#61489=CARTESIAN_POINT('Ctrl Pts',(28.1427778843342,504.379918632784,-38.1063341641738)) ;
#61490=CARTESIAN_POINT('Ctrl Pts',(28.1256770795843,504.381664176009,-38.0783010876621)) ;
#61491=CARTESIAN_POINT('Ctrl Pts',(28.0564219140068,504.388881012845,-37.9583994939058)) ;
#61492=CARTESIAN_POINT('Ctrl Pts',(28.0107158627895,504.394026474673,-37.8629829110937)) ;
#61493=CARTESIAN_POINT('Ctrl Pts',(27.9205134428556,504.406123512417,-37.6301597935089)) ;
#61494=CARTESIAN_POINT('Ctrl Pts',(27.8827489167825,504.413041687382,-37.4907663634845)) ;
#61495=CARTESIAN_POINT('Ctrl Pts',(27.8512031161613,504.423234806284,-37.2947089638861)) ;
#61496=CARTESIAN_POINT('Ctrl Pts',(27.8446856426347,504.426094497572,-37.2405250451073)) ;
#61497=CARTESIAN_POINT('Ctrl Pts',(27.8361919969776,504.431809923338,-37.1344407125451)) ;
#61498=CARTESIAN_POINT('Ctrl Pts',(27.8340118596933,504.434656792618,-37.0825979546641)) ;
#61499=CARTESIAN_POINT('Ctrl Pts',(27.8333907404359,504.443004252779,-36.933699146649)) ;
#61500=CARTESIAN_POINT('Ctrl Pts',(27.8398597229981,504.44865278662,-36.8367718348499)) ;
#61501=CARTESIAN_POINT('Ctrl Pts',(27.8718630661051,504.462548232292,-36.6053613124954)) ;
#61502=CARTESIAN_POINT('Ctrl Pts',(27.904022200339,504.470893467997,-36.4722556065769)) ;
#61503=CARTESIAN_POINT('Ctrl Pts',(27.9643312583325,504.481562027557,-36.299957102833)) ;
#61504=CARTESIAN_POINT('Ctrl Pts',(27.9809634875001,504.484200708119,-36.2571055145642)) ;
#61505=CARTESIAN_POINT('Ctrl Pts',(28.0104662349016,504.488387610518,-36.1880548465334)) ;
#61506=CARTESIAN_POINT('Ctrl Pts',(28.0224804906909,504.489978912064,-36.1615123860689)) ;
#61507=CARTESIAN_POINT('Ctrl Pts',(28.0540773742399,504.493892480927,-36.0954825385167)) ;
#61508=CARTESIAN_POINT('Ctrl Pts',(28.0743723871633,504.496174775951,-36.0563545557368)) ;
#61509=CARTESIAN_POINT('Ctrl Pts',(28.1255351294484,504.501482940851,-35.9650278341757)) ;
#61510=CARTESIAN_POINT('Ctrl Pts',(28.1574857105561,504.504464093686,-35.9134825958934)) ;
#61511=CARTESIAN_POINT('Ctrl Pts',(28.2846566893434,504.515445262384,-35.7272530740073)) ;
#61512=CARTESIAN_POINT('Ctrl Pts',(28.393688025964,504.523270905339,-35.602780418299)) ;
#61513=CARTESIAN_POINT('Ctrl Pts',(28.5569189335517,504.534531985956,-35.4563454578015)) ;
#61514=CARTESIAN_POINT('Ctrl Pts',(28.5988398778898,504.537384910656,-35.4216408142721)) ;
#61515=CARTESIAN_POINT('Ctrl Pts',(28.6833922257485,504.543098697741,-35.357123884478)) ;
#61516=CARTESIAN_POINT('Ctrl Pts',(28.7258760073268,504.545951287438,-35.3271859281487)) ;
#61517=CARTESIAN_POINT('Ctrl Pts',(28.851944265802,504.554381603345,-35.2453178548258)) ;
#61518=CARTESIAN_POINT('Ctrl Pts',(28.9381730330999,504.56011285664,-35.1977436287525)) ;
#61519=CARTESIAN_POINT('Ctrl Pts',(29.1557118326525,504.574373885363,-35.0973410652257)) ;
#61520=CARTESIAN_POINT('Ctrl Pts',(29.2897146013487,504.583011428528,-35.0515332237529)) ;
#61521=CARTESIAN_POINT('Ctrl Pts',(29.4687426135226,504.593694047923,-35.010299877618)) ;
#61522=CARTESIAN_POINT('Ctrl Pts',(29.5104182485432,504.596120142491,-35.0020524700819)) ;
#61523=CARTESIAN_POINT('Ctrl Pts',(29.5811185464928,504.600100505977,-34.9903262099202)) ;
#61524=CARTESIAN_POINT('Ctrl Pts',(29.6100105628021,504.601687189038,-34.9861645957613)) ;
#61525=CARTESIAN_POINT('Ctrl Pts',(29.6715541801972,504.604988205767,-34.9786346361948)) ;
#61526=CARTESIAN_POINT('Ctrl Pts',(29.7042143846149,504.606695294684,-34.9754303519592)) ;
#61527=CARTESIAN_POINT('Ctrl Pts',(29.7868420118162,504.610932294638,-34.9693178657169)) ;
#61528=CARTESIAN_POINT('Ctrl Pts',(29.8368657604163,504.613422434739,-34.9674502061277)) ;
#61529=CARTESIAN_POINT('Ctrl Pts',(29.8869100116458,504.615880093082,-34.9674108084909)) ;
#61530=CARTESIAN_POINT('Ctrl Pts',(29.8869092286308,504.615880054629,-34.9674108091075)) ;
#61531=CARTESIAN_POINT('Ctrl Pts',(29.9743151528632,504.620172534274,-34.9673419649612)) ;
#61532=CARTESIAN_POINT('Ctrl Pts',(30.061638319728,504.624361881162,-34.9728503261362)) ;
#61533=CARTESIAN_POINT('Ctrl Pts',(30.2214344170103,504.63219255041,-34.9932197654128)) ;
#61534=CARTESIAN_POINT('Ctrl Pts',(30.2939642411405,504.635810289608,-35.0064602112025)) ;
#61535=CARTESIAN_POINT('Ctrl Pts',(30.425659735867,504.642647313586,-35.0378979797031)) ;
#61536=CARTESIAN_POINT('Ctrl Pts',(30.4850155008177,504.645832003589,-35.0549264318618)) ;
#61537=CARTESIAN_POINT('Ctrl Pts',(30.5908536792851,504.651754221207,-35.0905208552764)) ;
#61538=CARTESIAN_POINT('Ctrl Pts',(30.6375962064229,504.654458877904,-35.108162266111)) ;
#61539=CARTESIAN_POINT('Ctrl Pts',(30.7487274051546,504.661125615687,-35.154799658217)) ;
#61540=CARTESIAN_POINT('Ctrl Pts',(30.8123511196922,504.665142224397,-35.185443691651)) ;
#61541=CARTESIAN_POINT('Ctrl Pts',(31.0019409790919,504.677723377999,-35.2891045421784)) ;
#61542=CARTESIAN_POINT('Ctrl Pts',(31.121831933475,504.686584265912,-35.3722738701345)) ;
#61543=CARTESIAN_POINT('Ctrl Pts',(31.2838060677299,504.699342497518,-35.5122270559041)) ;
#61544=CARTESIAN_POINT('Ctrl Pts',(31.333421582142,504.703372433043,-35.5596339402745)) ;
#61545=CARTESIAN_POINT('Ctrl Pts',(31.401818237834,504.708999622481,-35.6318711465972)) ;
#61546=CARTESIAN_POINT('Ctrl Pts',(31.4225531129196,504.710715619432,-35.6547837498582)) ;
#61547=CARTESIAN_POINT('Ctrl Pts',(31.4657496508298,504.714297294096,-35.7047373248478)) ;
#61548=CARTESIAN_POINT('Ctrl Pts',(31.4880495041329,504.716152799631,-35.7319034690109)) ;
#61549=CARTESIAN_POINT('Ctrl Pts',(31.593358102968,504.725021404996,-35.8671219264988)) ;
#61550=CARTESIAN_POINT('Ctrl Pts',(31.6661831868102,504.731509519045,-35.9826849514427)) ;
#61551=CARTESIAN_POINT('Ctrl Pts',(31.778293017743,504.743681266819,-36.2073227102153)) ;
#61552=CARTESIAN_POINT('Ctrl Pts',(31.8208504252621,504.749309037469,-36.3141357762717)) ;
#61553=CARTESIAN_POINT('Ctrl Pts',(31.8696406631956,504.757961556692,-36.4744579849168)) ;
#61554=CARTESIAN_POINT('Ctrl Pts',(31.8830615941412,504.760745441822,-36.5255515500389)) ;
#61555=CARTESIAN_POINT('Ctrl Pts',(31.9060456359246,504.766471640629,-36.6291456036399)) ;
#61556=CARTESIAN_POINT('Ctrl Pts',(31.9155617208057,504.769413009454,-36.6816144397597)) ;
#61557=CARTESIAN_POINT('Ctrl Pts',(31.9454256999068,504.781433213952,-36.8927495277647)) ;
#61558=CARTESIAN_POINT('Ctrl Pts',(31.9492557443054,504.791034735987,-37.0531607336239)) ;
#61559=CARTESIAN_POINT('Ctrl Pts',(31.9256039450413,504.806389351844,-37.3075750369586)) ;
#61560=CARTESIAN_POINT('Ctrl Pts',(31.9101157301214,504.812103960265,-37.4020628904223)) ;
#61561=CARTESIAN_POINT('Ctrl Pts',(31.8806027134349,504.81940071634,-37.5268338033386)) ;
#61562=CARTESIAN_POINT('Ctrl Pts',(31.8723513646039,504.82122148254,-37.5583525758758)) ;
#61563=CARTESIAN_POINT('Ctrl Pts',(31.8542977183121,504.82478662451,-37.6211764952282)) ;
#61564=CARTESIAN_POINT('Ctrl Pts',(31.8444884026176,504.826530000501,-37.6524698798109)) ;
#61565=CARTESIAN_POINT('Ctrl Pts',(31.7893531194999,504.835458551802,-37.8146523877921)) ;
#61566=CARTESIAN_POINT('Ctrl Pts',(31.7316223416336,504.842062177886,-37.94095946727)) ;
#61567=CARTESIAN_POINT('Ctrl Pts',(31.6181486770615,504.852940150495,-38.1347277298167)) ;
#61568=CARTESIAN_POINT('Ctrl Pts',(31.5700842716764,504.857132155032,-38.206115626978)) ;
#61569=CARTESIAN_POINT('Ctrl Pts',(31.5177151883675,504.861461047188,-38.2742565926321)) ;
#61570=CARTESIAN_POINT('Ctrl Pts',(31.5177152522312,504.803366924184,-38.2742565095347)) ;
#61571=CARTESIAN_POINT('Ctrl Pts',(31.518055454289,504.803339675502,-38.27381384952)) ;
#61572=CARTESIAN_POINT('Ctrl Pts',(31.5183954781065,504.803312429802,-38.2733710480293)) ;
#61573=CARTESIAN_POINT('Ctrl Pts',(31.6278180883491,504.794540871479,-38.1307533994567)) ;
#61574=CARTESIAN_POINT('Ctrl Pts',(31.7178262718211,504.786071609238,-37.9749324629393)) ;
#61575=CARTESIAN_POINT('Ctrl Pts',(31.8064571919854,504.774108590257,-37.7612553613457)) ;
#61576=CARTESIAN_POINT('Ctrl Pts',(31.8245903385251,504.771356396023,-37.7123601691067)) ;
#61577=CARTESIAN_POINT('Ctrl Pts',(31.8574845436478,504.76565699939,-37.6121216766635)) ;
#61578=CARTESIAN_POINT('Ctrl Pts',(31.8721420816032,504.762708888452,-37.5607869959292)) ;
#61579=CARTESIAN_POINT('Ctrl Pts',(31.9135740012181,504.752839934177,-37.3908781454159)) ;
#61580=CARTESIAN_POINT('Ctrl Pts',(31.931829461122,504.745656491413,-37.2705072137826)) ;
#61581=CARTESIAN_POINT('Ctrl Pts',(31.9473741596984,504.73057002732,-37.0196557489838)) ;
#61582=CARTESIAN_POINT('Ctrl Pts',(31.9431040933741,504.722686426204,-36.8895910022409)) ;
#61583=CARTESIAN_POINT('Ctrl Pts',(31.9223320987491,504.713364966716,-36.7276168785901)) ;
#61584=CARTESIAN_POINT('Ctrl Pts',(31.9172675922358,504.711489515848,-36.6945463286282)) ;
#61585=CARTESIAN_POINT('Ctrl Pts',(31.9058501141434,504.707930362346,-36.6304880935951)) ;
#61586=CARTESIAN_POINT('Ctrl Pts',(31.8995849282361,504.706243281743,-36.5994951572382)) ;
#61587=CARTESIAN_POINT('Ctrl Pts',(31.8751326170149,504.700446169061,-36.4914375426429)) ;
#61588=CARTESIAN_POINT('Ctrl Pts',(31.8532082194561,504.696511771494,-36.4152843082838)) ;
#61589=CARTESIAN_POINT('Ctrl Pts',(31.7658565660364,504.683639719898,-36.1668560123068)) ;
#61590=CARTESIAN_POINT('Ctrl Pts',(31.6817022353868,504.674959848809,-36.0021439832749)) ;
#61591=CARTESIAN_POINT('Ctrl Pts',(31.5471179687585,504.662740588675,-35.8081693594873)) ;
#61592=CARTESIAN_POINT('Ctrl Pts',(31.5159023175279,504.659996309372,-35.7666337562143)) ;
#61593=CARTESIAN_POINT('Ctrl Pts',(31.4493226785199,504.654288909477,-35.6847024350061)) ;
#61594=CARTESIAN_POINT('Ctrl Pts',(31.4138826545651,504.651323752432,-35.6444208412975)) ;
#61595=CARTESIAN_POINT('Ctrl Pts',(31.3306339529066,504.644504095972,-35.5569528916296)) ;
#61596=CARTESIAN_POINT('Ctrl Pts',(31.2820073201595,504.640616945316,-35.5106324505666)) ;
#61597=CARTESIAN_POINT('Ctrl Pts',(31.1289495665657,504.628696319042,-35.3785060219119)) ;
#61598=CARTESIAN_POINT('Ctrl Pts',(31.0182463937016,504.620457396717,-35.3005394412097)) ;
#61599=CARTESIAN_POINT('Ctrl Pts',(30.8488917454572,504.608925125323,-35.204677817596)) ;
#61600=CARTESIAN_POINT('Ctrl Pts',(30.7958312837281,504.605452863158,-35.1776161687232)) ;
#61601=CARTESIAN_POINT('Ctrl Pts',(30.7144288796586,504.600411297327,-35.1404638333113)) ;
#61602=CARTESIAN_POINT('Ctrl Pts',(30.6869204004802,504.598755356804,-35.1286281849115)) ;
#61603=CARTESIAN_POINT('Ctrl Pts',(30.6252205371183,504.595158362591,-35.1036655864817)) ;
#61604=CARTESIAN_POINT('Ctrl Pts',(30.5909188484938,504.593233448648,-35.0908433033592)) ;
#61605=CARTESIAN_POINT('Ctrl Pts',(30.5132768639043,504.58900425143,-35.0641625676601)) ;
#61606=CARTESIAN_POINT('Ctrl Pts',(30.4697818309885,504.586722099753,-35.0508128627286)) ;
#61607=CARTESIAN_POINT('Ctrl Pts',(30.3102779048337,504.578551617017,-35.0075960671411)) ;
#61608=CARTESIAN_POINT('Ctrl Pts',(30.1921591688437,504.572863673324,-34.9864412659003)) ;
#61609=CARTESIAN_POINT('Ctrl Pts',(29.9835043897067,504.562604900725,-34.9676462385594)) ;
#61610=CARTESIAN_POINT('Ctrl Pts',(29.8937183611511,504.558125843547,-34.965459190854)) ;
#61611=CARTESIAN_POINT('Ctrl Pts',(29.7530225855961,504.550810306761,-34.971246375075)) ;
#61612=CARTESIAN_POINT('Ctrl Pts',(29.7020629906538,504.548100485852,-34.9752504693354)) ;
#61613=CARTESIAN_POINT('Ctrl Pts',(29.596698643478,504.542347393465,-34.9874965832376)) ;
#61614=CARTESIAN_POINT('Ctrl Pts',(29.5423698634712,504.539296670944,-34.9960323250186)) ;
#61615=CARTESIAN_POINT('Ctrl Pts',(29.3750845272703,504.529626961228,-35.0292396050918)) ;
#61616=CARTESIAN_POINT('Ctrl Pts',(29.2638314811684,504.522785926783,-35.061266247792)) ;
#61617=CARTESIAN_POINT('Ctrl Pts',(29.0350649430583,504.508087502773,-35.1485755269603)) ;
#61618=CARTESIAN_POINT('Ctrl Pts',(28.9188728071577,504.500237696303,-35.2059852861536)) ;
#61619=CARTESIAN_POINT('Ctrl Pts',(28.7803530824693,504.490943534214,-35.2915336865619)) ;
#61620=CARTESIAN_POINT('Ctrl Pts',(28.7522952996634,504.489065841819,-35.3098239759593)) ;
#61621=CARTESIAN_POINT('Ctrl Pts',(28.6986673940265,504.48550611848,-35.346681835444)) ;
#61622=CARTESIAN_POINT('Ctrl Pts',(28.6730544150619,504.483820562522,-35.3651689085796)) ;
#61623=CARTESIAN_POINT('Ctrl Pts',(28.5851449218539,504.478049445089,-35.4317563831467)) ;
#61624=CARTESIAN_POINT('Ctrl Pts',(28.5251886937477,504.47413725332,-35.4828421873308)) ;
#61625=CARTESIAN_POINT('Ctrl Pts',(28.3345871126536,504.461242576263,-35.6651398318796)) ;
#61626=CARTESIAN_POINT('Ctrl Pts',(28.2187641410032,504.452525603814,-35.8104983358359)) ;
#61627=CARTESIAN_POINT('Ctrl Pts',(28.0973544399116,504.440259969451,-36.0139969402947)) ;
#61628=CARTESIAN_POINT('Ctrl Pts',(28.0724490295943,504.437515996184,-36.0595842707441)) ;
#61629=CARTESIAN_POINT('Ctrl Pts',(28.0253561422967,504.431805206114,-36.1541317303312)) ;
#61630=CARTESIAN_POINT('Ctrl Pts',(28.0033093359974,504.428836168213,-36.2031164721737)) ;
#61631=CARTESIAN_POINT('Ctrl Pts',(27.9580771506564,504.422012024509,-36.3151493027802)) ;
#61632=CARTESIAN_POINT('Ctrl Pts',(27.9360140165513,504.418124462712,-36.3785821329784)) ;
#61633=CARTESIAN_POINT('Ctrl Pts',(27.8788522900084,504.406168821206,-36.5731498245496)) ;
#61634=CARTESIAN_POINT('Ctrl Pts',(27.853598022308,504.397893463499,-36.7067815836235)) ;
#61635=CARTESIAN_POINT('Ctrl Pts',(27.8365293408457,504.386369138365,-36.9006179389331)) ;
#61636=CARTESIAN_POINT('Ctrl Pts',(27.8338874974816,504.38293466512,-36.9595139539795)) ;
#61637=CARTESIAN_POINT('Ctrl Pts',(27.8337274547556,504.377947841857,-37.0480613630741)) ;
#61638=CARTESIAN_POINT('Ctrl Pts',(27.8343141637769,504.376310370602,-37.0776765652497)) ;
#61639=CARTESIAN_POINT('Ctrl Pts',(27.8370603179552,504.372727553615,-37.14391591728)) ;
#61640=CARTESIAN_POINT('Ctrl Pts',(27.8395603316326,504.370799329269,-37.1805140851523)) ;
#61641=CARTESIAN_POINT('Ctrl Pts',(27.8473627635365,504.366561213734,-37.2624146340991)) ;
#61642=CARTESIAN_POINT('Ctrl Pts',(27.8531962550742,504.364273560524,-37.3076472120647)) ;
#61643=CARTESIAN_POINT('Ctrl Pts',(27.8799175670082,504.356059128149,-37.4716180204413)) ;
#61644=CARTESIAN_POINT('Ctrl Pts',(27.9097359245385,504.350334210273,-37.5886510114655)) ;
#61645=CARTESIAN_POINT('Ctrl Pts',(27.9790501523618,504.340073501606,-37.7862176954731)) ;
#61646=CARTESIAN_POINT('Ctrl Pts',(28.0138591111613,504.335635127387,-37.8680348136569)) ;
#61647=CARTESIAN_POINT('Ctrl Pts',(28.0768311937259,504.328365975392,-37.9929117547693)) ;
#61648=CARTESIAN_POINT('Ctrl Pts',(28.1015008840197,504.325658279698,-38.037609528763)) ;
#61649=CARTESIAN_POINT('Ctrl Pts',(28.1562403639933,504.319896474891,-38.1286053015315)) ;
#61650=CARTESIAN_POINT('Ctrl Pts',(28.1865626300446,504.316834308049,-38.1747027098842)) ;
#61651=CARTESIAN_POINT('Ctrl Pts',(28.2870125577057,504.307056071724,-38.3147890656886)) ;
#61652=CARTESIAN_POINT('Ctrl Pts',(28.3633438674579,504.300110143312,-38.4040242422746)) ;
#61653=CARTESIAN_POINT('Ctrl Pts',(28.5371863629811,504.285457836782,-38.5752042210906)) ;
#61654=CARTESIAN_POINT('Ctrl Pts',(28.6355603256371,504.277767426526,-38.6556061117652)) ;
#61655=CARTESIAN_POINT('Ctrl Pts',(28.7686590801501,504.268600732772,-38.7452465046634)) ;
#61656=CARTESIAN_POINT('Ctrl Pts',(28.7970566316433,504.266710787157,-38.7633733810208)) ;
#61657=CARTESIAN_POINT('Ctrl Pts',(28.8526763420077,504.263153847954,-38.7969810758505)) ;
#61658=CARTESIAN_POINT('Ctrl Pts',(28.8798308692204,504.261482306544,-38.8125534513021)) ;
#61659=CARTESIAN_POINT('Ctrl Pts',(28.9736421709229,504.255890950561,-38.8635395831377)) ;
#61660=CARTESIAN_POINT('Ctrl Pts',(29.041894354526,504.25212994789,-38.8959017889211)) ;
#61661=CARTESIAN_POINT('Ctrl Pts',(29.248364237253,504.241210692672,-38.9802088696638)) ;
#61662=CARTESIAN_POINT('Ctrl Pts',(29.3905556206666,504.234238383345,-39.0211069554706)) ;
#61663=CARTESIAN_POINT('Ctrl Pts',(29.5999831926082,504.223573199036,-39.0575890228591)) ;
#61664=CARTESIAN_POINT('Ctrl Pts',(29.6645527094485,504.220238474504,-39.0657018596547)) ;
#61665=CARTESIAN_POINT('Ctrl Pts',(29.7785069944165,504.214205655444,-39.074553801887)) ;
#61666=CARTESIAN_POINT('Ctrl Pts',(29.8277374144049,504.211551793415,-39.0766012432058)) ;
#61667=CARTESIAN_POINT('Ctrl Pts',(29.9413063160695,504.205301172694,-39.077238892392)) ;
#61668=CARTESIAN_POINT('Ctrl Pts',(30.0055972247018,504.201667030928,-39.0745800969795)) ;
#61669=CARTESIAN_POINT('Ctrl Pts',(30.1489717595916,504.193348731315,-39.061892298022)) ;
#61670=CARTESIAN_POINT('Ctrl Pts',(30.2278094507371,504.188626390787,-39.0502687459828)) ;
#61671=CARTESIAN_POINT('Ctrl Pts',(30.4381553867794,504.175744078493,-39.0066467437805)) ;
#61672=CARTESIAN_POINT('Ctrl Pts',(30.5675134413197,504.167500694065,-38.9661917702435)) ;
#61673=CARTESIAN_POINT('Ctrl Pts',(30.7243120763826,504.157724969001,-38.8995778782788)) ;
#61674=CARTESIAN_POINT('Ctrl Pts',(30.7563054070292,504.155743969045,-38.8850060993159)) ;
#61675=CARTESIAN_POINT('Ctrl Pts',(30.8155589582394,504.152122661215,-38.856160179725)) ;
#61676=CARTESIAN_POINT('Ctrl Pts',(30.8429013725043,504.150472955122,-38.842081583614)) ;
#61677=CARTESIAN_POINT('Ctrl Pts',(30.9285457798979,504.145344093845,-38.795522179738)) ;
#61678=CARTESIAN_POINT('Ctrl Pts',(30.9855909658659,504.141984230631,-38.7608102471607)) ;
#61679=CARTESIAN_POINT('Ctrl Pts',(31.1866293936743,504.129992369155,-38.6246368304838)) ;
#61680=CARTESIAN_POINT('Ctrl Pts',(31.3191086112689,504.12172427263,-38.5075692674377)) ;
#61681=CARTESIAN_POINT('Ctrl Pts',(31.4636786648758,504.110543446074,-38.3423072292991)) ;
#61682=CARTESIAN_POINT('Ctrl Pts',(31.4912659857281,504.1082936835,-38.3086742357782)) ;
#61683=CARTESIAN_POINT('Ctrl Pts',(31.5177642178171,504.106001566445,-38.2741927945048)) ;
#61684=CARTESIAN_POINT('Origin',(179.888527625402,502.164639879998,-37.0221601717597)) ;
#61685=CARTESIAN_POINT('Ctrl Pts',(181.517728902313,504.164526607599,-38.2742387482923)) ;
#61686=CARTESIAN_POINT('Ctrl Pts',(181.440913164261,504.170928309153,-38.374191180086)) ;
#61687=CARTESIAN_POINT('Ctrl Pts',(181.35506384574,504.176928754324,-38.4668625482387)) ;
#61688=CARTESIAN_POINT('Ctrl Pts',(181.204907912824,504.186728917933,-38.6016770715163)) ;
#61689=CARTESIAN_POINT('Ctrl Pts',(181.145816360762,504.190439335762,-38.6491066326943)) ;
#61690=CARTESIAN_POINT('Ctrl Pts',(181.033260293955,504.197417411237,-38.7296481294601)) ;
#61691=CARTESIAN_POINT('Ctrl Pts',(180.980636552643,504.200647192836,-38.7637758254983)) ;
#61692=CARTESIAN_POINT('Ctrl Pts',(180.883452293891,504.206612952502,-38.8206637034777)) ;
#61693=CARTESIAN_POINT('Ctrl Pts',(180.839464486277,504.209313228368,-38.8443041082496)) ;
#61694=CARTESIAN_POINT('Ctrl Pts',(180.73251015871,504.215897768503,-38.8968565464999)) ;
#61695=CARTESIAN_POINT('Ctrl Pts',(180.66886019815,504.219832450438,-38.9242307549692)) ;
#61696=CARTESIAN_POINT('Ctrl Pts',(180.465331173095,504.232453396912,-38.999826165136)) ;
#61697=CARTESIAN_POINT('Ctrl Pts',(180.321560766012,504.241459026997,-39.0361959147464)) ;
#61698=CARTESIAN_POINT('Ctrl Pts',(180.106812157454,504.254388550514,-39.0664480224822)) ;
#61699=CARTESIAN_POINT('Ctrl Pts',(180.038021849696,504.258446141896,-39.072626955555)) ;
#61700=CARTESIAN_POINT('Ctrl Pts',(179.938131845848,504.2641020352,-39.0765442973059)) ;
#61701=CARTESIAN_POINT('Ctrl Pts',(179.907191208821,504.265820788362,-39.0770584195075)) ;
#61702=CARTESIAN_POINT('Ctrl Pts',(179.841166522842,504.269402347307,-39.0766638041493)) ;
#61703=CARTESIAN_POINT('Ctrl Pts',(179.806094792212,504.271255225189,-39.0755557500163)) ;
#61704=CARTESIAN_POINT('Ctrl Pts',(179.634610612812,504.280145333299,-39.0657366804744)) ;
#61705=CARTESIAN_POINT('Ctrl Pts',(179.499260612516,504.286653222637,-39.0443267796173)) ;
#61706=CARTESIAN_POINT('Ctrl Pts',(179.256309646013,504.298832240622,-38.9805781054524)) ;
#61707=CARTESIAN_POINT('Ctrl Pts',(179.148219145409,504.304445777928,-38.9423269265333)) ;
#61708=CARTESIAN_POINT('Ctrl Pts',(178.99575486251,504.31308179847,-38.8735763113426)) ;
#61709=CARTESIAN_POINT('Ctrl Pts',(178.948483943041,504.315865097047,-38.8500283632146)) ;
#61710=CARTESIAN_POINT('Ctrl Pts',(178.855395438623,504.32159179624,-38.7990898285438)) ;
#61711=CARTESIAN_POINT('Ctrl Pts',(178.809633831471,504.324534331084,-38.7716825485577)) ;
#61712=CARTESIAN_POINT('Ctrl Pts',(178.661238632831,504.334526305746,-38.6747688768215)) ;
#61713=CARTESIAN_POINT('Ctrl Pts',(178.563840814428,504.341853162214,-38.5977715028224)) ;
#61714=CARTESIAN_POINT('Ctrl Pts',(178.393637076305,504.355943085441,-38.4362220257068)) ;
#61715=CARTESIAN_POINT('Ctrl Pts',(178.319587058913,504.362655105734,-38.3535864992456)) ;
#61716=CARTESIAN_POINT('Ctrl Pts',(178.227362585419,504.371507105705,-38.2322272324966)) ;
#61717=CARTESIAN_POINT('Ctrl Pts',(178.203179249806,504.373882736117,-38.1983119214529)) ;
#61718=CARTESIAN_POINT('Ctrl Pts',(178.163793444985,504.377816283238,-38.1393642562015)) ;
#61719=CARTESIAN_POINT('Ctrl Pts',(178.148067727621,504.379404068034,-38.1147041890701)) ;
#61720=CARTESIAN_POINT('Ctrl Pts',(178.107364097086,504.383570437789,-38.0477645233996)) ;
#61721=CARTESIAN_POINT('Ctrl Pts',(178.083366678306,504.386092698709,-38.004912672078)) ;
#61722=CARTESIAN_POINT('Ctrl Pts',(177.998025423101,504.395483358698,-37.8388246028883)) ;
#61723=CARTESIAN_POINT('Ctrl Pts',(177.947579870272,504.401985048399,-37.7103940374137)) ;
#61724=CARTESIAN_POINT('Ctrl Pts',(177.885351094748,504.413236022972,-37.4888796374843)) ;
#61725=CARTESIAN_POINT('Ctrl Pts',(177.866386046882,504.417841610328,-37.3983042318141)) ;
#61726=CARTESIAN_POINT('Ctrl Pts',(177.846441135689,504.425316724334,-37.2556966914539)) ;
#61727=CARTESIAN_POINT('Ctrl Pts',(177.841224186185,504.428049352477,-37.2043812530813)) ;
#61728=CARTESIAN_POINT('Ctrl Pts',(177.834432741539,504.433834770224,-37.0978828472443)) ;
#61729=CARTESIAN_POINT('Ctrl Pts',(177.833140556721,504.436894316832,-37.0427242136307)) ;
#61730=CARTESIAN_POINT('Ctrl Pts',(177.836718001565,504.448944858561,-36.8301591850571)) ;
#61731=CARTESIAN_POINT('Ctrl Pts',(177.857452810433,504.458423953639,-36.6735797595066)) ;
#61732=CARTESIAN_POINT('Ctrl Pts',(177.911263524934,504.471671538578,-36.4596503776431)) ;
#61733=CARTESIAN_POINT('Ctrl Pts',(177.929497424505,504.475447271999,-36.3991096166263)) ;
#61734=CARTESIAN_POINT('Ctrl Pts',(177.9655117281,504.481775975183,-36.2968665391766)) ;
#61735=CARTESIAN_POINT('Ctrl Pts',(177.981934223607,504.484369062807,-36.2547338184999)) ;
#61736=CARTESIAN_POINT('Ctrl Pts',(178.011205183651,504.488511203235,-36.1863929626504)) ;
#61737=CARTESIAN_POINT('Ctrl Pts',(178.023243498962,504.490101032807,-36.1598599183415)) ;
#61738=CARTESIAN_POINT('Ctrl Pts',(178.05521750411,504.494050632914,-36.0931938066943)) ;
#61739=CARTESIAN_POINT('Ctrl Pts',(178.075908005558,504.496368083601,-36.0534418427131)) ;
#61740=CARTESIAN_POINT('Ctrl Pts',(178.164605420021,504.50552645065,-35.8958400356843)) ;
#61741=CARTESIAN_POINT('Ctrl Pts',(178.242940964506,504.511965062077,-35.784196219905)) ;
#61742=CARTESIAN_POINT('Ctrl Pts',(178.396348330988,504.523419415139,-35.6061102895555)) ;
#61743=CARTESIAN_POINT('Ctrl Pts',(178.466284305852,504.528325858958,-35.535883756918)) ;
#61744=CARTESIAN_POINT('Ctrl Pts',(178.580267068193,504.536147179058,-35.4368662155772)) ;
#61745=CARTESIAN_POINT('Ctrl Pts',(178.620809020646,504.538897663563,-35.4042629262864)) ;
#61746=CARTESIAN_POINT('Ctrl Pts',(178.706171672828,504.544653910776,-35.3407953024403)) ;
#61747=CARTESIAN_POINT('Ctrl Pts',(178.751068485251,504.54766335062,-35.3101031261099)) ;
#61748=CARTESIAN_POINT('Ctrl Pts',(178.937276180553,504.560093262962,-35.1933683108459)) ;
#61749=CARTESIAN_POINT('Ctrl Pts',(179.087505572358,504.570071373715,-35.1227638647846)) ;
#61750=CARTESIAN_POINT('Ctrl Pts',(179.32708243113,504.585209454714,-35.0436929019299)) ;
#61751=CARTESIAN_POINT('Ctrl Pts',(179.411280315052,504.59037977148,-35.021712479621)) ;
#61752=CARTESIAN_POINT('Ctrl Pts',(179.528230841388,504.597151750432,-34.9989892605366)) ;
#61753=CARTESIAN_POINT('Ctrl Pts',(179.559980876531,504.59894931193,-34.9935912971791)) ;
#61754=CARTESIAN_POINT('Ctrl Pts',(179.62474426433,504.602514977737,-34.984141241318)) ;
#61755=CARTESIAN_POINT('Ctrl Pts',(179.657755137529,504.604280277299,-34.9801398079141)) ;
#61756=CARTESIAN_POINT('Ctrl Pts',(179.823917863895,504.612969092488,-34.9640796485024)) ;
#61757=CARTESIAN_POINT('Ctrl Pts',(179.957937769981,504.619359703623,-34.9642340272171)) ;
#61758=CARTESIAN_POINT('Ctrl Pts',(180.173504743855,504.629850002885,-34.9855800162206)) ;
#61759=CARTESIAN_POINT('Ctrl Pts',(180.255432393552,504.633884390789,-34.9987347141687)) ;
#61760=CARTESIAN_POINT('Ctrl Pts',(180.400696273933,504.641348689964,-35.0311731383869)) ;
#61761=CARTESIAN_POINT('Ctrl Pts',(180.464320305686,504.644728187107,-35.0486334452597)) ;
#61762=CARTESIAN_POINT('Ctrl Pts',(180.574351535492,504.650837753467,-35.0846035066313)) ;
#61763=CARTESIAN_POINT('Ctrl Pts',(180.621129735626,504.653522249129,-35.1018024419299)) ;
#61764=CARTESIAN_POINT('Ctrl Pts',(180.727697206733,504.659861336601,-35.1454447190358)) ;
#61765=CARTESIAN_POINT('Ctrl Pts',(180.786939439681,504.663554778688,-35.1730735488531)) ;
#61766=CARTESIAN_POINT('Ctrl Pts',(180.978470201232,504.676066557894,-35.2737771131301)) ;
#61767=CARTESIAN_POINT('Ctrl Pts',(181.104010017504,504.685251276406,-35.3586062399055)) ;
#61768=CARTESIAN_POINT('Ctrl Pts',(181.274653865825,504.698626313589,-35.5036192872005)) ;
#61769=CARTESIAN_POINT('Ctrl Pts',(181.327659970123,504.702924288147,-35.5537555068308)) ;
#61770=CARTESIAN_POINT('Ctrl Pts',(181.399429990766,504.708826035816,-35.6292678656424)) ;
#61771=CARTESIAN_POINT('Ctrl Pts',(181.42044973339,504.710565262194,-35.6524193208363)) ;
#61772=CARTESIAN_POINT('Ctrl Pts',(181.463553326009,504.714138602677,-35.7021285112233)) ;
#61773=CARTESIAN_POINT('Ctrl Pts',(181.48551199562,504.715964875973,-35.7287805774248)) ;
#61774=CARTESIAN_POINT('Ctrl Pts',(181.593731484256,504.72506888717,-35.8670917293213)) ;
#61775=CARTESIAN_POINT('Ctrl Pts',(181.669006722605,504.731772047075,-35.9868794797552)) ;
#61776=CARTESIAN_POINT('Ctrl Pts',(181.780072730742,504.743955363404,-36.212123658951)) ;
#61777=CARTESIAN_POINT('Ctrl Pts',(181.820721975699,504.749357624635,-36.3145416644425)) ;
#61778=CARTESIAN_POINT('Ctrl Pts',(181.868557806522,504.757771508443,-36.4705239191078)) ;
#61779=CARTESIAN_POINT('Ctrl Pts',(181.882161842062,504.760569876128,-36.5219162361649)) ;
#61780=CARTESIAN_POINT('Ctrl Pts',(181.905323977497,504.766292051518,-36.6255000310409)) ;
#61781=CARTESIAN_POINT('Ctrl Pts',(181.914883514516,504.769213319355,-36.6776491231629)) ;
#61782=CARTESIAN_POINT('Ctrl Pts',(181.939492009862,504.77896197232,-36.8490247851047)) ;
#61783=CARTESIAN_POINT('Ctrl Pts',(181.946103516199,504.786047048548,-36.9691959949358)) ;
#61784=CARTESIAN_POINT('Ctrl Pts',(181.937761955812,504.80137204501,-37.2245696335507)) ;
#61785=CARTESIAN_POINT('Ctrl Pts',(181.919975887731,504.809608289459,-37.3591359994321)) ;
#61786=CARTESIAN_POINT('Ctrl Pts',(181.881529340343,504.819212584416,-37.5231957434927)) ;
#61787=CARTESIAN_POINT('Ctrl Pts',(181.873201881488,504.821064985777,-37.5552275842933)) ;
#61788=CARTESIAN_POINT('Ctrl Pts',(181.855220564076,504.824637147744,-37.6181136416478)) ;
#61789=CARTESIAN_POINT('Ctrl Pts',(181.84560527541,504.826358000672,-37.6489687073554)) ;
#61790=CARTESIAN_POINT('Ctrl Pts',(181.80667823877,504.832710206947,-37.7642376514148)) ;
#61791=CARTESIAN_POINT('Ctrl Pts',(181.772596783725,504.837113637798,-37.8469432779841)) ;
#61792=CARTESIAN_POINT('Ctrl Pts',(181.67307874025,504.848105449872,-38.0497930125789)) ;
#61793=CARTESIAN_POINT('Ctrl Pts',(181.600877032597,504.854608447747,-38.1660466247542)) ;
#61794=CARTESIAN_POINT('Ctrl Pts',(181.517728902317,504.861481368308,-38.2742387482878)) ;
#61795=CARTESIAN_POINT('Ctrl Pts',(181.517728902323,504.803342258844,-38.2742387482803)) ;
#61796=CARTESIAN_POINT('Ctrl Pts',(181.518028016694,504.803318300742,-38.2738495414643)) ;
#61797=CARTESIAN_POINT('Ctrl Pts',(181.518326993276,504.803294344944,-38.2734602252776)) ;
#61798=CARTESIAN_POINT('Ctrl Pts',(181.627767714738,504.794522084801,-38.1308448219171)) ;
#61799=CARTESIAN_POINT('Ctrl Pts',(181.717819695322,504.786049499824,-37.9749595168889)) ;
#61800=CARTESIAN_POINT('Ctrl Pts',(181.806476315796,504.774082118455,-37.7612059974817)) ;
#61801=CARTESIAN_POINT('Ctrl Pts',(181.824609459599,504.771329674729,-37.7123068130391)) ;
#61802=CARTESIAN_POINT('Ctrl Pts',(181.857506971475,504.765629080746,-37.6120482968176)) ;
#61803=CARTESIAN_POINT('Ctrl Pts',(181.872166873395,504.762679991535,-37.5606973031445)) ;
#61804=CARTESIAN_POINT('Ctrl Pts',(181.913635425447,504.752799861929,-37.3905989044251)) ;
#61805=CARTESIAN_POINT('Ctrl Pts',(181.931895584619,504.745605303935,-37.2700491280813)) ;
#61806=CARTESIAN_POINT('Ctrl Pts',(181.947356611009,504.730523974722,-37.0192871434651)) ;
#61807=CARTESIAN_POINT('Ctrl Pts',(181.94308082157,504.722657547747,-36.889495447667)) ;
#61808=CARTESIAN_POINT('Ctrl Pts',(181.922353731829,504.713349563908,-36.7277634461602)) ;
#61809=CARTESIAN_POINT('Ctrl Pts',(181.917287616793,504.711472599095,-36.6946677947558)) ;
#61810=CARTESIAN_POINT('Ctrl Pts',(181.905870401056,504.707912402934,-36.6305933326396)) ;
#61811=CARTESIAN_POINT('Ctrl Pts',(181.899608710014,504.706225719172,-36.5996090117794)) ;
#61812=CARTESIAN_POINT('Ctrl Pts',(181.875203730563,504.70043796528,-36.4917299682928)) ;
#61813=CARTESIAN_POINT('Ctrl Pts',(181.853342369544,504.696511686355,-36.4157416647703)) ;
#61814=CARTESIAN_POINT('Ctrl Pts',(181.766032252826,504.683632891777,-36.1671796841624)) ;
#61815=CARTESIAN_POINT('Ctrl Pts',(181.681762985447,504.674940800863,-36.0021987516026)) ;
#61816=CARTESIAN_POINT('Ctrl Pts',(181.546996452941,504.662706166569,-35.8080034781573)) ;
#61817=CARTESIAN_POINT('Ctrl Pts',(181.515778358693,504.659961892883,-35.7664732167796)) ;
#61818=CARTESIAN_POINT('Ctrl Pts',(181.449173072119,504.654252700115,-35.6845266298854)) ;
#61819=CARTESIAN_POINT('Ctrl Pts',(181.413707839674,504.651285662178,-35.6442261211981)) ;
#61820=CARTESIAN_POINT('Ctrl Pts',(181.330426191572,504.644463889159,-35.5567484845012)) ;
#61821=CARTESIAN_POINT('Ctrl Pts',(181.281793787348,504.640576592862,-35.5104356700513)) ;
#61822=CARTESIAN_POINT('Ctrl Pts',(181.12853432545,504.628641293187,-35.3781727513209)) ;
#61823=CARTESIAN_POINT('Ctrl Pts',(181.017606262631,504.620387003001,-35.30010048392)) ;
#61824=CARTESIAN_POINT('Ctrl Pts',(180.848201149098,504.608856792096,-35.2043208977969)) ;
#61825=CARTESIAN_POINT('Ctrl Pts',(180.79534571144,504.6053993151,-35.1773851168643)) ;
#61826=CARTESIAN_POINT('Ctrl Pts',(180.714440195643,504.600389570668,-35.1404737476219)) ;
#61827=CARTESIAN_POINT('Ctrl Pts',(180.687219932894,504.598750833435,-35.1287594286665)) ;
#61828=CARTESIAN_POINT('Ctrl Pts',(180.625958612455,504.595177921618,-35.103952062463)) ;
#61829=CARTESIAN_POINT('Ctrl Pts',(180.591804811688,504.593260290426,-35.0911686224346)) ;
#61830=CARTESIAN_POINT('Ctrl Pts',(180.514592305773,504.589052083592,-35.0645894294843)) ;
#61831=CARTESIAN_POINT('Ctrl Pts',(180.471381841536,504.586783267168,-35.0512919397479)) ;
#61832=CARTESIAN_POINT('Ctrl Pts',(180.314100324172,504.578721260657,-35.0085164763534)) ;
#61833=CARTESIAN_POINT('Ctrl Pts',(180.197984746224,504.573123677812,-34.9874338794217)) ;
#61834=CARTESIAN_POINT('Ctrl Pts',(179.989562315985,504.562884367147,-34.9678552236461)) ;
#61835=CARTESIAN_POINT('Ctrl Pts',(179.897963378539,504.558321740006,-34.9653943885215)) ;
#61836=CARTESIAN_POINT('Ctrl Pts',(179.755301446587,504.550909531777,-34.9710933981785)) ;
#61837=CARTESIAN_POINT('Ctrl Pts',(179.704190277625,504.548193738326,-34.9750541082729)) ;
#61838=CARTESIAN_POINT('Ctrl Pts',(179.598916875681,504.54244972914,-34.9871864247966)) ;
#61839=CARTESIAN_POINT('Ctrl Pts',(179.544826574092,504.539415056052,-34.9956209271563)) ;
#61840=CARTESIAN_POINT('Ctrl Pts',(179.425441148235,504.53252098311,-35.019154271756)) ;
#61841=CARTESIAN_POINT('Ctrl Pts',(179.360419218725,504.528632480622,-35.0353079012343)) ;
#61842=CARTESIAN_POINT('Ctrl Pts',(179.156270978218,504.516039286217,-35.0967552175052)) ;
#61843=CARTESIAN_POINT('Ctrl Pts',(179.021144422686,504.507088525318,-35.1537309963188)) ;
#61844=CARTESIAN_POINT('Ctrl Pts',(178.849805901742,504.495589521322,-35.2485997198334)) ;
#61845=CARTESIAN_POINT('Ctrl Pts',(178.807279082472,504.492725907566,-35.2742008342211)) ;
#61846=CARTESIAN_POINT('Ctrl Pts',(178.74132796563,504.48831890564,-35.3172324231881)) ;
#61847=CARTESIAN_POINT('Ctrl Pts',(178.717278624554,504.486720843645,-35.3336632704159)) ;
#61848=CARTESIAN_POINT('Ctrl Pts',(178.660466362811,504.482972048318,-35.3742766086214)) ;
#61849=CARTESIAN_POINT('Ctrl Pts',(178.628058559032,504.48085094912,-35.3989310153388)) ;
#61850=CARTESIAN_POINT('Ctrl Pts',(178.510467902888,504.473133906769,-35.4940357445329)) ;
#61851=CARTESIAN_POINT('Ctrl Pts',(178.430274201759,504.467821699576,-35.5703634924208)) ;
#61852=CARTESIAN_POINT('Ctrl Pts',(178.27277520858,504.45638458646,-35.7465568457832)) ;
#61853=CARTESIAN_POINT('Ctrl Pts',(178.197738689864,504.450263196797,-35.8478310884731)) ;
#61854=CARTESIAN_POINT('Ctrl Pts',(178.104869142975,504.44104583485,-36.0007007918042)) ;
#61855=CARTESIAN_POINT('Ctrl Pts',(178.079072130116,504.438252376895,-36.0471283913144)) ;
#61856=CARTESIAN_POINT('Ctrl Pts',(178.031434095232,504.432568707919,-36.1412800646791)) ;
#61857=CARTESIAN_POINT('Ctrl Pts',(178.00956564923,504.429682293223,-36.1889451226498)) ;
#61858=CARTESIAN_POINT('Ctrl Pts',(177.94729477266,504.420513207317,-36.3396281130938)) ;
#61859=CARTESIAN_POINT('Ctrl Pts',(177.913375173728,504.41402135162,-36.4450967596812)) ;
#61860=CARTESIAN_POINT('Ctrl Pts',(177.855400178598,504.398841192147,-36.6921708900916)) ;
#61861=CARTESIAN_POINT('Ctrl Pts',(177.837350195796,504.390100604637,-36.8346122735709)) ;
#61862=CARTESIAN_POINT('Ctrl Pts',(177.833519635185,504.379961133188,-37.0119064910454)) ;
#61863=CARTESIAN_POINT('Ctrl Pts',(177.83363286823,504.378043815694,-37.0460521233854)) ;
#61864=CARTESIAN_POINT('Ctrl Pts',(177.83547817841,504.374464050053,-37.1113756246714)) ;
#61865=CARTESIAN_POINT('Ctrl Pts',(177.837069933862,504.372795816064,-37.1425465031698)) ;
#61866=CARTESIAN_POINT('Ctrl Pts',(177.844791726139,504.367306501627,-37.2469830457464)) ;
#61867=CARTESIAN_POINT('Ctrl Pts',(177.854143340816,504.36363476977,-37.3199591266994)) ;
#61868=CARTESIAN_POINT('Ctrl Pts',(177.893866962334,504.35281746537,-37.5368793385124)) ;
#61869=CARTESIAN_POINT('Ctrl Pts',(177.935785576385,504.345869198863,-37.6782137245616)) ;
#61870=CARTESIAN_POINT('Ctrl Pts',(178.018009868928,504.335177442307,-37.8751369016024)) ;
#61871=CARTESIAN_POINT('Ctrl Pts',(178.046545225707,504.331778264457,-37.9351254848763)) ;
#61872=CARTESIAN_POINT('Ctrl Pts',(178.101343350485,504.325666389523,-38.0372571276467)) ;
#61873=CARTESIAN_POINT('Ctrl Pts',(178.126322274646,504.323001277131,-38.08002650189)) ;
#61874=CARTESIAN_POINT('Ctrl Pts',(178.18702404461,504.316764617251,-38.1758358404909)) ;
#61875=CARTESIAN_POINT('Ctrl Pts',(178.223725018205,504.31315764344,-38.2281920927415)) ;
#61876=CARTESIAN_POINT('Ctrl Pts',(178.310861191262,504.304933612228,-38.3409253500451)) ;
#61877=CARTESIAN_POINT('Ctrl Pts',(178.362443030331,504.300280441195,-38.4002882820591)) ;
#61878=CARTESIAN_POINT('Ctrl Pts',(178.513623239173,504.287309550931,-38.5553519931561)) ;
#61879=CARTESIAN_POINT('Ctrl Pts',(178.619663512684,504.278895790228,-38.6442039587384)) ;
#61880=CARTESIAN_POINT('Ctrl Pts',(178.762609281968,504.268994138379,-38.7413220174802)) ;
#61881=CARTESIAN_POINT('Ctrl Pts',(178.791900328897,504.267034818895,-38.76015282612)) ;
#61882=CARTESIAN_POINT('Ctrl Pts',(178.847840154085,504.263442816442,-38.7941380770124)) ;
#61883=CARTESIAN_POINT('Ctrl Pts',(178.874375218896,504.261801502184,-38.8094573120819)) ;
#61884=CARTESIAN_POINT('Ctrl Pts',(178.96030286957,504.256654423801,-38.8565350906304)) ;
#61885=CARTESIAN_POINT('Ctrl Pts',(179.020922335966,504.253272027075,-38.8859721620507)) ;
#61886=CARTESIAN_POINT('Ctrl Pts',(179.211230834465,504.24308241426,-38.9670849493294)) ;
#61887=CARTESIAN_POINT('Ctrl Pts',(179.344816204064,504.236492319199,-39.0085747583076)) ;
#61888=CARTESIAN_POINT('Ctrl Pts',(179.554135230827,504.225900001773,-39.0508688107427)) ;
#61889=CARTESIAN_POINT('Ctrl Pts',(179.627425372828,504.222148885058,-39.0615966499812)) ;
#61890=CARTESIAN_POINT('Ctrl Pts',(179.750587587933,504.215671034999,-39.0728763037185)) ;
#61891=CARTESIAN_POINT('Ctrl Pts',(179.800189524387,504.213016184586,-39.075610900755)) ;
#61892=CARTESIAN_POINT('Ctrl Pts',(179.908396181734,504.207103240459,-39.0776486663926)) ;
#61893=CARTESIAN_POINT('Ctrl Pts',(179.966968790785,504.203824794166,-39.076247243386)) ;
#61894=CARTESIAN_POINT('Ctrl Pts',(180.092828594785,504.196606627187,-39.0678448660369)) ;
#61895=CARTESIAN_POINT('Ctrl Pts',(180.159991247105,504.192646753089,-39.0600195915755)) ;
#61896=CARTESIAN_POINT('Ctrl Pts',(180.362318746089,504.180447566007,-39.02626597024)) ;
#61897=CARTESIAN_POINT('Ctrl Pts',(180.495375183035,504.172030998369,-38.9900659627336)) ;
#61898=CARTESIAN_POINT('Ctrl Pts',(180.668181903654,504.161180978865,-38.9238421250475)) ;
#61899=CARTESIAN_POINT('Ctrl Pts',(180.711949044893,504.158443621116,-38.9053045910474)) ;
#61900=CARTESIAN_POINT('Ctrl Pts',(180.781409624588,504.154161161521,-38.8729992385101)) ;
#61901=CARTESIAN_POINT('Ctrl Pts',(180.807517941004,504.15256793519,-38.8601755591509)) ;
#61902=CARTESIAN_POINT('Ctrl Pts',(180.871116499867,504.148727728224,-38.8272433925758)) ;
#61903=CARTESIAN_POINT('Ctrl Pts',(180.908269665468,504.146515743246,-38.8065180416558)) ;
#61904=CARTESIAN_POINT('Ctrl Pts',(180.993837159418,504.141434216021,-38.7552391119479)) ;
#61905=CARTESIAN_POINT('Ctrl Pts',(181.04167168088,504.138603296537,-38.7237862290604)) ;
#61906=CARTESIAN_POINT('Ctrl Pts',(181.210378483855,504.128435505628,-38.6024700488032)) ;
#61907=CARTESIAN_POINT('Ctrl Pts',(181.322585764394,504.121276173305,-38.5013983472221)) ;
#61908=CARTESIAN_POINT('Ctrl Pts',(181.455800306384,504.111119709196,-38.3518682265149)) ;
#61909=CARTESIAN_POINT('Ctrl Pts',(181.487498334288,504.108555055911,-38.3135777294949)) ;
#61910=CARTESIAN_POINT('Ctrl Pts',(181.517775728527,504.105934865979,-38.2741778157906)) ;
#61911=CARTESIAN_POINT('Origin',(179.888527625407,535.710565160536,-48.5221601717598)) ;
#61912=CARTESIAN_POINT('Ctrl Pts',(181.451956083968,536.286106171205,-48.8631290382246)) ;
#61913=CARTESIAN_POINT('Ctrl Pts',(181.445401841449,536.303910444207,-48.8618925414681)) ;
#61914=CARTESIAN_POINT('Ctrl Pts',(181.438543835126,536.321601758001,-48.8606411710218)) ;
#61915=CARTESIAN_POINT('Ctrl Pts',(181.41945812941,536.368445833857,-48.8572568591724)) ;
#61916=CARTESIAN_POINT('Ctrl Pts',(181.406702462457,536.397369164468,-48.8550902797562)) ;
#61917=CARTESIAN_POINT('Ctrl Pts',(181.343426241339,536.530460296774,-48.8448105556143)) ;
#61918=CARTESIAN_POINT('Ctrl Pts',(181.282959873888,536.629539463379,-48.8362823401656)) ;
#61919=CARTESIAN_POINT('Ctrl Pts',(181.171658204911,536.775323279961,-48.8229818495332)) ;
#61920=CARTESIAN_POINT('Ctrl Pts',(181.127358346787,536.826555328311,-48.8181274957693)) ;
#61921=CARTESIAN_POINT('Ctrl Pts',(181.039987027751,536.915963358886,-48.8093647000216)) ;
#61922=CARTESIAN_POINT('Ctrl Pts',(180.997819204767,536.954879094015,-48.8054300663977)) ;
#61923=CARTESIAN_POINT('Ctrl Pts',(180.914350770737,537.024286967429,-48.798156968782)) ;
#61924=CARTESIAN_POINT('Ctrl Pts',(180.873486662309,537.055196989528,-48.7948033931466)) ;
#61925=CARTESIAN_POINT('Ctrl Pts',(180.715645399245,537.163525867764,-48.7825128141501)) ;
#61926=CARTESIAN_POINT('Ctrl Pts',(180.590480353423,537.227958858901,-48.7741053222124)) ;
#61927=CARTESIAN_POINT('Ctrl Pts',(180.410704605132,537.29344170527,-48.762355655858)) ;
#61928=CARTESIAN_POINT('Ctrl Pts',(180.361917082431,537.308710533985,-48.7591900680543)) ;
#61929=CARTESIAN_POINT('Ctrl Pts',(180.275541773772,537.331440621175,-48.7535062333762)) ;
#61930=CARTESIAN_POINT('Ctrl Pts',(180.238254393896,537.339892570055,-48.7510272515709)) ;
#61931=CARTESIAN_POINT('Ctrl Pts',(180.170299363026,537.352856047998,-48.7464093436077)) ;
#61932=CARTESIAN_POINT('Ctrl Pts',(180.139735210229,537.357807947996,-48.74429300956)) ;
#61933=CARTESIAN_POINT('Ctrl Pts',(179.987727526603,537.378107754513,-48.7336211306909)) ;
#61934=CARTESIAN_POINT('Ctrl Pts',(179.864992040077,537.380889079062,-48.7245850571382)) ;
#61935=CARTESIAN_POINT('Ctrl Pts',(179.677579684228,537.364463130775,-48.7109590783032)) ;
#61936=CARTESIAN_POINT('Ctrl Pts',(179.612484000194,537.354851945904,-48.7062521308366)) ;
#61937=CARTESIAN_POINT('Ctrl Pts',(179.492811896352,537.329872854313,-48.6976972489222)) ;
#61938=CARTESIAN_POINT('Ctrl Pts',(179.438121068129,537.315521117356,-48.6938264852776)) ;
#61939=CARTESIAN_POINT('Ctrl Pts',(179.33514120235,537.282816849689,-48.6865971965219)) ;
#61940=CARTESIAN_POINT('Ctrl Pts',(179.286769577754,537.264946104945,-48.6832272746554)) ;
#61941=CARTESIAN_POINT('Ctrl Pts',(179.115251273482,537.192369101227,-48.671288502312)) ;
#61942=CARTESIAN_POINT('Ctrl Pts',(178.998028122189,537.125030674743,-48.6631930146316)) ;
#61943=CARTESIAN_POINT('Ctrl Pts',(178.847759472658,537.012550643929,-48.6516808887462)) ;
#61944=CARTESIAN_POINT('Ctrl Pts',(178.806875249398,536.978789074268,-48.6484047620819)) ;
#61945=CARTESIAN_POINT('Ctrl Pts',(178.738765680519,536.916852876371,-48.6425563659384)) ;
#61946=CARTESIAN_POINT('Ctrl Pts',(178.71079555728,536.889560130116,-48.6400268733404)) ;
#61947=CARTESIAN_POINT('Ctrl Pts',(178.662632282902,536.8391381328,-48.6353781704473)) ;
#61948=CARTESIAN_POINT('Ctrl Pts',(178.642071541905,536.816387463089,-48.6332852885324)) ;
#61949=CARTESIAN_POINT('Ctrl Pts',(178.549411150272,536.707989706724,-48.6233743524902)) ;
#61950=CARTESIAN_POINT('Ctrl Pts',(178.485437852139,536.615785632238,-48.6151467179976)) ;
#61951=CARTESIAN_POINT('Ctrl Pts',(178.396802099555,536.455782669324,-48.6018597914381)) ;
#61952=CARTESIAN_POINT('Ctrl Pts',(178.366406883428,536.391553010678,-48.5967507811819)) ;
#61953=CARTESIAN_POINT('Ctrl Pts',(178.31851456452,536.270980796986,-48.5876322998191)) ;
#61954=CARTESIAN_POINT('Ctrl Pts',(178.299730034168,536.215273403371,-48.5835905679914)) ;
#61955=CARTESIAN_POINT('Ctrl Pts',(178.270432344023,536.110365552277,-48.5762775624481)) ;
#61956=CARTESIAN_POINT('Ctrl Pts',(178.259126820571,536.061459177897,-48.5729833740857)) ;
#61957=CARTESIAN_POINT('Ctrl Pts',(178.232962589701,535.919293550546,-48.5636769772334)) ;
#61958=CARTESIAN_POINT('Ctrl Pts',(178.223796957473,535.825186275962,-48.557853867868)) ;
#61959=CARTESIAN_POINT('Ctrl Pts',(178.221376978864,535.625950363706,-48.5456708139611)) ;
#61960=CARTESIAN_POINT('Ctrl Pts',(178.230005028246,535.521226599191,-48.53934884585)) ;
#61961=CARTESIAN_POINT('Ctrl Pts',(178.254756245185,535.382461903842,-48.5303373125597)) ;
#61962=CARTESIAN_POINT('Ctrl Pts',(178.262252961617,535.347122083389,-48.5279841224477)) ;
#61963=CARTESIAN_POINT('Ctrl Pts',(178.278538014051,535.281017240628,-48.5234239778264)) ;
#61964=CARTESIAN_POINT('Ctrl Pts',(178.287075476337,535.25020836675,-48.5212299604185)) ;
#61965=CARTESIAN_POINT('Ctrl Pts',(178.30774854546,535.183163191395,-48.5163301324382)) ;
#61966=CARTESIAN_POINT('Ctrl Pts',(178.320256251134,535.147058456146,-48.5136097353657)) ;
#61967=CARTESIAN_POINT('Ctrl Pts',(178.366486174142,535.027111182489,-48.5043603339154)) ;
#61968=CARTESIAN_POINT('Ctrl Pts',(178.405783940426,534.945587344092,-48.4977266488301)) ;
#61969=CARTESIAN_POINT('Ctrl Pts',(178.493675145285,534.795747387831,-48.4851855682641)) ;
#61970=CARTESIAN_POINT('Ctrl Pts',(178.541193720555,534.727101837503,-48.4792784118901)) ;
#61971=CARTESIAN_POINT('Ctrl Pts',(178.625345330398,534.62315430444,-48.4701100576345)) ;
#61972=CARTESIAN_POINT('Ctrl Pts',(178.658791882695,534.585468346556,-48.4667301383124)) ;
#61973=CARTESIAN_POINT('Ctrl Pts',(178.736071673144,534.505964667386,-48.4594429830431)) ;
#61974=CARTESIAN_POINT('Ctrl Pts',(178.780580798885,534.464903785589,-48.4555728702336)) ;
#61975=CARTESIAN_POINT('Ctrl Pts',(178.958787414233,534.317630590756,-48.4410694757553)) ;
#61976=CARTESIAN_POINT('Ctrl Pts',(179.10624318588,534.229789053832,-48.4311323402834)) ;
#61977=CARTESIAN_POINT('Ctrl Pts',(179.29526323438,534.153420779713,-48.4180006057553)) ;
#61978=CARTESIAN_POINT('Ctrl Pts',(179.32645130277,534.141893394678,-48.4158186048797)) ;
#61979=CARTESIAN_POINT('Ctrl Pts',(179.390488483832,534.120379481555,-48.4112673043479)) ;
#61980=CARTESIAN_POINT('Ctrl Pts',(179.423343033481,534.11046006711,-48.4088962401272)) ;
#61981=CARTESIAN_POINT('Ctrl Pts',(179.557139774496,534.074532848963,-48.3991601142111)) ;
#61982=CARTESIAN_POINT('Ctrl Pts',(179.660110853324,534.057010448843,-48.3915011029027)) ;
#61983=CARTESIAN_POINT('Ctrl Pts',(179.862707993671,534.041829151286,-48.3767506686075)) ;
#61984=CARTESIAN_POINT('Ctrl Pts',(179.961854862796,534.04323927891,-48.3696797205071)) ;
#61985=CARTESIAN_POINT('Ctrl Pts',(180.110228486116,534.058619666808,-48.3594307531145)) ;
#61986=CARTESIAN_POINT('Ctrl Pts',(180.159897218995,534.066048611531,-48.3560535462152)) ;
#61987=CARTESIAN_POINT('Ctrl Pts',(180.266667645582,534.08698870835,-48.3488844496936)) ;
#61988=CARTESIAN_POINT('Ctrl Pts',(180.323544845949,534.101294624443,-48.3451234572799)) ;
#61989=CARTESIAN_POINT('Ctrl Pts',(180.447084181674,534.13939855112,-48.3369868187775)) ;
#61990=CARTESIAN_POINT('Ctrl Pts',(180.513222545071,534.164503324822,-48.3326533681225)) ;
#61991=CARTESIAN_POINT('Ctrl Pts',(180.680225631726,534.240366806741,-48.3214482268071)) ;
#61992=CARTESIAN_POINT('Ctrl Pts',(180.777867842923,534.297293941667,-48.3146381713659)) ;
#61993=CARTESIAN_POINT('Ctrl Pts',(180.893743191954,534.381642909102,-48.3053136498849)) ;
#61994=CARTESIAN_POINT('Ctrl Pts',(180.917981307947,534.400329422626,-48.3032841039066)) ;
#61995=CARTESIAN_POINT('Ctrl Pts',(180.972107525708,534.444488057351,-48.2985389957307)) ;
#61996=CARTESIAN_POINT('Ctrl Pts',(181.00163143216,534.470365211504,-48.2957998556565)) ;
#61997=CARTESIAN_POINT('Ctrl Pts',(181.069101746028,534.533852611671,-48.2892279578467)) ;
#61998=CARTESIAN_POINT('Ctrl Pts',(181.106208234236,534.572294134727,-48.2853613355198)) ;
#61999=CARTESIAN_POINT('Ctrl Pts',(181.229501700653,534.712963394802,-48.2717564119641)) ;
#62000=CARTESIAN_POINT('Ctrl Pts',(181.305202518358,534.823736110179,-48.2620257177712)) ;
#62001=CARTESIAN_POINT('Ctrl Pts',(181.39066097337,534.988196008883,-48.2492352804052)) ;
#62002=CARTESIAN_POINT('Ctrl Pts',(181.412327276743,535.035096845546,-48.2457464992169)) ;
#62003=CARTESIAN_POINT('Ctrl Pts',(181.453019193062,535.13515229458,-48.2386040333602)) ;
#62004=CARTESIAN_POINT('Ctrl Pts',(181.471593911735,535.188419461946,-48.2349695293695)) ;
#62005=CARTESIAN_POINT('Ctrl Pts',(181.505816833914,535.305332469606,-48.2272682045055)) ;
#62006=CARTESIAN_POINT('Ctrl Pts',(181.520485072712,535.369165421784,-48.2232332206311)) ;
#62007=CARTESIAN_POINT('Ctrl Pts',(181.55186846701,535.555384353464,-48.2116735151591)) ;
#62008=CARTESIAN_POINT('Ctrl Pts',(181.558789752985,535.678953015432,-48.2042749395757)) ;
#62009=CARTESIAN_POINT('Ctrl Pts',(181.550311947402,535.832969013319,-48.194252299259)) ;
#62010=CARTESIAN_POINT('Ctrl Pts',(181.547757461034,535.863751558768,-48.192206796657)) ;
#62011=CARTESIAN_POINT('Ctrl Pts',(181.540088429022,535.932810408178,-48.1874920233069)) ;
#62012=CARTESIAN_POINT('Ctrl Pts',(181.534496277019,535.971012136138,-48.1848018162824)) ;
#62013=CARTESIAN_POINT('Ctrl Pts',(181.51039947183,536.103364346698,-48.1752708839214)) ;
#62014=CARTESIAN_POINT('Ctrl Pts',(181.485096229393,536.196082005249,-48.1682298305151)) ;
#62015=CARTESIAN_POINT('Ctrl Pts',(181.451957355136,536.286102718128,-48.1612691418708)) ;
#62016=CARTESIAN_POINT('Ctrl Pts',(181.451956072328,536.286106202824,-49.0537499415271)) ;
#62017=CARTESIAN_POINT('Ctrl Pts',(181.444652999706,536.305944634229,-49.0524601164881)) ;
#62018=CARTESIAN_POINT('Ctrl Pts',(181.436969948344,536.325650536645,-49.0511716725108)) ;
#62019=CARTESIAN_POINT('Ctrl Pts',(181.401722665985,536.411200822763,-49.0455280065106)) ;
#62020=CARTESIAN_POINT('Ctrl Pts',(181.370324467744,536.475370143754,-49.0411597533643)) ;
#62021=CARTESIAN_POINT('Ctrl Pts',(181.305647465685,536.588519950892,-49.0329685862384)) ;
#62022=CARTESIAN_POINT('Ctrl Pts',(181.273690047954,536.638119483931,-49.0291894357721)) ;
#62023=CARTESIAN_POINT('Ctrl Pts',(181.209813010097,536.726575040688,-49.0220066308013)) ;
#62024=CARTESIAN_POINT('Ctrl Pts',(181.178634484178,536.765882404595,-49.0186354002201)) ;
#62025=CARTESIAN_POINT('Ctrl Pts',(181.085945636468,536.872481132761,-49.0089363043924)) ;
#62026=CARTESIAN_POINT('Ctrl Pts',(181.020626926734,536.936209896215,-49.0024509014762)) ;
#62027=CARTESIAN_POINT('Ctrl Pts',(180.868614765786,537.061957551611,-48.9881600908592)) ;
#62028=CARTESIAN_POINT('Ctrl Pts',(180.780507366938,537.121666028037,-48.980342893649)) ;
#62029=CARTESIAN_POINT('Ctrl Pts',(180.65463160926,537.190439372448,-48.970204552058)) ;
#62030=CARTESIAN_POINT('Ctrl Pts',(180.621356086709,537.207196714229,-48.9676152587733)) ;
#62031=CARTESIAN_POINT('Ctrl Pts',(180.558838462443,537.236094385003,-48.9629524177518)) ;
#62032=CARTESIAN_POINT('Ctrl Pts',(180.529760797672,537.248543118926,-48.9608641801791)) ;
#62033=CARTESIAN_POINT('Ctrl Pts',(180.391697573253,537.303053895975,-48.9512479597624)) ;
#62034=CARTESIAN_POINT('Ctrl Pts',(180.27882477886,537.334411235509,-48.9442228422084)) ;
#62035=CARTESIAN_POINT('Ctrl Pts',(180.096912622584,537.364863107974,-48.9329483632415)) ;
#62036=CARTESIAN_POINT('Ctrl Pts',(180.029624869013,537.371955112813,-48.9287911807169)) ;
#62037=CARTESIAN_POINT('Ctrl Pts',(179.90470500665,537.377476825306,-48.9209023403871)) ;
#62038=CARTESIAN_POINT('Ctrl Pts',(179.847227053245,537.37704325759,-48.9172064998977)) ;
#62039=CARTESIAN_POINT('Ctrl Pts',(179.738370101123,537.370586985611,-48.9100060099322)) ;
#62040=CARTESIAN_POINT('Ctrl Pts',(179.687024674893,537.365139205087,-48.9065242777309)) ;
#62041=CARTESIAN_POINT('Ctrl Pts',(179.500305910478,537.336508301739,-48.8935053166676)) ;
#62042=CARTESIAN_POINT('Ctrl Pts',(179.367707059889,537.299004414284,-48.8835069489898)) ;
#62043=CARTESIAN_POINT('Ctrl Pts',(179.193147628988,537.225400735127,-48.8697376387081)) ;
#62044=CARTESIAN_POINT('Ctrl Pts',(179.146031075378,537.20287199927,-48.8659626691381)) ;
#62045=CARTESIAN_POINT('Ctrl Pts',(179.065899411207,537.159820659145,-48.8595178109888)) ;
#62046=CARTESIAN_POINT('Ctrl Pts',(179.032398413199,537.14028613622,-48.8568157003346)) ;
#62047=CARTESIAN_POINT('Ctrl Pts',(178.973261105123,537.102977998372,-48.8520719412159)) ;
#62048=CARTESIAN_POINT('Ctrl Pts',(178.947387077376,537.085621851242,-48.8500095409117)) ;
#62049=CARTESIAN_POINT('Ctrl Pts',(178.834923491124,537.005519484749,-48.8410421838967)) ;
#62050=CARTESIAN_POINT('Ctrl Pts',(178.753994818018,536.935240637472,-48.8345618743026)) ;
#62051=CARTESIAN_POINT('Ctrl Pts',(178.630138063676,536.804791151174,-48.8235765835784)) ;
#62052=CARTESIAN_POINT('Ctrl Pts',(178.583451858269,536.748664888205,-48.8191130998566)) ;
#62053=CARTESIAN_POINT('Ctrl Pts',(178.505516622669,536.641370883671,-48.8107782544506)) ;
#62054=CARTESIAN_POINT('Ctrl Pts',(178.473062448466,536.591232938511,-48.8069534916042)) ;
#62055=CARTESIAN_POINT('Ctrl Pts',(178.418293457785,536.495745312112,-48.7997066121985)) ;
#62056=CARTESIAN_POINT('Ctrl Pts',(178.39521601073,536.450913618259,-48.7963186085098)) ;
#62057=CARTESIAN_POINT('Ctrl Pts',(178.336353782971,536.322575784734,-48.7866241266458)) ;
#62058=CARTESIAN_POINT('Ctrl Pts',(178.305316414915,536.237099286703,-48.7801631208431)) ;
#62059=CARTESIAN_POINT('Ctrl Pts',(178.253256203703,536.046498800338,-48.7658526358325)) ;
#62060=CARTESIAN_POINT('Ctrl Pts',(178.235086652117,535.940995749693,-48.7579883362068)) ;
#62061=CARTESIAN_POINT('Ctrl Pts',(178.224362427726,535.797207742188,-48.7477950802033)) ;
#62062=CARTESIAN_POINT('Ctrl Pts',(178.222837322931,535.75985133355,-48.745196186547)) ;
#62063=CARTESIAN_POINT('Ctrl Pts',(178.222343869998,535.69080745543,-48.7405208954119)) ;
#62064=CARTESIAN_POINT('Ctrl Pts',(178.223020334068,535.659142554616,-48.7384295397676)) ;
#62065=CARTESIAN_POINT('Ctrl Pts',(178.230404250324,535.511204908019,-48.7288318244825)) ;
#62066=CARTESIAN_POINT('Ctrl Pts',(178.248389465455,535.395808185701,-48.7218240282482)) ;
#62067=CARTESIAN_POINT('Ctrl Pts',(178.295612571426,535.217869548388,-48.7105663841804)) ;
#62068=CARTESIAN_POINT('Ctrl Pts',(178.316916691311,535.153640201641,-48.7064072989536)) ;
#62069=CARTESIAN_POINT('Ctrl Pts',(178.36342938303,535.037563497842,-48.698515865777)) ;
#62070=CARTESIAN_POINT('Ctrl Pts',(178.387537498471,534.985387040199,-48.6948193333161)) ;
#62071=CARTESIAN_POINT('Ctrl Pts',(178.438341439578,534.888870314242,-48.6876157633278)) ;
#62072=CARTESIAN_POINT('Ctrl Pts',(178.464502047986,534.844324712763,-48.684131552719)) ;
#62073=CARTESIAN_POINT('Ctrl Pts',(178.569907934526,534.682553841477,-48.6708215229749)) ;
#62074=CARTESIAN_POINT('Ctrl Pts',(178.661897798574,534.574374419796,-48.660498575176)) ;
#62075=CARTESIAN_POINT('Ctrl Pts',(178.803485296674,534.445355900407,-48.6465828522548)) ;
#62076=CARTESIAN_POINT('Ctrl Pts',(178.842065012611,534.413264898068,-48.6429605774959)) ;
#62077=CARTESIAN_POINT('Ctrl Pts',(178.912190338064,534.360101021607,-48.6367340936556)) ;
#62078=CARTESIAN_POINT('Ctrl Pts',(178.94311786213,534.338271877889,-48.634100274279)) ;
#62079=CARTESIAN_POINT('Ctrl Pts',(179.001047698554,534.300273216161,-48.6294055322539)) ;
#62080=CARTESIAN_POINT('Ctrl Pts',(179.027813286086,534.283780331266,-48.6273275451756)) ;
#62081=CARTESIAN_POINT('Ctrl Pts',(179.157917175369,534.20860507297,-48.6175823518427)) ;
#62082=CARTESIAN_POINT('Ctrl Pts',(179.266883086093,534.160325895569,-48.610440547418)) ;
#62083=CARTESIAN_POINT('Ctrl Pts',(179.443825287085,534.103618447951,-48.5990757277951)) ;
#62084=CARTESIAN_POINT('Ctrl Pts',(179.508748118981,534.08704908744,-48.5949546844974)) ;
#62085=CARTESIAN_POINT('Ctrl Pts',(179.63063155382,534.063654758555,-48.5871182169442)) ;
#62086=CARTESIAN_POINT('Ctrl Pts',(179.687286753632,534.055776605915,-48.583437285437)) ;
#62087=CARTESIAN_POINT('Ctrl Pts',(179.795814145927,534.046341244903,-48.5762393202312)) ;
#62088=CARTESIAN_POINT('Ctrl Pts',(179.847573567845,534.044264241712,-48.5727437584416)) ;
#62089=CARTESIAN_POINT('Ctrl Pts',(180.034568195186,534.045477986089,-48.5598464440853)) ;
#62090=CARTESIAN_POINT('Ctrl Pts',(180.169163967346,534.062817256202,-48.5500025875058)) ;
#62091=CARTESIAN_POINT('Ctrl Pts',(180.351477600845,534.109303564848,-48.5363217538065)) ;
#62092=CARTESIAN_POINT('Ctrl Pts',(180.402151257672,534.124831001583,-48.5324880718608)) ;
#62093=CARTESIAN_POINT('Ctrl Pts',(180.488803868579,534.155973967457,-48.5259596796516)) ;
#62094=CARTESIAN_POINT('Ctrl Pts',(180.525132849965,534.170493810251,-48.5232317045762)) ;
#62095=CARTESIAN_POINT('Ctrl Pts',(180.589251907854,534.198778027206,-48.5184743512113)) ;
#62096=CARTESIAN_POINT('Ctrl Pts',(180.617229312525,534.212062967201,-48.516422586656)) ;
#62097=CARTESIAN_POINT('Ctrl Pts',(180.742393017326,534.275831332575,-48.5072931253819)) ;
#62098=CARTESIAN_POINT('Ctrl Pts',(180.834839625239,534.335047927997,-48.5006664165278)) ;
#62099=CARTESIAN_POINT('Ctrl Pts',(180.977346854394,534.447546447001,-48.4895790086613)) ;
#62100=CARTESIAN_POINT('Ctrl Pts',(181.03092297632,534.495791339069,-48.485168003849)) ;
#62101=CARTESIAN_POINT('Ctrl Pts',(181.122620489224,534.589811388457,-48.4769093360181)) ;
#62102=CARTESIAN_POINT('Ctrl Pts',(181.161732696112,534.634450968694,-48.4731064116664)) ;
#62103=CARTESIAN_POINT('Ctrl Pts',(181.229560756722,534.720750794004,-48.4658773324031)) ;
#62104=CARTESIAN_POINT('Ctrl Pts',(181.258920868448,534.761816651075,-48.462483822048)) ;
#62105=CARTESIAN_POINT('Ctrl Pts',(181.341294615768,534.888850300523,-48.4520836994211)) ;
#62106=CARTESIAN_POINT('Ctrl Pts',(181.388397610983,534.978355510868,-48.4448672258863)) ;
#62107=CARTESIAN_POINT('Ctrl Pts',(181.45648639386,535.142297088654,-48.4319750445597)) ;
#62108=CARTESIAN_POINT('Ctrl Pts',(181.480953159586,535.214979947161,-48.4263675132201)) ;
#62109=CARTESIAN_POINT('Ctrl Pts',(181.512473276413,535.335519004315,-48.4174345830246)) ;
#62110=CARTESIAN_POINT('Ctrl Pts',(181.522603784557,535.382456640829,-48.4140444255247)) ;
#62111=CARTESIAN_POINT('Ctrl Pts',(181.535686926608,535.458970665944,-48.4087253486124)) ;
#62112=CARTESIAN_POINT('Ctrl Pts',(181.539899835167,535.488295862052,-48.4067387604865)) ;
#62113=CARTESIAN_POINT('Ctrl Pts',(181.549578645045,535.571351609852,-48.4012463685222)) ;
#62114=CARTESIAN_POINT('Ctrl Pts',(181.553218199038,535.625256866763,-48.3978298650265)) ;
#62115=CARTESIAN_POINT('Ctrl Pts',(181.556289051666,535.788596880453,-48.3876709276972)) ;
#62116=CARTESIAN_POINT('Ctrl Pts',(181.54757277394,535.897882975501,-48.3811197798381)) ;
#62117=CARTESIAN_POINT('Ctrl Pts',(181.515501205169,536.076165957159,-48.3699036379122)) ;
#62118=CARTESIAN_POINT('Ctrl Pts',(181.498244779974,536.145899165917,-48.3653807724651)) ;
#62119=CARTESIAN_POINT('Ctrl Pts',(181.468896035144,536.238421419071,-48.3590621823926)) ;
#62120=CARTESIAN_POINT('Ctrl Pts',(181.460696278165,536.262363870131,-48.3573978200419)) ;
#62121=CARTESIAN_POINT('Ctrl Pts',(181.451956078709,536.28610618549,-48.355715363061)) ;
#62122=CARTESIAN_POINT('Origin',(179.888527625416,585.710565160536,-48.5221601717598)) ;
#62123=CARTESIAN_POINT('Ctrl Pts',(181.45195815568,586.286100543496,-48.8631342200737)) ;
#62124=CARTESIAN_POINT('Ctrl Pts',(181.445395417149,586.303928093434,-48.8618961238889)) ;
#62125=CARTESIAN_POINT('Ctrl Pts',(181.438528122193,586.321642385202,-48.8606431156781)) ;
#62126=CARTESIAN_POINT('Ctrl Pts',(181.419427296626,586.368518069373,-48.8572563811899)) ;
#62127=CARTESIAN_POINT('Ctrl Pts',(181.406666054341,586.39745010849,-48.8550890352828)) ;
#62128=CARTESIAN_POINT('Ctrl Pts',(181.343417378162,586.530462932121,-48.8448147933775)) ;
#62129=CARTESIAN_POINT('Ctrl Pts',(181.283002087658,586.629463725066,-48.8362937062396)) ;
#62130=CARTESIAN_POINT('Ctrl Pts',(181.171755641747,586.775207597148,-48.8229978111714)) ;
#62131=CARTESIAN_POINT('Ctrl Pts',(181.127441967481,586.826464164859,-48.8181413755912)) ;
#62132=CARTESIAN_POINT('Ctrl Pts',(181.040047552031,586.915906154756,-48.8093755878045)) ;
#62133=CARTESIAN_POINT('Ctrl Pts',(180.99787200679,586.954832615455,-48.8054399988221)) ;
#62134=CARTESIAN_POINT('Ctrl Pts',(180.914395907013,587.024251727405,-48.7981659313724)) ;
#62135=CARTESIAN_POINT('Ctrl Pts',(180.873532736041,587.055163244635,-48.7948123002097)) ;
#62136=CARTESIAN_POINT('Ctrl Pts',(180.715655128551,587.163525002694,-48.7825184509087)) ;
#62137=CARTESIAN_POINT('Ctrl Pts',(180.590445938783,587.227979253165,-48.774108240018)) ;
#62138=CARTESIAN_POINT('Ctrl Pts',(180.410634822879,587.293464258157,-48.762356370403)) ;
#62139=CARTESIAN_POINT('Ctrl Pts',(180.361860493631,587.308726833761,-48.7591916229672)) ;
#62140=CARTESIAN_POINT('Ctrl Pts',(180.275504485808,587.331449378907,-48.7535090170231)) ;
#62141=CARTESIAN_POINT('Ctrl Pts',(180.238222929237,587.33989917927,-48.751030397237)) ;
#62142=CARTESIAN_POINT('Ctrl Pts',(180.170269341545,587.352861282907,-48.7464125459367)) ;
#62143=CARTESIAN_POINT('Ctrl Pts',(180.139700671585,587.357813298877,-48.7442958734795)) ;
#62144=CARTESIAN_POINT('Ctrl Pts',(179.987725477292,587.378105106976,-48.7336261613859)) ;
#62145=CARTESIAN_POINT('Ctrl Pts',(179.865028084288,587.380886821715,-48.7245929831802)) ;
#62146=CARTESIAN_POINT('Ctrl Pts',(179.677640701921,587.36447138691,-48.7109687723047)) ;
#62147=CARTESIAN_POINT('Ctrl Pts',(179.612532850842,587.3548606239,-48.7062609154197)) ;
#62148=CARTESIAN_POINT('Ctrl Pts',(179.492842393294,587.329880523963,-48.6977046826171)) ;
#62149=CARTESIAN_POINT('Ctrl Pts',(179.43814528453,587.315528132511,-48.6938334596435)) ;
#62150=CARTESIAN_POINT('Ctrl Pts',(179.335158039324,587.282822812466,-48.6866036349422)) ;
#62151=CARTESIAN_POINT('Ctrl Pts',(179.286785175313,587.26495218045,-48.683233620141)) ;
#62152=CARTESIAN_POINT('Ctrl Pts',(179.115253043243,587.192371220558,-48.671293872118)) ;
#62153=CARTESIAN_POINT('Ctrl Pts',(178.998018526856,587.125025886462,-48.663197625617)) ;
#62154=CARTESIAN_POINT('Ctrl Pts',(178.84774373324,587.012537920548,-48.6516848633598)) ;
#62155=CARTESIAN_POINT('Ctrl Pts',(178.806862571575,586.978778116054,-48.6484089329801)) ;
#62156=CARTESIAN_POINT('Ctrl Pts',(178.738756907588,586.916844477785,-48.6425607993073)) ;
#62157=CARTESIAN_POINT('Ctrl Pts',(178.710787785175,586.889552328761,-48.6400313659057)) ;
#62158=CARTESIAN_POINT('Ctrl Pts',(178.662623663881,586.839128846284,-48.6353825280805)) ;
#62159=CARTESIAN_POINT('Ctrl Pts',(178.642061242138,586.816375930667,-48.6332894402456)) ;
#62160=CARTESIAN_POINT('Ctrl Pts',(178.549416667474,586.707994274046,-48.6233800000476)) ;
#62161=CARTESIAN_POINT('Ctrl Pts',(178.485456818061,586.615811900013,-48.6151542993375)) ;
#62162=CARTESIAN_POINT('Ctrl Pts',(178.396822941643,586.455825344801,-48.6018684335083)) ;
#62163=CARTESIAN_POINT('Ctrl Pts',(178.366421779789,586.391587352801,-48.596758660419)) ;
#62164=CARTESIAN_POINT('Ctrl Pts',(178.318521859579,586.271001776633,-48.5876390544956)) ;
#62165=CARTESIAN_POINT('Ctrl Pts',(178.299735014943,586.21528968548,-48.5835969449305)) ;
#62166=CARTESIAN_POINT('Ctrl Pts',(178.270434656485,586.11037515806,-48.5762834346059)) ;
#62167=CARTESIAN_POINT('Ctrl Pts',(178.259128428237,586.061466924438,-48.5729891081358)) ;
#62168=CARTESIAN_POINT('Ctrl Pts',(178.232963221671,585.919298844015,-48.5636825260079)) ;
#62169=CARTESIAN_POINT('Ctrl Pts',(178.223797245764,585.825190974939,-48.557859367918)) ;
#62170=CARTESIAN_POINT('Ctrl Pts',(178.22137675862,585.625953374547,-48.5456761923845)) ;
#62171=CARTESIAN_POINT('Ctrl Pts',(178.230004741034,585.521228521675,-48.5393541532479)) ;
#62172=CARTESIAN_POINT('Ctrl Pts',(178.254756216032,585.382461959764,-48.5303424845386)) ;
#62173=CARTESIAN_POINT('Ctrl Pts',(178.26225310819,585.347121347018,-48.5279892366432)) ;
#62174=CARTESIAN_POINT('Ctrl Pts',(178.278538896352,585.281013784409,-48.5234288901615)) ;
#62175=CARTESIAN_POINT('Ctrl Pts',(178.287076979221,585.250202999452,-48.5212347256081)) ;
#62176=CARTESIAN_POINT('Ctrl Pts',(178.307751910826,585.183152866943,-48.5163345054779)) ;
#62177=CARTESIAN_POINT('Ctrl Pts',(178.320260961917,585.147045123671,-48.5136138596793)) ;
#62178=CARTESIAN_POINT('Ctrl Pts',(178.366499301835,585.027079748457,-48.5043629778704)) ;
#62179=CARTESIAN_POINT('Ctrl Pts',(178.405806400911,584.945541844804,-48.4977280397341)) ;
#62180=CARTESIAN_POINT('Ctrl Pts',(178.493729271822,584.795661767691,-48.4851833753854)) ;
#62181=CARTESIAN_POINT('Ctrl Pts',(178.541272145921,584.726991521092,-48.4792739398857)) ;
#62182=CARTESIAN_POINT('Ctrl Pts',(178.625453742743,584.62302852524,-48.4701038447424)) ;
#62183=CARTESIAN_POINT('Ctrl Pts',(178.658901939437,584.585348205591,-48.4667242798575)) ;
#62184=CARTESIAN_POINT('Ctrl Pts',(178.736214594653,584.505825972784,-48.4594350348387)) ;
#62185=CARTESIAN_POINT('Ctrl Pts',(178.780758089445,584.464744206344,-48.455562626252)) ;
#62186=CARTESIAN_POINT('Ctrl Pts',(178.959201873152,584.317325055665,-48.4410427013598)) ;
#62187=CARTESIAN_POINT('Ctrl Pts',(179.106897446745,584.229416393242,-48.4310931826386)) ;
#62188=CARTESIAN_POINT('Ctrl Pts',(179.296062549795,584.153119208356,-48.4179493718058)) ;
#62189=CARTESIAN_POINT('Ctrl Pts',(179.327135949902,584.141650947657,-48.4157749251129)) ;
#62190=CARTESIAN_POINT('Ctrl Pts',(179.391202653044,584.120152722041,-48.4112206507534)) ;
#62191=CARTESIAN_POINT('Ctrl Pts',(179.424206587051,584.110206027197,-48.4088383029963)) ;
#62192=CARTESIAN_POINT('Ctrl Pts',(179.558225010919,584.074309879143,-48.3990843113958)) ;
#62193=CARTESIAN_POINT('Ctrl Pts',(179.661262958337,584.056848209297,-48.3914204243538)) ;
#62194=CARTESIAN_POINT('Ctrl Pts',(179.863536560141,584.041839676472,-48.3766955582062)) ;
#62195=CARTESIAN_POINT('Ctrl Pts',(179.96228948806,584.04328162874,-48.3696536971554)) ;
#62196=CARTESIAN_POINT('Ctrl Pts',(180.110276131934,584.058625983096,-48.3594314119205)) ;
#62197=CARTESIAN_POINT('Ctrl Pts',(180.159947212651,584.066056782849,-48.3560540289076)) ;
#62198=CARTESIAN_POINT('Ctrl Pts',(180.266728468062,584.087002546081,-48.3488841559948)) ;
#62199=CARTESIAN_POINT('Ctrl Pts',(180.323613961205,584.101312976819,-48.3451225870087)) ;
#62200=CARTESIAN_POINT('Ctrl Pts',(180.447179470846,584.139431521646,-48.3369841059589)) ;
#62201=CARTESIAN_POINT('Ctrl Pts',(180.513335099721,584.164547884762,-48.3326494265749)) ;
#62202=CARTESIAN_POINT('Ctrl Pts',(180.680285102839,584.240404310523,-48.321447250591)) ;
#62203=CARTESIAN_POINT('Ctrl Pts',(180.7778639742,584.297297199941,-48.3146411259093)) ;
#62204=CARTESIAN_POINT('Ctrl Pts',(180.893689803835,584.38160239818,-48.30532097844)) ;
#62205=CARTESIAN_POINT('Ctrl Pts',(180.917933084389,584.400291403845,-48.3032910877185)) ;
#62206=CARTESIAN_POINT('Ctrl Pts',(180.972056869607,584.444445034939,-48.2985463549472)) ;
#62207=CARTESIAN_POINT('Ctrl Pts',(181.0015738731,584.470313890453,-48.2958079822345)) ;
#62208=CARTESIAN_POINT('Ctrl Pts',(181.069021994091,584.533773710968,-48.2892386090915)) ;
#62209=CARTESIAN_POINT('Ctrl Pts',(181.106114365626,584.572194870677,-48.2853737720822)) ;
#62210=CARTESIAN_POINT('Ctrl Pts',(181.229463972879,584.712900760287,-48.2717640399015)) ;
#62211=CARTESIAN_POINT('Ctrl Pts',(181.305217422334,584.823746490405,-48.2620265180577)) ;
#62212=CARTESIAN_POINT('Ctrl Pts',(181.390704991926,584.988287792071,-48.2492303228113)) ;
#62213=CARTESIAN_POINT('Ctrl Pts',(181.412367059358,585.035186857292,-48.245741817317)) ;
#62214=CARTESIAN_POINT('Ctrl Pts',(181.453055904458,585.13525110279,-48.2385989756737)) ;
#62215=CARTESIAN_POINT('Ctrl Pts',(181.471630510021,585.188529314956,-48.2349638650926)) ;
#62216=CARTESIAN_POINT('Ctrl Pts',(181.50585425358,585.305477954741,-48.2272604845742)) ;
#62217=CARTESIAN_POINT('Ctrl Pts',(181.520521678923,585.369335839379,-48.2232240970912)) ;
#62218=CARTESIAN_POINT('Ctrl Pts',(181.551870665631,585.555485732305,-48.2116689419256)) ;
#62219=CARTESIAN_POINT('Ctrl Pts',(181.558782590793,585.678956048735,-48.204275786974)) ;
#62220=CARTESIAN_POINT('Ctrl Pts',(181.550318332245,585.832884809784,-48.1942591949648)) ;
#62221=CARTESIAN_POINT('Ctrl Pts',(181.547764491754,585.863677390899,-48.1922131102694)) ;
#62222=CARTESIAN_POINT('Ctrl Pts',(181.540098764288,585.932730875518,-48.1874988546373)) ;
#62223=CARTESIAN_POINT('Ctrl Pts',(181.534510895044,585.970917420704,-48.1848098243074)) ;
#62224=CARTESIAN_POINT('Ctrl Pts',(181.510419429662,586.103290542427,-48.1752777881762)) ;
#62225=CARTESIAN_POINT('Ctrl Pts',(181.485110124035,586.196043274498,-48.1682341296462)) ;
#62226=CARTESIAN_POINT('Ctrl Pts',(181.451959398854,586.286097166427,-48.1612709156719)) ;
#62227=CARTESIAN_POINT('Ctrl Pts',(181.451958155526,586.286100543914,-49.0537403040458)) ;
#62228=CARTESIAN_POINT('Ctrl Pts',(181.442367045837,586.312154604425,-49.0520465268598)) ;
#62229=CARTESIAN_POINT('Ctrl Pts',(181.432121158642,586.337978443246,-49.0503552040013)) ;
#62230=CARTESIAN_POINT('Ctrl Pts',(181.394454146755,586.426391658561,-49.0444887226731)) ;
#62231=CARTESIAN_POINT('Ctrl Pts',(181.36384202225,586.487526345688,-49.0402953049949)) ;
#62232=CARTESIAN_POINT('Ctrl Pts',(181.300623160239,586.596493277071,-49.0323589745846)) ;
#62233=CARTESIAN_POINT('Ctrl Pts',(181.269112464359,586.644838511793,-49.0286536151324)) ;
#62234=CARTESIAN_POINT('Ctrl Pts',(181.20506708751,586.73276501538,-49.0214791337567)) ;
#62235=CARTESIAN_POINT('Ctrl Pts',(181.173090421842,586.772669727805,-49.0180352194983)) ;
#62236=CARTESIAN_POINT('Ctrl Pts',(181.045386686211,586.917818712398,-49.0047277504003)) ;
#62237=CARTESIAN_POINT('Ctrl Pts',(180.938167836179,587.012111900912,-48.9943543232183)) ;
#62238=CARTESIAN_POINT('Ctrl Pts',(180.77850569482,587.119833939444,-48.9803618603223)) ;
#62239=CARTESIAN_POINT('Ctrl Pts',(180.735436557747,587.146129635776,-48.9767187236512)) ;
#62240=CARTESIAN_POINT('Ctrl Pts',(180.657977597534,587.188720591738,-48.9704631244622)) ;
#62241=CARTESIAN_POINT('Ctrl Pts',(180.624098116846,587.205868935525,-48.9678206681173)) ;
#62242=CARTESIAN_POINT('Ctrl Pts',(180.561256328243,587.235023240386,-48.9631255841729)) ;
#62243=CARTESIAN_POINT('Ctrl Pts',(180.53248750204,587.247397015689,-48.9610551831426)) ;
#62244=CARTESIAN_POINT('Ctrl Pts',(180.391846290724,587.303245000643,-48.9512392153902)) ;
#62245=CARTESIAN_POINT('Ctrl Pts',(180.275831654044,587.335361323865,-48.9440332098066)) ;
#62246=CARTESIAN_POINT('Ctrl Pts',(180.091559152841,587.365491014052,-48.9326153625952)) ;
#62247=CARTESIAN_POINT('Ctrl Pts',(180.025176612528,587.372289398275,-48.9285112382682)) ;
#62248=CARTESIAN_POINT('Ctrl Pts',(179.901573398395,587.377490501998,-48.9207000501558)) ;
#62249=CARTESIAN_POINT('Ctrl Pts',(179.844498083288,587.376959616676,-48.9170269918634)) ;
#62250=CARTESIAN_POINT('Ctrl Pts',(179.735888500295,587.37036569637,-48.9098376558024)) ;
#62251=CARTESIAN_POINT('Ctrl Pts',(179.684389951565,587.364821273548,-48.9063424581797)) ;
#62252=CARTESIAN_POINT('Ctrl Pts',(179.50018944562,587.336257913998,-48.893486501548)) ;
#62253=CARTESIAN_POINT('Ctrl Pts',(179.370153955682,587.299577166926,-48.8836886288801)) ;
#62254=CARTESIAN_POINT('Ctrl Pts',(179.196977890182,587.22718490761,-48.8700421522576)) ;
#62255=CARTESIAN_POINT('Ctrl Pts',(179.148982901137,587.204369289545,-48.8661983357896)) ;
#62256=CARTESIAN_POINT('Ctrl Pts',(179.067625799373,587.160810119648,-48.859655666143)) ;
#62257=CARTESIAN_POINT('Ctrl Pts',(179.033753333724,587.141107642177,-48.8569233855499)) ;
#62258=CARTESIAN_POINT('Ctrl Pts',(178.974361948848,587.103697949959,-48.8521586859097)) ;
#62259=CARTESIAN_POINT('Ctrl Pts',(178.948586800191,587.086439142605,-48.850103824995)) ;
#62260=CARTESIAN_POINT('Ctrl Pts',(178.834401945849,587.005274691068,-48.8409993708825)) ;
#62261=CARTESIAN_POINT('Ctrl Pts',(178.751905171419,586.933491905227,-48.8343959081399)) ;
#62262=CARTESIAN_POINT('Ctrl Pts',(178.627491283675,586.801687413218,-48.8233257170684)) ;
#62263=CARTESIAN_POINT('Ctrl Pts',(178.58143371168,586.746067414824,-48.8189073122065)) ;
#62264=CARTESIAN_POINT('Ctrl Pts',(178.504311454519,586.639557009385,-48.8106376494352)) ;
#62265=CARTESIAN_POINT('Ctrl Pts',(178.472093520653,586.589651834192,-48.8068313364632)) ;
#62266=CARTESIAN_POINT('Ctrl Pts',(178.417532366746,586.494323749243,-48.7995971454438)) ;
#62267=CARTESIAN_POINT('Ctrl Pts',(178.394462227524,586.449396804079,-48.7962020175189)) ;
#62268=CARTESIAN_POINT('Ctrl Pts',(178.332902696884,586.31479994524,-48.786034767644)) ;
#62269=CARTESIAN_POINT('Ctrl Pts',(178.300210156406,586.222727714971,-48.7790724057875)) ;
#62270=CARTESIAN_POINT('Ctrl Pts',(178.24953364727,586.02709734253,-48.7644060715532)) ;
#62271=CARTESIAN_POINT('Ctrl Pts',(178.232898034086,585.923606423054,-48.7567170633223)) ;
#62272=CARTESIAN_POINT('Ctrl Pts',(178.223788995917,585.784254712189,-48.7468898710452)) ;
#62273=CARTESIAN_POINT('Ctrl Pts',(178.2226068193,585.749207279291,-48.7444639976611)) ;
#62274=CARTESIAN_POINT('Ctrl Pts',(178.222460322143,585.681036389742,-48.7398667560257)) ;
#62275=CARTESIAN_POINT('Ctrl Pts',(178.223376160584,585.647930394898,-48.7376912221731)) ;
#62276=CARTESIAN_POINT('Ctrl Pts',(178.235112625915,585.443939353843,-48.7245176558765)) ;
#62277=CARTESIAN_POINT('Ctrl Pts',(178.271237097301,585.275526077541,-48.7145486788468)) ;
#62278=CARTESIAN_POINT('Ctrl Pts',(178.354107592696,585.058795222922,-48.6999919552509)) ;
#62279=CARTESIAN_POINT('Ctrl Pts',(178.378898080143,585.003270210825,-48.6961054971068)) ;
#62280=CARTESIAN_POINT('Ctrl Pts',(178.429836563856,584.904123752046,-48.6887778830967)) ;
#62281=CARTESIAN_POINT('Ctrl Pts',(178.455054280415,584.860106137367,-48.6853738374054)) ;
#62282=CARTESIAN_POINT('Ctrl Pts',(178.561582772263,584.692393615485,-48.6717467517413)) ;
#62283=CARTESIAN_POINT('Ctrl Pts',(178.657205466419,584.578627161155,-48.6609542442595)) ;
#62284=CARTESIAN_POINT('Ctrl Pts',(178.80360883029,584.445251161344,-48.6465667609292)) ;
#62285=CARTESIAN_POINT('Ctrl Pts',(178.842168195389,584.413182836259,-48.6429467251942)) ;
#62286=CARTESIAN_POINT('Ctrl Pts',(178.912262244202,584.360049409252,-48.6367234201416)) ;
#62287=CARTESIAN_POINT('Ctrl Pts',(178.943180031159,584.338229414607,-48.6340905778274)) ;
#62288=CARTESIAN_POINT('Ctrl Pts',(179.001108605256,584.300234666821,-48.6293961419528)) ;
#62289=CARTESIAN_POINT('Ctrl Pts',(179.027883497909,584.28373775712,-48.6273175512703)) ;
#62290=CARTESIAN_POINT('Ctrl Pts',(179.157926532345,584.208607252175,-48.6175774891948)) ;
#62291=CARTESIAN_POINT('Ctrl Pts',(179.266812928399,584.160360557507,-48.6104404346335)) ;
#62292=CARTESIAN_POINT('Ctrl Pts',(179.443693055667,584.103653972866,-48.5990792733714)) ;
#62293=CARTESIAN_POINT('Ctrl Pts',(179.508639704786,584.087073388664,-48.5949567190845)) ;
#62294=CARTESIAN_POINT('Ctrl Pts',(179.630560220302,584.063665472465,-48.5871178953679)) ;
#62295=CARTESIAN_POINT('Ctrl Pts',(179.687228202661,584.055783271736,-48.5834361639714)) ;
#62296=CARTESIAN_POINT('Ctrl Pts',(179.79577160293,584.046343517895,-48.5762371771017)) ;
#62297=CARTESIAN_POINT('Ctrl Pts',(179.847534112949,584.044265114454,-48.57274142944)) ;
#62298=CARTESIAN_POINT('Ctrl Pts',(180.034557113231,584.045474966471,-48.5598422314382)) ;
#62299=CARTESIAN_POINT('Ctrl Pts',(180.169178146,584.062817604246,-48.5499964691717)) ;
#62300=CARTESIAN_POINT('Ctrl Pts',(180.351509828747,584.109313062743,-48.5363141986945)) ;
#62301=CARTESIAN_POINT('Ctrl Pts',(180.402177987646,584.124839841457,-48.5324809233746)) ;
#62302=CARTESIAN_POINT('Ctrl Pts',(180.488823509572,584.155981592902,-48.5259530604896)) ;
#62303=CARTESIAN_POINT('Ctrl Pts',(180.52515078838,584.170501267112,-48.5232252152166)) ;
#62304=CARTESIAN_POINT('Ctrl Pts',(180.589272508025,584.198787475713,-48.5184676721755)) ;
#62305=CARTESIAN_POINT('Ctrl Pts',(180.617254126349,584.212074933187,-48.5164156067623)) ;
#62306=CARTESIAN_POINT('Ctrl Pts',(180.742381452353,584.27582783167,-48.5072888127749)) ;
#62307=CARTESIAN_POINT('Ctrl Pts',(180.834791665601,584.335018464639,-48.500664618126)) ;
#62308=CARTESIAN_POINT('Ctrl Pts',(180.97728528003,584.447492319991,-48.4895788123734)) ;
#62309=CARTESIAN_POINT('Ctrl Pts',(181.030877204606,584.495747206756,-48.485166742301)) ;
#62310=CARTESIAN_POINT('Ctrl Pts',(181.122596725458,584.589784719551,-48.4769063994183)) ;
#62311=CARTESIAN_POINT('Ctrl Pts',(181.161716030833,584.634430728337,-48.4731028998787)) ;
#62312=CARTESIAN_POINT('Ctrl Pts',(181.229553247931,584.720740420858,-48.4658729695989)) ;
#62313=CARTESIAN_POINT('Ctrl Pts',(181.25891591204,584.761809283354,-48.4624792060419)) ;
#62314=CARTESIAN_POINT('Ctrl Pts',(181.341261194128,584.888798207312,-48.4520827394775)) ;
#62315=CARTESIAN_POINT('Ctrl Pts',(181.38834236011,584.978250184839,-48.4448705192446)) ;
#62316=CARTESIAN_POINT('Ctrl Pts',(181.45644186305,585.142168860621,-48.4319797407391)) ;
#62317=CARTESIAN_POINT('Ctrl Pts',(181.480926438181,585.214887932324,-48.4263692302537)) ;
#62318=CARTESIAN_POINT('Ctrl Pts',(181.512464138701,585.335477694045,-48.4174323641217)) ;
#62319=CARTESIAN_POINT('Ctrl Pts',(181.522598529847,585.382428474779,-48.4140411988247)) ;
#62320=CARTESIAN_POINT('Ctrl Pts',(181.535685102336,585.458958414956,-48.4087209712909)) ;
#62321=CARTESIAN_POINT('Ctrl Pts',(181.539898578278,585.48828617496,-48.4067341949588)) ;
#62322=CARTESIAN_POINT('Ctrl Pts',(181.549578169499,585.571345527602,-48.40124154138)) ;
#62323=CARTESIAN_POINT('Ctrl Pts',(181.553217974826,585.625251824746,-48.3978249627858)) ;
#62324=CARTESIAN_POINT('Ctrl Pts',(181.55628927666,585.788594905675,-48.3876658151951)) ;
#62325=CARTESIAN_POINT('Ctrl Pts',(181.547572900447,585.897883036014,-48.3811145423157)) ;
#62326=CARTESIAN_POINT('Ctrl Pts',(181.515500295583,586.076170512365,-48.3698980979893)) ;
#62327=CARTESIAN_POINT('Ctrl Pts',(181.498242999368,586.145906175836,-48.3653750592674)) ;
#62328=CARTESIAN_POINT('Ctrl Pts',(181.468894521793,586.23842569739,-48.3590566210714)) ;
#62329=CARTESIAN_POINT('Ctrl Pts',(181.46069644486,586.262363153745,-48.3573926027051)) ;
#62330=CARTESIAN_POINT('Ctrl Pts',(181.45195815042,586.286100557784,-48.3557104975402)) ;
#62331=CARTESIAN_POINT('Origin',(29.8885276254069,535.710565160562,-48.522160171753)) ;
#62332=CARTESIAN_POINT('Ctrl Pts',(31.4519498095241,536.286123215158,-48.8631108318347)) ;
#62333=CARTESIAN_POINT('Ctrl Pts',(31.4454204319241,536.303859347433,-48.8618790238479)) ;
#62334=CARTESIAN_POINT('Ctrl Pts',(31.4385896048817,536.321483393227,-48.8606324540074)) ;
#62335=CARTESIAN_POINT('Ctrl Pts',(31.4195487156195,536.368233484221,-48.8572553542794)) ;
#62336=CARTESIAN_POINT('Ctrl Pts',(31.4068100232744,536.397129905838,-48.8550911380751)) ;
#62337=CARTESIAN_POINT('Ctrl Pts',(31.3434502247697,536.530457439493,-48.8447948905069)) ;
#62338=CARTESIAN_POINT('Ctrl Pts',(31.2828288436453,536.629773665628,-48.8362451218479)) ;
#62339=CARTESIAN_POINT('Ctrl Pts',(31.1713604166045,536.775676648282,-48.8229308955179)) ;
#62340=CARTESIAN_POINT('Ctrl Pts',(31.1271033933445,536.826833134008,-48.8180829824099)) ;
#62341=CARTESIAN_POINT('Ctrl Pts',(31.0398039156606,536.916136337417,-48.8093294678809)) ;
#62342=CARTESIAN_POINT('Ctrl Pts',(30.9976603212316,536.955018864236,-48.8053978137976)) ;
#62343=CARTESIAN_POINT('Ctrl Pts',(30.9142162610716,537.024391960484,-48.7981277594601)) ;
#62344=CARTESIAN_POINT('Ctrl Pts',(30.8733495719742,537.055297371613,-48.794774374771)) ;
#62345=CARTESIAN_POINT('Ctrl Pts',(30.7156180138062,537.16352740695,-48.7824936744457)) ;
#62346=CARTESIAN_POINT('Ctrl Pts',(30.5905858503303,537.227896599009,-48.7740943799516)) ;
#62347=CARTESIAN_POINT('Ctrl Pts',(30.4109162759848,537.293373274499,-48.7623513479098)) ;
#62348=CARTESIAN_POINT('Ctrl Pts',(30.3620887671397,537.308661068351,-48.7591832191955)) ;
#62349=CARTESIAN_POINT('Ctrl Pts',(30.2756551508876,537.33141398117,-48.7534956830553)) ;
#62350=CARTESIAN_POINT('Ctrl Pts',(30.2383503147815,537.339872410809,-48.7510156211688)) ;
#62351=CARTESIAN_POINT('Ctrl Pts',(30.1703921943881,537.352839841649,-48.7463976368524)) ;
#62352=CARTESIAN_POINT('Ctrl Pts',(30.1398428321677,537.357791256459,-48.7442824094505)) ;
#62353=CARTESIAN_POINT('Ctrl Pts',(29.987731379682,537.37811640213,-48.7336036163793)) ;
#62354=CARTESIAN_POINT('Ctrl Pts',(29.8648738658647,537.380896271859,-48.7245582714606)) ;
#62355=CARTESIAN_POINT('Ctrl Pts',(29.6773821562647,537.364436380474,-48.7109266828766)) ;
#62356=CARTESIAN_POINT('Ctrl Pts',(29.6123260643387,537.354823869722,-48.706222695061)) ;
#62357=CARTESIAN_POINT('Ctrl Pts',(29.4927138369646,537.329848175287,-48.6976722198205)) ;
#62358=CARTESIAN_POINT('Ctrl Pts',(29.4380435956142,537.315498654276,-48.6938029609648)) ;
#62359=CARTESIAN_POINT('Ctrl Pts',(29.3350882176055,537.282798068093,-48.6865754484628)) ;
#62360=CARTESIAN_POINT('Ctrl Pts',(29.2867209456151,537.264927143662,-48.6832058505681)) ;
#62361=CARTESIAN_POINT('Ctrl Pts',(29.1152457585742,537.192362540044,-48.6712701212747)) ;
#62362=CARTESIAN_POINT('Ctrl Pts',(28.998057623687,537.1250453891,-48.6631769723867)) ;
#62363=CARTESIAN_POINT('Ctrl Pts',(28.8478081536067,537.012589980382,-48.651666825322)) ;
#62364=CARTESIAN_POINT('Ctrl Pts',(28.8069147261988,536.978823177535,-48.6483901126609)) ;
#62365=CARTESIAN_POINT('Ctrl Pts',(28.7387935325007,536.916879526409,-48.6425409460339)) ;
#62366=CARTESIAN_POINT('Ctrl Pts',(28.7108205091927,536.889585160937,-48.640011290118)) ;
#62367=CARTESIAN_POINT('Ctrl Pts',(28.6626605689291,536.839168600924,-48.6353630801209)) ;
#62368=CARTESIAN_POINT('Ctrl Pts',(28.6421055286096,536.816425509455,-48.6332708921402)) ;
#62369=CARTESIAN_POINT('Ctrl Pts',(28.549392551664,536.707974202544,-48.6233549760745)) ;
#62370=CARTESIAN_POINT('Ctrl Pts',(28.4853744705787,536.615697813506,-48.6151208936581)) ;
#62371=CARTESIAN_POINT('Ctrl Pts',(28.3967325088784,536.455640164154,-48.6018304252883)) ;
#62372=CARTESIAN_POINT('Ctrl Pts',(28.3663571120631,536.391438263774,-48.5967239532406)) ;
#62373=CARTESIAN_POINT('Ctrl Pts',(28.318490152092,536.270910588629,-48.5876092144972)) ;
#62374=CARTESIAN_POINT('Ctrl Pts',(28.2997133518178,536.215218872086,-48.5835687403659)) ;
#62375=CARTESIAN_POINT('Ctrl Pts',(28.2704246069845,536.110333400511,-48.5762574203631)) ;
#62376=CARTESIAN_POINT('Ctrl Pts',(28.259121460215,536.061433331987,-48.5729636965277)) ;
#62377=CARTESIAN_POINT('Ctrl Pts',(28.2329604690923,535.91927585596,-48.5636579051796)) ;
#62378=CARTESIAN_POINT('Ctrl Pts',(28.2237959757104,535.825170423279,-48.5578349424046)) ;
#62379=CARTESIAN_POINT('Ctrl Pts',(28.2213777302767,535.625940040585,-48.5456522682261)) ;
#62380=CARTESIAN_POINT('Ctrl Pts',(28.2300060161302,535.521219947478,-48.5393305262647)) ;
#62381=CARTESIAN_POINT('Ctrl Pts',(28.2547562692319,535.382462152631,-48.5303194648317)) ;
#62382=CARTESIAN_POINT('Ctrl Pts',(28.2622522500082,535.347125600081,-48.5279665035358)) ;
#62383=CARTESIAN_POINT('Ctrl Pts',(28.2785345438782,535.28103077109,-48.5234070892657)) ;
#62384=CARTESIAN_POINT('Ctrl Pts',(28.2870698025533,535.250228593131,-48.521213582298)) ;
#62385=CARTESIAN_POINT('Ctrl Pts',(28.3077363051077,535.183200708031,-48.5163151105162)) ;
#62386=CARTESIAN_POINT('Ctrl Pts',(28.3202392904089,535.147106435088,-48.5135955718699)) ;
#62387=CARTESIAN_POINT('Ctrl Pts',(28.3664397794752,535.027222173313,-48.5043512989633)) ;
#62388=CARTESIAN_POINT('Ctrl Pts',(28.405704959675,534.945747298854,-48.4977219557218)) ;
#62389=CARTESIAN_POINT('Ctrl Pts',(28.4934975528425,534.796026881753,-48.4851916210285)) ;
#62390=CARTESIAN_POINT('Ctrl Pts',(28.54094623985,534.727449032701,-48.4792907597104)) ;
#62391=CARTESIAN_POINT('Ctrl Pts',(28.6250116790044,534.62354155731,-48.4701270667798)) ;
#62392=CARTESIAN_POINT('Ctrl Pts',(28.6584532530235,534.585838145977,-48.4667460351904)) ;
#62393=CARTESIAN_POINT('Ctrl Pts',(28.7356312282708,534.506392334471,-48.4594653505644)) ;
#62394=CARTESIAN_POINT('Ctrl Pts',(28.7800337381957,534.465396515331,-48.4556023595078)) ;
#62395=CARTESIAN_POINT('Ctrl Pts',(28.8843572636623,534.379091212892,-48.4471069074285)) ;
#62396=CARTESIAN_POINT('Ctrl Pts',(28.9453102389704,534.335238677291,-48.4425257259063)) ;
#62397=CARTESIAN_POINT('Ctrl Pts',(29.0949855695054,534.242200691369,-48.4317667231819)) ;
#62398=CARTESIAN_POINT('Ctrl Pts',(29.1856389041805,534.196714042877,-48.4256155216174)) ;
#62399=CARTESIAN_POINT('Ctrl Pts',(29.3090086461524,534.148292666523,-48.4170224739412)) ;
#62400=CARTESIAN_POINT('Ctrl Pts',(29.3384886336853,534.137671469888,-48.4149521926076)) ;
#62401=CARTESIAN_POINT('Ctrl Pts',(29.4036597539175,534.116247595698,-48.4103055797973)) ;
#62402=CARTESIAN_POINT('Ctrl Pts',(29.4394467489295,534.105800020707,-48.4077136888816)) ;
#62403=CARTESIAN_POINT('Ctrl Pts',(29.5788803365027,534.070122923199,-48.3975380933083)) ;
#62404=CARTESIAN_POINT('Ctrl Pts',(29.6845063342131,534.053668596351,-48.3896855205373)) ;
#62405=CARTESIAN_POINT('Ctrl Pts',(29.8813784485332,534.042121123562,-48.3754021542157)) ;
#62406=CARTESIAN_POINT('Ctrl Pts',(29.9720738372828,534.044197455524,-48.3689563092193)) ;
#62407=CARTESIAN_POINT('Ctrl Pts',(30.1119849461126,534.058859300089,-48.3592958865846)) ;
#62408=CARTESIAN_POINT('Ctrl Pts',(30.1615495460964,534.066325093203,-48.3559270262173)) ;
#62409=CARTESIAN_POINT('Ctrl Pts',(30.2685177041821,534.087409153804,-48.348746804829)) ;
#62410=CARTESIAN_POINT('Ctrl Pts',(30.3256873163134,534.101863643287,-48.3449677232646)) ;
#62411=CARTESIAN_POINT('Ctrl Pts',(30.4502107481799,534.140478632447,-48.3367674456449)) ;
#62412=CARTESIAN_POINT('Ctrl Pts',(30.5170165955757,534.166006242255,-48.3323900406877)) ;
#62413=CARTESIAN_POINT('Ctrl Pts',(30.6824974099923,534.24175983126,-48.3212747043782)) ;
#62414=CARTESIAN_POINT('Ctrl Pts',(30.7781710719915,534.297658692539,-48.3145903065853)) ;
#62415=CARTESIAN_POINT('Ctrl Pts',(30.89246928846,534.380676967541,-48.3054068684597)) ;
#62416=CARTESIAN_POINT('Ctrl Pts',(30.9168412750927,534.399431150226,-48.3033692886197)) ;
#62417=CARTESIAN_POINT('Ctrl Pts',(30.9707476966025,534.443340014193,-48.2986496486544)) ;
#62418=CARTESIAN_POINT('Ctrl Pts',(30.9999477732322,534.468870957812,-48.2959456836003)) ;
#62419=CARTESIAN_POINT('Ctrl Pts',(31.0663987464412,534.53119484749,-48.289488103178)) ;
#62420=CARTESIAN_POINT('Ctrl Pts',(31.1028596158002,534.568771895611,-48.2857020423812)) ;
#62421=CARTESIAN_POINT('Ctrl Pts',(31.2279575461114,534.710480065302,-48.2719588210758)) ;
#62422=CARTESIAN_POINT('Ctrl Pts',(31.3054876975347,534.823727772674,-48.2619993719887)) ;
#62423=CARTESIAN_POINT('Ctrl Pts',(31.3919382314065,534.990872532076,-48.24902413267)) ;
#62424=CARTESIAN_POINT('Ctrl Pts',(31.4134391968092,535.03762634286,-48.2455520136143)) ;
#62425=CARTESIAN_POINT('Ctrl Pts',(31.454065443006,535.137961759983,-48.2383995061277)) ;
#62426=CARTESIAN_POINT('Ctrl Pts',(31.4726807808057,535.191678584579,-48.2347403570559)) ;
#62427=CARTESIAN_POINT('Ctrl Pts',(31.5070335174782,535.310054343029,-48.2269553265335)) ;
#62428=CARTESIAN_POINT('Ctrl Pts',(31.5217179082243,535.374915461387,-48.2228632113497)) ;
#62429=CARTESIAN_POINT('Ctrl Pts',(31.5519263648473,535.558791651747,-48.2114628275883)) ;
#62430=CARTESIAN_POINT('Ctrl Pts',(31.5585322927592,535.678834988884,-48.2042620913468)) ;
#62431=CARTESIAN_POINT('Ctrl Pts',(31.5505560086946,535.829694152295,-48.1944607941727)) ;
#62432=CARTESIAN_POINT('Ctrl Pts',(31.5480328185513,535.860806461547,-48.1923970588143)) ;
#62433=CARTESIAN_POINT('Ctrl Pts',(31.54053205366,535.929336850383,-48.1877251296333)) ;
#62434=CARTESIAN_POINT('Ctrl Pts',(31.5351541337926,535.966690612461,-48.1850996528049)) ;
#62435=CARTESIAN_POINT('Ctrl Pts',(31.5113175405677,536.099990816266,-48.1755200396746)) ;
#62436=CARTESIAN_POINT('Ctrl Pts',(31.4856974378523,536.194451838716,-48.1683484248333)) ;
#62437=CARTESIAN_POINT('Ctrl Pts',(31.451951253523,536.286119292724,-48.161260329976)) ;
#62438=CARTESIAN_POINT('Ctrl Pts',(31.4519498093678,536.286123215583,-49.053781357604)) ;
#62439=CARTESIAN_POINT('Ctrl Pts',(31.4421205686183,536.312822960126,-49.0520449154176)) ;
#62440=CARTESIAN_POINT('Ctrl Pts',(31.4316037221729,536.339280832236,-49.0503110614434)) ;
#62441=CARTESIAN_POINT('Ctrl Pts',(31.3937051203419,536.427928965283,-49.0444228981946)) ;
#62442=CARTESIAN_POINT('Ctrl Pts',(31.3632095023766,536.488692706009,-49.0402501160774)) ;
#62443=CARTESIAN_POINT('Ctrl Pts',(31.3002108353399,536.597138557633,-49.0323447179619)) ;
#62444=CARTESIAN_POINT('Ctrl Pts',(31.2687782099982,536.645321263705,-49.0286488811754)) ;
#62445=CARTESIAN_POINT('Ctrl Pts',(31.2047763014379,536.733142823493,-49.0214786452748)) ;
#62446=CARTESIAN_POINT('Ctrl Pts',(31.1727448169078,536.773090852571,-49.0180286330047)) ;
#62447=CARTESIAN_POINT('Ctrl Pts',(31.045525067889,536.917582596926,-49.0047712786818)) ;
#62448=CARTESIAN_POINT('Ctrl Pts',(30.9390154262382,537.011331975432,-48.9944625987745)) ;
#62449=CARTESIAN_POINT('Ctrl Pts',(30.7799073340656,537.118961076065,-48.9805020290253)) ;
#62450=CARTESIAN_POINT('Ctrl Pts',(30.736545836289,537.145487669707,-48.9768303167691)) ;
#62451=CARTESIAN_POINT('Ctrl Pts',(30.6586460790295,537.188376554804,-48.9705341909782)) ;
#62452=CARTESIAN_POINT('Ctrl Pts',(30.6246301766632,537.205611172816,-48.9678792523042)) ;
#62453=CARTESIAN_POINT('Ctrl Pts',(30.5617479321509,537.234803998063,-48.963178571334)) ;
#62454=CARTESIAN_POINT('Ctrl Pts',(30.5330825030713,537.247145373332,-48.9611142101719)) ;
#62455=CARTESIAN_POINT('Ctrl Pts',(30.4062318452574,537.29758362935,-48.9522545644049)) ;
#62456=CARTESIAN_POINT('Ctrl Pts',(30.3048952988687,537.327132303877,-48.9458690541033)) ;
#62457=CARTESIAN_POINT('Ctrl Pts',(30.1291327364573,537.360742121137,-48.9349458198824)) ;
#62458=CARTESIAN_POINT('Ctrl Pts',(30.0559966536166,537.369760128288,-48.930444779145)) ;
#62459=CARTESIAN_POINT('Ctrl Pts',(29.9226393734231,537.377294919229,-48.9220561003875)) ;
#62460=CARTESIAN_POINT('Ctrl Pts',(29.8626383459254,537.377442512114,-48.9182165652561)) ;
#62461=CARTESIAN_POINT('Ctrl Pts',(29.7519770257693,537.371738297544,-48.9109261301689)) ;
#62462=CARTESIAN_POINT('Ctrl Pts',(29.7013411892077,537.366796578201,-48.9075090647033)) ;
#62463=CARTESIAN_POINT('Ctrl Pts',(29.5613095774384,537.346627004707,-48.8977970203768)) ;
#62464=CARTESIAN_POINT('Ctrl Pts',(29.4728222904853,537.326409953065,-48.8913497197765)) ;
#62465=CARTESIAN_POINT('Ctrl Pts',(29.2846788589956,537.266942440775,-48.877062579661)) ;
#62466=CARTESIAN_POINT('Ctrl Pts',(29.1862519074647,537.225079489781,-48.8692076446659)) ;
#62467=CARTESIAN_POINT('Ctrl Pts',(29.0596865745791,537.156239416906,-48.8590246154616)) ;
#62468=CARTESIAN_POINT('Ctrl Pts',(29.0274759559766,537.137289427105,-48.8564273766625)) ;
#62469=CARTESIAN_POINT('Ctrl Pts',(28.9691398590744,537.100273251785,-48.8517500090167)) ;
#62470=CARTESIAN_POINT('Ctrl Pts',(28.9428432952346,537.082514045143,-48.8496551588635)) ;
#62471=CARTESIAN_POINT('Ctrl Pts',(28.8228277652379,536.996371012458,-48.8400846281266)) ;
#62472=CARTESIAN_POINT('Ctrl Pts',(28.7358964591998,536.919060786394,-48.8331020510572)) ;
#62473=CARTESIAN_POINT('Ctrl Pts',(28.6120290203898,536.783271594557,-48.8218629018146)) ;
#62474=CARTESIAN_POINT('Ctrl Pts',(28.5694611510534,536.730472224843,-48.8176949640231)) ;
#62475=CARTESIAN_POINT('Ctrl Pts',(28.4969242682058,536.628336572284,-48.8097900613749)) ;
#62476=CARTESIAN_POINT('Ctrl Pts',(28.4660742189961,536.579754065192,-48.8060891793899)) ;
#62477=CARTESIAN_POINT('Ctrl Pts',(28.4124117211227,536.484712618079,-48.7988812822438)) ;
#62478=CARTESIAN_POINT('Ctrl Pts',(28.3891303541027,536.438596229111,-48.79539733326)) ;
#62479=CARTESIAN_POINT('Ctrl Pts',(28.3117554211104,536.265815650094,-48.7823481043735)) ;
#62480=CARTESIAN_POINT('Ctrl Pts',(28.2712856127787,536.133682124281,-48.7723185326411)) ;
#62481=CARTESIAN_POINT('Ctrl Pts',(28.2385286580393,535.946741599366,-48.7585210768233)) ;
#62482=CARTESIAN_POINT('Ctrl Pts',(28.2319437995907,535.894973950611,-48.7547483986554)) ;
#62483=CARTESIAN_POINT('Ctrl Pts',(28.2247186035574,535.80435638508,-48.7483067016716)) ;
#62484=CARTESIAN_POINT('Ctrl Pts',(28.2229870553385,535.76563313255,-48.7456054799053)) ;
#62485=CARTESIAN_POINT('Ctrl Pts',(28.2223032057972,535.695809024691,-48.7408674607804)) ;
#62486=CARTESIAN_POINT('Ctrl Pts',(28.2228682259566,535.664734565818,-48.7388097405462)) ;
#62487=CARTESIAN_POINT('Ctrl Pts',(28.2292703114838,535.526135406332,-48.7297971737671)) ;
#62488=CARTESIAN_POINT('Ctrl Pts',(28.244654448591,535.419297890581,-48.7232748848117)) ;
#62489=CARTESIAN_POINT('Ctrl Pts',(28.2875103192788,535.244113187678,-48.7122620083713)) ;
#62490=CARTESIAN_POINT('Ctrl Pts',(28.3093700686501,535.17475338164,-48.7078152279912)) ;
#62491=CARTESIAN_POINT('Ctrl Pts',(28.3572599854346,535.051533722027,-48.6995057005265)) ;
#62492=CARTESIAN_POINT('Ctrl Pts',(28.3817935899067,534.997224954907,-48.6956890215672)) ;
#62493=CARTESIAN_POINT('Ctrl Pts',(28.4323434189617,534.89962725477,-48.6884528302141)) ;
#62494=CARTESIAN_POINT('Ctrl Pts',(28.4575210253998,534.855982290588,-48.6850670821177)) ;
#62495=CARTESIAN_POINT('Ctrl Pts',(28.5337123354556,534.736737625771,-48.6753505723693)) ;
#62496=CARTESIAN_POINT('Ctrl Pts',(28.589003469921,534.664096461363,-48.6688633113024)) ;
#62497=CARTESIAN_POINT('Ctrl Pts',(28.7211304162431,534.517221958731,-48.6545527618538)) ;
#62498=CARTESIAN_POINT('Ctrl Pts',(28.799733098023,534.445096067159,-48.6467170500542)) ;
#62499=CARTESIAN_POINT('Ctrl Pts',(28.9144493430178,534.358485740725,-48.6365565910861)) ;
#62500=CARTESIAN_POINT('Ctrl Pts',(28.9449669730364,534.337014608568,-48.6339631071992)) ;
#62501=CARTESIAN_POINT('Ctrl Pts',(29.0026784291749,534.299243107175,-48.6292931361974)) ;
#62502=CARTESIAN_POINT('Ctrl Pts',(29.0296637178229,534.282660515776,-48.6272019168331)) ;
#62503=CARTESIAN_POINT('Ctrl Pts',(29.1579836052175,534.208762064253,-48.6176079360074)) ;
#62504=CARTESIAN_POINT('Ctrl Pts',(29.2646857390792,534.161392511465,-48.610603227281)) ;
#62505=CARTESIAN_POINT('Ctrl Pts',(29.4398334887716,534.104698864893,-48.599346790951)) ;
#62506=CARTESIAN_POINT('Ctrl Pts',(29.5054045485285,534.087805567345,-48.595185547943)) ;
#62507=CARTESIAN_POINT('Ctrl Pts',(29.6282356498718,534.064021358175,-48.5872907661045)) ;
#62508=CARTESIAN_POINT('Ctrl Pts',(29.6851755961976,534.056024397277,-48.5835931198444)) ;
#62509=CARTESIAN_POINT('Ctrl Pts',(29.7938399477841,534.04645705887,-48.5763891853042)) ;
#62510=CARTESIAN_POINT('Ctrl Pts',(29.8454467967628,534.044322519761,-48.572905819667)) ;
#62511=CARTESIAN_POINT('Ctrl Pts',(30.0344919646107,534.045291275285,-48.559874997899)) ;
#62512=CARTESIAN_POINT('Ctrl Pts',(30.1712819879578,534.062997633868,-48.5498654329698)) ;
#62513=CARTESIAN_POINT('Ctrl Pts',(30.354861364568,534.110310902991,-48.5360839772566)) ;
#62514=CARTESIAN_POINT('Ctrl Pts',(30.4047726488978,534.125707882412,-48.5323079446873)) ;
#62515=CARTESIAN_POINT('Ctrl Pts',(30.490346221921,534.156578956215,-48.5258616200494)) ;
#62516=CARTESIAN_POINT('Ctrl Pts',(30.5263448359197,534.171003999066,-48.5231590718303)) ;
#62517=CARTESIAN_POINT('Ctrl Pts',(30.5902304062684,534.199229808851,-48.5184200337856)) ;
#62518=CARTESIAN_POINT('Ctrl Pts',(30.6182933053543,534.212578675798,-48.5163625553282)) ;
#62519=CARTESIAN_POINT('Ctrl Pts',(30.7419759751355,534.275712845991,-48.5073424179834)) ;
#62520=CARTESIAN_POINT('Ctrl Pts',(30.8330148628258,534.333929549948,-48.5008134722058)) ;
#62521=CARTESIAN_POINT('Ctrl Pts',(30.9749136575361,534.445418049187,-48.4897945293355)) ;
#62522=CARTESIAN_POINT('Ctrl Pts',(31.0290298718726,534.49397753817,-48.4853486686103)) ;
#62523=CARTESIAN_POINT('Ctrl Pts',(31.121438346133,534.588498110605,-48.4770399616097)) ;
#62524=CARTESIAN_POINT('Ctrl Pts',(31.1607563698252,534.633283390558,-48.4732231409905)) ;
#62525=CARTESIAN_POINT('Ctrl Pts',(31.2287526516097,534.719660932539,-48.4659857941293)) ;
#62526=CARTESIAN_POINT('Ctrl Pts',(31.2581007393871,534.760637355124,-48.4625989939174)) ;
#62527=CARTESIAN_POINT('Ctrl Pts',(31.3354475186327,534.879681277916,-48.4528511260399)) ;
#62528=CARTESIAN_POINT('Ctrl Pts',(31.3789234103375,534.96045798176,-48.4463313835402)) ;
#62529=CARTESIAN_POINT('Ctrl Pts',(31.4488258018835,535.120687430415,-48.4336674869897)) ;
#62530=CARTESIAN_POINT('Ctrl Pts',(31.476347860618,535.199377132828,-48.4275632007741)) ;
#62531=CARTESIAN_POINT('Ctrl Pts',(31.5108055247004,535.328109887804,-48.4179905323981)) ;
#62532=CARTESIAN_POINT('Ctrl Pts',(31.5215571408749,535.376988614597,-48.4144491906886)) ;
#62533=CARTESIAN_POINT('Ctrl Pts',(31.535137920552,535.455409534496,-48.408987186366)) ;
#62534=CARTESIAN_POINT('Ctrl Pts',(31.5394058780599,535.484664384523,-48.4070008085166)) ;
#62535=CARTESIAN_POINT('Ctrl Pts',(31.5491582978217,535.566754525897,-48.4015617422502)) ;
#62536=CARTESIAN_POINT('Ctrl Pts',(31.5528988245009,535.619760350806,-48.3981950541164)) ;
#62537=CARTESIAN_POINT('Ctrl Pts',(31.556609044588,535.783653537267,-48.387985950332)) ;
#62538=CARTESIAN_POINT('Ctrl Pts',(31.5480563565674,535.894423330942,-48.381351556632)) ;
#62539=CARTESIAN_POINT('Ctrl Pts',(31.5158807242769,536.074546829631,-48.3700259558492)) ;
#62540=CARTESIAN_POINT('Ctrl Pts',(31.4985962826607,536.144659280053,-48.3654814587207)) ;
#62541=CARTESIAN_POINT('Ctrl Pts',(31.4690916639415,536.237850375347,-48.3591199242599)) ;
#62542=CARTESIAN_POINT('Ctrl Pts',(31.4607976500271,536.26208930646,-48.3574353418366)) ;
#62543=CARTESIAN_POINT('Ctrl Pts',(31.4519498042747,536.286123229417,-48.3557322092704)) ;
#62544=CARTESIAN_POINT('Origin',(29.8885276254157,585.710565160562,-48.522160171753)) ;
#62545=CARTESIAN_POINT('Ctrl Pts',(31.451951903833,586.286117526255,-48.8631174034081)) ;
#62546=CARTESIAN_POINT('Ctrl Pts',(31.445414274508,586.303876272495,-48.8618840380574)) ;
#62547=CARTESIAN_POINT('Ctrl Pts',(31.4385744286486,586.321522643009,-48.8606358738028)) ;
#62548=CARTESIAN_POINT('Ctrl Pts',(31.419518555509,586.36830420647,-48.8572563572135)) ;
#62549=CARTESIAN_POINT('Ctrl Pts',(31.4067741013603,586.39720983254,-48.8550913335529)) ;
#62550=CARTESIAN_POINT('Ctrl Pts',(31.3434426454872,586.530457434389,-48.8448006684502)) ;
#62551=CARTESIAN_POINT('Ctrl Pts',(31.2828738267999,586.629693428051,-48.8362581932297)) ;
#62552=CARTESIAN_POINT('Ctrl Pts',(31.1714618048038,586.775556366407,-48.8229485875785)) ;
#62553=CARTESIAN_POINT('Ctrl Pts',(31.1271901091252,586.826738668564,-48.8180984699313)) ;
#62554=CARTESIAN_POINT('Ctrl Pts',(31.0398659904931,586.916077711557,-48.809341775052)) ;
#62555=CARTESIAN_POINT('Ctrl Pts',(30.9977140564705,586.954971606289,-48.8054090976715)) ;
#62556=CARTESIAN_POINT('Ctrl Pts',(30.9142615818459,587.024356587802,-48.7981379971501)) ;
#62557=CARTESIAN_POINT('Ctrl Pts',(30.8733957523154,587.055263559717,-48.7947845459238)) ;
#62558=CARTESIAN_POINT('Ctrl Pts',(30.7156269223439,587.163527102585,-48.7825004886115)) ;
#62559=CARTESIAN_POINT('Ctrl Pts',(30.5905496439846,587.227917914789,-48.7740984093909)) ;
#62560=CARTESIAN_POINT('Ctrl Pts',(30.4108440838895,587.293396616897,-48.7623531259073)) ;
#62561=CARTESIAN_POINT('Ctrl Pts',(30.3620302084178,587.308677942517,-48.759185862631)) ;
#62562=CARTESIAN_POINT('Ctrl Pts',(30.2756164453555,587.331423077509,-48.7534995852661)) ;
#62563=CARTESIAN_POINT('Ctrl Pts',(30.2383175334423,587.33987930196,-48.7510198891862)) ;
#62564=CARTESIAN_POINT('Ctrl Pts',(30.1703602760856,587.352845416816,-48.7464019168162)) ;
#62565=CARTESIAN_POINT('Ctrl Pts',(30.1398057068966,587.357797017178,-48.7442863000492)) ;
#62566=CARTESIAN_POINT('Ctrl Pts',(29.9877304410739,587.378113357972,-48.7336099174467)) ;
#62567=CARTESIAN_POINT('Ctrl Pts',(29.8649155294811,587.380893766487,-48.7245678091076)) ;
#62568=CARTESIAN_POINT('Ctrl Pts',(29.6774514396149,587.364445766459,-48.7109381722721)) ;
#62569=CARTESIAN_POINT('Ctrl Pts',(29.6123814452612,587.354833717225,-48.7062331452597)) ;
#62570=CARTESIAN_POINT('Ctrl Pts',(29.4927481734006,587.329856819,-48.6976811214779)) ;
#62571=CARTESIAN_POINT('Ctrl Pts',(29.4380706841677,587.315506510809,-48.6938113330393)) ;
#62572=CARTESIAN_POINT('Ctrl Pts',(29.3351066489178,587.282804603572,-48.6865831930285)) ;
#62573=CARTESIAN_POINT('Ctrl Pts',(29.2867378096245,587.264933721043,-48.6832134788407)) ;
#62574=CARTESIAN_POINT('Ctrl Pts',(29.1152476886922,587.192364817326,-48.671276695858)) ;
#62575=CARTESIAN_POINT('Ctrl Pts',(28.9980474770585,587.125040331794,-48.663182740517)) ;
#62576=CARTESIAN_POINT('Ctrl Pts',(28.84779135783,587.012576410687,-48.6516719089149)) ;
#62577=CARTESIAN_POINT('Ctrl Pts',(28.8069010735547,586.978811385645,-48.6483953959183)) ;
#62578=CARTESIAN_POINT('Ctrl Pts',(28.7387838345676,586.916870248669,-48.6425464901203)) ;
#62579=CARTESIAN_POINT('Ctrl Pts',(28.7108117873238,586.889576413327,-48.6400168881208)) ;
#62580=CARTESIAN_POINT('Ctrl Pts',(28.6626506075018,586.83915787209,-48.6353684987152)) ;
#62581=CARTESIAN_POINT('Ctrl Pts',(28.6420935377327,586.816412087286,-48.6332760642411)) ;
#62582=CARTESIAN_POINT('Ctrl Pts',(28.5493991477983,586.70797970938,-48.6233619092092)) ;
#62583=CARTESIAN_POINT('Ctrl Pts',(28.4853969049893,586.615728900754,-48.6151301082404)) ;
#62584=CARTESIAN_POINT('Ctrl Pts',(28.3967571336742,586.455690593489,-48.6018408934074)) ;
#62585=CARTESIAN_POINT('Ctrl Pts',(28.3663747245201,586.391478871241,-48.5967335237128)) ;
#62586=CARTESIAN_POINT('Ctrl Pts',(28.3184987900759,586.270935432396,-48.5876174612283)) ;
#62587=CARTESIAN_POINT('Ctrl Pts',(28.2997192532535,586.215238164086,-48.5835765421571)) ;
#62588=CARTESIAN_POINT('Ctrl Pts',(28.2704273385842,586.110344754646,-48.5762646252609)) ;
#62589=CARTESIAN_POINT('Ctrl Pts',(28.259123348422,586.061442440133,-48.5729707365131)) ;
#62590=CARTESIAN_POINT('Ctrl Pts',(28.2329612179784,585.919282092521,-48.5636647331985)) ;
#62591=CARTESIAN_POINT('Ctrl Pts',(28.2237963249913,585.825176036673,-48.5578417212622)) ;
#62592=CARTESIAN_POINT('Ctrl Pts',(28.2213774626171,585.625943716043,-48.5456589164728)) ;
#62593=CARTESIAN_POINT('Ctrl Pts',(28.2300056645136,585.521222313689,-48.5393370956589)) ;
#62594=CARTESIAN_POINT('Ctrl Pts',(28.2547562756177,585.382461980831,-48.5303258642098)) ;
#62595=CARTESIAN_POINT('Ctrl Pts',(28.2622525376537,585.347124186651,-48.5279728170235)) ;
#62596=CARTESIAN_POINT('Ctrl Pts',(28.2785358516811,585.281025679962,-48.5234131361376)) ;
#62597=CARTESIAN_POINT('Ctrl Pts',(28.2870719106186,585.250221083006,-48.5212194454555)) ;
#62598=CARTESIAN_POINT('Ctrl Pts',(28.3077407921973,585.183186959741,-48.5163204859633)) ;
#62599=CARTESIAN_POINT('Ctrl Pts',(28.3202454848325,585.147088915202,-48.5136006387902)) ;
#62600=CARTESIAN_POINT('Ctrl Pts',(28.3664566130891,585.027181913957,-48.5043545186396)) ;
#62601=CARTESIAN_POINT('Ctrl Pts',(28.4057335667357,584.94568936655,-48.4977236111895)) ;
#62602=CARTESIAN_POINT('Ctrl Pts',(28.4935581090456,584.795932053103,-48.485189927585)) ;
#62603=CARTESIAN_POINT('Ctrl Pts',(28.5410274421894,584.727335442535,-48.4792872991504)) ;
#62604=CARTESIAN_POINT('Ctrl Pts',(28.6251184481247,584.623417601101,-48.4701223348718)) ;
#62605=CARTESIAN_POINT('Ctrl Pts',(28.6585617390161,584.585719641628,-48.4667416485274)) ;
#62606=CARTESIAN_POINT('Ctrl Pts',(28.7357727542759,584.506254866704,-48.4594588549308)) ;
#62607=CARTESIAN_POINT('Ctrl Pts',(28.7802097380882,584.465237936564,-48.4555935583331)) ;
#62608=CARTESIAN_POINT('Ctrl Pts',(28.8846519841829,584.378863586232,-48.4470900730299)) ;
#62609=CARTESIAN_POINT('Ctrl Pts',(28.9456941544283,584.334970228841,-48.4425033676714)) ;
#62610=CARTESIAN_POINT('Ctrl Pts',(29.095284272208,584.242055365075,-48.431752711962)) ;
#62611=CARTESIAN_POINT('Ctrl Pts',(29.1857337121211,584.196685595261,-48.4256148653484)) ;
#62612=CARTESIAN_POINT('Ctrl Pts',(29.308895433532,584.148334388459,-48.4170364395786)) ;
#62613=CARTESIAN_POINT('Ctrl Pts',(29.3383877677785,584.137706469837,-48.4149653444503)) ;
#62614=CARTESIAN_POINT('Ctrl Pts',(29.4035476772101,584.11628225571,-48.4103196186268)) ;
#62615=CARTESIAN_POINT('Ctrl Pts',(29.4393104057071,584.10583874822,-48.4077295406124)) ;
#62616=CARTESIAN_POINT('Ctrl Pts',(29.5785795201811,584.070188940319,-48.3975660997385)) ;
#62617=CARTESIAN_POINT('Ctrl Pts',(29.6840607939237,584.053732638662,-48.3897242915992)) ;
#62618=CARTESIAN_POINT('Ctrl Pts',(29.8809666072766,584.042113179148,-48.3754372096816)) ;
#62619=CARTESIAN_POINT('Ctrl Pts',(29.9718429293535,584.044176114987,-48.3689779597763)) ;
#62620=CARTESIAN_POINT('Ctrl Pts',(30.1119402854631,584.058853043998,-48.3593044710473)) ;
#62621=CARTESIAN_POINT('Ctrl Pts',(30.1615120803415,584.066318656834,-48.3559350558121)) ;
#62622=CARTESIAN_POINT('Ctrl Pts',(30.2684818203681,584.08740096651,-48.348754602551)) ;
#62623=CARTESIAN_POINT('Ctrl Pts',(30.3256460785242,584.101852652511,-48.3449758032274)) ;
#62624=CARTESIAN_POINT('Ctrl Pts',(30.4501491659698,584.140457359066,-48.3367767317666)) ;
#62625=CARTESIAN_POINT('Ctrl Pts',(30.5169405733026,584.165976078781,-48.3324002121253)) ;
#62626=CARTESIAN_POINT('Ctrl Pts',(30.6824466268293,584.241729411495,-48.3212832619082)) ;
#62627=CARTESIAN_POINT('Ctrl Pts',(30.7781559128771,584.297646062732,-48.3145965096427)) ;
#62628=CARTESIAN_POINT('Ctrl Pts',(30.8924838136642,584.380687968153,-48.3054103738149)) ;
#62629=CARTESIAN_POINT('Ctrl Pts',(30.9168543912333,584.399441473042,-48.3033728420633)) ;
#62630=CARTESIAN_POINT('Ctrl Pts',(30.9707692336124,584.443358012326,-48.2986523179648)) ;
#62631=CARTESIAN_POINT('Ctrl Pts',(30.9999785026842,584.468898061059,-48.2959473720544)) ;
#62632=CARTESIAN_POINT('Ctrl Pts',(31.0664577942132,584.531252549733,-48.2894866498209)) ;
#62633=CARTESIAN_POINT('Ctrl Pts',(31.1029364879462,584.568852341852,-48.2856983870331)) ;
#62634=CARTESIAN_POINT('Ctrl Pts',(31.2279978609192,584.710543075024,-48.271957567134)) ;
#62635=CARTESIAN_POINT('Ctrl Pts',(31.3054875040584,584.823737638272,-48.2620029832366)) ;
#62636=CARTESIAN_POINT('Ctrl Pts',(31.3919167571382,584.990827162992,-48.2490314326713)) ;
#62637=CARTESIAN_POINT('Ctrl Pts',(31.4134220282484,585.037586891647,-48.2455587370126)) ;
#62638=CARTESIAN_POINT('Ctrl Pts',(31.4540496185314,585.137919422736,-48.238406203904)) ;
#62639=CARTESIAN_POINT('Ctrl Pts',(31.4726634996755,585.191626850893,-48.2347475537479)) ;
#62640=CARTESIAN_POINT('Ctrl Pts',(31.5070119830165,585.309971010306,-48.226964295642)) ;
#62641=CARTESIAN_POINT('Ctrl Pts',(31.5216952390433,585.374809568827,-48.222873409492)) ;
#62642=CARTESIAN_POINT('Ctrl Pts',(31.5519254659926,585.558728309999,-48.2114699996543)) ;
#62643=CARTESIAN_POINT('Ctrl Pts',(31.5585372407686,585.678839707607,-48.2042653578465)) ;
#62644=CARTESIAN_POINT('Ctrl Pts',(31.5505511352172,585.829760711676,-48.194459660826)) ;
#62645=CARTESIAN_POINT('Ctrl Pts',(31.5480271865968,585.86086753712,-48.1923962024582)) ;
#62646=CARTESIAN_POINT('Ctrl Pts',(31.5405221375054,585.929415790313,-48.1877228879381)) ;
#62647=CARTESIAN_POINT('Ctrl Pts',(31.5351387999145,585.966792651816,-48.1850956588018)) ;
#62648=CARTESIAN_POINT('Ctrl Pts',(31.5112957067943,586.100070682857,-48.1755171306818)) ;
#62649=CARTESIAN_POINT('Ctrl Pts',(31.4856838387136,586.194487787323,-48.1683488037984)) ;
#62650=CARTESIAN_POINT('Ctrl Pts',(31.4519532733313,586.286113806151,-48.1612639293305)) ;
#62651=CARTESIAN_POINT('Ctrl Pts',(31.4519519036772,586.286117526679,-49.0537704297648)) ;
#62652=CARTESIAN_POINT('Ctrl Pts',(31.421888077714,586.367782581286,-49.0484597996442)) ;
#62653=CARTESIAN_POINT('Ctrl Pts',(31.3854244428663,586.44709620345,-49.0431716762742)) ;
#62654=CARTESIAN_POINT('Ctrl Pts',(31.3130425560406,586.576615087064,-49.033878018227)) ;
#62655=CARTESIAN_POINT('Ctrl Pts',(31.2803461721985,586.628238848599,-49.0299782559106)) ;
#62656=CARTESIAN_POINT('Ctrl Pts',(31.2156925895508,586.718889554863,-49.0226674544353)) ;
#62657=CARTESIAN_POINT('Ctrl Pts',(31.1846563998223,586.758484131325,-49.0192959156207)) ;
#62658=CARTESIAN_POINT('Ctrl Pts',(31.0546535773857,586.909711023892,-49.0056355997136)) ;
#62659=CARTESIAN_POINT('Ctrl Pts',(30.9426962060906,587.0092223164,-48.9947606263072)) ;
#62660=CARTESIAN_POINT('Ctrl Pts',(30.7774075023683,587.12051796513,-48.980283192767)) ;
#62661=CARTESIAN_POINT('Ctrl Pts',(30.734533338749,587.146653362595,-48.9766582859475)) ;
#62662=CARTESIAN_POINT('Ctrl Pts',(30.6573775015316,587.189029753654,-48.9704291484922)) ;
#62663=CARTESIAN_POINT('Ctrl Pts',(30.6235983888595,587.206111630206,-48.9677952116997)) ;
#62664=CARTESIAN_POINT('Ctrl Pts',(30.5608394961429,587.235207520903,-48.9631070895318)) ;
#62665=CARTESIAN_POINT('Ctrl Pts',(30.5320490588203,587.247581059817,-48.9610355313183)) ;
#62666=CARTESIAN_POINT('Ctrl Pts',(30.3916611088348,587.303280178125,-48.9512388317041)) ;
#62667=CARTESIAN_POINT('Ctrl Pts',(30.2759473600757,587.335310846125,-48.9440495531446)) ;
#62668=CARTESIAN_POINT('Ctrl Pts',(30.0919257833265,587.365448569377,-48.9326459202487)) ;
#62669=CARTESIAN_POINT('Ctrl Pts',(30.0254808689942,587.372266915703,-48.9285377892994)) ;
#62670=CARTESIAN_POINT('Ctrl Pts',(29.9017875197256,587.377489738618,-48.9207207309675)) ;
#62671=CARTESIAN_POINT('Ctrl Pts',(29.8446850354306,587.376965472036,-48.9170459215576)) ;
#62672=CARTESIAN_POINT('Ctrl Pts',(29.736049637312,587.370380450138,-48.9098548858993)) ;
#62673=CARTESIAN_POINT('Ctrl Pts',(29.6845523622667,587.364841250242,-48.9063598316317)) ;
#62674=CARTESIAN_POINT('Ctrl Pts',(29.5002524777121,587.336281214402,-48.8934972606977)) ;
#62675=CARTESIAN_POINT('Ctrl Pts',(29.3701198079592,587.29957445332,-48.8836918630579)) ;
#62676=CARTESIAN_POINT('Ctrl Pts',(29.1968897407221,587.227143495319,-48.8700407225077)) ;
#62677=CARTESIAN_POINT('Ctrl Pts',(29.1489272394888,587.204340498131,-48.8661994840422)) ;
#62678=CARTESIAN_POINT('Ctrl Pts',(29.06761643464,587.16080436013,-48.8596605593172)) ;
#62679=CARTESIAN_POINT('Ctrl Pts',(29.0337586969931,587.141110381612,-48.8569294932786)) ;
#62680=CARTESIAN_POINT('Ctrl Pts',(28.974393253501,587.103718173652,-48.8521669165994)) ;
#62681=CARTESIAN_POINT('Ctrl Pts',(28.9486295188721,587.086468003505,-48.8501129820764)) ;
#62682=CARTESIAN_POINT('Ctrl Pts',(28.8561505308132,587.020737934175,-48.8427393643579)) ;
#62683=CARTESIAN_POINT('Ctrl Pts',(28.7925708362745,586.968037745833,-48.8376588523299)) ;
#62684=CARTESIAN_POINT('Ctrl Pts',(28.6710461307095,586.85105862289,-48.82733849245)) ;
#62685=CARTESIAN_POINT('Ctrl Pts',(28.6136785386213,586.786551045327,-48.8221145311418)) ;
#62686=CARTESIAN_POINT('Ctrl Pts',(28.5224275940193,586.666345239656,-48.8126989284406)) ;
#62687=CARTESIAN_POINT('Ctrl Pts',(28.4863360466501,586.612564081683,-48.8085843937042)) ;
#62688=CARTESIAN_POINT('Ctrl Pts',(28.4279568623936,586.513566449864,-48.8010610254608)) ;
#62689=CARTESIAN_POINT('Ctrl Pts',(28.404418967938,586.469181383288,-48.7977051784176)) ;
#62690=CARTESIAN_POINT('Ctrl Pts',(28.3480024142957,586.350089594821,-48.7887071723738)) ;
#62691=CARTESIAN_POINT('Ctrl Pts',(28.3185478323463,586.273920507988,-48.7829530214212)) ;
#62692=CARTESIAN_POINT('Ctrl Pts',(28.2669922487746,586.104626910196,-48.7702109246683)) ;
#62693=CARTESIAN_POINT('Ctrl Pts',(28.2470882004441,586.011126920369,-48.7631999164279)) ;
#62694=CARTESIAN_POINT('Ctrl Pts',(28.2304679835342,585.877661701334,-48.7535126220154)) ;
#62695=CARTESIAN_POINT('Ctrl Pts',(28.227004525409,585.838723128789,-48.7507259943334)) ;
#62696=CARTESIAN_POINT('Ctrl Pts',(28.2231776958819,585.767296041769,-48.7457251098162)) ;
#62697=CARTESIAN_POINT('Ctrl Pts',(28.2223884530683,585.734847620626,-48.7434951728177)) ;
#62698=CARTESIAN_POINT('Ctrl Pts',(28.2227240337122,585.666442687974,-48.7389096624418)) ;
#62699=CARTESIAN_POINT('Ctrl Pts',(28.2240639783314,585.630504682275,-48.736565180261)) ;
#62700=CARTESIAN_POINT('Ctrl Pts',(28.2378119829954,585.43341528436,-48.7239246318286)) ;
#62701=CARTESIAN_POINT('Ctrl Pts',(28.2724559474573,585.274676180999,-48.7144649842797)) ;
#62702=CARTESIAN_POINT('Ctrl Pts',(28.3512561311783,585.065438731575,-48.7004641075677)) ;
#62703=CARTESIAN_POINT('Ctrl Pts',(28.3762965010787,585.008747985914,-48.6965108910803)) ;
#62704=CARTESIAN_POINT('Ctrl Pts',(28.4273717777081,584.90861218639,-48.6891317848915)) ;
#62705=CARTESIAN_POINT('Ctrl Pts',(28.4523417666481,584.86470808054,-48.6857478278277)) ;
#62706=CARTESIAN_POINT('Ctrl Pts',(28.5596588195656,584.694501603386,-48.6719682983997)) ;
#62707=CARTESIAN_POINT('Ctrl Pts',(28.6569732335752,584.578517479455,-48.6609732722238)) ;
#62708=CARTESIAN_POINT('Ctrl Pts',(28.8052809840315,584.443837473444,-48.6464230819893)) ;
#62709=CARTESIAN_POINT('Ctrl Pts',(28.8435227762707,584.412109223283,-48.642837843674)) ;
#62710=CARTESIAN_POINT('Ctrl Pts',(28.9131194039447,584.359436159431,-48.6366646784877)) ;
#62711=CARTESIAN_POINT('Ctrl Pts',(28.9438748394614,584.337756919394,-48.6340477808887)) ;
#62712=CARTESIAN_POINT('Ctrl Pts',(29.0017071522415,584.299856403518,-48.6293638583321)) ;
#62713=CARTESIAN_POINT('Ctrl Pts',(29.028558958392,584.283328746974,-48.627280734223)) ;
#62714=CARTESIAN_POINT('Ctrl Pts',(29.1579455116045,584.208667712314,-48.6175964913183)) ;
#62715=CARTESIAN_POINT('Ctrl Pts',(29.2660028768451,584.160753273113,-48.6105096961675)) ;
#62716=CARTESIAN_POINT('Ctrl Pts',(29.442221951244,584.104051306547,-48.5991886678688)) ;
#62717=CARTESIAN_POINT('Ctrl Pts',(29.5074019498371,584.087352992751,-48.5950517058598)) ;
#62718=CARTESIAN_POINT('Ctrl Pts',(29.6296597897424,584.063803169192,-48.5871922612557)) ;
#62719=CARTESIAN_POINT('Ctrl Pts',(29.6864264019397,584.055877426931,-48.5835048295577)) ;
#62720=CARTESIAN_POINT('Ctrl Pts',(29.7949988572825,584.046388953304,-48.5763051782396)) ;
#62721=CARTESIAN_POINT('Ctrl Pts',(29.8466900049273,584.044288276869,-48.5728150229549)) ;
#62722=CARTESIAN_POINT('Ctrl Pts',(30.0345413500177,584.045400398924,-48.5598619412075)) ;
#62723=CARTESIAN_POINT('Ctrl Pts',(30.1700582728422,584.062893874096,-48.5499485511959)) ;
#62724=CARTESIAN_POINT('Ctrl Pts',(30.3529006932756,584.109726391023,-48.536225666219)) ;
#62725=CARTESIAN_POINT('Ctrl Pts',(30.4032513462971,584.125198553051,-48.5324164110218)) ;
#62726=CARTESIAN_POINT('Ctrl Pts',(30.4894467492368,584.156225994577,-48.5259227950453)) ;
#62727=CARTESIAN_POINT('Ctrl Pts',(30.5256357001918,584.17070543898,-48.5232055973716)) ;
#62728=CARTESIAN_POINT('Ctrl Pts',(30.5896520775957,584.198962751141,-48.5184562772016)) ;
#62729=CARTESIAN_POINT('Ctrl Pts',(30.6176620905825,584.212272669135,-48.5164023509664)) ;
#62730=CARTESIAN_POINT('Ctrl Pts',(30.7422349836639,584.275789097501,-48.5073165282251)) ;
#62731=CARTESIAN_POINT('Ctrl Pts',(30.8341215230322,584.334608235735,-48.5007286935346)) ;
#62732=CARTESIAN_POINT('Ctrl Pts',(30.9763833581684,584.446702867174,-48.489668800352)) ;
#62733=CARTESIAN_POINT('Ctrl Pts',(31.0301709562402,584.495070409924,-48.4852441815845)) ;
#62734=CARTESIAN_POINT('Ctrl Pts',(31.1221461897108,584.589284357062,-48.476966073771)) ;
#62735=CARTESIAN_POINT('Ctrl Pts',(31.1613383716971,584.633979402702,-48.4731578284577)) ;
#62736=CARTESIAN_POINT('Ctrl Pts',(31.22922902557,584.720303373162,-48.4659260123143)) ;
#62737=CARTESIAN_POINT('Ctrl Pts',(31.2585820130292,584.761329328733,-48.4625355183699)) ;
#62738=CARTESIAN_POINT('Ctrl Pts',(31.337393397172,584.882768649674,-48.4525926100329)) ;
#62739=CARTESIAN_POINT('Ctrl Pts',(31.3819343939489,584.96612572113,-48.4458671290233)) ;
#62740=CARTESIAN_POINT('Ctrl Pts',(31.4512199610634,585.127354135424,-48.4331435908763)) ;
#62741=CARTESIAN_POINT('Ctrl Pts',(31.4777714568495,585.204159432916,-48.427195361869)) ;
#62742=CARTESIAN_POINT('Ctrl Pts',(31.5113096004686,585.330335151134,-48.4178223601859)) ;
#62743=CARTESIAN_POINT('Ctrl Pts',(31.5218711356606,585.37862203405,-48.4143271422184)) ;
#62744=CARTESIAN_POINT('Ctrl Pts',(31.5353000636259,585.456456457616,-48.4089090160608)) ;
#62745=CARTESIAN_POINT('Ctrl Pts',(31.5395513003226,585.48572785121,-48.4069228541789)) ;
#62746=CARTESIAN_POINT('Ctrl Pts',(31.5493436735007,585.568615969838,-48.4014340330348)) ;
#62747=CARTESIAN_POINT('Ctrl Pts',(31.5530664315368,585.622409624868,-48.398020883997)) ;
#62748=CARTESIAN_POINT('Ctrl Pts',(31.55643863621,585.786309141962,-48.3878199607563)) ;
#62749=CARTESIAN_POINT('Ctrl Pts',(31.547797451983,585.896279176642,-48.3812304434282)) ;
#62750=CARTESIAN_POINT('Ctrl Pts',(31.5156784419345,586.075410171445,-48.3699638980023)) ;
#62751=CARTESIAN_POINT('Ctrl Pts',(31.4984095576746,586.145317801445,-48.3654311046471)) ;
#62752=CARTESIAN_POINT('Ctrl Pts',(31.4689881640764,586.238152638679,-48.3590924580401)) ;
#62753=CARTESIAN_POINT('Ctrl Pts',(31.4607434316487,586.262236314981,-48.3574184609264)) ;
#62754=CARTESIAN_POINT('Ctrl Pts',(31.4519518985791,586.286117540527,-48.355726152802)) ;
#62755=CARTESIAN_POINT('Origin',(179.888527625407,535.710565160536,-51.0680854522974)) ;
#62756=CARTESIAN_POINT('Ctrl Pts',(178.636454050031,537.339770280938,-49.0681970943831)) ;
#62757=CARTESIAN_POINT('Ctrl Pts',(178.542327710974,537.267432488475,-49.0621684907212)) ;
#62758=CARTESIAN_POINT('Ctrl Pts',(178.454647768142,537.187075486664,-49.0564967090507)) ;
#62759=CARTESIAN_POINT('Ctrl Pts',(178.296795779322,537.015004255062,-49.0451737686981)) ;
#62760=CARTESIAN_POINT('Ctrl Pts',(178.226433855834,536.924077643581,-49.0395455094629)) ;
#62761=CARTESIAN_POINT('Ctrl Pts',(178.135310039735,536.783419696863,-49.0308913314428)) ;
#62762=CARTESIAN_POINT('Ctrl Pts',(178.108307493668,536.737991246653,-49.028106053429)) ;
#62763=CARTESIAN_POINT('Ctrl Pts',(178.057607625607,536.644683744705,-49.022374987254)) ;
#62764=CARTESIAN_POINT('Ctrl Pts',(178.033966845089,536.596820840721,-49.0194300557263)) ;
#62765=CARTESIAN_POINT('Ctrl Pts',(177.962776448962,536.437333645756,-49.0095833748824)) ;
#62766=CARTESIAN_POINT('Ctrl Pts',(177.923246874237,536.322426621875,-49.0024193971002)) ;
#62767=CARTESIAN_POINT('Ctrl Pts',(177.866987766582,536.095360924845,-48.9883797828834)) ;
#62768=CARTESIAN_POINT('Ctrl Pts',(177.848931848885,535.983955093438,-48.9815479914339)) ;
#62769=CARTESIAN_POINT('Ctrl Pts',(177.836804776698,535.829720497406,-48.9725576625325)) ;
#62770=CARTESIAN_POINT('Ctrl Pts',(177.834796270281,535.787718764495,-48.9701579616603)) ;
#62771=CARTESIAN_POINT('Ctrl Pts',(177.83357816501,535.716455883667,-48.9662014726683)) ;
#62772=CARTESIAN_POINT('Ctrl Pts',(177.833702239804,535.687225142105,-48.9646136316033)) ;
#62773=CARTESIAN_POINT('Ctrl Pts',(177.835692606149,535.609445264445,-48.9604736885088)) ;
#62774=CARTESIAN_POINT('Ctrl Pts',(177.838656619331,535.560944270059,-48.9579761577606)) ;
#62775=CARTESIAN_POINT('Ctrl Pts',(177.8565806548,535.375778778729,-48.9486128266382)) ;
#62776=CARTESIAN_POINT('Ctrl Pts',(177.883518922326,535.240634029496,-48.9421178793161)) ;
#62777=CARTESIAN_POINT('Ctrl Pts',(177.950998588688,535.020170561269,-48.9308475096296)) ;
#62778=CARTESIAN_POINT('Ctrl Pts',(177.984259739123,534.933117475896,-48.9262118917525)) ;
#62779=CARTESIAN_POINT('Ctrl Pts',(178.04495061424,534.80178355098,-48.9187028320399)) ;
#62780=CARTESIAN_POINT('Ctrl Pts',(178.068351768507,534.755777531711,-48.9159688748401)) ;
#62781=CARTESIAN_POINT('Ctrl Pts',(178.120244690292,534.662613248668,-48.9101884388951)) ;
#62782=CARTESIAN_POINT('Ctrl Pts',(178.14895075701,534.615622587636,-48.9071355627331)) ;
#62783=CARTESIAN_POINT('Ctrl Pts',(178.267581401577,534.437890957758,-48.895025771416)) ;
#62784=CARTESIAN_POINT('Ctrl Pts',(178.370631361474,534.316598532573,-48.8854704416936)) ;
#62785=CARTESIAN_POINT('Ctrl Pts',(178.532510892978,534.165520463416,-48.8721722636474)) ;
#62786=CARTESIAN_POINT('Ctrl Pts',(178.580384473297,534.124782478099,-48.8684188322932)) ;
#62787=CARTESIAN_POINT('Ctrl Pts',(178.665657526472,534.058713124868,-48.8621216119247)) ;
#62788=CARTESIAN_POINT('Ctrl Pts',(178.702163908397,534.03230172305,-48.8595381348249)) ;
#62789=CARTESIAN_POINT('Ctrl Pts',(178.763657146783,533.990823251127,-48.8554058869055)) ;
#62790=CARTESIAN_POINT('Ctrl Pts',(178.788144971627,533.975052538786,-48.8538167890008)) ;
#62791=CARTESIAN_POINT('Ctrl Pts',(178.851230495965,533.93629652699,-48.8498621324231)) ;
#62792=CARTESIAN_POINT('Ctrl Pts',(178.890260028631,533.914047165523,-48.8475392796793)) ;
#62793=CARTESIAN_POINT('Ctrl Pts',(179.05036044178,533.829609950303,-48.8383745189989)) ;
#62794=CARTESIAN_POINT('Ctrl Pts',(179.17674740049,533.778237287736,-48.8319339113943)) ;
#62795=CARTESIAN_POINT('Ctrl Pts',(179.402040691413,533.71179406825,-48.8204859190186)) ;
#62796=CARTESIAN_POINT('Ctrl Pts',(179.498672341653,533.690722193766,-48.8155887901258)) ;
#62797=CARTESIAN_POINT('Ctrl Pts',(179.64791508429,533.669289151764,-48.8077777470804)) ;
#62798=CARTESIAN_POINT('Ctrl Pts',(179.699651023047,533.663853868523,-48.8050272740284)) ;
#62799=CARTESIAN_POINT('Ctrl Pts',(179.805824777175,533.656759330293,-48.7992684846683)) ;
#62800=CARTESIAN_POINT('Ctrl Pts',(179.860233484665,533.655289804287,-48.7962563727491)) ;
#62801=CARTESIAN_POINT('Ctrl Pts',(180.060831435104,533.65783858587,-48.7849090068978)) ;
#62802=CARTESIAN_POINT('Ctrl Pts',(180.206395009497,533.675295226187,-48.7761617775762)) ;
#62803=CARTESIAN_POINT('Ctrl Pts',(180.418356560313,533.724019094757,-48.7630829499242)) ;
#62804=CARTESIAN_POINT('Ctrl Pts',(180.486986681768,533.743605190038,-48.758800857569)) ;
#62805=CARTESIAN_POINT('Ctrl Pts',(180.600415187797,533.782464218616,-48.7517703501032)) ;
#62806=CARTESIAN_POINT('Ctrl Pts',(180.645799812939,533.799833179317,-48.7489710346728)) ;
#62807=CARTESIAN_POINT('Ctrl Pts',(180.717440523858,533.830204730404,-48.7446213841963)) ;
#62808=CARTESIAN_POINT('Ctrl Pts',(180.744105244593,533.842186404612,-48.743019913562)) ;
#62809=CARTESIAN_POINT('Ctrl Pts',(180.808484487784,533.87278260655,-48.7391991236654)) ;
#62810=CARTESIAN_POINT('Ctrl Pts',(180.845898957911,533.891992650726,-48.7370132501454)) ;
#62811=CARTESIAN_POINT('Ctrl Pts',(181.000076963651,533.977231923506,-48.7280453755306)) ;
#62812=CARTESIAN_POINT('Ctrl Pts',(181.110827040934,534.053466505995,-48.7216838029734)) ;
#62813=CARTESIAN_POINT('Ctrl Pts',(181.269343003033,534.187177494918,-48.7116001408561)) ;
#62814=CARTESIAN_POINT('Ctrl Pts',(181.322755927236,534.237354603126,-48.7080023363249)) ;
#62815=CARTESIAN_POINT('Ctrl Pts',(181.415897884025,534.334730027453,-48.70119524651)) ;
#62816=CARTESIAN_POINT('Ctrl Pts',(181.456400456788,534.381070506793,-48.6980198342083)) ;
#62817=CARTESIAN_POINT('Ctrl Pts',(181.525934523147,534.468230711574,-48.692104578938)) ;
#62818=CARTESIAN_POINT('Ctrl Pts',(181.555669429729,534.508427971447,-48.6893969376608)) ;
#62819=CARTESIAN_POINT('Ctrl Pts',(181.624023351724,534.608252295365,-48.6827023965866)) ;
#62820=CARTESIAN_POINT('Ctrl Pts',(181.661071639527,534.668871785708,-48.6786597196493)) ;
#62821=CARTESIAN_POINT('Ctrl Pts',(181.763938740653,534.858619681276,-48.6660864400596)) ;
#62822=CARTESIAN_POINT('Ctrl Pts',(181.819309924628,534.992894583591,-48.6572660636923)) ;
#62823=CARTESIAN_POINT('Ctrl Pts',(181.879379417516,535.197541619153,-48.6445552557715)) ;
#62824=CARTESIAN_POINT('Ctrl Pts',(181.895367130346,535.26415639492,-48.6405325459092)) ;
#62825=CARTESIAN_POINT('Ctrl Pts',(181.913699937431,535.361811682268,-48.634912396563)) ;
#62826=CARTESIAN_POINT('Ctrl Pts',(181.918714878817,535.392301082679,-48.6331966618825)) ;
#62827=CARTESIAN_POINT('Ctrl Pts',(181.927966025126,535.457728881311,-48.629613135694)) ;
#62828=CARTESIAN_POINT('Ctrl Pts',(181.931996191779,535.492685115481,-48.627755627963)) ;
#62829=CARTESIAN_POINT('Ctrl Pts',(181.947227091345,535.663174854721,-48.6188993033526)) ;
#62830=CARTESIAN_POINT('Ctrl Pts',(181.945852949278,535.799500654536,-48.6124229137948)) ;
#62831=CARTESIAN_POINT('Ctrl Pts',(181.922365983171,536.013530295561,-48.6019847066371)) ;
#62832=CARTESIAN_POINT('Ctrl Pts',(181.909159696295,536.091788707267,-48.5981130198768)) ;
#62833=CARTESIAN_POINT('Ctrl Pts',(181.877106418538,536.231806048838,-48.5908917623806)) ;
#62834=CARTESIAN_POINT('Ctrl Pts',(181.859810998182,536.293813363811,-48.5875861792547)) ;
#62835=CARTESIAN_POINT('Ctrl Pts',(181.824006354894,536.402232700357,-48.5815496659751)) ;
#62836=CARTESIAN_POINT('Ctrl Pts',(181.80666045951,536.448974073297,-48.5788594790524)) ;
#62837=CARTESIAN_POINT('Ctrl Pts',(181.762036317524,536.557003540419,-48.5724143353593)) ;
#62838=CARTESIAN_POINT('Ctrl Pts',(181.7334239354,536.617675355295,-48.5686154819313)) ;
#62839=CARTESIAN_POINT('Ctrl Pts',(181.63271996048,536.806663580111,-48.5562035521406)) ;
#62840=CARTESIAN_POINT('Ctrl Pts',(181.549801374464,536.928678549378,-48.5472607754822)) ;
#62841=CARTESIAN_POINT('Ctrl Pts',(181.407306384613,537.096437276941,-48.5341137218446)) ;
#62842=CARTESIAN_POINT('Ctrl Pts',(181.357092275105,537.149540529168,-48.5298080754178)) ;
#62843=CARTESIAN_POINT('Ctrl Pts',(181.281485390623,537.221407412791,-48.5238984437335)) ;
#62844=CARTESIAN_POINT('Ctrl Pts',(181.258326345418,537.242435756466,-48.5221585157646)) ;
#62845=CARTESIAN_POINT('Ctrl Pts',(181.208618406476,537.285541064528,-48.5185850498275)) ;
#62846=CARTESIAN_POINT('Ctrl Pts',(181.181975882962,537.307493676342,-48.5167593004295)) ;
#62847=CARTESIAN_POINT('Ctrl Pts',(181.043600486761,537.415774257984,-48.5076503615033)) ;
#62848=CARTESIAN_POINT('Ctrl Pts',(180.923726042842,537.491099983794,-48.5009428001874)) ;
#62849=CARTESIAN_POINT('Ctrl Pts',(180.698429482008,537.602164841813,-48.4887570785792)) ;
#62850=CARTESIAN_POINT('Ctrl Pts',(180.596058661144,537.642788524634,-48.4833572372502)) ;
#62851=CARTESIAN_POINT('Ctrl Pts',(180.440124522023,537.690606352748,-48.4749459309971)) ;
#62852=CARTESIAN_POINT('Ctrl Pts',(180.388730237061,537.704209792353,-48.4721474456496)) ;
#62853=CARTESIAN_POINT('Ctrl Pts',(180.285135981776,537.727371919115,-48.4664246655478)) ;
#62854=CARTESIAN_POINT('Ctrl Pts',(180.232978296029,537.736931535074,-48.4635028946538)) ;
#62855=CARTESIAN_POINT('Ctrl Pts',(180.061413179173,537.761561294265,-48.4537433732945)) ;
#62856=CARTESIAN_POINT('Ctrl Pts',(179.941058030172,537.768162804701,-48.4466469575906)) ;
#62857=CARTESIAN_POINT('Ctrl Pts',(179.685782989789,537.759747996101,-48.4313271939612)) ;
#62858=CARTESIAN_POINT('Ctrl Pts',(179.551496092749,537.741985659295,-48.4231086697372)) ;
#62859=CARTESIAN_POINT('Ctrl Pts',(179.387676844545,537.703613770197,-48.413518022559)) ;
#62860=CARTESIAN_POINT('Ctrl Pts',(179.355618173539,537.695282286733,-48.4116639825675)) ;
#62861=CARTESIAN_POINT('Ctrl Pts',(179.292723724043,537.677303095676,-48.4080911972685)) ;
#62862=CARTESIAN_POINT('Ctrl Pts',(179.26188651879,537.66769610399,-48.4063712621669)) ;
#62863=CARTESIAN_POINT('Ctrl Pts',(179.147036168478,537.628922584521,-48.4000418752808)) ;
#62864=CARTESIAN_POINT('Ctrl Pts',(179.06471211879,537.595037439013,-48.3956580320164)) ;
#62865=CARTESIAN_POINT('Ctrl Pts',(178.861732865358,537.495636268589,-48.3846614012211)) ;
#62866=CARTESIAN_POINT('Ctrl Pts',(178.745034004208,537.423215937803,-48.3781367500008)) ;
#62867=CARTESIAN_POINT('Ctrl Pts',(178.636454050035,537.339770280941,-48.3712393117967)) ;
#62868=CARTESIAN_POINT('Ctrl Pts',(178.636454050048,537.339770280952,-48.4293891818575)) ;
#62869=CARTESIAN_POINT('Ctrl Pts',(178.636971408351,537.340167880156,-48.4294210284128)) ;
#62870=CARTESIAN_POINT('Ctrl Pts',(178.637488959893,537.340565235887,-48.4294528708969)) ;
#62871=CARTESIAN_POINT('Ctrl Pts',(178.780097725288,537.449946708084,-48.4382225368371)) ;
#62872=CARTESIAN_POINT('Ctrl Pts',(178.935813278076,537.539881613079,-48.4466864846988)) ;
#62873=CARTESIAN_POINT('Ctrl Pts',(179.149382963027,537.628476018642,-48.4586434944128)) ;
#62874=CARTESIAN_POINT('Ctrl Pts',(179.19829007531,537.646614839493,-48.4613963560147)) ;
#62875=CARTESIAN_POINT('Ctrl Pts',(179.298549919782,537.679517489769,-48.4670969686892)) ;
#62876=CARTESIAN_POINT('Ctrl Pts',(179.349893935389,537.69417801563,-48.4700456192522)) ;
#62877=CARTESIAN_POINT('Ctrl Pts',(179.519851071119,537.735621469847,-48.4799174054492)) ;
#62878=CARTESIAN_POINT('Ctrl Pts',(179.640262191138,537.753879282824,-48.4871033321921)) ;
#62879=CARTESIAN_POINT('Ctrl Pts',(179.89110237037,537.769408324738,-48.5021891641325)) ;
#62880=CARTESIAN_POINT('Ctrl Pts',(180.021114633496,537.76513718705,-48.5100694564814)) ;
#62881=CARTESIAN_POINT('Ctrl Pts',(180.183045563217,537.744373440327,-48.5193885071454)) ;
#62882=CARTESIAN_POINT('Ctrl Pts',(180.216124256574,537.739308041724,-48.521264432017)) ;
#62883=CARTESIAN_POINT('Ctrl Pts',(180.280196624903,537.727888342959,-48.5248243783715)) ;
#62884=CARTESIAN_POINT('Ctrl Pts',(180.311195563918,537.721621945074,-48.5265117823724)) ;
#62885=CARTESIAN_POINT('Ctrl Pts',(180.419294269943,537.697159832723,-48.5323110754626)) ;
#62886=CARTESIAN_POINT('Ctrl Pts',(180.495481631618,537.675223071724,-48.5362471587008)) ;
#62887=CARTESIAN_POINT('Ctrl Pts',(180.743906180651,537.587856790418,-48.5491190278353)) ;
#62888=CARTESIAN_POINT('Ctrl Pts',(180.908584110323,537.503713271122,-48.5577974545466)) ;
#62889=CARTESIAN_POINT('Ctrl Pts',(181.102539616882,537.369140397392,-48.5700155075771)) ;
#62890=CARTESIAN_POINT('Ctrl Pts',(181.144084836481,537.337916496415,-48.5727604521371)) ;
#62891=CARTESIAN_POINT('Ctrl Pts',(181.226037430217,537.271316176251,-48.5784694697332)) ;
#62892=CARTESIAN_POINT('Ctrl Pts',(181.266330419729,537.235863460076,-48.581435588996)) ;
#62893=CARTESIAN_POINT('Ctrl Pts',(181.353808703011,537.152596646698,-48.5882564558795)) ;
#62894=CARTESIAN_POINT('Ctrl Pts',(181.400128732297,537.1039653957,-48.5921438162043)) ;
#62895=CARTESIAN_POINT('Ctrl Pts',(181.53230899464,536.950828532717,-48.6040700566887)) ;
#62896=CARTESIAN_POINT('Ctrl Pts',(181.610315525784,536.840040140144,-48.6123146745958)) ;
#62897=CARTESIAN_POINT('Ctrl Pts',(181.70614253534,536.670672330255,-48.6238455357941)) ;
#62898=CARTESIAN_POINT('Ctrl Pts',(181.733153573353,536.617695803122,-48.6273117274549)) ;
#62899=CARTESIAN_POINT('Ctrl Pts',(181.770259725125,536.536384764315,-48.6323471814532)) ;
#62900=CARTESIAN_POINT('Ctrl Pts',(181.782092367469,536.508880071567,-48.6340027366087)) ;
#62901=CARTESIAN_POINT('Ctrl Pts',(181.807064850906,536.447148879245,-48.6376012347852)) ;
#62902=CARTESIAN_POINT('Ctrl Pts',(181.819897969242,536.412811280288,-48.6395279238708)) ;
#62903=CARTESIAN_POINT('Ctrl Pts',(181.846605937451,536.335066409508,-48.6437621246174)) ;
#62904=CARTESIAN_POINT('Ctrl Pts',(181.859969572937,536.291503686283,-48.6460474120062)) ;
#62905=CARTESIAN_POINT('Ctrl Pts',(181.903291734283,536.131488033617,-48.6542426215403)) ;
#62906=CARTESIAN_POINT('Ctrl Pts',(181.924464708046,536.01291003996,-48.659950998467)) ;
#62907=CARTESIAN_POINT('Ctrl Pts',(181.943090230063,535.804143040914,-48.6702165823836)) ;
#62908=CARTESIAN_POINT('Ctrl Pts',(181.945215475097,535.714712803232,-48.6746791616568)) ;
#62909=CARTESIAN_POINT('Ctrl Pts',(181.939396636824,535.574389554094,-48.68197639383)) ;
#62910=CARTESIAN_POINT('Ctrl Pts',(181.935377235313,535.523446093756,-48.6846857933659)) ;
#62911=CARTESIAN_POINT('Ctrl Pts',(181.923090441906,535.418019053855,-48.6904432295553)) ;
#62912=CARTESIAN_POINT('Ctrl Pts',(181.914521731202,535.363612522553,-48.6934989588403)) ;
#62913=CARTESIAN_POINT('Ctrl Pts',(181.881078947393,535.195521010333,-48.7032176551853)) ;
#62914=CARTESIAN_POINT('Ctrl Pts',(181.848732447318,535.083570532672,-48.7101061513494)) ;
#62915=CARTESIAN_POINT('Ctrl Pts',(181.761288957932,534.855501686841,-48.7247698132129)) ;
#62916=CARTESIAN_POINT('Ctrl Pts',(181.704422434309,534.740566048844,-48.7325330824152)) ;
#62917=CARTESIAN_POINT('Ctrl Pts',(181.619591387979,534.603070477832,-48.7417581963727)) ;
#62918=CARTESIAN_POINT('Ctrl Pts',(181.601251361125,534.574913838014,-48.7436425089385)) ;
#62919=CARTESIAN_POINT('Ctrl Pts',(181.56438689509,534.52124340208,-48.7472050893983)) ;
#62920=CARTESIAN_POINT('Ctrl Pts',(181.545950176528,534.495681972897,-48.7488872653828)) ;
#62921=CARTESIAN_POINT('Ctrl Pts',(181.480047069673,534.408605392416,-48.7546034202228)) ;
#62922=CARTESIAN_POINT('Ctrl Pts',(181.429681854904,534.349360116707,-48.7584687418977)) ;
#62923=CARTESIAN_POINT('Ctrl Pts',(181.273963861487,534.185942174509,-48.7695102238633)) ;
#62924=CARTESIAN_POINT('Ctrl Pts',(181.160573000626,534.090130181396,-48.7765146665075)) ;
#62925=CARTESIAN_POINT('Ctrl Pts',(180.984912313923,533.971594213003,-48.7871719685216)) ;
#62926=CARTESIAN_POINT('Ctrl Pts',(180.930319458856,533.938349581176,-48.790455091714)) ;
#62927=CARTESIAN_POINT('Ctrl Pts',(180.830786329668,533.883928308802,-48.7964528939476)) ;
#62928=CARTESIAN_POINT('Ctrl Pts',(180.786459782168,533.861735557778,-48.7991275880171)) ;
#62929=CARTESIAN_POINT('Ctrl Pts',(180.680817007635,533.813539615423,-48.8055292643042)) ;
#62930=CARTESIAN_POINT('Ctrl Pts',(180.618955979563,533.788872837457,-48.8092993194072)) ;
#62931=CARTESIAN_POINT('Ctrl Pts',(180.389830696127,533.710173452179,-48.8233338555193)) ;
#62932=CARTESIAN_POINT('Ctrl Pts',(180.217041684975,533.674653078495,-48.8341250616248)) ;
#62933=CARTESIAN_POINT('Ctrl Pts',(179.989017568001,533.657590038913,-48.8475964982882)) ;
#62934=CARTESIAN_POINT('Ctrl Pts',(179.936041739681,533.655681131174,-48.8506661055594)) ;
#62935=CARTESIAN_POINT('Ctrl Pts',(179.853655294818,533.655900858353,-48.8552882948924)) ;
#62936=CARTESIAN_POINT('Ctrl Pts',(179.824266671069,533.656609860909,-48.856905972248)) ;
#62937=CARTESIAN_POINT('Ctrl Pts',(179.755849666641,533.659730669324,-48.860591705264)) ;
#62938=CARTESIAN_POINT('Ctrl Pts',(179.716856847382,533.662625925228,-48.8626355136992)) ;
#62939=CARTESIAN_POINT('Ctrl Pts',(179.568071522617,533.677953338839,-48.8702955296407)) ;
#62940=CARTESIAN_POINT('Ctrl Pts',(179.459258029982,533.698120245836,-48.8756148325543)) ;
#62941=CARTESIAN_POINT('Ctrl Pts',(179.228026559658,533.760594960374,-48.8872078832518)) ;
#62942=CARTESIAN_POINT('Ctrl Pts',(179.106919887448,533.80590482709,-48.89347780094)) ;
#62943=CARTESIAN_POINT('Ctrl Pts',(178.943213025649,533.885411792385,-48.9028593082998)) ;
#62944=CARTESIAN_POINT('Ctrl Pts',(178.896471964068,533.910390337433,-48.9056474956303)) ;
#62945=CARTESIAN_POINT('Ctrl Pts',(178.805490493409,533.963631240722,-48.9113271240036)) ;
#62946=CARTESIAN_POINT('Ctrl Pts',(178.761264010578,533.99183784831,-48.9142150947648)) ;
#62947=CARTESIAN_POINT('Ctrl Pts',(178.626669037012,534.085110493024,-48.9234270354854)) ;
#62948=CARTESIAN_POINT('Ctrl Pts',(178.540486606791,534.155840212777,-48.9299639722328)) ;
#62949=CARTESIAN_POINT('Ctrl Pts',(178.358085762492,534.332152980644,-48.9451470628023)) ;
#62950=CARTESIAN_POINT('Ctrl Pts',(178.266268253122,534.441490734593,-48.9538406640168)) ;
#62951=CARTESIAN_POINT('Ctrl Pts',(178.16730741226,534.587813506215,-48.9639471366811)) ;
#62952=CARTESIAN_POINT('Ctrl Pts',(178.148833270806,534.616657410548,-48.9658716624541)) ;
#62953=CARTESIAN_POINT('Ctrl Pts',(178.115042963914,534.672437679025,-48.9694461467811)) ;
#62954=CARTESIAN_POINT('Ctrl Pts',(178.099598845633,534.699283587368,-48.9711026825243)) ;
#62955=CARTESIAN_POINT('Ctrl Pts',(178.050707002889,534.788897992079,-48.9764573449579)) ;
#62956=CARTESIAN_POINT('Ctrl Pts',(178.019907961577,534.853058713529,-48.9800162413306)) ;
#62957=CARTESIAN_POINT('Ctrl Pts',(177.930404605978,535.067362316777,-48.9914230800628)) ;
#62958=CARTESIAN_POINT('Ctrl Pts',(177.886015249744,535.222814075474,-48.9990057158956)) ;
#62959=CARTESIAN_POINT('Ctrl Pts',(177.850398961521,535.442584475366,-49.0102419279424)) ;
#62960=CARTESIAN_POINT('Ctrl Pts',(177.843290433788,535.503717489371,-49.0134140804978)) ;
#62961=CARTESIAN_POINT('Ctrl Pts',(177.83544145771,535.614289026611,-49.0192895888663)) ;
#62962=CARTESIAN_POINT('Ctrl Pts',(177.833721894218,535.663610719697,-49.0219592191754)) ;
#62963=CARTESIAN_POINT('Ctrl Pts',(177.833858254744,535.781406596256,-49.0284696142769)) ;
#62964=CARTESIAN_POINT('Ctrl Pts',(177.837359097982,535.849816219465,-49.0323600333312)) ;
#62965=CARTESIAN_POINT('Ctrl Pts',(177.857248770573,536.045905170736,-49.0438188647945)) ;
#62966=CARTESIAN_POINT('Ctrl Pts',(177.882220800885,536.172381287622,-49.0516067850136)) ;
#62967=CARTESIAN_POINT('Ctrl Pts',(177.941698773642,536.372603416275,-49.0641531800656)) ;
#62968=CARTESIAN_POINT('Ctrl Pts',(177.969038821971,536.448130014332,-49.068932319098)) ;
#62969=CARTESIAN_POINT('Ctrl Pts',(178.014183418213,536.553175701456,-49.0754770465997)) ;
#62970=CARTESIAN_POINT('Ctrl Pts',(178.028415695389,536.584145522984,-49.077392895849)) ;
#62971=CARTESIAN_POINT('Ctrl Pts',(178.057235292496,536.642955988185,-49.0809840392975)) ;
#62972=CARTESIAN_POINT('Ctrl Pts',(178.071703392011,536.670843303878,-49.0826649097805)) ;
#62973=CARTESIAN_POINT('Ctrl Pts',(178.122411753081,536.763331824808,-49.0882002710017)) ;
#62974=CARTESIAN_POINT('Ctrl Pts',(178.16150626327,536.82630797845,-49.0919048209158)) ;
#62975=CARTESIAN_POINT('Ctrl Pts',(178.297112211223,537.020483729812,-49.10354519564)) ;
#62976=CARTESIAN_POINT('Ctrl Pts',(178.40582557567,537.142376886713,-49.1112419490159)) ;
#62977=CARTESIAN_POINT('Ctrl Pts',(178.562993620517,537.281286422608,-49.1219018392419)) ;
#62978=CARTESIAN_POINT('Ctrl Pts',(178.599258286014,537.311186851907,-49.1243301742461)) ;
#62979=CARTESIAN_POINT('Ctrl Pts',(178.63651424806,537.339816542443,-49.1268080620001)) ;
#62980=CARTESIAN_POINT('Origin',(29.8885276254068,535.710565160562,-51.0680854522906)) ;
#62981=CARTESIAN_POINT('',(31.9432771690465,535.708946382626,-48.6168383787018)) ;
#62982=CARTESIAN_POINT('Ctrl Pts',(28.6364362889498,537.339756631099,-49.0682055192064)) ;
#62983=CARTESIAN_POINT('Ctrl Pts',(28.6324425150367,537.336687274423,-49.0679497338304)) ;
#62984=CARTESIAN_POINT('Ctrl Pts',(28.6284598996157,537.333603134144,-49.0676945819357)) ;
#62985=CARTESIAN_POINT('Ctrl Pts',(28.51677826253,537.246457910494,-49.0605360378214)) ;
#62986=CARTESIAN_POINT('Ctrl Pts',(28.4177123018037,537.151873699214,-49.0540733584487)) ;
#62987=CARTESIAN_POINT('Ctrl Pts',(28.2657666768744,536.97468919814,-49.042685031261)) ;
#62988=CARTESIAN_POINT('Ctrl Pts',(28.2080430766881,536.89687532036,-49.0378797303259)) ;
#62989=CARTESIAN_POINT('Ctrl Pts',(28.1281316220551,536.771552535011,-49.0301745650768)) ;
#62990=CARTESIAN_POINT('Ctrl Pts',(28.1019109186819,536.72677792836,-49.0274294076523)) ;
#62991=CARTESIAN_POINT('Ctrl Pts',(28.0516125755643,536.632912548862,-49.0216629927892)) ;
#62992=CARTESIAN_POINT('Ctrl Pts',(28.0277438456033,536.583757304117,-49.0186370725674)) ;
#62993=CARTESIAN_POINT('Ctrl Pts',(27.9483571866116,536.402187847095,-49.0074208738758)) ;
#62994=CARTESIAN_POINT('Ctrl Pts',(27.9047996613618,536.265015932918,-48.9988384691246)) ;
#62995=CARTESIAN_POINT('Ctrl Pts',(27.8545262406192,536.020546151499,-48.9838273769015)) ;
#62996=CARTESIAN_POINT('Ctrl Pts',(27.8412358140034,535.915136749459,-48.9774553494339)) ;
#62997=CARTESIAN_POINT('Ctrl Pts',(27.8345687442573,535.776361161162,-48.9695417164412)) ;
#62998=CARTESIAN_POINT('Ctrl Pts',(27.8337793709737,535.743521102824,-48.9677043882939)) ;
#62999=CARTESIAN_POINT('Ctrl Pts',(27.8337759013759,535.67812415242,-48.9641348791646)) ;
#63000=CARTESIAN_POINT('Ctrl Pts',(27.8345476296576,535.645576735634,-48.962402611237)) ;
#63001=CARTESIAN_POINT('Ctrl Pts',(27.8405969987939,535.518241148965,-48.9557517569802)) ;
#63002=CARTESIAN_POINT('Ctrl Pts',(27.851667278428,535.423839206406,-48.9510924372246)) ;
#63003=CARTESIAN_POINT('Ctrl Pts',(27.8990110077315,535.172277947907,-48.9386604529326)) ;
#63004=CARTESIAN_POINT('Ctrl Pts',(27.9472912575291,535.018085829451,-48.9309784834429)) ;
#63005=CARTESIAN_POINT('Ctrl Pts',(28.0348116369868,534.822553301613,-48.9199338804978)) ;
#63006=CARTESIAN_POINT('Ctrl Pts',(28.0584231785513,534.774859517256,-48.9171333661)) ;
#63007=CARTESIAN_POINT('Ctrl Pts',(28.1091407291144,534.681693853697,-48.9114161674706)) ;
#63008=CARTESIAN_POINT('Ctrl Pts',(28.1362057121994,534.636246274519,-48.9085024603027)) ;
#63009=CARTESIAN_POINT('Ctrl Pts',(28.2286148084511,534.493871405869,-48.8989480131398)) ;
#63010=CARTESIAN_POINT('Ctrl Pts',(28.30047605584,534.401466254605,-48.8920668280111)) ;
#63011=CARTESIAN_POINT('Ctrl Pts',(28.4752737908205,534.212401433728,-48.876633558149)) ;
#63012=CARTESIAN_POINT('Ctrl Pts',(28.581113391671,534.119196927386,-48.8680620072579)) ;
#63013=CARTESIAN_POINT('Ctrl Pts',(28.7221750027698,534.018619385244,-48.8582014538988)) ;
#63014=CARTESIAN_POINT('Ctrl Pts',(28.7491495677121,534.000338016805,-48.8563802461583)) ;
#63015=CARTESIAN_POINT('Ctrl Pts',(28.8041220381912,533.964960046678,-48.8528144706223)) ;
#63016=CARTESIAN_POINT('Ctrl Pts',(28.8321173586955,533.947876783207,-48.8510708699381)) ;
#63017=CARTESIAN_POINT('Ctrl Pts',(28.9499475578021,533.879790849504,-48.8439769161771)) ;
#63018=CARTESIAN_POINT('Ctrl Pts',(29.0431628404374,533.83492400264,-48.8389371565802)) ;
#63019=CARTESIAN_POINT('Ctrl Pts',(29.2767405583929,533.743465911539,-48.8267790113076)) ;
#63020=CARTESIAN_POINT('Ctrl Pts',(29.4194970411273,533.704631513566,-48.8197028533382)) ;
#63021=CARTESIAN_POINT('Ctrl Pts',(29.6187965722154,533.672872678016,-48.8093352506182)) ;
#63022=CARTESIAN_POINT('Ctrl Pts',(29.6727287167303,533.666457628644,-48.8064870501227)) ;
#63023=CARTESIAN_POINT('Ctrl Pts',(29.7787379813608,533.658090293649,-48.8007724108854)) ;
#63024=CARTESIAN_POINT('Ctrl Pts',(29.830760445896,533.655968096278,-48.7979137395599)) ;
#63025=CARTESIAN_POINT('Ctrl Pts',(29.9824955487993,533.65554544796,-48.7894009621829)) ;
#63026=CARTESIAN_POINT('Ctrl Pts',(30.0820626933322,533.662523190496,-48.7835877643077)) ;
#63027=CARTESIAN_POINT('Ctrl Pts',(30.3151523885225,533.696009649856,-48.769562464539)) ;
#63028=CARTESIAN_POINT('Ctrl Pts',(30.4473363445353,533.72860262887,-48.7612678171605)) ;
#63029=CARTESIAN_POINT('Ctrl Pts',(30.6171791367185,533.788837952158,-48.7507588141903)) ;
#63030=CARTESIAN_POINT('Ctrl Pts',(30.6585320936462,533.805030538939,-48.7482151736987)) ;
#63031=CARTESIAN_POINT('Ctrl Pts',(30.7260980516117,533.834046583491,-48.7441218990153)) ;
#63032=CARTESIAN_POINT('Ctrl Pts',(30.7526162537398,533.846108877327,-48.74253395379)) ;
#63033=CARTESIAN_POINT('Ctrl Pts',(30.819970134706,533.878492087609,-48.738545449447)) ;
#63034=CARTESIAN_POINT('Ctrl Pts',(30.8604005153898,533.899614972793,-48.7361898069779)) ;
#63035=CARTESIAN_POINT('Ctrl Pts',(30.955898902664,533.953628603919,-48.7306414550289)) ;
#63036=CARTESIAN_POINT('Ctrl Pts',(31.010195932004,533.987785849383,-48.7274994543444)) ;
#63037=CARTESIAN_POINT('Ctrl Pts',(31.1981508725158,534.118683852124,-48.7163686221103)) ;
#63038=CARTESIAN_POINT('Ctrl Pts',(31.3216407479201,534.228882736553,-48.7085137277512)) ;
#63039=CARTESIAN_POINT('Ctrl Pts',(31.4655997208718,534.392368978522,-48.6972711351371)) ;
#63040=CARTESIAN_POINT('Ctrl Pts',(31.4990198184368,534.433415293354,-48.6944828469524)) ;
#63041=CARTESIAN_POINT('Ctrl Pts',(31.5627846218381,534.518218501526,-48.6887591937053)) ;
#63042=CARTESIAN_POINT('Ctrl Pts',(31.5930870619016,534.561955817211,-48.6858253189656)) ;
#63043=CARTESIAN_POINT('Ctrl Pts',(31.6856910679613,534.707364593144,-48.6761112697115)) ;
#63044=CARTESIAN_POINT('Ctrl Pts',(31.7408456107136,534.81328088647,-48.6690796140408)) ;
#63045=CARTESIAN_POINT('Ctrl Pts',(31.8384573846933,535.048627739519,-48.6537975852015)) ;
#63046=CARTESIAN_POINT('Ctrl Pts',(31.8778850749625,535.178730600246,-48.6455482266552)) ;
#63047=CARTESIAN_POINT('Ctrl Pts',(31.9106149382367,535.344162998822,-48.6359380080728)) ;
#63048=CARTESIAN_POINT('Ctrl Pts',(31.9162416944623,535.376703532573,-48.6340900384243)) ;
#63049=CARTESIAN_POINT('Ctrl Pts',(31.9258295824852,535.441404932666,-48.6305183482567)) ;
#63050=CARTESIAN_POINT('Ctrl Pts',(31.9298192211171,535.473551783346,-48.6287938333755)) ;
#63051=CARTESIAN_POINT('Ctrl Pts',(31.9398089868692,535.573287498696,-48.6235614691451)) ;
#63052=CARTESIAN_POINT('Ctrl Pts',(31.9432235565964,535.64109270422,-48.6201703425734)) ;
#63053=CARTESIAN_POINT('Ctrl Pts',(31.9432769883604,535.708947154935,-48.6168380267463)) ;
#63054=CARTESIAN_POINT('Ctrl Pts',(31.9432769877401,535.708946367384,-48.6168380654227)) ;
#63055=CARTESIAN_POINT('Ctrl Pts',(31.9433994816354,535.864429017549,-48.6092023486022)) ;
#63056=CARTESIAN_POINT('Ctrl Pts',(31.9258746531393,536.019420798674,-48.6018725754436)) ;
#63057=CARTESIAN_POINT('Ctrl Pts',(31.8766814814539,536.233389829389,-48.5908301659164)) ;
#63058=CARTESIAN_POINT('Ctrl Pts',(31.859417119639,536.295111929032,-48.5875377078832)) ;
#63059=CARTESIAN_POINT('Ctrl Pts',(31.8236473630234,536.403235796962,-48.581514804191)) ;
#63060=CARTESIAN_POINT('Ctrl Pts',(31.8062804514816,536.44995984631,-48.5788242838928)) ;
#63061=CARTESIAN_POINT('Ctrl Pts',(31.7614976556292,536.5582169947,-48.5723623498924)) ;
#63062=CARTESIAN_POINT('Ctrl Pts',(31.7327221843561,536.619121888355,-48.5685461748127)) ;
#63063=CARTESIAN_POINT('Ctrl Pts',(31.6298850923612,536.811687078903,-48.5558881187871)) ;
#63064=CARTESIAN_POINT('Ctrl Pts',(31.5442977966927,536.936620651887,-48.5466946167372)) ;
#63065=CARTESIAN_POINT('Ctrl Pts',(31.4004416894612,537.103745188659,-48.5335453159337)) ;
#63066=CARTESIAN_POINT('Ctrl Pts',(31.3524180486736,537.154123674196,-48.5294550128805)) ;
#63067=CARTESIAN_POINT('Ctrl Pts',(31.2794410996137,537.223283600136,-48.5237657056771)) ;
#63068=CARTESIAN_POINT('Ctrl Pts',(31.2564728611837,537.244085171439,-48.522044267435)) ;
#63069=CARTESIAN_POINT('Ctrl Pts',(31.2065821095409,537.287256036464,-48.5184648764438)) ;
#63070=CARTESIAN_POINT('Ctrl Pts',(31.1795418673164,537.309472377918,-48.5166165292592)) ;
#63071=CARTESIAN_POINT('Ctrl Pts',(31.0435489340074,537.415503873464,-48.50768938979)) ;
#63072=CARTESIAN_POINT('Ctrl Pts',(30.926934016215,537.488938109116,-48.501147638137)) ;
#63073=CARTESIAN_POINT('Ctrl Pts',(30.7017056914125,537.601002973052,-48.4889493883153)) ;
#63074=CARTESIAN_POINT('Ctrl Pts',(30.595514389154,537.643226552039,-48.4833532886448)) ;
#63075=CARTESIAN_POINT('Ctrl Pts',(30.4358719594056,537.69177648773,-48.4747370646156)) ;
#63076=CARTESIAN_POINT('Ctrl Pts',(30.384798153687,537.705182674746,-48.4719540982873)) ;
#63077=CARTESIAN_POINT('Ctrl Pts',(30.2811864843987,537.728153412873,-48.4662266093179)) ;
#63078=CARTESIAN_POINT('Ctrl Pts',(30.2286792967238,537.737666396398,-48.4632828832545)) ;
#63079=CARTESIAN_POINT('Ctrl Pts',(30.017917873202,537.767431832564,-48.4512830000069)) ;
#63080=CARTESIAN_POINT('Ctrl Pts',(29.8579320127544,537.771266737994,-48.4417077840596)) ;
#63081=CARTESIAN_POINT('Ctrl Pts',(29.6036802310208,537.747732561675,-48.4263631350217)) ;
#63082=CARTESIAN_POINT('Ctrl Pts',(29.5089433938644,537.732224836442,-48.4206330006412)) ;
#63083=CARTESIAN_POINT('Ctrl Pts',(29.383919780426,537.702657086295,-48.4133213628132)) ;
#63084=CARTESIAN_POINT('Ctrl Pts',(29.3523905594172,537.694404028775,-48.4114999668074)) ;
#63085=CARTESIAN_POINT('Ctrl Pts',(29.289560406237,537.67635014148,-48.4079344305652)) ;
#63086=CARTESIAN_POINT('Ctrl Pts',(29.2582710338655,537.666542978867,-48.406191258963)) ;
#63087=CARTESIAN_POINT('Ctrl Pts',(29.0960265949812,537.611391948595,-48.3972592222333)) ;
#63088=CARTESIAN_POINT('Ctrl Pts',(28.969658196228,537.553630041063,-48.3906526202095)) ;
#63089=CARTESIAN_POINT('Ctrl Pts',(28.775882258398,537.440133668493,-48.3797737830095)) ;
#63090=CARTESIAN_POINT('Ctrl Pts',(28.7045376370665,537.392094934182,-48.3755841735163)) ;
#63091=CARTESIAN_POINT('Ctrl Pts',(28.6364362059859,537.339756567338,-48.3712578505663)) ;
#63092=CARTESIAN_POINT('Ctrl Pts',(28.6364362890811,537.3397566312,-48.4293659750649)) ;
#63093=CARTESIAN_POINT('Ctrl Pts',(28.6369341345453,537.340139243068,-48.4293966207162)) ;
#63094=CARTESIAN_POINT('Ctrl Pts',(28.6374321589537,537.340521629481,-48.4294272625968)) ;
#63095=CARTESIAN_POINT('Ctrl Pts',(28.7800462888248,537.44991782317,-48.4381976533586)) ;
#63096=CARTESIAN_POINT('Ctrl Pts',(28.9357932715107,537.539874897829,-48.4466631603452)) ;
#63097=CARTESIAN_POINT('Ctrl Pts',(29.1493914937462,537.628479096233,-48.4586217370792)) ;
#63098=CARTESIAN_POINT('Ctrl Pts',(29.1982914004728,537.646615103932,-48.4613741865881)) ;
#63099=CARTESIAN_POINT('Ctrl Pts',(29.2985341710519,537.679512495968,-48.4670738079441)) ;
#63100=CARTESIAN_POINT('Ctrl Pts',(29.3498682754265,537.69417077506,-48.4700218739289)) ;
#63101=CARTESIAN_POINT('Ctrl Pts',(29.5197401231057,537.735596653561,-48.4798886385651)) ;
#63102=CARTESIAN_POINT('Ctrl Pts',(29.6400734380034,537.753851770086,-48.4870697365803)) ;
#63103=CARTESIAN_POINT('Ctrl Pts',(29.890948668675,537.769415700826,-48.5021575738849)) ;
#63104=CARTESIAN_POINT('Ctrl Pts',(30.0210758289075,537.765146895875,-48.5100450976257)) ;
#63105=CARTESIAN_POINT('Ctrl Pts',(30.1831069739731,537.744364345731,-48.5193697278809)) ;
#63106=CARTESIAN_POINT('Ctrl Pts',(30.2161734596322,537.739299894654,-48.5212449249387)) ;
#63107=CARTESIAN_POINT('Ctrl Pts',(30.2802337054626,537.727881144985,-48.5248041479331)) ;
#63108=CARTESIAN_POINT('Ctrl Pts',(30.3112326378434,537.721614154638,-48.5264915296209)) ;
#63109=CARTESIAN_POINT('Ctrl Pts',(30.4193712226151,537.697140916015,-48.5322929018191)) ;
#63110=CARTESIAN_POINT('Ctrl Pts',(30.4955972493127,537.675189013209,-48.5362308872873)) ;
#63111=CARTESIAN_POINT('Ctrl Pts',(30.7439778340765,537.587816240299,-48.549100545008)) ;
#63112=CARTESIAN_POINT('Ctrl Pts',(30.9085813624795,537.503706560625,-48.5577755381623)) ;
#63113=CARTESIAN_POINT('Ctrl Pts',(31.1024713760036,537.369190175353,-48.5699889667854)) ;
#63114=CARTESIAN_POINT('Ctrl Pts',(31.1440135884473,537.337971291506,-48.5727335794584)) ;
#63115=CARTESIAN_POINT('Ctrl Pts',(31.2259504847639,537.27139003543,-48.5784411871001)) ;
#63116=CARTESIAN_POINT('Ctrl Pts',(31.2662314798376,537.235952166069,-48.5814061958917)) ;
#63117=CARTESIAN_POINT('Ctrl Pts',(31.3537013792073,537.152705633824,-48.5882257457261)) ;
#63118=CARTESIAN_POINT('Ctrl Pts',(31.4000241652538,537.104078763425,-48.5921129488544)) ;
#63119=CARTESIAN_POINT('Ctrl Pts',(31.532130969245,536.951050407056,-48.6040313840824)) ;
#63120=CARTESIAN_POINT('Ctrl Pts',(31.610081524474,536.84038136237,-48.612267924402)) ;
#63121=CARTESIAN_POINT('Ctrl Pts',(31.7059545915688,536.671036217124,-48.6238002968767)) ;
#63122=CARTESIAN_POINT('Ctrl Pts',(31.7330344859247,536.617946572958,-48.6272746542249)) ;
#63123=CARTESIAN_POINT('Ctrl Pts',(31.770204887291,536.536510033042,-48.6323184695661)) ;
#63124=CARTESIAN_POINT('Ctrl Pts',(31.7820428516438,536.508997847162,-48.6339746771135)) ;
#63125=CARTESIAN_POINT('Ctrl Pts',(31.8070057707924,536.447300556583,-48.6375715962633)) ;
#63126=CARTESIAN_POINT('Ctrl Pts',(31.8198265633701,536.41300534071,-48.6394961948287)) ;
#63127=CARTESIAN_POINT('Ctrl Pts',(31.8465031839903,536.335382547397,-48.6437244550515)) ;
#63128=CARTESIAN_POINT('Ctrl Pts',(31.8598507509704,536.291900369335,-48.6460060016628)) ;
#63129=CARTESIAN_POINT('Ctrl Pts',(31.9030471562376,536.132501638755,-48.6541713204406)) ;
#63130=CARTESIAN_POINT('Ctrl Pts',(31.9241989758048,536.014478360057,-48.6598549254506)) ;
#63131=CARTESIAN_POINT('Ctrl Pts',(31.9430323379677,535.805828438005,-48.6701129849498)) ;
#63132=CARTESIAN_POINT('Ctrl Pts',(31.9452321466234,535.715949847246,-48.6745963046339)) ;
#63133=CARTESIAN_POINT('Ctrl Pts',(31.9394476928602,535.575151268958,-48.6819168956853)) ;
#63134=CARTESIAN_POINT('Ctrl Pts',(31.935444950985,535.524181471041,-48.6846271532407)) ;
#63135=CARTESIAN_POINT('Ctrl Pts',(31.9232023026646,535.41881509033,-48.6903801553537)) ;
#63136=CARTESIAN_POINT('Ctrl Pts',(31.9146700888374,535.364494303113,-48.6934303048282)) ;
#63137=CARTESIAN_POINT('Ctrl Pts',(31.8814923869037,535.197316851374,-48.7030933440012)) ;
#63138=CARTESIAN_POINT('Ctrl Pts',(31.8495080041542,535.08615953212,-48.7099277833718)) ;
#63139=CARTESIAN_POINT('Ctrl Pts',(31.7622215685892,534.857317338191,-48.7246294358381)) ;
#63140=CARTESIAN_POINT('Ctrl Pts',(31.7047468601355,534.74097130568,-48.7324896348168)) ;
#63141=CARTESIAN_POINT('Ctrl Pts',(31.619111806607,534.602324927815,-48.7417921002564)) ;
#63142=CARTESIAN_POINT('Ctrl Pts',(31.6008272848172,534.574278139409,-48.7436690093868)) ;
#63143=CARTESIAN_POINT('Ctrl Pts',(31.5639681048963,534.520651299094,-48.7472285686689)) ;
#63144=CARTESIAN_POINT('Ctrl Pts',(31.5454729735806,534.495029041029,-48.7489146878207)) ;
#63145=CARTESIAN_POINT('Ctrl Pts',(31.478769457113,534.406974371609,-48.7546952049357)) ;
#63146=CARTESIAN_POINT('Ctrl Pts',(31.4275605618832,534.346894424055,-48.7586153935346)) ;
#63147=CARTESIAN_POINT('Ctrl Pts',(31.2452598331507,534.156402940385,-48.7715048480354)) ;
#63148=CARTESIAN_POINT('Ctrl Pts',(31.100087052131,534.04075517695,-48.7802110641077)) ;
#63149=CARTESIAN_POINT('Ctrl Pts',(30.8968010888553,533.919453643736,-48.7924637012187)) ;
#63150=CARTESIAN_POINT('Ctrl Pts',(30.8512036997583,533.894539288516,-48.7952082236486)) ;
#63151=CARTESIAN_POINT('Ctrl Pts',(30.7566582376927,533.84744164903,-48.8009187729786)) ;
#63152=CARTESIAN_POINT('Ctrl Pts',(30.707686431377,533.825397247532,-48.8038869570241)) ;
#63153=CARTESIAN_POINT('Ctrl Pts',(30.5956643458089,533.780160627255,-48.8107102818242)) ;
#63154=CARTESIAN_POINT('Ctrl Pts',(30.5322287080541,533.758091959801,-48.8145979272861)) ;
#63155=CARTESIAN_POINT('Ctrl Pts',(30.3377825727375,533.70095309641,-48.8265458852118)) ;
#63156=CARTESIAN_POINT('Ctrl Pts',(30.2042809237263,533.675702165735,-48.8348129996362)) ;
#63157=CARTESIAN_POINT('Ctrl Pts',(30.0104620705288,533.658586862171,-48.8463374070203)) ;
#63158=CARTESIAN_POINT('Ctrl Pts',(29.9514522259461,533.655930259869,-48.8497788664516)) ;
#63159=CARTESIAN_POINT('Ctrl Pts',(29.862778450047,533.65576290418,-48.8547730708599)) ;
#63160=CARTESIAN_POINT('Ctrl Pts',(29.8331510395665,533.65634774999,-48.8564113135559)) ;
#63161=CARTESIAN_POINT('Ctrl Pts',(29.7669271382415,533.659089140959,-48.8599934643313)) ;
#63162=CARTESIAN_POINT('Ctrl Pts',(29.7303565076276,533.661584245061,-48.8619203514904)) ;
#63163=CARTESIAN_POINT('Ctrl Pts',(29.6485352682143,533.669370640701,-48.8661546058384)) ;
#63164=CARTESIAN_POINT('Ctrl Pts',(29.6033541592041,533.675191010724,-48.868439803436)) ;
#63165=CARTESIAN_POINT('Ctrl Pts',(29.4397931584769,533.701815382174,-48.8766340387472)) ;
#63166=CARTESIAN_POINT('Ctrl Pts',(29.3231049050991,533.731490330573,-48.8823421003453)) ;
#63167=CARTESIAN_POINT('Ctrl Pts',(29.1255303987832,533.800648702973,-48.8925983927261)) ;
#63168=CARTESIAN_POINT('Ctrl Pts',(29.0433982438944,533.83554521826,-48.8970516434834)) ;
#63169=CARTESIAN_POINT('Ctrl Pts',(28.9181967859105,533.898642697004,-48.9043377886449)) ;
#63170=CARTESIAN_POINT('Ctrl Pts',(28.8734731992443,533.923313404962,-48.9070463441136)) ;
#63171=CARTESIAN_POINT('Ctrl Pts',(28.782495903055,533.978015763905,-48.9128055638768)) ;
#63172=CARTESIAN_POINT('Ctrl Pts',(28.7364393900242,534.008294486009,-48.9158640837821)) ;
#63173=CARTESIAN_POINT('Ctrl Pts',(28.5968448723203,534.108329479567,-48.9256045307346)) ;
#63174=CARTESIAN_POINT('Ctrl Pts',(28.5080007968297,534.184215561842,-48.9325135703255)) ;
#63175=CARTESIAN_POINT('Ctrl Pts',(28.3363244911219,534.358163329451,-48.9471897982566)) ;
#63176=CARTESIAN_POINT('Ctrl Pts',(28.2552406649746,534.457288384783,-48.9549440754408)) ;
#63177=CARTESIAN_POINT('Ctrl Pts',(28.1651226857596,534.591189234342,-48.9641622118551)) ;
#63178=CARTESIAN_POINT('Ctrl Pts',(28.1470435395733,534.619528713667,-48.9660475985244)) ;
#63179=CARTESIAN_POINT('Ctrl Pts',(28.1134540115264,534.675145102815,-48.9696032458967)) ;
#63180=CARTESIAN_POINT('Ctrl Pts',(28.0978575945542,534.702357842372,-48.9712777588851)) ;
#63181=CARTESIAN_POINT('Ctrl Pts',(28.0464988262082,534.796923280355,-48.9769119178478)) ;
#63182=CARTESIAN_POINT('Ctrl Pts',(28.0138625654261,534.86590868834,-48.9807092093426)) ;
#63183=CARTESIAN_POINT('Ctrl Pts',(27.9295186082834,535.073321377053,-48.9916672182404)) ;
#63184=CARTESIAN_POINT('Ctrl Pts',(27.8888064204059,535.215679883322,-48.9986472242326)) ;
#63185=CARTESIAN_POINT('Ctrl Pts',(27.8527272342222,535.424769497181,-49.0093009088516)) ;
#63186=CARTESIAN_POINT('Ctrl Pts',(27.8447565767471,535.488841886332,-49.0126121056994)) ;
#63187=CARTESIAN_POINT('Ctrl Pts',(27.8360411363504,535.602292071308,-49.018621250477)) ;
#63188=CARTESIAN_POINT('Ctrl Pts',(27.8340357012717,535.651521140232,-49.0212764843941)) ;
#63189=CARTESIAN_POINT('Ctrl Pts',(27.8334920706155,535.765581350514,-49.0275576199013)) ;
#63190=CARTESIAN_POINT('Ctrl Pts',(27.8362496176875,535.830363180296,-49.0312223608911)) ;
#63191=CARTESIAN_POINT('Ctrl Pts',(27.8493044253744,535.975294799131,-49.0396387495613)) ;
#63192=CARTESIAN_POINT('Ctrl Pts',(27.8612762282024,536.055185266311,-49.0444303922878)) ;
#63193=CARTESIAN_POINT('Ctrl Pts',(27.9067613413416,536.27108303815,-49.0576690138394)) ;
#63194=CARTESIAN_POINT('Ctrl Pts',(27.9495207150067,536.404707790326,-49.0662027057441)) ;
#63195=CARTESIAN_POINT('Ctrl Pts',(28.0185405257698,536.562740188445,-49.0760279359963)) ;
#63196=CARTESIAN_POINT('Ctrl Pts',(28.032255570223,536.592216121502,-49.0778468905781)) ;
#63197=CARTESIAN_POINT('Ctrl Pts',(28.0611434151041,536.650635032118,-49.08140578559)) ;
#63198=CARTESIAN_POINT('Ctrl Pts',(28.0763185331564,536.679566137274,-49.0831452063993)) ;
#63199=CARTESIAN_POINT('Ctrl Pts',(28.1391848763923,536.792772324395,-49.089906784842)) ;
#63200=CARTESIAN_POINT('Ctrl Pts',(28.1921209509982,536.873999898044,-49.0946614201394)) ;
#63201=CARTESIAN_POINT('Ctrl Pts',(28.3293440963686,537.055167643582,-49.1057178054702)) ;
#63202=CARTESIAN_POINT('Ctrl Pts',(28.4178107731256,537.151398051176,-49.1119736958817)) ;
#63203=CARTESIAN_POINT('Ctrl Pts',(28.554053713274,537.273883161158,-49.1212418129166)) ;
#63204=CARTESIAN_POINT('Ctrl Pts',(28.5946501464557,537.307645068652,-49.1239612214735)) ;
#63205=CARTESIAN_POINT('Ctrl Pts',(28.636499183292,537.339804965697,-49.1267434461298)) ;
#63206=CARTESIAN_POINT('Origin',(29.8885276254155,585.710565160562,-51.0680854522906)) ;
#63207=CARTESIAN_POINT('Ctrl Pts',(27.8735990520585,585.307997890694,-48.9453612460011)) ;
#63208=CARTESIAN_POINT('Ctrl Pts',(27.8828319451009,585.261785440258,-48.9430764260291)) ;
#63209=CARTESIAN_POINT('Ctrl Pts',(27.8936579797779,585.215873972431,-48.940800625095)) ;
#63210=CARTESIAN_POINT('Ctrl Pts',(27.9347516972393,585.065070751935,-48.9332117860105)) ;
#63211=CARTESIAN_POINT('Ctrl Pts',(27.9717770230872,584.962255467665,-48.92784200937)) ;
#63212=CARTESIAN_POINT('Ctrl Pts',(28.0384706308186,584.814993064186,-48.9194872141135)) ;
#63213=CARTESIAN_POINT('Ctrl Pts',(28.0619826295612,584.767966110018,-48.9167139106165)) ;
#63214=CARTESIAN_POINT('Ctrl Pts',(28.1130495345266,584.674927375609,-48.9109820561371)) ;
#63215=CARTESIAN_POINT('Ctrl Pts',(28.140654051435,584.62898979262,-48.908023163243)) ;
#63216=CARTESIAN_POINT('Ctrl Pts',(28.25590551563,584.453151570968,-48.8961604357202)) ;
#63217=CARTESIAN_POINT('Ctrl Pts',(28.3564845074397,584.332387613501,-48.8867614008555)) ;
#63218=CARTESIAN_POINT('Ctrl Pts',(28.5404134475904,584.156821291141,-48.8714760146908)) ;
#63219=CARTESIAN_POINT('Ctrl Pts',(28.6157669081412,584.094515943848,-48.8656341455121)) ;
#63220=CARTESIAN_POINT('Ctrl Pts',(28.7218404423022,584.018848949306,-48.8582168333091)) ;
#63221=CARTESIAN_POINT('Ctrl Pts',(28.7488595555702,584.00053016038,-48.8563920678079)) ;
#63222=CARTESIAN_POINT('Ctrl Pts',(28.8038317937748,583.965141364442,-48.8528254229299)) ;
#63223=CARTESIAN_POINT('Ctrl Pts',(28.8317795338927,583.948080260942,-48.8510842726652)) ;
#63224=CARTESIAN_POINT('Ctrl Pts',(28.9805311904364,583.86208383587,-48.8421258450719)) ;
#63225=CARTESIAN_POINT('Ctrl Pts',(29.1077080427244,583.804870949162,-48.8354958606823)) ;
#63226=CARTESIAN_POINT('Ctrl Pts',(29.3164592093386,583.73539949144,-48.8248356009852)) ;
#63227=CARTESIAN_POINT('Ctrl Pts',(29.3946545399406,583.714411338987,-48.820891855375)) ;
#63228=CARTESIAN_POINT('Ctrl Pts',(29.5375992007793,583.68495925355,-48.8135627439636)) ;
#63229=CARTESIAN_POINT('Ctrl Pts',(29.6019008912608,583.67486526629,-48.810224167102)) ;
#63230=CARTESIAN_POINT('Ctrl Pts',(29.7161079886277,583.662455767892,-48.8041554036916)) ;
#63231=CARTESIAN_POINT('Ctrl Pts',(29.7658226386929,583.658877197722,-48.8014681105815)) ;
#63232=CARTESIAN_POINT('Ctrl Pts',(29.8818194143827,583.654758492743,-48.7950728714387)) ;
#63233=CARTESIAN_POINT('Ctrl Pts',(29.9480922703889,583.655610974656,-48.7913234000719)) ;
#63234=CARTESIAN_POINT('Ctrl Pts',(30.1613217624503,583.668677305342,-48.7789552567645)) ;
#63235=CARTESIAN_POINT('Ctrl Pts',(30.3070337244956,583.693496225898,-48.7699997001851)) ;
#63236=CARTESIAN_POINT('Ctrl Pts',(30.5201616922284,583.753900882992,-48.7567619853803)) ;
#63237=CARTESIAN_POINT('Ctrl Pts',(30.5903670728376,583.777971065631,-48.7523863572617)) ;
#63238=CARTESIAN_POINT('Ctrl Pts',(30.6881942252481,583.81754788722,-48.7464057891474)) ;
#63239=CARTESIAN_POINT('Ctrl Pts',(30.7169959342009,583.829974367012,-48.7446604082429)) ;
#63240=CARTESIAN_POINT('Ctrl Pts',(30.776733898433,583.857387403823,-48.7410894368781)) ;
#63241=CARTESIAN_POINT('Ctrl Pts',(30.8076006084095,583.872500052541,-48.7392710751644)) ;
#63242=CARTESIAN_POINT('Ctrl Pts',(30.9643078236209,583.95416085008,-48.7301062112254)) ;
#63243=CARTESIAN_POINT('Ctrl Pts',(31.08337668112,584.03288708128,-48.7233476818017)) ;
#63244=CARTESIAN_POINT('Ctrl Pts',(31.2793757498751,584.19401049874,-48.7110370886051)) ;
#63245=CARTESIAN_POINT('Ctrl Pts',(31.3594962772446,584.27159173016,-48.7055656014119)) ;
#63246=CARTESIAN_POINT('Ctrl Pts',(31.4676760674295,584.394866718269,-48.6970930090278)) ;
#63247=CARTESIAN_POINT('Ctrl Pts',(31.5008820584609,584.435777060235,-48.6943148732855)) ;
#63248=CARTESIAN_POINT('Ctrl Pts',(31.5645546291345,584.520695390366,-48.6885847556892)) ;
#63249=CARTESIAN_POINT('Ctrl Pts',(31.5949468372883,584.564707708841,-48.6856329809055)) ;
#63250=CARTESIAN_POINT('Ctrl Pts',(31.7082083532369,584.743242369691,-48.6737082586726)) ;
#63251=CARTESIAN_POINT('Ctrl Pts',(31.7771541839664,584.885928113124,-48.6642293704264)) ;
#63252=CARTESIAN_POINT('Ctrl Pts',(31.8608933388827,585.126491965216,-48.6489198893472)) ;
#63253=CARTESIAN_POINT('Ctrl Pts',(31.8862189720269,585.220054905014,-48.6431314359125)) ;
#63254=CARTESIAN_POINT('Ctrl Pts',(31.911132813277,585.347068647145,-48.6357643033073)) ;
#63255=CARTESIAN_POINT('Ctrl Pts',(31.9166485219174,585.379223371689,-48.633940884459)) ;
#63256=CARTESIAN_POINT('Ctrl Pts',(31.9261678452045,585.443929675183,-48.63037338205)) ;
#63257=CARTESIAN_POINT('Ctrl Pts',(31.930162588974,585.476473087068,-48.628630178473)) ;
#63258=CARTESIAN_POINT('Ctrl Pts',(31.9399954942879,585.576276100018,-48.6234023185067)) ;
#63259=CARTESIAN_POINT('Ctrl Pts',(31.9433001626235,585.643742882456,-48.6200309199534)) ;
#63260=CARTESIAN_POINT('Ctrl Pts',(31.9432268809865,585.862142072657,-48.6093098625096)) ;
#63261=CARTESIAN_POINT('Ctrl Pts',(31.9265570734146,586.012561161177,-48.6021883339017)) ;
#63262=CARTESIAN_POINT('Ctrl Pts',(31.8791982766796,586.223933774399,-48.5913218257441)) ;
#63263=CARTESIAN_POINT('Ctrl Pts',(31.8617617266439,586.287334633891,-48.5879525832714)) ;
#63264=CARTESIAN_POINT('Ctrl Pts',(31.8258196602408,586.397135777016,-48.5818536579686)) ;
#63265=CARTESIAN_POINT('Ctrl Pts',(31.8086049423566,586.443901463165,-48.5791688934032)) ;
#63266=CARTESIAN_POINT('Ctrl Pts',(31.7648496519996,586.55062944245,-48.5728179108504)) ;
#63267=CARTESIAN_POINT('Ctrl Pts',(31.7371060415975,586.610036573832,-48.5691122456167)) ;
#63268=CARTESIAN_POINT('Ctrl Pts',(31.6683752720788,586.740545806259,-48.5605811907351)) ;
#63269=CARTESIAN_POINT('Ctrl Pts',(31.625873047702,586.810722795197,-48.5557143506426)) ;
#63270=CARTESIAN_POINT('Ctrl Pts',(31.5019234464376,586.990210141892,-48.5426325634253)) ;
#63271=CARTESIAN_POINT('Ctrl Pts',(31.413602052318,587.0942881016,-48.5343477697469)) ;
#63272=CARTESIAN_POINT('Ctrl Pts',(31.2918750230757,587.211799269043,-48.5247059847297)) ;
#63273=CARTESIAN_POINT('Ctrl Pts',(31.2675689369299,587.234157335596,-48.5228579173838)) ;
#63274=CARTESIAN_POINT('Ctrl Pts',(31.2183674720407,587.277272892066,-48.5192856052886)) ;
#63275=CARTESIAN_POINT('Ctrl Pts',(31.1934990656334,587.298046468125,-48.5175605810797)) ;
#63276=CARTESIAN_POINT('Ctrl Pts',(31.0969248872281,587.37491495707,-48.5111173943664)) ;
#63277=CARTESIAN_POINT('Ctrl Pts',(31.0220055134937,587.426815492891,-48.5066362620309)) ;
#63278=CARTESIAN_POINT('Ctrl Pts',(30.8084278084011,587.5546651062,-48.4945322749571)) ;
#63279=CARTESIAN_POINT('Ctrl Pts',(30.6640884365156,587.619864514387,-48.4870182239858)) ;
#63280=CARTESIAN_POINT('Ctrl Pts',(30.461216012842,587.684662981642,-48.4761035926813)) ;
#63281=CARTESIAN_POINT('Ctrl Pts',(30.4080735160824,587.699309868848,-48.4732194884917)) ;
#63282=CARTESIAN_POINT('Ctrl Pts',(30.3041724313787,587.723497724343,-48.4674975042467)) ;
#63283=CARTESIAN_POINT('Ctrl Pts',(30.2535163502199,587.733296150955,-48.4646706110966)) ;
#63284=CARTESIAN_POINT('Ctrl Pts',(30.1109173362283,587.755348132967,-48.4565926048347)) ;
#63285=CARTESIAN_POINT('Ctrl Pts',(30.0184430545465,587.763298232305,-48.4512109170444)) ;
#63286=CARTESIAN_POINT('Ctrl Pts',(29.7881874387505,587.767470850485,-48.4375458956304)) ;
#63287=CARTESIAN_POINT('Ctrl Pts',(29.6507208797945,587.756139860824,-48.4291382587002)) ;
#63288=CARTESIAN_POINT('Ctrl Pts',(29.4673457254583,587.722279197781,-48.418199947024)) ;
#63289=CARTESIAN_POINT('Ctrl Pts',(29.419599086166,587.71168842582,-48.4153815054089)) ;
#63290=CARTESIAN_POINT('Ctrl Pts',(29.3439784790511,587.692059110938,-48.411013048576)) ;
#63291=CARTESIAN_POINT('Ctrl Pts',(29.3158444361789,587.684111794925,-48.4094108937611)) ;
#63292=CARTESIAN_POINT('Ctrl Pts',(29.2479414463373,587.66335584115,-48.4056037101182)) ;
#63293=CARTESIAN_POINT('Ctrl Pts',(29.2083769251862,587.649930420049,-48.4034312895463)) ;
#63294=CARTESIAN_POINT('Ctrl Pts',(29.0649387296169,587.596327198067,-48.3956329475004)) ;
#63295=CARTESIAN_POINT('Ctrl Pts',(28.9639642494161,587.548929494315,-48.3902876589681)) ;
#63296=CARTESIAN_POINT('Ctrl Pts',(28.7605616866109,587.432432512032,-48.3789415175016)) ;
#63297=CARTESIAN_POINT('Ctrl Pts',(28.6595147948651,587.361824738476,-48.3729455374816)) ;
#63298=CARTESIAN_POINT('Ctrl Pts',(28.5245997117867,587.248271804966,-48.3638584784995)) ;
#63299=CARTESIAN_POINT('Ctrl Pts',(28.4851572127738,587.212361374696,-48.3610527891648)) ;
#63300=CARTESIAN_POINT('Ctrl Pts',(28.4095418356387,587.137934913229,-48.3553365899688)) ;
#63301=CARTESIAN_POINT('Ctrl Pts',(28.3733689587353,587.099477274376,-48.3524296095634)) ;
#63302=CARTESIAN_POINT('Ctrl Pts',(28.2637347117484,586.973533130021,-48.3430345374575)) ;
#63303=CARTESIAN_POINT('Ctrl Pts',(28.1960723420737,586.881303856626,-48.3363197263494)) ;
#63304=CARTESIAN_POINT('Ctrl Pts',(28.0647700036677,586.666976164258,-48.3212673541831)) ;
#63305=CARTESIAN_POINT('Ctrl Pts',(28.0050033170084,586.543123266581,-48.3129077669416)) ;
#63306=CARTESIAN_POINT('Ctrl Pts',(27.9460310373271,586.381334024594,-48.303041472131)) ;
#63307=CARTESIAN_POINT('Ctrl Pts',(27.9348807829284,586.348129439641,-48.3010707738538)) ;
#63308=CARTESIAN_POINT('Ctrl Pts',(27.9154793199297,586.285053645666,-48.2974500155675)) ;
#63309=CARTESIAN_POINT('Ctrl Pts',(27.9070448732466,586.255251131039,-48.2957915775275)) ;
#63310=CARTESIAN_POINT('Ctrl Pts',(27.8819134032908,586.158122291074,-48.2905239125927)) ;
#63311=CARTESIAN_POINT('Ctrl Pts',(27.8679490942094,586.090133423294,-48.2870460380664)) ;
#63312=CARTESIAN_POINT('Ctrl Pts',(27.8347763925141,585.87348791356,-48.2762644177513)) ;
#63313=CARTESIAN_POINT('Ctrl Pts',(27.828363726723,585.723379597226,-48.2692008448875)) ;
#63314=CARTESIAN_POINT('Ctrl Pts',(27.8428558433911,585.505966301211,-48.2583071991447)) ;
#63315=CARTESIAN_POINT('Ctrl Pts',(27.8507581869572,585.438300178,-48.2548284056049)) ;
#63316=CARTESIAN_POINT('Ctrl Pts',(27.8655401484261,585.35004119791,-48.2501155276743)) ;
#63317=CARTESIAN_POINT('Ctrl Pts',(27.869405730716,585.328986290629,-48.2489781223699)) ;
#63318=CARTESIAN_POINT('Ctrl Pts',(27.8735990532433,585.307997884764,-48.2478302996211)) ;
#63319=CARTESIAN_POINT('Ctrl Pts',(27.8735990519255,585.30799789136,-48.3063633758768)) ;
#63320=CARTESIAN_POINT('Ctrl Pts',(27.8690228437001,585.330902716012,-48.3075791955719)) ;
#63321=CARTESIAN_POINT('Ctrl Pts',(27.8648370620205,585.353886230142,-48.3087777345022)) ;
#63322=CARTESIAN_POINT('Ctrl Pts',(27.8390652940413,585.510503910103,-48.3168292564892)) ;
#63323=CARTESIAN_POINT('Ctrl Pts',(27.8303373251784,585.645923443368,-48.3232401464756)) ;
#63324=CARTESIAN_POINT('Ctrl Pts',(27.8384534431231,585.881794760119,-48.3347322963557)) ;
#63325=CARTESIAN_POINT('Ctrl Pts',(27.8492967927589,585.981966326658,-48.3397132810064)) ;
#63326=CARTESIAN_POINT('Ctrl Pts',(27.8767835625487,586.131961236808,-48.3476078620855)) ;
#63327=CARTESIAN_POINT('Ctrl Pts',(27.8880629202371,586.182612978086,-48.3503494002897)) ;
#63328=CARTESIAN_POINT('Ctrl Pts',(27.9148999336193,586.284740695226,-48.3560593161279)) ;
#63329=CARTESIAN_POINT('Ctrl Pts',(27.9305853769514,586.336141047699,-48.3590301089257)) ;
#63330=CARTESIAN_POINT('Ctrl Pts',(28.0041461221571,586.547182336332,-48.3716558018206)) ;
#63331=CARTESIAN_POINT('Ctrl Pts',(28.0796746256448,586.699936179463,-48.3819088839737)) ;
#63332=CARTESIAN_POINT('Ctrl Pts',(28.2195680883585,586.912104584204,-48.3971489536296)) ;
#63333=CARTESIAN_POINT('Ctrl Pts',(28.2703364620774,586.979652496502,-48.4021628299502)) ;
#63334=CARTESIAN_POINT('Ctrl Pts',(28.3458498138865,587.068196646234,-48.4087753481411)) ;
#63335=CARTESIAN_POINT('Ctrl Pts',(28.367144985269,587.092018480801,-48.4105583281068)) ;
#63336=CARTESIAN_POINT('Ctrl Pts',(28.4115786577177,587.139449722224,-48.4140988523607)) ;
#63337=CARTESIAN_POINT('Ctrl Pts',(28.4347483876723,587.163016726596,-48.4158535092086)) ;
#63338=CARTESIAN_POINT('Ctrl Pts',(28.5152613527078,587.241052220625,-48.4216904835596)) ;
#63339=CARTESIAN_POINT('Ctrl Pts',(28.5751797018589,587.292769400038,-48.4256068227319)) ;
#63340=CARTESIAN_POINT('Ctrl Pts',(28.7800497785067,587.449919877474,-48.4382057697603)) ;
#63341=CARTESIAN_POINT('Ctrl Pts',(28.9357954566398,587.539875874447,-48.4466712248569)) ;
#63342=CARTESIAN_POINT('Ctrl Pts',(29.1493943090872,587.628480243647,-48.4586298525516)) ;
#63343=CARTESIAN_POINT('Ctrl Pts',(29.1982964077967,587.646616950942,-48.4613824294678)) ;
#63344=CARTESIAN_POINT('Ctrl Pts',(29.2985454382891,587.679515985023,-48.4670824176221)) ;
#63345=CARTESIAN_POINT('Ctrl Pts',(29.3498836496353,587.694175061945,-48.4700307273956)) ;
#63346=CARTESIAN_POINT('Ctrl Pts',(29.5197955539668,587.735608946595,-48.4798998520205)) ;
#63347=CARTESIAN_POINT('Ctrl Pts',(29.6401659782254,587.753865198461,-48.4870832547293)) ;
#63348=CARTESIAN_POINT('Ctrl Pts',(29.8910236896231,587.769412130909,-48.5021700893767)) ;
#63349=CARTESIAN_POINT('Ctrl Pts',(30.0210952415389,587.765142155608,-48.5100541145676)) ;
#63350=CARTESIAN_POINT('Ctrl Pts',(30.1830775202678,587.744368702829,-48.5193760254863)) ;
#63351=CARTESIAN_POINT('Ctrl Pts',(30.2161495560777,587.739303846438,-48.5212515552003)) ;
#63352=CARTESIAN_POINT('Ctrl Pts',(30.2802145057086,587.727884859259,-48.5248110660856)) ;
#63353=CARTESIAN_POINT('Ctrl Pts',(30.3112126400379,587.721618344097,-48.5264984170095)) ;
#63354=CARTESIAN_POINT('Ctrl Pts',(30.4193240139567,587.697152442163,-48.532298366769)) ;
#63355=CARTESIAN_POINT('Ctrl Pts',(30.4955244199026,587.675210415306,-48.5362350923644)) ;
#63356=CARTESIAN_POINT('Ctrl Pts',(30.7439283858594,587.587843422684,-48.5491059307094)) ;
#63357=CARTESIAN_POINT('Ctrl Pts',(30.908576037651,587.503714459816,-48.557782942845)) ;
#63358=CARTESIAN_POINT('Ctrl Pts',(31.1025033561642,587.369166800985,-48.5699989843105)) ;
#63359=CARTESIAN_POINT('Ctrl Pts',(31.1440457843143,587.337946485946,-48.5727436769571)) ;
#63360=CARTESIAN_POINT('Ctrl Pts',(31.2259880310742,587.271358123653,-48.5784518041368)) ;
#63361=CARTESIAN_POINT('Ctrl Pts',(31.266273824805,587.235914186997,-48.581417268506)) ;
#63362=CARTESIAN_POINT('Ctrl Pts',(31.3537467349999,587.152659559672,-48.5882373460527)) ;
#63363=CARTESIAN_POINT('Ctrl Pts',(31.4000681015528,587.104031113529,-48.5921246004308)) ;
#63364=CARTESIAN_POINT('Ctrl Pts',(31.5322058028293,586.950957186232,-48.6040463371314)) ;
#63365=CARTESIAN_POINT('Ctrl Pts',(31.6101800892929,586.84023768012,-48.6122863132611)) ;
#63366=CARTESIAN_POINT('Ctrl Pts',(31.7060343973457,586.670881816087,-48.6238181605086)) ;
#63367=CARTESIAN_POINT('Ctrl Pts',(31.7330857332409,586.617838816955,-48.6272891512746)) ;
#63368=CARTESIAN_POINT('Ctrl Pts',(31.7702293329091,586.536454196947,-48.6323295091933)) ;
#63369=CARTESIAN_POINT('Ctrl Pts',(31.7820649612693,586.508945264748,-48.6339854382212)) ;
#63370=CARTESIAN_POINT('Ctrl Pts',(31.8070315711429,586.447234262973,-48.6375829953204)) ;
#63371=CARTESIAN_POINT('Ctrl Pts',(31.8198573330843,586.412921674962,-48.6395084525387)) ;
#63372=CARTESIAN_POINT('Ctrl Pts',(31.8465466046069,586.335248895486,-48.6437391508926)) ;
#63373=CARTESIAN_POINT('Ctrl Pts',(31.8599006469411,586.291733757156,-48.6460222327522)) ;
#63374=CARTESIAN_POINT('Ctrl Pts',(31.9031482904717,586.132082169862,-48.6541998254054)) ;
#63375=CARTESIAN_POINT('Ctrl Pts',(31.9243086278689,586.013831499553,-48.6598936094312)) ;
#63376=CARTESIAN_POINT('Ctrl Pts',(31.9430560449183,585.805137605915,-48.6701546020348)) ;
#63377=CARTESIAN_POINT('Ctrl Pts',(31.9452252036312,585.715446883614,-48.6746292400956)) ;
#63378=CARTESIAN_POINT('Ctrl Pts',(31.9394273758999,585.574848092713,-48.6819400183033)) ;
#63379=CARTESIAN_POINT('Ctrl Pts',(31.9354181095184,585.523889967366,-48.6846498826931)) ;
#63380=CARTESIAN_POINT('Ctrl Pts',(31.9231581134606,585.418500244412,-48.6904046266792)) ;
#63381=CARTESIAN_POINT('Ctrl Pts',(31.9146113726914,585.364144952808,-48.6934570295856)) ;
#63382=CARTESIAN_POINT('Ctrl Pts',(31.8813274578258,585.196599033984,-48.7031425264944)) ;
#63383=CARTESIAN_POINT('Ctrl Pts',(31.8491976755306,585.085121853984,-48.7099987741587)) ;
#63384=CARTESIAN_POINT('Ctrl Pts',(31.7618473796161,584.856588605335,-48.7246853652262)) ;
#63385=CARTESIAN_POINT('Ctrl Pts',(31.7046165347513,584.740808679616,-48.7325066943848)) ;
#63386=CARTESIAN_POINT('Ctrl Pts',(31.6193039812691,584.602623578027,-48.7417782112384)) ;
#63387=CARTESIAN_POINT('Ctrl Pts',(31.6009968757251,584.574532278801,-48.743658131563)) ;
#63388=CARTESIAN_POINT('Ctrl Pts',(31.564135806747,584.520888379468,-48.7472188962191)) ;
#63389=CARTESIAN_POINT('Ctrl Pts',(31.5456647166443,584.495291354427,-48.7489033896821)) ;
#63390=CARTESIAN_POINT('Ctrl Pts',(31.4792960486314,584.407646868004,-48.7546569552136)) ;
#63391=CARTESIAN_POINT('Ctrl Pts',(31.4284408198576,584.347917075783,-48.7585541613219)) ;
#63392=CARTESIAN_POINT('Ctrl Pts',(31.2461032371271,584.157044787966,-48.7714616286157)) ;
#63393=CARTESIAN_POINT('Ctrl Pts',(31.1003368320949,584.040848178069,-48.7802013217019)) ;
#63394=CARTESIAN_POINT('Ctrl Pts',(30.8963609148751,583.91920677185,-48.792495130875)) ;
#63395=CARTESIAN_POINT('Ctrl Pts',(30.8507831878443,583.894317270325,-48.795238442322)) ;
#63396=CARTESIAN_POINT('Ctrl Pts',(30.7562128637324,583.847232878694,-48.8009504752684)) ;
#63397=CARTESIAN_POINT('Ctrl Pts',(30.7071940154448,583.825182060003,-48.8039215382368)) ;
#63398=CARTESIAN_POINT('Ctrl Pts',(30.5951231463654,583.779962696501,-48.8107479231404)) ;
#63399=CARTESIAN_POINT('Ctrl Pts',(30.5316876920127,583.757913907858,-48.8146356004414)) ;
#63400=CARTESIAN_POINT('Ctrl Pts',(30.3368011223745,583.700703582632,-48.8266105337954)) ;
#63401=CARTESIAN_POINT('Ctrl Pts',(30.2028394406781,583.675449026812,-48.8349061745544)) ;
#63402=CARTESIAN_POINT('Ctrl Pts',(30.0096246377573,583.658567824103,-48.8463896495128)) ;
#63403=CARTESIAN_POINT('Ctrl Pts',(29.9516866572799,583.655967981502,-48.8497677902681)) ;
#63404=CARTESIAN_POINT('Ctrl Pts',(29.8636999550514,583.655745975151,-48.8547258247118)) ;
#63405=CARTESIAN_POINT('Ctrl Pts',(29.8336871087152,583.656327775443,-48.8563859616068)) ;
#63406=CARTESIAN_POINT('Ctrl Pts',(29.7671110994842,583.659078834743,-48.8599873619322)) ;
#63407=CARTESIAN_POINT('Ctrl Pts',(29.7305731984307,583.661568119779,-48.8619126603701)) ;
#63408=CARTESIAN_POINT('Ctrl Pts',(29.6488461600364,583.669335506126,-48.8661423306649)) ;
#63409=CARTESIAN_POINT('Ctrl Pts',(29.6037261636613,583.675140322987,-48.8684246141494)) ;
#63410=CARTESIAN_POINT('Ctrl Pts',(29.4406495549682,583.701650174253,-48.8765949855997)) ;
#63411=CARTESIAN_POINT('Ctrl Pts',(29.3243685952474,583.731156027315,-48.8822831449036)) ;
#63412=CARTESIAN_POINT('Ctrl Pts',(29.126784185655,583.800130410762,-48.8925342947638)) ;
#63413=CARTESIAN_POINT('Ctrl Pts',(29.0442790184281,583.835130255024,-48.897005152448)) ;
#63414=CARTESIAN_POINT('Ctrl Pts',(28.9186937752864,583.898375876284,-48.9043114003962)) ;
#63415=CARTESIAN_POINT('Ctrl Pts',(28.8739400100024,583.923047596241,-48.907020956715)) ;
#63416=CARTESIAN_POINT('Ctrl Pts',(28.7829843422024,583.977706208729,-48.9127771452116)) ;
#63417=CARTESIAN_POINT('Ctrl Pts',(28.7369756716019,584.007933853613,-48.915831396764)) ;
#63418=CARTESIAN_POINT('Ctrl Pts',(28.5979521401743,584.107486581062,-48.9255279598643)) ;
#63419=CARTESIAN_POINT('Ctrl Pts',(28.5095622067334,584.182856292733,-48.9323942184793)) ;
#63420=CARTESIAN_POINT('Ctrl Pts',(28.337296920253,584.356935707098,-48.9470991196433)) ;
#63421=CARTESIAN_POINT('Ctrl Pts',(28.2554111077127,584.456944982158,-48.9549286022389)) ;
#63422=CARTESIAN_POINT('Ctrl Pts',(28.1647351501012,584.591788832908,-48.9642070074243)) ;
#63423=CARTESIAN_POINT('Ctrl Pts',(28.1467139496469,584.620057762267,-48.9660868586587)) ;
#63424=CARTESIAN_POINT('Ctrl Pts',(28.1131460555267,584.675670902665,-48.9696409850396)) ;
#63425=CARTESIAN_POINT('Ctrl Pts',(28.0975200670127,584.70295516496,-48.971319153325)) ;
#63426=CARTESIAN_POINT('Ctrl Pts',(28.0456916234135,584.798469928606,-48.9770072326492)) ;
#63427=CARTESIAN_POINT('Ctrl Pts',(28.0127105198681,584.868380767047,-48.9808502668949)) ;
#63428=CARTESIAN_POINT('Ctrl Pts',(27.9355998469476,585.058990289846,-48.9909079132612)) ;
#63429=CARTESIAN_POINT('Ctrl Pts',(27.8987327219357,585.182198904562,-48.9969997855251)) ;
#63430=CARTESIAN_POINT('Ctrl Pts',(27.873599044712,585.307997927464,-49.0033678610064)) ;
#63431=CARTESIAN_POINT('Origin',(179.888527625416,585.710565160536,-51.0680854522974)) ;
#63432=CARTESIAN_POINT('Ctrl Pts',(178.636459914524,587.339774787883,-49.0681958067691)) ;
#63433=CARTESIAN_POINT('Ctrl Pts',(178.522689824047,587.252341068882,-49.0609089955289)) ;
#63434=CARTESIAN_POINT('Ctrl Pts',(178.418390122109,587.153232145152,-49.0541378047761)) ;
#63435=CARTESIAN_POINT('Ctrl Pts',(178.263316915004,586.971436619688,-49.0424708890543)) ;
#63436=CARTESIAN_POINT('Ctrl Pts',(178.206516730537,586.894602127817,-49.0377266465304)) ;
#63437=CARTESIAN_POINT('Ctrl Pts',(178.127449532883,586.77041603943,-49.0300912475289)) ;
#63438=CARTESIAN_POINT('Ctrl Pts',(178.101297597512,586.725694763998,-49.0273491424362)) ;
#63439=CARTESIAN_POINT('Ctrl Pts',(178.051005767729,586.631713724577,-49.021575057535)) ;
#63440=CARTESIAN_POINT('Ctrl Pts',(178.027092924293,586.58238010058,-49.0185377642252)) ;
#63441=CARTESIAN_POINT('Ctrl Pts',(177.940642160745,586.384206873234,-49.0062942105506)) ;
#63442=CARTESIAN_POINT('Ctrl Pts',(177.893768281776,586.229189329091,-48.9965660400011)) ;
#63443=CARTESIAN_POINT('Ctrl Pts',(177.854678192988,586.0093725406,-48.9831611277426)) ;
#63444=CARTESIAN_POINT('Ctrl Pts',(177.846599334791,585.947965532311,-48.9794652477825)) ;
#63445=CARTESIAN_POINT('Ctrl Pts',(177.837487294457,585.841805777013,-48.9732488868553)) ;
#63446=CARTESIAN_POINT('Ctrl Pts',(177.835119794265,585.797210488457,-48.9706899204887)) ;
#63447=CARTESIAN_POINT('Ctrl Pts',(177.833611346328,585.723437875262,-48.9665810771249)) ;
#63448=CARTESIAN_POINT('Ctrl Pts',(177.833635366424,585.694297698019,-48.9649921358541)) ;
#63449=CARTESIAN_POINT('Ctrl Pts',(177.835281913436,585.619799203005,-48.9610139143282)) ;
#63450=CARTESIAN_POINT('Ctrl Pts',(177.837786954949,585.574478011413,-48.9586687963965)) ;
#63451=CARTESIAN_POINT('Ctrl Pts',(177.853814028621,585.3935360709,-48.9494781205464)) ;
#63452=CARTESIAN_POINT('Ctrl Pts',(177.879310822462,585.25932244537,-48.9430298320477)) ;
#63453=CARTESIAN_POINT('Ctrl Pts',(177.945645425027,585.034698538346,-48.9316092583279)) ;
#63454=CARTESIAN_POINT('Ctrl Pts',(177.980056095126,584.942892878263,-48.9267512485983)) ;
#63455=CARTESIAN_POINT('Ctrl Pts',(178.042531888474,584.806687457151,-48.9189858219906)) ;
#63456=CARTESIAN_POINT('Ctrl Pts',(178.065966781665,584.760319675901,-48.916238143136)) ;
#63457=CARTESIAN_POINT('Ctrl Pts',(178.117532437603,584.667233005862,-48.9104776963002)) ;
#63458=CARTESIAN_POINT('Ctrl Pts',(178.145816310086,584.620646628206,-48.9074607853636)) ;
#63459=CARTESIAN_POINT('Ctrl Pts',(178.266774481441,584.438183718587,-48.8950746231816)) ;
#63460=CARTESIAN_POINT('Ctrl Pts',(178.373746595138,584.31254505927,-48.8851563924031)) ;
#63461=CARTESIAN_POINT('Ctrl Pts',(178.558831940002,584.141625852043,-48.8700354875747)) ;
#63462=CARTESIAN_POINT('Ctrl Pts',(178.626881298135,584.086400061102,-48.8648260157736)) ;
#63463=CARTESIAN_POINT('Ctrl Pts',(178.724517861708,584.017013502868,-48.8580161973399)) ;
#63464=CARTESIAN_POINT('Ctrl Pts',(178.751222167727,583.998965739427,-48.8562168865875)) ;
#63465=CARTESIAN_POINT('Ctrl Pts',(178.80627834916,583.963614600199,-48.8526517590939)) ;
#63466=CARTESIAN_POINT('Ctrl Pts',(178.834647057342,583.946355482336,-48.8508885711469)) ;
#63467=CARTESIAN_POINT('Ctrl Pts',(178.979752297396,583.862825547564,-48.8421723516118)) ;
#63468=CARTESIAN_POINT('Ctrl Pts',(179.102376273154,583.807412948333,-48.8357574399702)) ;
#63469=CARTESIAN_POINT('Ctrl Pts',(179.344054085458,583.725580796474,-48.823399720558)) ;
#63470=CARTESIAN_POINT('Ctrl Pts',(179.461759004591,583.696991396647,-48.8174947155024)) ;
#63471=CARTESIAN_POINT('Ctrl Pts',(179.633719296693,583.670986157263,-48.8085216136563)) ;
#63472=CARTESIAN_POINT('Ctrl Pts',(179.686437232935,583.665090012014,-48.8057280772725)) ;
#63473=CARTESIAN_POINT('Ctrl Pts',(179.792320510631,583.657380911096,-48.8000024926176)) ;
#63474=CARTESIAN_POINT('Ctrl Pts',(179.845445508399,583.655579867296,-48.7970723574146)) ;
#63475=CARTESIAN_POINT('Ctrl Pts',(180.060926335081,583.656633792174,-48.7849335265143)) ;
#63476=CARTESIAN_POINT('Ctrl Pts',(180.222587067262,583.676666557783,-48.7751812275339)) ;
#63477=CARTESIAN_POINT('Ctrl Pts',(180.471670050796,583.738048384186,-48.7597680186341)) ;
#63478=CARTESIAN_POINT('Ctrl Pts',(180.561514710261,583.766865389574,-48.7541406330392)) ;
#63479=CARTESIAN_POINT('Ctrl Pts',(180.679291883315,583.81379215604,-48.7469266060518)) ;
#63480=CARTESIAN_POINT('Ctrl Pts',(180.709226004425,583.826550719338,-48.7451084662837)) ;
#63481=CARTESIAN_POINT('Ctrl Pts',(180.768790643142,583.853627757196,-48.7415404569656)) ;
#63482=CARTESIAN_POINT('Ctrl Pts',(180.798405516458,583.867957768318,-48.7397918942574)) ;
#63483=CARTESIAN_POINT('Ctrl Pts',(180.964286668989,583.953199439178,-48.7300732103009)) ;
#63484=CARTESIAN_POINT('Ctrl Pts',(181.092620945734,584.038511801579,-48.722820078209)) ;
#63485=CARTESIAN_POINT('Ctrl Pts',(181.266798320066,584.184845340799,-48.7117627085179)) ;
#63486=CARTESIAN_POINT('Ctrl Pts',(181.320735472359,584.235359807794,-48.7081372771924)) ;
#63487=CARTESIAN_POINT('Ctrl Pts',(181.414609481846,584.333287916784,-48.7012880526855)) ;
#63488=CARTESIAN_POINT('Ctrl Pts',(181.455346038366,584.379814425805,-48.6980991100151)) ;
#63489=CARTESIAN_POINT('Ctrl Pts',(181.525108527616,584.467143560612,-48.6921715423448)) ;
#63490=CARTESIAN_POINT('Ctrl Pts',(181.554858950221,584.507305576374,-48.6894660025777)) ;
#63491=CARTESIAN_POINT('Ctrl Pts',(181.623006311283,584.606682601377,-48.6828008938031)) ;
#63492=CARTESIAN_POINT('Ctrl Pts',(181.65987240215,584.666865477177,-48.6787869761349)) ;
#63493=CARTESIAN_POINT('Ctrl Pts',(181.763135641178,584.856725704305,-48.6662039900775)) ;
#63494=CARTESIAN_POINT('Ctrl Pts',(181.81890660503,584.99165820294,-48.6573377394081)) ;
#63495=CARTESIAN_POINT('Ctrl Pts',(181.87928210976,585.197145618763,-48.6445728069065)) ;
#63496=CARTESIAN_POINT('Ctrl Pts',(181.895313275056,585.263893045385,-48.6405415153138)) ;
#63497=CARTESIAN_POINT('Ctrl Pts',(181.913680446364,585.361697291086,-48.6349124431078)) ;
#63498=CARTESIAN_POINT('Ctrl Pts',(181.91869925795,585.392200109153,-48.6331958475187)) ;
#63499=CARTESIAN_POINT('Ctrl Pts',(181.92795281846,585.457624697237,-48.6296123162934)) ;
#63500=CARTESIAN_POINT('Ctrl Pts',(181.931982999312,585.4925641147,-48.6277555916354)) ;
#63501=CARTESIAN_POINT('Ctrl Pts',(181.947236975738,585.663182508792,-48.6188920450278)) ;
#63502=CARTESIAN_POINT('Ctrl Pts',(181.945855938037,585.799656253923,-48.6124091025634)) ;
#63503=CARTESIAN_POINT('Ctrl Pts',(181.922326698606,586.013781540776,-48.6019658601517)) ;
#63504=CARTESIAN_POINT('Ctrl Pts',(181.909119525765,586.091991740365,-48.598096296473)) ;
#63505=CARTESIAN_POINT('Ctrl Pts',(181.877070329413,586.23194127789,-48.5908781356076)) ;
#63506=CARTESIAN_POINT('Ctrl Pts',(181.859776295897,586.293928463719,-48.5875734407832)) ;
#63507=CARTESIAN_POINT('Ctrl Pts',(181.823970948016,586.40233213641,-48.5815375256033)) ;
#63508=CARTESIAN_POINT('Ctrl Pts',(181.806620827009,586.449077359126,-48.5788469790017)) ;
#63509=CARTESIAN_POINT('Ctrl Pts',(181.761973727089,586.557145164089,-48.5723991884735)) ;
#63510=CARTESIAN_POINT('Ctrl Pts',(181.733339478999,586.617849994804,-48.5685979421081)) ;
#63511=CARTESIAN_POINT('Ctrl Pts',(181.632601722606,586.806849982821,-48.556183876341)) ;
#63512=CARTESIAN_POINT('Ctrl Pts',(181.549677715302,586.928845632812,-48.547241692017)) ;
#63513=CARTESIAN_POINT('Ctrl Pts',(181.407207624141,587.09654285752,-48.5340987047981)) ;
#63514=CARTESIAN_POINT('Ctrl Pts',(181.357024989695,587.149606648158,-48.5297961754443)) ;
#63515=CARTESIAN_POINT('Ctrl Pts',(181.281454639671,587.221435715396,-48.5238896250166)) ;
#63516=CARTESIAN_POINT('Ctrl Pts',(181.258296910142,587.242462029363,-48.5221498622642)) ;
#63517=CARTESIAN_POINT('Ctrl Pts',(181.208581063148,587.28557262162,-48.5185759543543)) ;
#63518=CARTESIAN_POINT('Ctrl Pts',(181.181928866263,587.307532011327,-48.5167496317691)) ;
#63519=CARTESIAN_POINT('Ctrl Pts',(181.043599643916,587.415768600393,-48.5076442549347)) ;
#63520=CARTESIAN_POINT('Ctrl Pts',(180.923790899984,587.491056305203,-48.5009400328627)) ;
#63521=CARTESIAN_POINT('Ctrl Pts',(180.698526771038,587.602125994094,-48.4887557721398)) ;
#63522=CARTESIAN_POINT('Ctrl Pts',(180.596112403444,587.642771595279,-48.4833537154891)) ;
#63523=CARTESIAN_POINT('Ctrl Pts',(180.440126484713,587.690605967853,-48.474939652445)) ;
#63524=CARTESIAN_POINT('Ctrl Pts',(180.388726357869,587.704210926344,-48.4721408598607)) ;
#63525=CARTESIAN_POINT('Ctrl Pts',(180.285120463092,587.727375122811,-48.4664174503528)) ;
#63526=CARTESIAN_POINT('Ctrl Pts',(180.23295699744,587.736935306598,-48.46349535866)) ;
#63527=CARTESIAN_POINT('Ctrl Pts',(180.0613123979,587.761574140313,-48.4537313138675)) ;
#63528=CARTESIAN_POINT('Ctrl Pts',(179.940882315252,587.76817161978,-48.4466303077961)) ;
#63529=CARTESIAN_POINT('Ctrl Pts',(179.685650283496,587.75972720534,-48.4313129222973)) ;
#63530=CARTESIAN_POINT('Ctrl Pts',(179.551480027487,587.741975269937,-48.4231018376695)) ;
#63531=CARTESIAN_POINT('Ctrl Pts',(179.38776014391,587.703634904507,-48.4135168793249)) ;
#63532=CARTESIAN_POINT('Ctrl Pts',(179.355689312904,587.695301590795,-48.4116621103499)) ;
#63533=CARTESIAN_POINT('Ctrl Pts',(179.292788168715,587.677322521817,-48.4080889064942)) ;
#63534=CARTESIAN_POINT('Ctrl Pts',(179.26195620651,587.667718319085,-48.4063692453072)) ;
#63535=CARTESIAN_POINT('Ctrl Pts',(179.147243409052,587.628996148952,-48.4000473936535)) ;
#63536=CARTESIAN_POINT('Ctrl Pts',(179.065045314335,587.595176417414,-48.3956700578852)) ;
#63537=CARTESIAN_POINT('Ctrl Pts',(178.862019777161,587.495813986433,-48.3846717806871)) ;
#63538=CARTESIAN_POINT('Ctrl Pts',(178.745170702555,587.423320370498,-48.3781399215745)) ;
#63539=CARTESIAN_POINT('Ctrl Pts',(178.636459914529,587.339774787887,-48.3712343220044)) ;
#63540=CARTESIAN_POINT('Ctrl Pts',(178.636459914542,587.339774787898,-48.4293959864656)) ;
#63541=CARTESIAN_POINT('Ctrl Pts',(178.636986385796,587.340179387555,-48.4294283938969)) ;
#63542=CARTESIAN_POINT('Ctrl Pts',(178.637513057153,587.340583735086,-48.4294607971127)) ;
#63543=CARTESIAN_POINT('Ctrl Pts',(178.780119962262,587.449959164934,-48.4382301728603)) ;
#63544=CARTESIAN_POINT('Ctrl Pts',(178.9358216619,587.539884349372,-48.4466934278485)) ;
#63545=CARTESIAN_POINT('Ctrl Pts',(179.149377938323,587.628474150212,-48.4586496940449)) ;
#63546=CARTESIAN_POINT('Ctrl Pts',(179.198287363263,587.646613939987,-48.4614026870224)) ;
#63547=CARTESIAN_POINT('Ctrl Pts',(179.298552188786,587.6795182441,-48.4671035874245)) ;
#63548=CARTESIAN_POINT('Ctrl Pts',(179.349898874392,587.694179430637,-48.4700523947607)) ;
#63549=CARTESIAN_POINT('Ctrl Pts',(179.519877132353,587.735627344895,-48.4799254234614)) ;
#63550=CARTESIAN_POINT('Ctrl Pts',(179.640307299081,587.753885882769,-48.4871125309897)) ;
#63551=CARTESIAN_POINT('Ctrl Pts',(179.891138871261,587.769406518002,-48.5021978670502)) ;
#63552=CARTESIAN_POINT('Ctrl Pts',(180.021122982765,587.765134883684,-48.5100763857469)) ;
#63553=CARTESIAN_POINT('Ctrl Pts',(180.183029478466,587.744375820552,-48.5193940738666)) ;
#63554=CARTESIAN_POINT('Ctrl Pts',(180.216111276431,587.739310188868,-48.5212701829362)) ;
#63555=CARTESIAN_POINT('Ctrl Pts',(180.280186931822,587.727890227682,-48.5248303227102)) ;
#63556=CARTESIAN_POINT('Ctrl Pts',(180.311186074878,587.721623942164,-48.5265177421839)) ;
#63557=CARTESIAN_POINT('Ctrl Pts',(180.419277045108,587.697164106773,-48.5323166307148)) ;
#63558=CARTESIAN_POINT('Ctrl Pts',(180.495456715961,587.675230437209,-48.536252332983)) ;
#63559=CARTESIAN_POINT('Ctrl Pts',(180.743893023261,587.587864663703,-48.5491247834839)) ;
#63560=CARTESIAN_POINT('Ctrl Pts',(180.908588464011,587.503712761536,-48.5578040218231)) ;
#63561=CARTESIAN_POINT('Ctrl Pts',(181.102559876962,587.36912563149,-48.5700232054645)) ;
#63562=CARTESIAN_POINT('Ctrl Pts',(181.144106331474,587.337899977141,-48.5727682676786)) ;
#63563=CARTESIAN_POINT('Ctrl Pts',(181.22606380259,587.271293763494,-48.5784777140493)) ;
#63564=CARTESIAN_POINT('Ctrl Pts',(181.26636025404,587.235836702338,-48.5814441526807)) ;
#63565=CARTESIAN_POINT('Ctrl Pts',(181.353841079801,587.15256377485,-48.5882654064029)) ;
#63566=CARTESIAN_POINT('Ctrl Pts',(181.400160421775,587.103931045937,-48.5921528202506)) ;
#63567=CARTESIAN_POINT('Ctrl Pts',(181.532362375625,586.95076192346,-48.6040813560957)) ;
#63568=CARTESIAN_POINT('Ctrl Pts',(181.610385325454,586.839938278577,-48.6123283390582)) ;
#63569=CARTESIAN_POINT('Ctrl Pts',(181.706197873556,586.670565058768,-48.6238586293729)) ;
#63570=CARTESIAN_POINT('Ctrl Pts',(181.733187936688,586.617623274548,-48.6273223138455)) ;
#63571=CARTESIAN_POINT('Ctrl Pts',(181.770274577796,586.536350819265,-48.6323551986297)) ;
#63572=CARTESIAN_POINT('Ctrl Pts',(181.782105644378,586.508848474542,-48.6340105513203)) ;
#63573=CARTESIAN_POINT('Ctrl Pts',(181.807080991506,586.447107481161,-48.6376094994863)) ;
#63574=CARTESIAN_POINT('Ctrl Pts',(181.819917790566,586.412757439296,-48.6395367988921)) ;
#63575=CARTESIAN_POINT('Ctrl Pts',(181.846635156415,586.334976552407,-48.6437727439833)) ;
#63576=CARTESIAN_POINT('Ctrl Pts',(181.860003628662,586.291390001165,-48.646059132509)) ;
#63577=CARTESIAN_POINT('Ctrl Pts',(181.903363414394,586.131191237845,-48.6542631907058)) ;
#63578=CARTESIAN_POINT('Ctrl Pts',(181.924542793204,586.012448485831,-48.6599789005873)) ;
#63579=CARTESIAN_POINT('Ctrl Pts',(181.943107302616,585.803643157367,-48.6702468529653)) ;
#63580=CARTESIAN_POINT('Ctrl Pts',(181.945210561466,585.71434246134,-48.6747034291552)) ;
#63581=CARTESIAN_POINT('Ctrl Pts',(181.939380969133,585.574156434677,-48.6819939094418)) ;
#63582=CARTESIAN_POINT('Ctrl Pts',(181.935356419543,585.523220455332,-48.6847030665649)) ;
#63583=CARTESIAN_POINT('Ctrl Pts',(181.923056094147,585.417775264734,-48.6904618170837)) ;
#63584=CARTESIAN_POINT('Ctrl Pts',(181.914476361646,585.363343471826,-48.6935191872863)) ;
#63585=CARTESIAN_POINT('Ctrl Pts',(181.880953857306,585.194979441117,-48.7032544617348)) ;
#63586=CARTESIAN_POINT('Ctrl Pts',(181.848498568229,585.082792307793,-48.7101590874652)) ;
#63587=CARTESIAN_POINT('Ctrl Pts',(181.761008228129,584.854955107566,-48.7248112828564)) ;
#63588=CARTESIAN_POINT('Ctrl Pts',(181.704323616753,584.74044106589,-48.7325455574979)) ;
#63589=CARTESIAN_POINT('Ctrl Pts',(181.619732999493,584.603290776368,-48.7417474150512)) ;
#63590=CARTESIAN_POINT('Ctrl Pts',(181.601376933468,584.575102190356,-48.7436338706688)) ;
#63591=CARTESIAN_POINT('Ctrl Pts',(181.564510817635,584.521418669305,-48.7471973382189)) ;
#63592=CARTESIAN_POINT('Ctrl Pts',(181.546090854515,584.49587453644,-48.7488783845597)) ;
#63593=CARTESIAN_POINT('Ctrl Pts',(181.480410139887,584.409068774605,-48.7545766846394)) ;
#63594=CARTESIAN_POINT('Ctrl Pts',(181.430278388951,584.350054412464,-48.7584267985489)) ;
#63595=CARTESIAN_POINT('Ctrl Pts',(181.27490476644,584.186800623008,-48.7694526822597)) ;
#63596=CARTESIAN_POINT('Ctrl Pts',(181.161596854038,584.090937153969,-48.7764545529917)) ;
#63597=CARTESIAN_POINT('Ctrl Pts',(180.985874239071,583.972193801001,-48.7871167467605)) ;
#63598=CARTESIAN_POINT('Ctrl Pts',(180.931129520611,583.938818904161,-48.7904089452608)) ;
#63599=CARTESIAN_POINT('Ctrl Pts',(180.831445558496,583.884268596496,-48.7964156207729)) ;
#63600=CARTESIAN_POINT('Ctrl Pts',(180.787129616573,583.862061107398,-48.7990895235555)) ;
#63601=CARTESIAN_POINT('Ctrl Pts',(180.681710573235,583.813920899863,-48.8054772419058)) ;
#63602=CARTESIAN_POINT('Ctrl Pts',(180.62007072229,583.789304654493,-48.8092334701202)) ;
#63603=CARTESIAN_POINT('Ctrl Pts',(180.4778445923,583.740343394327,-48.8179444675618)) ;
#63604=CARTESIAN_POINT('Ctrl Pts',(180.396736848833,583.717881101102,-48.8229444977197)) ;
#63605=CARTESIAN_POINT('Ctrl Pts',(180.187165467769,583.67347121718,-48.8357998319232)) ;
#63606=CARTESIAN_POINT('Ctrl Pts',(180.057562166302,583.658647193278,-48.8437012290412)) ;
#63607=CARTESIAN_POINT('Ctrl Pts',(179.89399027169,583.655550361919,-48.8530372674224)) ;
#63608=CARTESIAN_POINT('Ctrl Pts',(179.860545511911,583.655733547046,-48.8549116000563)) ;
#63609=CARTESIAN_POINT('Ctrl Pts',(179.795417971214,583.657680861198,-48.8584746829691)) ;
#63610=CARTESIAN_POINT('Ctrl Pts',(179.763742952266,583.659362514779,-48.8601665525464)) ;
#63611=CARTESIAN_POINT('Ctrl Pts',(179.651856244361,583.66790420828,-48.8660362043115)) ;
#63612=CARTESIAN_POINT('Ctrl Pts',(179.572015914379,583.678743371446,-48.8700320578551)) ;
#63613=CARTESIAN_POINT('Ctrl Pts',(179.314517779207,583.72925344417,-48.8828505384156)) ;
#63614=CARTESIAN_POINT('Ctrl Pts',(179.141477145102,583.787807317399,-48.8914351977625)) ;
#63615=CARTESIAN_POINT('Ctrl Pts',(178.931781998375,583.891406220177,-48.9035367927947)) ;
#63616=CARTESIAN_POINT('Ctrl Pts',(178.886056600082,583.916198242564,-48.9062831764253)) ;
#63617=CARTESIAN_POINT('Ctrl Pts',(178.79529151434,583.969963319822,-48.9119847847951)) ;
#63618=CARTESIAN_POINT('Ctrl Pts',(178.750345892354,583.99901570397,-48.9149415781133)) ;
#63619=CARTESIAN_POINT('Ctrl Pts',(178.651772409613,584.068333547866,-48.9217452744036)) ;
#63620=CARTESIAN_POINT('Ctrl Pts',(178.59888008603,584.109535480401,-48.9256249255071)) ;
#63621=CARTESIAN_POINT('Ctrl Pts',(178.447004424898,584.240259080228,-48.9374369453836)) ;
#63622=CARTESIAN_POINT('Ctrl Pts',(178.354630428038,584.336903872117,-48.9455694340703)) ;
#63623=CARTESIAN_POINT('Ctrl Pts',(178.234368692083,584.490104303318,-48.957129339582)) ;
#63624=CARTESIAN_POINT('Ctrl Pts',(178.198641097553,584.540073278791,-48.9607168460511)) ;
#63625=CARTESIAN_POINT('Ctrl Pts',(178.148814213497,584.616809983714,-48.9658775253391)) ;
#63626=CARTESIAN_POINT('Ctrl Pts',(178.132980879125,584.64240825046,-48.9675438884388)) ;
#63627=CARTESIAN_POINT('Ctrl Pts',(178.099434896374,584.699405719882,-48.9711217962482)) ;
#63628=CARTESIAN_POINT('Ctrl Pts',(178.081975211821,584.730940269057,-48.9730190562814)) ;
#63629=CARTESIAN_POINT('Ctrl Pts',(178.044865471298,584.802335688029,-48.9771699064271)) ;
#63630=CARTESIAN_POINT('Ctrl Pts',(178.025660463273,584.842407764215,-48.9794027107795)) ;
#63631=CARTESIAN_POINT('Ctrl Pts',(177.962314334052,584.986383483853,-48.9871914348485)) ;
#63632=CARTESIAN_POINT('Ctrl Pts',(177.925448305642,585.093266179804,-48.9925637057962)) ;
#63633=CARTESIAN_POINT('Ctrl Pts',(177.873877502783,585.295414575354,-49.0027427539056)) ;
#63634=CARTESIAN_POINT('Ctrl Pts',(177.856724572656,585.389724127318,-49.0074980246381)) ;
#63635=CARTESIAN_POINT('Ctrl Pts',(177.840570104518,585.535912044658,-49.0151215943738)) ;
#63636=CARTESIAN_POINT('Ctrl Pts',(177.836845866824,585.587134834643,-49.0178380996845)) ;
#63637=CARTESIAN_POINT('Ctrl Pts',(177.833157123241,585.6921582474,-49.0235264691367)) ;
#63638=CARTESIAN_POINT('Ctrl Pts',(177.833379065138,585.745925210263,-49.0265021679117)) ;
#63639=CARTESIAN_POINT('Ctrl Pts',(177.838608917974,585.866481774079,-49.033327514973)) ;
#63640=CARTESIAN_POINT('Ctrl Pts',(177.844774267554,585.933158046879,-49.0372090984667)) ;
#63641=CARTESIAN_POINT('Ctrl Pts',(177.873441696996,586.13506393026,-49.0492495174707)) ;
#63642=CARTESIAN_POINT('Ctrl Pts',(177.906220531692,586.268441399001,-49.0576232844682)) ;
#63643=CARTESIAN_POINT('Ctrl Pts',(177.971353722208,586.452038896113,-49.0691718657179)) ;
#63644=CARTESIAN_POINT('Ctrl Pts',(177.992972818926,586.505682845048,-49.0725442484097)) ;
#63645=CARTESIAN_POINT('Ctrl Pts',(178.029191244183,586.585644459333,-49.0774950847042)) ;
#63646=CARTESIAN_POINT('Ctrl Pts',(178.042151912039,586.612669753336,-49.0791537483355)) ;
#63647=CARTESIAN_POINT('Ctrl Pts',(178.072414417961,586.672384959256,-49.0827751211145)) ;
#63648=CARTESIAN_POINT('Ctrl Pts',(178.090015742585,586.704909103596,-49.0847210505373)) ;
#63649=CARTESIAN_POINT('Ctrl Pts',(178.13146668355,586.776797264857,-49.0890010652727)) ;
#63650=CARTESIAN_POINT('Ctrl Pts',(178.15578028774,586.815871072237,-49.0913127622947)) ;
#63651=CARTESIAN_POINT('Ctrl Pts',(178.282026089867,587.004339213792,-49.1025487914152)) ;
#63652=CARTESIAN_POINT('Ctrl Pts',(178.402054396407,587.140634833927,-49.111026667567)) ;
#63653=CARTESIAN_POINT('Ctrl Pts',(178.570257765251,587.287254992632,-49.1224071453578)) ;
#63654=CARTESIAN_POINT('Ctrl Pts',(178.602987478482,587.314052749122,-49.1245976179241)) ;
#63655=CARTESIAN_POINT('Ctrl Pts',(178.636519276311,587.33982040643,-49.1268280924949)) ;
#63656=CARTESIAN_POINT('Origin',(212.388527625421,616.21056516053,-47.0221601717612)) ;
#63657=CARTESIAN_POINT('',(212.388527625421,616.71056516053,-47.0221601717612)) ;
#63658=CARTESIAN_POINT('',(212.388527625421,616.21056516053,-47.5221601717612)) ;
#63659=CARTESIAN_POINT('Origin',(212.388527625421,616.21056516053,-47.0221601717612)) ;
#63660=CARTESIAN_POINT('',(205.668527625421,616.710565160531,-47.0221601717609)) ;
#63661=CARTESIAN_POINT('',(212.388527625421,616.71056516053,-47.0221601717612)) ;
#63662=CARTESIAN_POINT('',(205.668527625421,616.210565160531,-47.5221601717609)) ;
#63663=CARTESIAN_POINT('Origin',(205.668527625421,616.210565160531,-47.0221601717609)) ;
#63664=CARTESIAN_POINT('',(212.388527625421,616.21056516053,-47.5221601717612)) ;
#63665=CARTESIAN_POINT('Origin',(-0.61147237455117,767.719724025967,-21.5221601717515)) ;
#63666=CARTESIAN_POINT('',(-2.61147237459719,505.710565160568,-21.5221601717515)) ;
#63667=CARTESIAN_POINT('',(-0.611472374577598,505.710565160568,-19.5221601717515)) ;
#63668=CARTESIAN_POINT('Origin',(-0.611472374597194,505.710565160567,-21.5221601717515)) ;
#63669=CARTESIAN_POINT('',(-2.61147237459754,503.710565160568,-21.5221601717515)) ;
#63670=CARTESIAN_POINT('',(-2.6114723745971,506.210565160568,-21.5221601717515)) ;
#63671=CARTESIAN_POINT('',(-0.611472374577924,503.710565160567,-19.5221601717515)) ;
#63672=CARTESIAN_POINT('Origin',(-0.611472374597545,503.710565160567,-21.5221601717515)) ;
#63673=CARTESIAN_POINT('',(-0.611472374577774,504.632344420872,-19.5221601717515)) ;
#63674=CARTESIAN_POINT('Origin',(210.388527625449,767.719724025931,-21.5221601717611)) ;
#63675=CARTESIAN_POINT('',(210.388527625403,505.71056516053,-19.5221601717611)) ;
#63676=CARTESIAN_POINT('',(212.388527625403,505.71056516053,-21.5221601717612)) ;
#63677=CARTESIAN_POINT('Origin',(210.388527625403,505.71056516053,-21.5221601717611)) ;
#63678=CARTESIAN_POINT('',(210.388527625403,503.71056516053,-19.5221601717611)) ;
#63679=CARTESIAN_POINT('',(210.388527625403,506.21056516053,-19.5221601717611)) ;
#63680=CARTESIAN_POINT('',(212.388527625402,503.71056516053,-21.5221601717612)) ;
#63681=CARTESIAN_POINT('Origin',(210.388527625403,503.71056516053,-21.5221601717611)) ;
#63682=CARTESIAN_POINT('',(212.388527625422,616.21056516053,-21.5221601717612)) ;
#63683=CARTESIAN_POINT('Origin',(210.388527625376,354.70143701573,-21.5221601717611)) ;
#63684=CARTESIAN_POINT('',(212.388527625422,616.71056516053,-21.5221601717612)) ;
#63685=CARTESIAN_POINT('',(210.388527625422,616.71056516053,-19.5221601717611)) ;
#63686=CARTESIAN_POINT('Origin',(210.388527625422,616.71056516053,-21.5221601717611)) ;
#63687=CARTESIAN_POINT('',(212.388527625423,618.71056516053,-21.5221601717612)) ;
#63688=CARTESIAN_POINT('',(212.388527625422,616.21056516053,-21.5221601717612)) ;
#63689=CARTESIAN_POINT('',(210.388527625423,618.71056516053,-19.5221601717611)) ;
#63690=CARTESIAN_POINT('Origin',(210.388527625423,618.71056516053,-21.5221601717611)) ;
#63691=CARTESIAN_POINT('',(210.388527625423,618.71056516053,-19.5221601717611)) ;
#63692=CARTESIAN_POINT('Origin',(-0.611472374623716,354.701437015767,-21.5221601717516)) ;
#63693=CARTESIAN_POINT('',(-0.611472374559485,616.710565160567,-19.5221601717515)) ;
#63694=CARTESIAN_POINT('',(-2.6114723745777,616.710565160568,-21.5221601717514)) ;
#63695=CARTESIAN_POINT('Origin',(-0.611472374577692,616.710565160567,-21.5221601717515)) ;
#63696=CARTESIAN_POINT('',(-0.611472374559158,618.710565160567,-19.5221601717515)) ;
#63697=CARTESIAN_POINT('',(-0.611472374577774,504.632344420872,-19.5221601717515)) ;
#63698=CARTESIAN_POINT('',(-2.61147237457735,618.710565160568,-21.5221601717514)) ;
#63699=CARTESIAN_POINT('Origin',(-0.611472374577341,618.710565160567,-21.5221601717515)) ;
#63700=CARTESIAN_POINT('',(-2.61147237457735,618.710565160568,-21.5221601717514)) ;
#63701=CARTESIAN_POINT('Origin',(212.388527625421,618.21056516053,-49.5221601717612)) ;
#63702=CARTESIAN_POINT('',(212.388527625402,506.210565160531,-47.5221601717613)) ;
#63703=CARTESIAN_POINT('',(212.388527625411,561.21056516053,-47.5221601717613)) ;
#63704=CARTESIAN_POINT('',(212.388527625402,505.71056516053,-47.0221601717613)) ;
#63705=CARTESIAN_POINT('Origin',(212.388527625402,506.21056516053,-47.0221601717613)) ;
#63706=CARTESIAN_POINT('',(212.388527625403,505.71056516053,-24.5221601717612)) ;
#63707=CARTESIAN_POINT('',(212.388527625401,503.71056516053,-47.5221601717613)) ;
#63708=CARTESIAN_POINT('',(212.388527625402,503.71056516053,-24.5221601717612)) ;
#63709=CARTESIAN_POINT('',(212.388527625402,505.71056516053,-49.5221601717612)) ;
#63710=CARTESIAN_POINT('Origin',(212.388527625402,505.71056516053,-47.5221601717612)) ;
#63711=CARTESIAN_POINT('',(212.388527625421,616.71056516053,-49.5221601717612)) ;
#63712=CARTESIAN_POINT('',(212.388527625411,561.21056516053,-49.5221601717612)) ;
#63713=CARTESIAN_POINT('',(212.388527625421,618.71056516053,-47.5221601717612)) ;
#63714=CARTESIAN_POINT('Origin',(212.388527625421,616.71056516053,-47.5221601717612)) ;
#63715=CARTESIAN_POINT('',(212.388527625421,618.71056516053,-49.5221601717612)) ;
#63716=CARTESIAN_POINT('',(212.388527625421,616.71056516053,-49.5221601717612)) ;
#63717=CARTESIAN_POINT('Origin',(-0.611472374624711,355.600165159967,-47.5221601717515)) ;
#63718=CARTESIAN_POINT('',(-2.6114723745982,506.335123681177,-47.5221601717515)) ;
#63719=CARTESIAN_POINT('',(-0.611472374598311,506.335123681177,-49.5221601717515)) ;
#63720=CARTESIAN_POINT('Origin',(-0.611472374598233,506.335123681177,-47.5221601717515)) ;
#63721=CARTESIAN_POINT('',(-2.61147237457892,616.077123681177,-47.5221601717515)) ;
#63722=CARTESIAN_POINT('',(-2.61147237459866,503.710565160568,-47.5221601717515)) ;
#63723=CARTESIAN_POINT('',(-0.611472374579034,616.077123681177,-49.5221601717515)) ;
#63724=CARTESIAN_POINT('Origin',(-0.611472374578956,616.077123681177,-47.5221601717515)) ;
#63725=CARTESIAN_POINT('',(-0.611472374598421,505.710565160567,-49.5221601717515)) ;
#63726=CARTESIAN_POINT('Origin',(0.388527625421986,503.131344420871,-46.5221601717516)) ;
#63727=CARTESIAN_POINT('',(-0.611472374577496,506.335123681177,-46.5221601717516)) ;
#63728=CARTESIAN_POINT('',(0.388527629159234,506.335123681176,-47.5221601717516)) ;
#63729=CARTESIAN_POINT('Origin',(0.388527625422509,506.335123681176,-46.5221601717516)) ;
#63730=CARTESIAN_POINT('',(0.388527629276449,616.077123681176,-47.5221601717516)) ;
#63731=CARTESIAN_POINT('',(0.388527625421941,503.131344420871,-47.5221601717516)) ;
#63732=CARTESIAN_POINT('',(-0.611472374559588,616.077123681177,-46.5221601717516)) ;
#63733=CARTESIAN_POINT('Origin',(0.388527625440417,616.077123681176,-46.5221601717516)) ;
#63734=CARTESIAN_POINT('',(-0.611472374578019,503.131344420871,-46.5221601717516)) ;
#63735=CARTESIAN_POINT('Origin',(212.388527625404,505.71056516053,0.477839828238782)) ;
#63736=CARTESIAN_POINT('',(104.888527625403,505.710565160549,-19.5221601717563)) ;
#63737=CARTESIAN_POINT('',(205.668527625402,505.710565160531,-47.022160171761)) ;
#63738=CARTESIAN_POINT('',(212.388527625402,505.71056516053,-47.0221601717613)) ;
#63739=CARTESIAN_POINT('',(205.668527625403,505.710565160531,-28.5221601717609)) ;
#63740=CARTESIAN_POINT('',(205.668527625403,505.710565160531,-24.5221601717609)) ;
#63741=CARTESIAN_POINT('',(201.668527625403,505.710565160532,-28.5221601717607)) ;
#63742=CARTESIAN_POINT('Origin',(203.668527625403,505.710565160532,-28.5221601717608)) ;
#63743=CARTESIAN_POINT('',(201.668527625402,505.710565160532,-47.0221601717608)) ;
#63744=CARTESIAN_POINT('',(201.668527625403,505.710565160532,-24.5221601717607)) ;
#63745=CARTESIAN_POINT('',(197.688527625402,505.710565160533,-47.0221601717606)) ;
#63746=CARTESIAN_POINT('',(212.388527625402,505.71056516053,-47.0221601717613)) ;
#63747=CARTESIAN_POINT('',(197.688527625403,505.710565160533,-28.5221601717605)) ;
#63748=CARTESIAN_POINT('',(197.688527625403,505.710565160533,-24.5221601717606)) ;
#63749=CARTESIAN_POINT('',(193.688527625403,505.710565160533,-28.5221601717604)) ;
#63750=CARTESIAN_POINT('Origin',(195.688527625403,505.710565160533,-28.5221601717604)) ;
#63751=CARTESIAN_POINT('',(193.688527625402,505.710565160533,-47.0221601717604)) ;
#63752=CARTESIAN_POINT('',(193.688527625403,505.710565160533,-24.5221601717604)) ;
#63753=CARTESIAN_POINT('',(0.388527634349991,505.710565160567,-47.0221601717516)) ;
#63754=CARTESIAN_POINT('',(212.388527625402,505.71056516053,-47.0221601717613)) ;
#63755=CARTESIAN_POINT('',(0.388527634349961,505.710565160567,-43.4900362557631)) ;
#63756=CARTESIAN_POINT('',(0.388527634349982,505.710565160567,-24.0060982137622)) ;
#63757=CARTESIAN_POINT('',(-2.61147237459819,505.710565160568,-43.4900362557631)) ;
#63758=CARTESIAN_POINT('',(103.388527625413,505.710565160549,-43.4900362557631)) ;
#63759=CARTESIAN_POINT('',(-2.6114723745962,505.710565160568,0.47783982824855)) ;
#63760=CARTESIAN_POINT('',(174.388527625403,505.710565160537,-25.7721601717595)) ;
#63761=CARTESIAN_POINT('',(171.638527625403,505.710565160537,-25.7721601717594)) ;
#63762=CARTESIAN_POINT('',(156.063527625403,505.71056516054,-25.7721601717586)) ;
#63763=CARTESIAN_POINT('',(171.638527625403,505.710565160537,-24.1221601717594)) ;
#63764=CARTESIAN_POINT('',(171.638527625403,505.710565160537,-24.1221601717594)) ;
#63765=CARTESIAN_POINT('',(87.7385276254027,505.710565160552,-24.1221601717556)) ;
#63766=CARTESIAN_POINT('',(171.638527625403,505.710565160537,-24.1221601717594)) ;
#63767=CARTESIAN_POINT('',(87.7385276254026,505.710565160552,-25.7721601717556)) ;
#63768=CARTESIAN_POINT('',(87.7385276254026,505.710565160552,-25.7721601717556)) ;
#63769=CARTESIAN_POINT('',(84.9885276254027,505.710565160552,-25.7721601717554)) ;
#63770=CARTESIAN_POINT('',(156.063527625403,505.71056516054,-25.7721601717586)) ;
#63771=CARTESIAN_POINT('',(84.9885276254021,505.710565160552,-38.1221601717554)) ;
#63772=CARTESIAN_POINT('',(84.9885276254033,505.710565160552,-11.8221601717554)) ;
#63773=CARTESIAN_POINT('',(89.9885276254019,505.710565358999,-43.122160465752)) ;
#63774=CARTESIAN_POINT('Origin',(89.9885276254021,505.710565160552,-38.1221601717556)) ;
#63775=CARTESIAN_POINT('',(169.388527625402,505.71056496209,-43.1221604706556)) ;
#63776=CARTESIAN_POINT('',(158.688527625402,505.710565160539,-43.1221607671016)) ;
#63777=CARTESIAN_POINT('',(174.388527625402,505.710565160537,-38.1221601717595)) ;
#63778=CARTESIAN_POINT('Origin',(169.388527625402,505.710565160538,-38.1221601717593)) ;
#63779=CARTESIAN_POINT('',(174.388527625402,505.710565160537,-37.2221601717595)) ;
#63780=CARTESIAN_POINT('',(174.388527625403,505.710565160537,-20.8221601717595)) ;
#63781=CARTESIAN_POINT('',(173.388527625402,505.710565160537,-37.2221601717594)) ;
#63782=CARTESIAN_POINT('',(192.888527625402,505.710565160533,-37.2221601717603)) ;
#63783=CARTESIAN_POINT('',(173.388527625402,505.710565160537,-30.2221601717594)) ;
#63784=CARTESIAN_POINT('',(173.388527625403,505.710565160537,-14.8721601717594)) ;
#63785=CARTESIAN_POINT('',(174.388527625402,505.710565160537,-30.2221601717595)) ;
#63786=CARTESIAN_POINT('',(191.888527625402,505.710565160534,-30.2221601717603)) ;
#63787=CARTESIAN_POINT('',(174.388527625403,505.710565160537,-20.8221601717595)) ;
#63788=CARTESIAN_POINT('',(181.555483800253,505.711440212721,-36.9689456432537)) ;
#63789=CARTESIAN_POINT('Ctrl Pts',(179.0652954453,505.710565160536,-38.9047876814238)) ;
#63790=CARTESIAN_POINT('Ctrl Pts',(179.135329608435,505.710565160536,-38.9278865069327)) ;
#63791=CARTESIAN_POINT('Ctrl Pts',(179.206482466064,505.710565160536,-38.9468076688786)) ;
#63792=CARTESIAN_POINT('Ctrl Pts',(179.278413970453,505.710565160536,-38.9616687602152)) ;
#63793=CARTESIAN_POINT('Ctrl Pts',(179.351549896252,505.710565160536,-38.9767786857272)) ;
#63794=CARTESIAN_POINT('Ctrl Pts',(179.425491802793,505.710565160536,-38.9876912772755)) ;
#63795=CARTESIAN_POINT('Ctrl Pts',(179.499885702151,505.710565160536,-38.9944761516692)) ;
#63796=CARTESIAN_POINT('Ctrl Pts',(179.574328731058,505.710565160536,-39.0012655067774)) ;
#63797=CARTESIAN_POINT('Ctrl Pts',(179.649225397864,505.710565160536,-39.003921398964)) ;
#63798=CARTESIAN_POINT('Ctrl Pts',(179.724208634386,505.710565160536,-39.0024636129629)) ;
#63799=CARTESIAN_POINT('Ctrl Pts',(179.740738841685,505.710565160536,-39.0021422410681)) ;
#63800=CARTESIAN_POINT('Ctrl Pts',(179.757273173814,505.710565160536,-39.0016207653068)) ;
#63801=CARTESIAN_POINT('Ctrl Pts',(179.77380753891,505.710565160536,-39.0008990928722)) ;
#63802=CARTESIAN_POINT('Ctrl Pts',(179.789271528614,505.710565160536,-39.0002241389182)) ;
#63803=CARTESIAN_POINT('Ctrl Pts',(179.804735546905,505.710565160536,-38.9993740682518)) ;
#63804=CARTESIAN_POINT('Ctrl Pts',(179.8201961877,505.710565160536,-38.9983487214072)) ;
#63805=CARTESIAN_POINT('Ctrl Pts',(179.834565840625,505.710565160536,-38.9973957286767)) ;
#63806=CARTESIAN_POINT('Ctrl Pts',(179.848934755005,505.710565160536,-38.996291021292)) ;
#63807=CARTESIAN_POINT('Ctrl Pts',(179.863277860849,505.710565160536,-38.9950366924248)) ;
#63808=CARTESIAN_POINT('Ctrl Pts',(179.936253785416,505.710565160536,-38.988654824384)) ;
#63809=CARTESIAN_POINT('Ctrl Pts',(180.008688241705,505.710565160536,-38.9783969957027)) ;
#63810=CARTESIAN_POINT('Ctrl Pts',(180.080246709531,505.710565160536,-38.9643329201609)) ;
#63811=CARTESIAN_POINT('Ctrl Pts',(180.150714553706,505.710565160536,-38.9504831953995)) ;
#63812=CARTESIAN_POINT('Ctrl Pts',(180.2203338107,505.710565160536,-38.9329419325712)) ;
#63813=CARTESIAN_POINT('Ctrl Pts',(180.288765667339,505.710565160536,-38.9117300713281)) ;
#63814=CARTESIAN_POINT('Ctrl Pts',(180.346723590668,505.710565160536,-38.8937648211074)) ;
#63815=CARTESIAN_POINT('Ctrl Pts',(180.403829740812,505.710565160536,-38.8731657442259)) ;
#63816=CARTESIAN_POINT('Ctrl Pts',(180.459860091428,505.710565160536,-38.8499225511445)) ;
#63817=CARTESIAN_POINT('Ctrl Pts',(180.48291298549,505.710565160536,-38.8403594686033)) ;
#63818=CARTESIAN_POINT('Ctrl Pts',(180.505783535886,505.710565160536,-38.8303485561633)) ;
#63819=CARTESIAN_POINT('Ctrl Pts',(180.528455065064,505.710565160536,-38.8198881408891)) ;
#63820=CARTESIAN_POINT('Ctrl Pts',(180.539030130832,505.710565160536,-38.8150089120284)) ;
#63821=CARTESIAN_POINT('Ctrl Pts',(180.549561885266,505.710565160536,-38.810031875954)) ;
#63822=CARTESIAN_POINT('Ctrl Pts',(180.560048582672,505.710565160536,-38.8049568234658)) ;
#63823=CARTESIAN_POINT('Ctrl Pts',(180.570864466054,505.710565160536,-38.7997224609455)) ;
#63824=CARTESIAN_POINT('Ctrl Pts',(180.581624773649,505.710565160536,-38.794387503373)) ;
#63825=CARTESIAN_POINT('Ctrl Pts',(180.592324290572,505.710565160536,-38.7889539836172)) ;
#63826=CARTESIAN_POINT('Ctrl Pts',(180.65367541487,505.710565160536,-38.7577981334676)) ;
#63827=CARTESIAN_POINT('Ctrl Pts',(180.713069228249,505.710565160536,-38.7233860504585)) ;
#63828=CARTESIAN_POINT('Ctrl Pts',(180.77020178144,505.710565160536,-38.6857410806322)) ;
#63829=CARTESIAN_POINT('Ctrl Pts',(180.822348458373,505.710565160536,-38.6513813335176)) ;
#63830=CARTESIAN_POINT('Ctrl Pts',(180.872611488785,505.710565160536,-38.6143276859924)) ;
#63831=CARTESIAN_POINT('Ctrl Pts',(180.92073330326,505.710565160536,-38.5745706438288)) ;
#63832=CARTESIAN_POINT('Ctrl Pts',(180.97729284033,505.710565160536,-38.5278425658338)) ;
#63833=CARTESIAN_POINT('Ctrl Pts',(181.030895815755,505.710565160536,-38.477379095277)) ;
#63834=CARTESIAN_POINT('Ctrl Pts',(181.081338141313,505.710565160536,-38.4235564497692)) ;
#63835=CARTESIAN_POINT('Ctrl Pts',(181.092527765842,505.710565160536,-38.4116169686347)) ;
#63836=CARTESIAN_POINT('Ctrl Pts',(181.103561628948,505.710565160536,-38.399512111087)) ;
#63837=CARTESIAN_POINT('Ctrl Pts',(181.114437100065,505.710565160536,-38.3872458806828)) ;
#63838=CARTESIAN_POINT('Ctrl Pts',(181.125083675749,505.710565160536,-38.3752378169457)) ;
#63839=CARTESIAN_POINT('Ctrl Pts',(181.135581757719,505.710565160536,-38.3630709576335)) ;
#63840=CARTESIAN_POINT('Ctrl Pts',(181.145909005854,505.710565160536,-38.3507731755607)) ;
#63841=CARTESIAN_POINT('Ctrl Pts',(181.190002102132,505.710565160536,-38.2982667109303)) ;
#63842=CARTESIAN_POINT('Ctrl Pts',(181.231048772417,505.710565160536,-38.2433074480089)) ;
#63843=CARTESIAN_POINT('Ctrl Pts',(181.268934008565,505.710565160536,-38.1862332430176)) ;
#63844=CARTESIAN_POINT('Ctrl Pts',(181.306814639129,505.710565160536,-38.1291659763522)) ;
#63845=CARTESIAN_POINT('Ctrl Pts',(181.341534914382,505.710565160536,-38.0699831659733)) ;
#63846=CARTESIAN_POINT('Ctrl Pts',(181.372931677357,505.710565160536,-38.0090034068331)) ;
#63847=CARTESIAN_POINT('Ctrl Pts',(181.395884966156,505.710565160536,-37.9644228230484)) ;
#63848=CARTESIAN_POINT('Ctrl Pts',(181.417060969264,505.710565160535,-37.9188813736391)) ;
#63849=CARTESIAN_POINT('Ctrl Pts',(181.436378199941,505.710565160536,-37.8725021900714)) ;
#63850=CARTESIAN_POINT('Ctrl Pts',(181.444366168592,505.710565160536,-37.8533236923572)) ;
#63851=CARTESIAN_POINT('Ctrl Pts',(181.452036113095,505.710565160536,-37.8340019566088)) ;
#63852=CARTESIAN_POINT('Ctrl Pts',(181.459381478451,505.710565160536,-37.8145457892129)) ;
#63853=CARTESIAN_POINT('Ctrl Pts',(181.464832557486,505.710565160536,-37.8001071464708)) ;
#63854=CARTESIAN_POINT('Ctrl Pts',(181.470104871676,505.710565160536,-37.7855944696366)) ;
#63855=CARTESIAN_POINT('Ctrl Pts',(181.475195571295,505.710565160535,-37.771011398043)) ;
#63856=CARTESIAN_POINT('Ctrl Pts',(181.479480142813,505.710565160535,-37.7587376011455)) ;
#63857=CARTESIAN_POINT('Ctrl Pts',(181.483633257897,505.710565160536,-37.746421893323)) ;
#63858=CARTESIAN_POINT('Ctrl Pts',(181.487652624753,505.710565160536,-37.7340700270267)) ;
#63859=CARTESIAN_POINT('Ctrl Pts',(181.508028361165,505.710565160536,-37.6714536048839)) ;
#63860=CARTESIAN_POINT('Ctrl Pts',(181.524981102548,505.710565160535,-37.6078787529545)) ;
#63861=CARTESIAN_POINT('Ctrl Pts',(181.538343022134,505.710565160536,-37.5436364340069)) ;
#63862=CARTESIAN_POINT('Ctrl Pts',(181.547803658224,505.710565160536,-37.4981509633619)) ;
#63863=CARTESIAN_POINT('Ctrl Pts',(181.555463195809,505.710565160536,-37.452330761803)) ;
#63864=CARTESIAN_POINT('Ctrl Pts',(181.56124651201,505.710565160536,-37.4062815313059)) ;
#63865=CARTESIAN_POINT('Ctrl Pts',(181.563093934278,505.710565160536,-37.3915715671793)) ;
#63866=CARTESIAN_POINT('Ctrl Pts',(181.56475002009,505.710565160536,-37.3768360133949)) ;
#63867=CARTESIAN_POINT('Ctrl Pts',(181.566211327952,505.710565160536,-37.3620856413917)) ;
#63868=CARTESIAN_POINT('Ctrl Pts',(181.572427964596,505.710565160536,-37.2993352070323)) ;
#63869=CARTESIAN_POINT('Ctrl Pts',(181.575112940977,505.710565160536,-37.2364324486792)) ;
#63870=CARTESIAN_POINT('Ctrl Pts',(181.574097520804,505.710565160536,-37.1736438710465)) ;
#63871=CARTESIAN_POINT('Ctrl Pts',(181.573151572664,505.710565160536,-37.1151511014797)) ;
#63872=CARTESIAN_POINT('Ctrl Pts',(181.568993905684,505.710565160536,-37.0567569444679)) ;
#63873=CARTESIAN_POINT('Ctrl Pts',(181.561449401405,505.710565160536,-36.9986897046275)) ;
#63874=CARTESIAN_POINT('Ctrl Pts',(181.560161212776,505.710565160536,-36.9887749964758)) ;
#63875=CARTESIAN_POINT('Ctrl Pts',(181.558774192941,505.710565160536,-36.9788698606881)) ;
#63876=CARTESIAN_POINT('Ctrl Pts',(181.557288983751,505.710565160535,-36.9689754712777)) ;
#63877=CARTESIAN_POINT('Ctrl Pts',(181.553679372624,505.711440212721,-36.969003246307)) ;
#63878=CARTESIAN_POINT('Ctrl Pts',(181.553434896476,505.711148528659,-36.9613449801169)) ;
#63879=CARTESIAN_POINT('Ctrl Pts',(181.553137587331,505.710856844597,-36.9536884005284)) ;
#63880=CARTESIAN_POINT('Ctrl Pts',(181.552787473488,505.710565160536,-36.9460342363074)) ;
#63881=CARTESIAN_POINT('Ctrl Pts',(179.569297170772,505.710565160536,-35.3870308445087)) ;
#63882=CARTESIAN_POINT('Ctrl Pts',(179.505455887236,505.710565160536,-35.3919881983916)) ;
#63883=CARTESIAN_POINT('Ctrl Pts',(179.442183898045,505.710565160536,-35.4009213613684)) ;
#63884=CARTESIAN_POINT('Ctrl Pts',(179.379716462264,505.710565160536,-35.4135293431981)) ;
#63885=CARTESIAN_POINT('Ctrl Pts',(179.317249026483,505.710565160536,-35.4261373250277)) ;
#63886=CARTESIAN_POINT('Ctrl Pts',(179.255585363968,505.710565160536,-35.4424204680216)) ;
#63887=CARTESIAN_POINT('Ctrl Pts',(179.194950373845,505.710565160536,-35.4621332783491)) ;
#63888=CARTESIAN_POINT('Ctrl Pts',(179.140136352604,505.710565160536,-35.4799536556892)) ;
#63889=CARTESIAN_POINT('Ctrl Pts',(179.086162428757,505.710565160536,-35.5005776890217)) ;
#63890=CARTESIAN_POINT('Ctrl Pts',(179.033195548199,505.710565160536,-35.5238594749927)) ;
#63891=CARTESIAN_POINT('Ctrl Pts',(179.006578591245,505.710565160536,-35.5355590557208)) ;
#63892=CARTESIAN_POINT('Ctrl Pts',(178.980216000577,505.710565160536,-35.5479302990645)) ;
#63893=CARTESIAN_POINT('Ctrl Pts',(178.954129652167,505.710565160536,-35.5609576253808)) ;
#63894=CARTESIAN_POINT('Ctrl Pts',(178.942328077973,505.710565160536,-35.5668512428259)) ;
#63895=CARTESIAN_POINT('Ctrl Pts',(178.930581721253,505.710565160536,-35.572880003767)) ;
#63896=CARTESIAN_POINT('Ctrl Pts',(178.918911283598,505.710565160536,-35.579032359671)) ;
#63897=CARTESIAN_POINT('Ctrl Pts',(178.859681619721,505.710565160536,-35.6102567218602)) ;
#63898=CARTESIAN_POINT('Ctrl Pts',(178.802297253821,505.710565160536,-35.6447138932495)) ;
#63899=CARTESIAN_POINT('Ctrl Pts',(178.74699869452,505.710565160536,-35.6821359841794)) ;
#63900=CARTESIAN_POINT('Ctrl Pts',(178.690694275589,505.710565160536,-35.7202387686217)) ;
#63901=CARTESIAN_POINT('Ctrl Pts',(178.636551275762,505.710565160536,-35.7614156281894)) ;
#63902=CARTESIAN_POINT('Ctrl Pts',(178.584831529575,505.710565160536,-35.805436907624)) ;
#63903=CARTESIAN_POINT('Ctrl Pts',(178.541450424535,505.710565160536,-35.84236074983)) ;
#63904=CARTESIAN_POINT('Ctrl Pts',(178.499774013886,505.710565160536,-35.8812868352562)) ;
#63905=CARTESIAN_POINT('Ctrl Pts',(178.459968650475,505.710565160536,-35.9221049529937)) ;
#63906=CARTESIAN_POINT('Ctrl Pts',(178.441578208832,505.710565160536,-35.9409632963904)) ;
#63907=CARTESIAN_POINT('Ctrl Pts',(178.423587340823,505.710565160536,-35.9602258002509)) ;
#63908=CARTESIAN_POINT('Ctrl Pts',(178.406013633541,505.710565160536,-35.9798830591776)) ;
#63909=CARTESIAN_POINT('Ctrl Pts',(178.398443666251,505.710565160536,-35.9883505273504)) ;
#63910=CARTESIAN_POINT('Ctrl Pts',(178.390951571984,505.710565160536,-35.9968908681941)) ;
#63911=CARTESIAN_POINT('Ctrl Pts',(178.383547395181,505.710565160536,-36.0054929611087)) ;
#63912=CARTESIAN_POINT('Ctrl Pts',(178.33772699916,505.710565160536,-36.0587266040186)) ;
#63913=CARTESIAN_POINT('Ctrl Pts',(178.295182788124,505.710565160536,-36.1144199624445)) ;
#63914=CARTESIAN_POINT('Ctrl Pts',(178.25618213975,505.710565160536,-36.1723214142079)) ;
#63915=CARTESIAN_POINT('Ctrl Pts',(178.221114088011,505.710565160536,-36.22438442318)) ;
#63916=CARTESIAN_POINT('Ctrl Pts',(178.188910651079,505.710565160536,-36.2782336378472)) ;
#63917=CARTESIAN_POINT('Ctrl Pts',(178.159784940565,505.710565160536,-36.3337168679626)) ;
#63918=CARTESIAN_POINT('Ctrl Pts',(178.128216735146,505.710565160536,-36.393852946179)) ;
#63919=CARTESIAN_POINT('Ctrl Pts',(178.10026275254,505.710565160536,-36.4559086037906)) ;
#63920=CARTESIAN_POINT('Ctrl Pts',(178.075864414872,505.710565160536,-36.519565756551)) ;
#63921=CARTESIAN_POINT('Ctrl Pts',(178.066551119335,505.710565160536,-36.5438648659713)) ;
#63922=CARTESIAN_POINT('Ctrl Pts',(178.057756368665,505.710565160536,-36.5683976281922)) ;
#63923=CARTESIAN_POINT('Ctrl Pts',(178.049478616365,505.710565160536,-36.5931473112284)) ;
#63924=CARTESIAN_POINT('Ctrl Pts',(178.045832898525,505.710565160536,-36.6040476568441)) ;
#63925=CARTESIAN_POINT('Ctrl Pts',(178.042287878707,505.710565160536,-36.6149891360053)) ;
#63926=CARTESIAN_POINT('Ctrl Pts',(178.038847045237,505.710565160536,-36.6259579956453)) ;
#63927=CARTESIAN_POINT('Ctrl Pts',(178.01790405103,505.710565160536,-36.6927211115773)) ;
#63928=CARTESIAN_POINT('Ctrl Pts',(178.000777075959,505.710565160536,-36.7606143234727)) ;
#63929=CARTESIAN_POINT('Ctrl Pts',(177.987357778769,505.710565160536,-36.8292734696092)) ;
#63930=CARTESIAN_POINT('Ctrl Pts',(177.973630974354,505.710565160536,-36.8995059606954)) ;
#63931=CARTESIAN_POINT('Ctrl Pts',(177.963783447185,505.710565160536,-36.9705407196561)) ;
#63932=CARTESIAN_POINT('Ctrl Pts',(177.957745517187,505.710565160536,-37.0420198942905)) ;
#63933=CARTESIAN_POINT('Ctrl Pts',(177.953182960546,505.710565160536,-37.0960330714913)) ;
#63934=CARTESIAN_POINT('Ctrl Pts',(177.95079664825,505.710565160536,-37.1503007792799)) ;
#63935=CARTESIAN_POINT('Ctrl Pts',(177.950574798142,505.710565160536,-37.2046756703304)) ;
#63936=CARTESIAN_POINT('Ctrl Pts',(177.950437322557,505.710565160536,-37.2383705827585)) ;
#63937=CARTESIAN_POINT('Ctrl Pts',(177.951131314102,505.710565160536,-37.2721067525419)) ;
#63938=CARTESIAN_POINT('Ctrl Pts',(177.952657081778,505.710565160536,-37.3058495799569)) ;
#63939=CARTESIAN_POINT('Ctrl Pts',(177.953240450954,505.710565160536,-37.3187509709948)) ;
#63940=CARTESIAN_POINT('Ctrl Pts',(177.953945590571,505.710565160536,-37.3316556206205)) ;
#63941=CARTESIAN_POINT('Ctrl Pts',(177.954772122753,505.710565160536,-37.3445541442168)) ;
#63942=CARTESIAN_POINT('Ctrl Pts',(177.95967870594,505.710565160536,-37.4211242770651)) ;
#63943=CARTESIAN_POINT('Ctrl Pts',(177.968845134531,505.710565160536,-37.4972918701055)) ;
#63944=CARTESIAN_POINT('Ctrl Pts',(177.982203495705,505.710565160536,-37.5726433698151)) ;
#63945=CARTESIAN_POINT('Ctrl Pts',(177.992222266586,505.710565160536,-37.6291569945974)) ;
#63946=CARTESIAN_POINT('Ctrl Pts',(178.004600133923,505.710565160536,-37.6852122341676)) ;
#63947=CARTESIAN_POINT('Ctrl Pts',(178.019329553784,505.710565160536,-37.7406380121571)) ;
#63948=CARTESIAN_POINT('Ctrl Pts',(178.024555821147,505.710565160536,-37.7603040911526)) ;
#63949=CARTESIAN_POINT('Ctrl Pts',(178.030078307587,505.710565160536,-37.7798909242228)) ;
#63950=CARTESIAN_POINT('Ctrl Pts',(178.035897233864,505.710565160536,-37.7993908321457)) ;
#63951=CARTESIAN_POINT('Ctrl Pts',(178.040304327293,505.710565160536,-37.8141595217615)) ;
#63952=CARTESIAN_POINT('Ctrl Pts',(178.044880075823,505.710565160536,-37.8288734635663)) ;
#63953=CARTESIAN_POINT('Ctrl Pts',(178.049621681044,505.710565160536,-37.8435217616764)) ;
#63954=CARTESIAN_POINT('Ctrl Pts',(178.072814492169,505.710565160536,-37.9151715923815)) ;
#63955=CARTESIAN_POINT('Ctrl Pts',(178.099987870132,505.710565160536,-37.9853065120389)) ;
#63956=CARTESIAN_POINT('Ctrl Pts',(178.1311097997,505.710565160536,-38.053547573471)) ;
#63957=CARTESIAN_POINT('Ctrl Pts',(178.156254670014,505.710565160536,-38.1086827358345)) ;
#63958=CARTESIAN_POINT('Ctrl Pts',(178.18397801006,505.710565160536,-38.1625820233426)) ;
#63959=CARTESIAN_POINT('Ctrl Pts',(178.214287553404,505.710565160536,-38.2150417422617)) ;
#63960=CARTESIAN_POINT('Ctrl Pts',(178.220262521689,505.710565160536,-38.2253832097409)) ;
#63961=CARTESIAN_POINT('Ctrl Pts',(178.226338061256,505.710565160578,-38.235668711766)) ;
#63962=CARTESIAN_POINT('Ctrl Pts',(178.232512830637,505.710565160538,-38.2458977135592)) ;
#63963=CARTESIAN_POINT('',(31.555447115217,505.711420702611,-36.9690600226526)) ;
#63964=CARTESIAN_POINT('Ctrl Pts',(29.0652954452959,505.710565160562,-38.9047876814153)) ;
#63965=CARTESIAN_POINT('Ctrl Pts',(29.1351327058573,505.710565160562,-38.9278215640738)) ;
#63966=CARTESIAN_POINT('Ctrl Pts',(29.2060816765201,505.710565160562,-38.9467022836268)) ;
#63967=CARTESIAN_POINT('Ctrl Pts',(29.2778052840572,505.710565160562,-38.9615463226794)) ;
#63968=CARTESIAN_POINT('Ctrl Pts',(29.3511852087307,505.710565160562,-38.9767331559262)) ;
#63969=CARTESIAN_POINT('Ctrl Pts',(29.4253770054866,505.710565160562,-38.987694611082)) ;
#63970=CARTESIAN_POINT('Ctrl Pts',(29.5000231783554,505.710565160562,-38.9945008791182)) ;
#63971=CARTESIAN_POINT('Ctrl Pts',(29.5628201759124,505.710565160562,-39.0002267345883)) ;
#63972=CARTESIAN_POINT('Ctrl Pts',(29.6259391294217,505.710565160562,-39.0030108311892)) ;
#63973=CARTESIAN_POINT('Ctrl Pts',(29.6891607397903,505.710565160562,-39.00286714337)) ;
#63974=CARTESIAN_POINT('Ctrl Pts',(29.7173582483808,505.710565160562,-39.0028030570791)) ;
#63975=CARTESIAN_POINT('Ctrl Pts',(29.7455760540432,505.710565160562,-39.0021562353623)) ;
#63976=CARTESIAN_POINT('Ctrl Pts',(29.7737939403674,505.710565160562,-39.000926394963)) ;
#63977=CARTESIAN_POINT('Ctrl Pts',(29.789259057995,505.710565160562,-39.0002523676379)) ;
#63978=CARTESIAN_POINT('Ctrl Pts',(29.8047241901967,505.710565160562,-38.9994032025605)) ;
#63979=CARTESIAN_POINT('Ctrl Pts',(29.8201859307895,505.710565160562,-38.9983787384855)) ;
#63980=CARTESIAN_POINT('Ctrl Pts',(29.8345524038282,505.710565160562,-38.9974268446529)) ;
#63981=CARTESIAN_POINT('Ctrl Pts',(29.8489181231788,505.710565160562,-38.9963233055562)) ;
#63982=CARTESIAN_POINT('Ctrl Pts',(29.8632580326653,505.710565160562,-38.9950702105724)) ;
#63983=CARTESIAN_POINT('Ctrl Pts',(29.9362310424626,505.710565160562,-38.9886934539679)) ;
#63984=CARTESIAN_POINT('Ctrl Pts',(30.0086623333364,505.710565160562,-38.9784410223258)) ;
#63985=CARTESIAN_POINT('Ctrl Pts',(30.0802175001885,505.710565160562,-38.9643824410455)) ;
#63986=CARTESIAN_POINT('Ctrl Pts',(30.15068071892,505.710565160562,-38.950538396913)) ;
#63987=CARTESIAN_POINT('Ctrl Pts',(30.2202952517954,505.710565160562,-38.9330030533077)) ;
#63988=CARTESIAN_POINT('Ctrl Pts',(30.288722414559,505.710565160562,-38.9117971678137)) ;
#63989=CARTESIAN_POINT('Ctrl Pts',(30.3466769629711,505.710565160562,-38.8938367926082)) ;
#63990=CARTESIAN_POINT('Ctrl Pts',(30.40377974218,505.710565160562,-38.87324257691)) ;
#63991=CARTESIAN_POINT('Ctrl Pts',(30.4598067999162,505.710565160562,-38.8500041179199)) ;
#63992=CARTESIAN_POINT('Ctrl Pts',(30.4828591313975,505.710565160562,-38.8404426545591)) ;
#63993=CARTESIAN_POINT('Ctrl Pts',(30.5057291199309,505.710565160562,-38.8304333089539)) ;
#63994=CARTESIAN_POINT('Ctrl Pts',(30.52840009156,505.710565160562,-38.8199743998416)) ;
#63995=CARTESIAN_POINT('Ctrl Pts',(30.5389784366907,505.710565160562,-38.8150942406631)) ;
#63996=CARTESIAN_POINT('Ctrl Pts',(30.5495134424306,505.710565160562,-38.8101161955752)) ;
#63997=CARTESIAN_POINT('Ctrl Pts',(30.5600033616957,505.710565160562,-38.8050400542981)) ;
#63998=CARTESIAN_POINT('Ctrl Pts',(30.5708146480521,505.710565160562,-38.799808401361)) ;
#63999=CARTESIAN_POINT('Ctrl Pts',(30.5815703870052,505.710565160562,-38.7944762261743)) ;
#64000=CARTESIAN_POINT('Ctrl Pts',(30.5922653929186,505.710565160562,-38.7890455472562)) ;
#64001=CARTESIAN_POINT('Ctrl Pts',(30.6536123337932,505.710565160562,-38.7578949764942)) ;
#64002=CARTESIAN_POINT('Ctrl Pts',(30.7130021980142,505.710565160562,-38.7234879257198)) ;
#64003=CARTESIAN_POINT('Ctrl Pts',(30.7701311541928,505.710565160562,-38.6858475731534)) ;
#64004=CARTESIAN_POINT('Ctrl Pts',(30.8222745637724,505.710565160562,-38.6514920299774)) ;
#64005=CARTESIAN_POINT('Ctrl Pts',(30.8725346189327,505.710565160562,-38.6144422392586)) ;
#64006=CARTESIAN_POINT('Ctrl Pts',(30.9206538443866,505.710565160562,-38.5746885745686)) ;
#64007=CARTESIAN_POINT('Ctrl Pts',(30.9747624901138,505.710565160562,-38.5299867544796)) ;
#64008=CARTESIAN_POINT('Ctrl Pts',(31.0261650707763,505.710565160562,-38.4818651599855)) ;
#64009=CARTESIAN_POINT('Ctrl Pts',(31.0746839447929,505.710565160562,-38.4306536883031)) ;
#64010=CARTESIAN_POINT('Ctrl Pts',(31.0881297831313,505.710565160562,-38.4164616613184)) ;
#64011=CARTESIAN_POINT('Ctrl Pts',(31.1013538653161,505.710565160562,-38.4020322344394)) ;
#64012=CARTESIAN_POINT('Ctrl Pts',(31.1143517243842,505.710565160562,-38.3873722484095)) ;
#64013=CARTESIAN_POINT('Ctrl Pts',(31.1249977190283,505.710565160562,-38.3753648761231)) ;
#64014=CARTESIAN_POINT('Ctrl Pts',(31.1354952461008,505.710565160562,-38.3631986878532)) ;
#64015=CARTESIAN_POINT('Ctrl Pts',(31.1458219666048,505.710565160562,-38.3509015553636)) ;
#64016=CARTESIAN_POINT('Ctrl Pts',(31.1899669478989,505.710565160562,-38.2983333965264)) ;
#64017=CARTESIAN_POINT('Ctrl Pts',(31.2310585244121,505.710565160562,-38.2433060254466)) ;
#64018=CARTESIAN_POINT('Ctrl Pts',(31.2689811923208,505.710565160562,-38.1861585964737)) ;
#64019=CARTESIAN_POINT('Ctrl Pts',(31.3068004310769,505.710565160562,-38.1291670296929)) ;
#64020=CARTESIAN_POINT('Ctrl Pts',(31.3414683117142,505.710565160562,-38.0700658327551)) ;
#64021=CARTESIAN_POINT('Ctrl Pts',(31.3728222915957,505.710565160562,-38.0091723393296)) ;
#64022=CARTESIAN_POINT('Ctrl Pts',(31.3957833184136,505.710565160562,-37.9645790487536)) ;
#64023=CARTESIAN_POINT('Ctrl Pts',(31.4169661685957,505.710565160562,-37.9190241163557)) ;
#64024=CARTESIAN_POINT('Ctrl Pts',(31.4362892673506,505.710565160562,-37.8726308157318)) ;
#64025=CARTESIAN_POINT('Ctrl Pts',(31.4442773849114,505.710565160562,-37.8534519488161)) ;
#64026=CARTESIAN_POINT('Ctrl Pts',(31.4519474920606,505.710565160562,-37.8341298171632)) ;
#64027=CARTESIAN_POINT('Ctrl Pts',(31.4592930323279,505.710565160562,-37.8146732297774)) ;
#64028=CARTESIAN_POINT('Ctrl Pts',(31.4647427469936,505.710565160562,-37.8002382330635)) ;
#64029=CARTESIAN_POINT('Ctrl Pts',(31.470013801544,505.710565160562,-37.7857292295818)) ;
#64030=CARTESIAN_POINT('Ctrl Pts',(31.4751033480087,505.710565160562,-37.7711498567442)) ;
#64031=CARTESIAN_POINT('Ctrl Pts',(31.4793889286833,505.710565160562,-37.7588735018837)) ;
#64032=CARTESIAN_POINT('Ctrl Pts',(31.4835430111578,505.710565160562,-37.7465552026881)) ;
#64033=CARTESIAN_POINT('Ctrl Pts',(31.4875632978035,505.710565160562,-37.7342007273561)) ;
#64034=CARTESIAN_POINT('Ctrl Pts',(31.5079397140028,505.710565160562,-37.6715833188298)) ;
#64035=CARTESIAN_POINT('Ctrl Pts',(31.5248932906129,505.710565160562,-37.6080072908746)) ;
#64036=CARTESIAN_POINT('Ctrl Pts',(31.5382561567857,505.710565160562,-37.5437636875823)) ;
#64037=CARTESIAN_POINT('Ctrl Pts',(31.5477173363443,505.710565160562,-37.4982779169113)) ;
#64038=CARTESIAN_POINT('Ctrl Pts',(31.5553775214832,505.710565160562,-37.4524573699572)) ;
#64039=CARTESIAN_POINT('Ctrl Pts',(31.5611615768446,505.710565160562,-37.4064077734896)) ;
#64040=CARTESIAN_POINT('Ctrl Pts',(31.5643673337055,505.710565160562,-37.380885229082)) ;
#64041=CARTESIAN_POINT('Ctrl Pts',(31.5669968524272,505.710565160562,-37.3552836260987)) ;
#64042=CARTESIAN_POINT('Ctrl Pts',(31.569032642096,505.710565160562,-37.329672801237)) ;
#64043=CARTESIAN_POINT('Ctrl Pts',(31.5740111853602,505.710565160562,-37.2670412820962)) ;
#64044=CARTESIAN_POINT('Ctrl Pts',(31.5754510607237,505.710565160562,-37.2043032363127)) ;
#64045=CARTESIAN_POINT('Ctrl Pts',(31.5731765569328,505.710565160562,-37.1417251266716)) ;
#64046=CARTESIAN_POINT('Ctrl Pts',(31.5714400801884,505.710565160562,-37.0939496810844)) ;
#64047=CARTESIAN_POINT('Ctrl Pts',(31.5675377050921,505.710565160562,-37.0462674954266)) ;
#64048=CARTESIAN_POINT('Ctrl Pts',(31.5613718805554,505.710565160562,-36.9988040978121)) ;
#64049=CARTESIAN_POINT('Ctrl Pts',(31.5600838674012,505.710565160562,-36.988889206445)) ;
#64050=CARTESIAN_POINT('Ctrl Pts',(31.558697022611,505.710565160562,-36.9789838905892)) ;
#64051=CARTESIAN_POINT('Ctrl Pts',(31.5572119880889,505.710565160562,-36.9690893241484)) ;
#64052=CARTESIAN_POINT('Ctrl Pts',(31.5536829752598,505.711420702611,-36.9691162197847)) ;
#64053=CARTESIAN_POINT('Ctrl Pts',(31.5534444962862,505.711135521928,-36.9616298895976)) ;
#64054=CARTESIAN_POINT('Ctrl Pts',(31.553155530141,505.710850341245,-36.9541451676964)) ;
#64055=CARTESIAN_POINT('Ctrl Pts',(31.5528161031074,505.710565160562,-36.9466627348581)) ;
#64056=CARTESIAN_POINT('Ctrl Pts',(29.5692971707754,505.710565160562,-35.3870308445009)) ;
#64057=CARTESIAN_POINT('Ctrl Pts',(29.5072625869895,505.710565160562,-35.3918479059347)) ;
#64058=CARTESIAN_POINT('Ctrl Pts',(29.4457654429815,505.710565160562,-35.4004180593316)) ;
#64059=CARTESIAN_POINT('Ctrl Pts',(29.3850217861476,505.710565160562,-35.4124646102939)) ;
#64060=CARTESIAN_POINT('Ctrl Pts',(29.3220357794238,505.710565160562,-35.4249558592481)) ;
#64061=CARTESIAN_POINT('Ctrl Pts',(29.2598592126282,505.710565160562,-35.4411849077502)) ;
#64062=CARTESIAN_POINT('Ctrl Pts',(29.1987222577426,505.710565160562,-35.460899523258)) ;
#64063=CARTESIAN_POINT('Ctrl Pts',(29.1426079052272,505.710565160562,-35.4789945181164)) ;
#64064=CARTESIAN_POINT('Ctrl Pts',(29.0873687600192,505.710565160562,-35.5000267520628)) ;
#64065=CARTESIAN_POINT('Ctrl Pts',(29.0331835132918,505.710565160562,-35.5238397755035)) ;
#64066=CARTESIAN_POINT('Ctrl Pts',(29.0065636304015,505.710565160562,-35.5355385299346)) ;
#64067=CARTESIAN_POINT('Ctrl Pts',(28.9801981719153,505.710565160562,-35.5479089719437)) ;
#64068=CARTESIAN_POINT('Ctrl Pts',(28.9541090217123,505.710565160562,-35.5609355344341)) ;
#64069=CARTESIAN_POINT('Ctrl Pts',(28.9423122115306,505.710565160562,-35.5668257947079)) ;
#64070=CARTESIAN_POINT('Ctrl Pts',(28.9305705845767,505.710565160562,-35.572851063511)) ;
#64071=CARTESIAN_POINT('Ctrl Pts',(28.9189048179306,505.710565160562,-35.5789998089842)) ;
#64072=CARTESIAN_POINT('Ctrl Pts',(28.8596712661301,505.710565160562,-35.6102203917833)) ;
#64073=CARTESIAN_POINT('Ctrl Pts',(28.8022832597293,505.710565160562,-35.6446737270167)) ;
#64074=CARTESIAN_POINT('Ctrl Pts',(28.7469813608305,505.710565160562,-35.6820920937285)) ;
#64075=CARTESIAN_POINT('Ctrl Pts',(28.6906751156464,505.710565160562,-35.7201900211489)) ;
#64076=CARTESIAN_POINT('Ctrl Pts',(28.6365304804,505.710565160562,-35.7613619677535)) ;
#64077=CARTESIAN_POINT('Ctrl Pts',(28.5848093271771,505.710565160562,-35.8053784761555)) ;
#64078=CARTESIAN_POINT('Ctrl Pts',(28.541430437791,505.710565160562,-35.8422954265743)) ;
#64079=CARTESIAN_POINT('Ctrl Pts',(28.4997561367543,505.710565160562,-35.8812144066662)) ;
#64080=CARTESIAN_POINT('Ctrl Pts',(28.4599527622968,505.710565160562,-35.9220253479791)) ;
#64081=CARTESIAN_POINT('Ctrl Pts',(28.4415595226414,505.710565160562,-35.9408841868178)) ;
#64082=CARTESIAN_POINT('Ctrl Pts',(28.423565992348,505.710565160563,-35.9601473342408)) ;
#64083=CARTESIAN_POINT('Ctrl Pts',(28.4059897676973,505.710565160563,-35.9798053930658)) ;
#64084=CARTESIAN_POINT('Ctrl Pts',(28.3984223584326,505.710565160563,-35.9882691319765)) ;
#64085=CARTESIAN_POINT('Ctrl Pts',(28.3909327876458,505.710565160563,-35.9968056872066)) ;
#64086=CARTESIAN_POINT('Ctrl Pts',(28.3835310782131,505.710565160563,-36.0054039637556)) ;
#64087=CARTESIAN_POINT('Ctrl Pts',(28.3377108760982,505.710565160563,-36.0586315016502)) ;
#64088=CARTESIAN_POINT('Ctrl Pts',(28.2951669675323,505.710565160563,-36.1143190826752)) ;
#64089=CARTESIAN_POINT('Ctrl Pts',(28.2561667463011,505.710565160563,-36.1722153095195)) ;
#64090=CARTESIAN_POINT('Ctrl Pts',(28.2211039769088,505.710565160563,-36.2242663488837)) ;
#64091=CARTESIAN_POINT('Ctrl Pts',(28.188905123424,505.710565160563,-36.2781035417552)) ;
#64092=CARTESIAN_POINT('Ctrl Pts',(28.1597832202372,505.710565160563,-36.333574922188)) ;
#64093=CARTESIAN_POINT('Ctrl Pts',(28.1282157438182,505.710565160563,-36.3937046287703)) ;
#64094=CARTESIAN_POINT('Ctrl Pts',(28.1002623563384,505.710565160563,-36.4557545291069)) ;
#64095=CARTESIAN_POINT('Ctrl Pts',(28.0758644739581,505.710565160563,-36.5194064672103)) ;
#64096=CARTESIAN_POINT('Ctrl Pts',(28.0665506287128,505.710565160563,-36.5437054736492)) ;
#64097=CARTESIAN_POINT('Ctrl Pts',(28.0577553884762,505.710565160563,-36.568238248327)) ;
#64098=CARTESIAN_POINT('Ctrl Pts',(28.0494772059523,505.710565160563,-36.5929880516034)) ;
#64099=CARTESIAN_POINT('Ctrl Pts',(28.0458314162721,505.710565160563,-36.6038880984567)) ;
#64100=CARTESIAN_POINT('Ctrl Pts',(28.0422863296697,505.710565160563,-36.6148292970828)) ;
#64101=CARTESIAN_POINT('Ctrl Pts',(28.0388454345643,505.710565160563,-36.6257978938512)) ;
#64102=CARTESIAN_POINT('Ctrl Pts',(28.0180863229789,505.710565160563,-36.6919720483306)) ;
#64103=CARTESIAN_POINT('Ctrl Pts',(28.0010766258327,505.710565160563,-36.7592571926018)) ;
#64104=CARTESIAN_POINT('Ctrl Pts',(27.9877106391096,505.710565160563,-36.8272984172306)) ;
#64105=CARTESIAN_POINT('Ctrl Pts',(27.9739059651428,505.710565160563,-36.8975728340585)) ;
#64106=CARTESIAN_POINT('Ctrl Pts',(27.963987764797,505.710565160563,-36.9686545452015)) ;
#64107=CARTESIAN_POINT('Ctrl Pts',(27.9578857860212,505.710565160563,-37.0401845046639)) ;
#64108=CARTESIAN_POINT('Ctrl Pts',(27.9532312624418,505.710565160563,-37.0947467860456)) ;
#64109=CARTESIAN_POINT('Ctrl Pts',(27.9507981351901,505.710565160563,-37.1495706606258)) ;
#64110=CARTESIAN_POINT('Ctrl Pts',(27.9505741662839,505.710565160563,-37.2045041243709)) ;
#64111=CARTESIAN_POINT('Ctrl Pts',(27.9504367813379,505.710565160563,-37.2382009043224)) ;
#64112=CARTESIAN_POINT('Ctrl Pts',(27.951130965593,505.710565160563,-37.271939021478)) ;
#64113=CARTESIAN_POINT('Ctrl Pts',(27.952657027207,505.710565160563,-37.3056838599239)) ;
#64114=CARTESIAN_POINT('Ctrl Pts',(27.953240415664,505.710565160563,-37.3185839611059)) ;
#64115=CARTESIAN_POINT('Ctrl Pts',(27.9539455506795,505.710565160563,-37.3314873315597)) ;
#64116=CARTESIAN_POINT('Ctrl Pts',(27.954772053826,505.710565160563,-37.3443845802242)) ;
#64117=CARTESIAN_POINT('Ctrl Pts',(27.959678903322,505.710565160563,-37.4209539900082)) ;
#64118=CARTESIAN_POINT('Ctrl Pts',(27.9688455129901,505.710565160563,-37.4971211765398)) ;
#64119=CARTESIAN_POINT('Ctrl Pts',(27.9822039608736,505.710565160563,-37.5724724789569)) ;
#64120=CARTESIAN_POINT('Ctrl Pts',(27.9922227967861,505.710565160563,-37.6289859557697)) ;
#64121=CARTESIAN_POINT('Ctrl Pts',(28.0046006760498,505.710565160562,-37.6850411652294)) ;
#64122=CARTESIAN_POINT('Ctrl Pts',(28.0193300502471,505.710565160562,-37.7404669874564)) ;
#64123=CARTESIAN_POINT('Ctrl Pts',(28.0245595644987,505.710565160562,-37.7601453609814)) ;
#64124=CARTESIAN_POINT('Ctrl Pts',(28.030085660545,505.710565160563,-37.7797443989801)) ;
#64125=CARTESIAN_POINT('Ctrl Pts',(28.0359085594318,505.710565160563,-37.799256405901)) ;
#64126=CARTESIAN_POINT('Ctrl Pts',(28.040317895285,505.710565160563,-37.8140316910907)) ;
#64127=CARTESIAN_POINT('Ctrl Pts',(28.0448960245853,505.710565160563,-37.8287521502641)) ;
#64128=CARTESIAN_POINT('Ctrl Pts',(28.049640158209,505.710565160563,-37.8434069169089)) ;
#64129=CARTESIAN_POINT('Ctrl Pts',(28.0728350792194,505.710565160563,-37.9150567020365)) ;
#64130=CARTESIAN_POINT('Ctrl Pts',(28.100010513494,505.710565160562,-37.9851915354304)) ;
#64131=CARTESIAN_POINT('Ctrl Pts',(28.1311344486129,505.710565160562,-38.0534323638883)) ;
#64132=CARTESIAN_POINT('Ctrl Pts',(28.1562723623073,505.710565160562,-38.1085485325109)) ;
#64133=CARTESIAN_POINT('Ctrl Pts',(28.1839869552626,505.710565160562,-38.1624295731364)) ;
#64134=CARTESIAN_POINT('Ctrl Pts',(28.2142859508539,505.710565160562,-38.2148719443432)) ;
#64135=CARTESIAN_POINT('Ctrl Pts',(28.2202649143704,505.710565160562,-38.2252205060049)) ;
#64136=CARTESIAN_POINT('Ctrl Pts',(28.2263445836864,505.710565160562,-38.2355130233344)) ;
#64137=CARTESIAN_POINT('Ctrl Pts',(28.2325236144401,505.710565160562,-38.2457489606755)) ;
#64138=CARTESIAN_POINT('',(4.83852762540252,505.710565160566,-24.0221601717538)) ;
#64139=CARTESIAN_POINT('Origin',(6.48852762540252,505.710565160566,-24.0221601717538)) ;
#64140=CARTESIAN_POINT('',(36.3885276254024,505.710565160561,-30.2221601717532)) ;
#64141=CARTESIAN_POINT('',(38.3885276254024,505.710565160561,-30.2221601717533)) ;
#64142=CARTESIAN_POINT('',(124.388527625402,505.710565160546,-30.2221601717572)) ;
#64143=CARTESIAN_POINT('',(36.3885276254021,505.710565160561,-37.2221601717532)) ;
#64144=CARTESIAN_POINT('',(36.388527625403,505.710565160561,-18.3721601717532)) ;
#64145=CARTESIAN_POINT('',(38.3885276254021,505.710565160561,-37.2221601717533)) ;
#64146=CARTESIAN_POINT('',(125.388527625402,505.710565160545,-37.2221601717573)) ;
#64147=CARTESIAN_POINT('',(38.3885276254031,505.710565160561,-14.8721601717533)) ;
#64148=CARTESIAN_POINT('',(186.388527625402,505.710565160535,-30.22216017176)) ;
#64149=CARTESIAN_POINT('',(188.388527625402,505.710565160534,-30.2221601717601)) ;
#64150=CARTESIAN_POINT('',(199.388527625402,505.710565160532,-30.2221601717606)) ;
#64151=CARTESIAN_POINT('',(186.388527625402,505.710565160535,-37.22216017176)) ;
#64152=CARTESIAN_POINT('',(186.388527625403,505.710565160535,-18.37216017176)) ;
#64153=CARTESIAN_POINT('',(188.388527625402,505.710565160534,-37.2221601717601)) ;
#64154=CARTESIAN_POINT('',(200.388527625402,505.710565160532,-37.2221601717607)) ;
#64155=CARTESIAN_POINT('',(188.388527625403,505.710565160534,-14.8721601717601)) ;
#64156=CARTESIAN_POINT('',(21.3885276254024,505.710565160564,-30.2221601717525)) ;
#64157=CARTESIAN_POINT('',(23.3885276254024,505.710565160563,-30.2221601717526)) ;
#64158=CARTESIAN_POINT('',(116.888527625402,505.710565160547,-30.2221601717569)) ;
#64159=CARTESIAN_POINT('',(21.3885276254021,505.710565160564,-37.2221601717525)) ;
#64160=CARTESIAN_POINT('',(21.388527625403,505.710565160564,-18.3721601717525)) ;
#64161=CARTESIAN_POINT('',(23.3885276254021,505.710565160563,-37.2221601717526)) ;
#64162=CARTESIAN_POINT('',(117.888527625402,505.710565160547,-37.2221601717569)) ;
#64163=CARTESIAN_POINT('',(23.3885276254031,505.710565160563,-14.8721601717526)) ;
#64164=CARTESIAN_POINT('',(185.73826464091,505.710565160535,-24.0199774237433)) ;
#64165=CARTESIAN_POINT('Origin',(187.388264603403,505.710565160534,-24.0203292412001)) ;
#64166=CARTESIAN_POINT('Origin',(212.388527625421,616.21056516053,-47.0221601717612)) ;
#64167=CARTESIAN_POINT('',(0.388527630194573,616.210565160567,-47.5221601717516)) ;
#64168=CARTESIAN_POINT('',(0.388527634368074,616.710565160567,-47.0221601717516)) ;
#64169=CARTESIAN_POINT('Origin',(0.388527634368039,616.210565160567,-47.0221601717516)) ;
#64170=CARTESIAN_POINT('',(140.388527625421,616.210565160543,-47.5221601717579)) ;
#64171=CARTESIAN_POINT('',(212.388527625421,616.21056516053,-47.5221601717612)) ;
#64172=CARTESIAN_POINT('',(140.388527625421,616.710565160543,-47.022160171758)) ;
#64173=CARTESIAN_POINT('Origin',(140.388527625421,616.210565160543,-47.022160171758)) ;
#64174=CARTESIAN_POINT('',(212.388527625421,616.71056516053,-47.0221601717612)) ;
#64175=CARTESIAN_POINT('Origin',(212.388527625421,616.71056516053,-49.5221601717612)) ;
#64176=CARTESIAN_POINT('',(104.888527625422,616.710565160549,-19.5221601717563)) ;
#64177=CARTESIAN_POINT('',(-2.6114723745787,616.710565160568,-43.4900362557631)) ;
#64178=CARTESIAN_POINT('',(-2.61147237457784,616.710565160568,-24.5221601717514)) ;
#64179=CARTESIAN_POINT('',(0.388527634368074,616.710565160567,-43.4900362557631)) ;
#64180=CARTESIAN_POINT('',(103.388527625431,616.710565160549,-43.4900362557631)) ;
#64181=CARTESIAN_POINT('',(0.388527634368081,616.710565160567,-49.0060982137622)) ;
#64182=CARTESIAN_POINT('',(140.388527625422,616.710565160543,-28.5221601717579)) ;
#64183=CARTESIAN_POINT('',(140.388527625421,616.710565160543,-49.5221601717579)) ;
#64184=CARTESIAN_POINT('',(144.388527625422,616.710565160542,-28.5221601717581)) ;
#64185=CARTESIAN_POINT('Origin',(142.388527625422,616.710565160542,-28.522160171758)) ;
#64186=CARTESIAN_POINT('',(144.388527625421,616.710565160542,-47.0221601717582)) ;
#64187=CARTESIAN_POINT('',(144.388527625422,616.710565160542,-38.0221601717581)) ;
#64188=CARTESIAN_POINT('',(148.388527625421,616.710565160541,-47.0221601717583)) ;
#64189=CARTESIAN_POINT('',(212.388527625421,616.71056516053,-47.0221601717612)) ;
#64190=CARTESIAN_POINT('',(148.388527625422,616.710565160541,-28.5221601717583)) ;
#64191=CARTESIAN_POINT('',(148.388527625421,616.710565160541,-49.5221601717583)) ;
#64192=CARTESIAN_POINT('',(152.388527625422,616.71056516054,-28.5221601717585)) ;
#64193=CARTESIAN_POINT('Origin',(150.388527625422,616.710565160541,-28.5221601717584)) ;
#64194=CARTESIAN_POINT('',(152.388527625421,616.71056516054,-47.0221601717585)) ;
#64195=CARTESIAN_POINT('',(152.388527625422,616.71056516054,-38.0221601717585)) ;
#64196=CARTESIAN_POINT('',(193.688527625421,616.710565160533,-47.0221601717604)) ;
#64197=CARTESIAN_POINT('',(212.388527625421,616.71056516053,-47.0221601717612)) ;
#64198=CARTESIAN_POINT('',(193.688527625422,616.710565160533,-28.5221601717604)) ;
#64199=CARTESIAN_POINT('',(193.688527625421,616.710565160533,-49.5221601717604)) ;
#64200=CARTESIAN_POINT('',(197.688527625422,616.710565160532,-28.5221601717605)) ;
#64201=CARTESIAN_POINT('Origin',(195.688527625422,616.710565160533,-28.5221601717604)) ;
#64202=CARTESIAN_POINT('',(197.688527625421,616.710565160533,-47.0221601717606)) ;
#64203=CARTESIAN_POINT('',(197.688527625421,616.710565160533,-49.5221601717605)) ;
#64204=CARTESIAN_POINT('',(201.668527625421,616.710565160532,-47.0221601717608)) ;
#64205=CARTESIAN_POINT('',(212.388527625421,616.71056516053,-47.0221601717612)) ;
#64206=CARTESIAN_POINT('',(201.668527625422,616.710565160532,-28.5221601717607)) ;
#64207=CARTESIAN_POINT('',(201.668527625421,616.710565160532,-49.5221601717607)) ;
#64208=CARTESIAN_POINT('',(205.668527625422,616.710565160531,-28.5221601717609)) ;
#64209=CARTESIAN_POINT('Origin',(203.668527625422,616.710565160532,-28.5221601717608)) ;
#64210=CARTESIAN_POINT('',(205.668527625421,616.710565160531,-49.5221601717609)) ;
#64211=CARTESIAN_POINT('',(4.83852762542202,616.710565160566,-24.0221601717537)) ;
#64212=CARTESIAN_POINT('Origin',(6.48852762542202,616.710565160566,-24.0221601717538)) ;
#64213=CARTESIAN_POINT('',(21.3885276254216,616.710565160564,-37.2221601717525)) ;
#64214=CARTESIAN_POINT('',(23.3885276254216,616.710565160563,-37.2221601717526)) ;
#64215=CARTESIAN_POINT('',(117.888527625422,616.710565160547,-37.2221601717569)) ;
#64216=CARTESIAN_POINT('',(21.3885276254219,616.710565160564,-30.2221601717525)) ;
#64217=CARTESIAN_POINT('',(21.3885276254213,616.710565160564,-43.3721601717525)) ;
#64218=CARTESIAN_POINT('',(23.3885276254219,616.710565160563,-30.2221601717526)) ;
#64219=CARTESIAN_POINT('',(116.888527625422,616.710565160547,-30.2221601717569)) ;
#64220=CARTESIAN_POINT('',(23.3885276254215,616.710565160563,-39.8721601717526)) ;
#64221=CARTESIAN_POINT('',(186.388527625422,616.710565160535,-37.22216017176)) ;
#64222=CARTESIAN_POINT('',(188.388527625422,616.710565160534,-37.2221601717601)) ;
#64223=CARTESIAN_POINT('',(200.388527625422,616.710565160532,-37.2221601717607)) ;
#64224=CARTESIAN_POINT('',(186.388527625422,616.710565160535,-30.22216017176)) ;
#64225=CARTESIAN_POINT('',(186.388527625421,616.710565160535,-43.37216017176)) ;
#64226=CARTESIAN_POINT('',(188.388527625422,616.710565160534,-30.2221601717601)) ;
#64227=CARTESIAN_POINT('',(199.388527625422,616.710565160532,-30.2221601717606)) ;
#64228=CARTESIAN_POINT('',(188.388527625421,616.710565160534,-39.8721601717601)) ;
#64229=CARTESIAN_POINT('',(171.388527625422,616.710565160537,-37.2221601717593)) ;
#64230=CARTESIAN_POINT('',(173.388527625422,616.710565160537,-37.2221601717594)) ;
#64231=CARTESIAN_POINT('',(192.888527625422,616.710565160533,-37.2221601717603)) ;
#64232=CARTESIAN_POINT('',(171.388527625422,616.710565160537,-30.2221601717593)) ;
#64233=CARTESIAN_POINT('',(171.388527625421,616.710565160537,-43.3721601717593)) ;
#64234=CARTESIAN_POINT('',(173.388527625422,616.710565160537,-30.2221601717594)) ;
#64235=CARTESIAN_POINT('',(191.888527625422,616.710565160534,-30.2221601717603)) ;
#64236=CARTESIAN_POINT('',(173.388527625421,616.710565160537,-39.8721601717594)) ;
#64237=CARTESIAN_POINT('',(36.3885276254216,616.710565160561,-37.2221601717532)) ;
#64238=CARTESIAN_POINT('',(38.3885276254216,616.710565160561,-37.2221601717533)) ;
#64239=CARTESIAN_POINT('',(125.388527625422,616.710565160545,-37.2221601717573)) ;
#64240=CARTESIAN_POINT('',(36.3885276254219,616.710565160561,-30.2221601717532)) ;
#64241=CARTESIAN_POINT('',(36.3885276254213,616.710565160561,-43.3721601717532)) ;
#64242=CARTESIAN_POINT('',(38.3885276254219,616.710565160561,-30.2221601717533)) ;
#64243=CARTESIAN_POINT('',(124.388527625422,616.710565160545,-30.2221601717572)) ;
#64244=CARTESIAN_POINT('',(38.3885276254215,616.710565160561,-39.8721601717533)) ;
#64245=CARTESIAN_POINT('',(187.382265311382,616.710565160534,-25.6703183346474)) ;
#64246=CARTESIAN_POINT('Origin',(187.388264603422,616.710565160534,-24.0203292412001)) ;
#64247=CARTESIAN_POINT('',(31.5554754095649,616.709694579094,-37.0753480170549)) ;
#64248=CARTESIAN_POINT('Ctrl Pts',(29.0652954453167,616.710565160562,-35.1395326620899)) ;
#64249=CARTESIAN_POINT('Ctrl Pts',(29.1351294046756,616.710565160562,-35.1164998682415)) ;
#64250=CARTESIAN_POINT('Ctrl Pts',(29.2060755187498,616.710565160562,-35.097620673558)) ;
#64251=CARTESIAN_POINT('Ctrl Pts',(29.2777966627579,616.710565160562,-35.0827784591697)) ;
#64252=CARTESIAN_POINT('Ctrl Pts',(29.3511765960227,616.710565160562,-35.0675929693622)) ;
#64253=CARTESIAN_POINT('Ctrl Pts',(29.4253688687927,616.710565160562,-35.0566334627366)) ;
#64254=CARTESIAN_POINT('Ctrl Pts',(29.5000158983603,616.710565160562,-35.0498295941094)) ;
#64255=CARTESIAN_POINT('Ctrl Pts',(29.5628148257399,616.710565160562,-35.0441056469638)) ;
#64256=CARTESIAN_POINT('Ctrl Pts',(29.6259359910898,616.710565160562,-35.0413238912052)) ;
#64257=CARTESIAN_POINT('Ctrl Pts',(29.6891600328717,616.710565160562,-35.0414702603465)) ;
#64258=CARTESIAN_POINT('Ctrl Pts',(29.7173612583189,616.710565160562,-35.0415355486299)) ;
#64259=CARTESIAN_POINT('Ctrl Pts',(29.7455828283297,616.710565160562,-35.0421837488871)) ;
#64260=CARTESIAN_POINT('Ctrl Pts',(29.7738045152508,616.710565160562,-35.04341513634)) ;
#64261=CARTESIAN_POINT('Ctrl Pts',(29.7892687576035,616.710565160562,-35.044089882469)) ;
#64262=CARTESIAN_POINT('Ctrl Pts',(29.8047330254023,616.710565160562,-35.0449397499688)) ;
#64263=CARTESIAN_POINT('Ctrl Pts',(29.8201939125384,616.710565160562,-35.0459648986994)) ;
#64264=CARTESIAN_POINT('Ctrl Pts',(29.8345628533837,616.710565160562,-35.0469176448995)) ;
#64265=CARTESIAN_POINT('Ctrl Pts',(29.8489310522879,616.710565160562,-35.0480220901629)) ;
#64266=CARTESIAN_POINT('Ctrl Pts',(29.8632734423503,616.710565160562,-35.0492761421653)) ;
#64267=CARTESIAN_POINT('Ctrl Pts',(29.9362514172939,616.710565160562,-35.0556570992591)) ;
#64268=CARTESIAN_POINT('Ctrl Pts',(30.008687827618,616.710565160562,-35.0659142384965)) ;
#64269=CARTESIAN_POINT('Ctrl Pts',(30.0802481411886,616.710565160562,-35.0799778810538)) ;
#64270=CARTESIAN_POINT('Ctrl Pts',(30.1507148608536,616.710565160562,-35.0938266012187)) ;
#64271=CARTESIAN_POINT('Ctrl Pts',(30.220332959107,616.710565160562,-35.1113668001717)) ;
#64272=CARTESIAN_POINT('Ctrl Pts',(30.2887636507385,616.710565160562,-35.1325775802419)) ;
#64273=CARTESIAN_POINT('Ctrl Pts',(30.346718206272,616.710565160562,-35.1505411767244)) ;
#64274=CARTESIAN_POINT('Ctrl Pts',(30.4038210539397,616.710565160562,-35.1711383711428)) ;
#64275=CARTESIAN_POINT('Ctrl Pts',(30.4598482127828,616.710565160562,-35.1943794772149)) ;
#64276=CARTESIAN_POINT('Ctrl Pts',(30.4829009790285,616.710565160562,-35.2039421928092)) ;
#64277=CARTESIAN_POINT('Ctrl Pts',(30.5057714016489,616.710565160562,-35.2139527496974)) ;
#64278=CARTESIAN_POINT('Ctrl Pts',(30.5284428038845,616.710565160562,-35.224412822659)) ;
#64279=CARTESIAN_POINT('Ctrl Pts',(30.5390186169923,616.710565160562,-35.229292263974)) ;
#64280=CARTESIAN_POINT('Ctrl Pts',(30.5495511123406,616.710565160562,-35.234269530304)) ;
#64281=CARTESIAN_POINT('Ctrl Pts',(30.5600385439176,616.710565160562,-35.2393448310897)) ;
#64282=CARTESIAN_POINT('Ctrl Pts',(30.5708533815617,616.710565160562,-35.244578577178)) ;
#64283=CARTESIAN_POINT('Ctrl Pts',(30.5816126498371,616.710565160562,-35.2499129016229)) ;
#64284=CARTESIAN_POINT('Ctrl Pts',(30.5923111405141,616.710565160562,-35.2553457748175)) ;
#64285=CARTESIAN_POINT('Ctrl Pts',(30.6536613282617,616.710565160562,-35.2865004302325)) ;
#64286=CARTESIAN_POINT('Ctrl Pts',(30.7130542560941,616.710565160562,-35.3209113718768)) ;
#64287=CARTESIAN_POINT('Ctrl Pts',(30.770186000803,616.710565160562,-35.3585552909014)) ;
#64288=CARTESIAN_POINT('Ctrl Pts',(30.8223319344572,616.710565160562,-35.3929140753906)) ;
#64289=CARTESIAN_POINT('Ctrl Pts',(30.8725942861496,616.710565160562,-35.4299668351395)) ;
#64290=CARTESIAN_POINT('Ctrl Pts',(30.9207155073971,616.710565160562,-35.4697230936572)) ;
#64291=CARTESIAN_POINT('Ctrl Pts',(30.977274484471,616.710565160562,-35.5164503639917)) ;
#64292=CARTESIAN_POINT('Ctrl Pts',(31.0308770037112,616.710565160562,-35.5669131889342)) ;
#64293=CARTESIAN_POINT('Ctrl Pts',(31.0813189646559,616.710565160562,-35.6207353285878)) ;
#64294=CARTESIAN_POINT('Ctrl Pts',(31.0925085957903,616.710565160562,-35.6326747908592)) ;
#64295=CARTESIAN_POINT('Ctrl Pts',(31.1035424675763,616.710565160562,-35.6447796390117)) ;
#64296=CARTESIAN_POINT('Ctrl Pts',(31.1144179492562,616.710565160562,-35.6570458691578)) ;
#64297=CARTESIAN_POINT('Ctrl Pts',(31.125064388927,616.710565160562,-35.6690537675742)) ;
#64298=CARTESIAN_POINT('Ctrl Pts',(31.1355623407383,616.710565160562,-35.6812204659215)) ;
#64299=CARTESIAN_POINT('Ctrl Pts',(31.1458894648435,616.710565160562,-35.6935180916591)) ;
#64300=CARTESIAN_POINT('Ctrl Pts',(31.1898516741418,616.710565160562,-35.7458686580936)) ;
#64301=CARTESIAN_POINT('Ctrl Pts',(31.2307855322649,616.710565160562,-35.8006576376647)) ;
#64302=CARTESIAN_POINT('Ctrl Pts',(31.268577106942,616.710565160562,-35.8575501098362)) ;
#64303=CARTESIAN_POINT('Ctrl Pts',(31.3064239741415,616.710565160562,-35.9145258208863)) ;
#64304=CARTESIAN_POINT('Ctrl Pts',(31.3411196762928,616.710565160562,-35.9736122848845)) ;
#64305=CARTESIAN_POINT('Ctrl Pts',(31.3725019056337,616.710565160562,-36.0344921687448)) ;
#64306=CARTESIAN_POINT('Ctrl Pts',(31.3956129454238,616.710565160562,-36.0793263773992)) ;
#64307=CARTESIAN_POINT('Ctrl Pts',(31.4169259867845,616.710565160562,-36.1251336930938)) ;
#64308=CARTESIAN_POINT('Ctrl Pts',(31.4363581232945,616.710565160562,-36.1717887688914)) ;
#64309=CARTESIAN_POINT('Ctrl Pts',(31.4443461212685,616.710565160562,-36.1909673420122)) ;
#64310=CARTESIAN_POINT('Ctrl Pts',(31.4520160980142,616.710565160562,-36.2102891591937)) ;
#64311=CARTESIAN_POINT('Ctrl Pts',(31.4593614982079,616.710565160562,-36.2297454134763)) ;
#64312=CARTESIAN_POINT('Ctrl Pts',(31.4648122432911,616.710565160562,-36.2441831676588)) ;
#64313=CARTESIAN_POINT('Ctrl Pts',(31.4700842485553,616.710565160562,-36.2586949491632)) ;
#64314=CARTESIAN_POINT('Ctrl Pts',(31.4751746647096,616.710565160562,-36.2732771191433)) ;
#64315=CARTESIAN_POINT('Ctrl Pts',(31.4794594741956,616.710565160562,-36.2855515223281)) ;
#64316=CARTESIAN_POINT('Ctrl Pts',(31.4836128170683,616.710565160562,-36.297867844351)) ;
#64317=CARTESIAN_POINT('Ctrl Pts',(31.4876324001455,616.710565160562,-36.3102203290086)) ;
#64318=CARTESIAN_POINT('Ctrl Pts',(31.5080082748776,616.710565160562,-36.3728369425173)) ;
#64319=CARTESIAN_POINT('Ctrl Pts',(31.524961188787,616.710565160562,-36.4364120290553)) ;
#64320=CARTESIAN_POINT('Ctrl Pts',(31.5383233055122,616.710565160562,-36.5006546081721)) ;
#64321=CARTESIAN_POINT('Ctrl Pts',(31.5477840532232,616.710565160562,-36.5461401286044)) ;
#64322=CARTESIAN_POINT('Ctrl Pts',(31.5554437254137,616.710565160562,-36.5919603907947)) ;
#64323=CARTESIAN_POINT('Ctrl Pts',(31.561227196496,616.710565160562,-36.6380096873979)) ;
#64324=CARTESIAN_POINT('Ctrl Pts',(31.5630746651284,616.710565160562,-36.6527196478715)) ;
#64325=CARTESIAN_POINT('Ctrl Pts',(31.5647307999987,616.710565160562,-36.6674551981726)) ;
#64326=CARTESIAN_POINT('Ctrl Pts',(31.5661921596199,616.710565160562,-36.6822055678034)) ;
#64327=CARTESIAN_POINT('Ctrl Pts',(31.5724090354787,616.710565160562,-36.7449561841024)) ;
#64328=CARTESIAN_POINT('Ctrl Pts',(31.5750942763573,616.710565160562,-36.8078591320246)) ;
#64329=CARTESIAN_POINT('Ctrl Pts',(31.574079138145,616.710565160562,-36.8706478918813)) ;
#64330=CARTESIAN_POINT('Ctrl Pts',(31.5731334449241,616.710565160562,-36.9291413106388)) ;
#64331=CARTESIAN_POINT('Ctrl Pts',(31.5689759954375,616.710565160562,-36.9875361088946)) ;
#64332=CARTESIAN_POINT('Ctrl Pts',(31.5614316605456,616.710565160562,-37.0456039639648)) ;
#64333=CARTESIAN_POINT('Ctrl Pts',(31.5601435095963,616.710565160562,-37.0555187097575)) ;
#64334=CARTESIAN_POINT('Ctrl Pts',(31.5587565273789,616.710565160562,-37.0654238825553)) ;
#64335=CARTESIAN_POINT('Ctrl Pts',(31.5572713557558,616.710565160562,-37.0753183083685)) ;
#64336=CARTESIAN_POINT('Ctrl Pts',(31.5536802139309,616.709694579094,-37.0752907371637)) ;
#64337=CARTESIAN_POINT('Ctrl Pts',(31.5534371170828,616.709984772917,-37.0829095784596)) ;
#64338=CARTESIAN_POINT('Ctrl Pts',(31.5531417298432,616.710274966739,-37.0905267513044)) ;
#64339=CARTESIAN_POINT('Ctrl Pts',(31.5527940800387,616.710565160562,-37.0981415381289)) ;
#64340=CARTESIAN_POINT('Ctrl Pts',(29.5692971707939,616.710565160562,-38.6572894990043)) ;
#64341=CARTESIAN_POINT('Ctrl Pts',(29.5054553546424,616.710565160562,-38.6523321037633)) ;
#64342=CARTESIAN_POINT('Ctrl Pts',(29.4421828366268,616.710565160562,-38.6433990979037)) ;
#64343=CARTESIAN_POINT('Ctrl Pts',(29.3797148829646,616.710565160562,-38.6307914294923)) ;
#64344=CARTESIAN_POINT('Ctrl Pts',(29.3172469293023,616.710565160562,-38.6181837610809)) ;
#64345=CARTESIAN_POINT('Ctrl Pts',(29.2555827598154,616.710565160562,-38.601901087878)) ;
#64346=CARTESIAN_POINT('Ctrl Pts',(29.1949472804358,616.710565160562,-38.5821888640866)) ;
#64347=CARTESIAN_POINT('Ctrl Pts',(29.1329194349116,616.710565160562,-38.5620239905707)) ;
#64348=CARTESIAN_POINT('Ctrl Pts',(29.071967191479,616.710565160562,-38.5382700716443)) ;
#64349=CARTESIAN_POINT('Ctrl Pts',(29.0123330057214,616.710565160562,-38.5111354809055)) ;
#64350=CARTESIAN_POINT('Ctrl Pts',(28.9927857260204,616.710565160562,-38.5022411289829)) ;
#64351=CARTESIAN_POINT('Ctrl Pts',(28.9733801346285,616.710565160562,-38.4929831301336)) ;
#64352=CARTESIAN_POINT('Ctrl Pts',(28.9541250633592,616.710565160562,-38.4833676492202)) ;
#64353=CARTESIAN_POINT('Ctrl Pts',(28.9423245452005,616.710565160562,-38.4774747779067)) ;
#64354=CARTESIAN_POINT('Ctrl Pts',(28.9305792368964,616.710565160562,-38.4714467930994)) ;
#64355=CARTESIAN_POINT('Ctrl Pts',(28.9189098346057,616.710565160562,-38.4652952396331)) ;
#64356=CARTESIAN_POINT('Ctrl Pts',(28.8596160434162,616.710565160562,-38.4340383750884)) ;
#64357=CARTESIAN_POINT('Ctrl Pts',(28.8021715482124,616.710565160562,-38.3995418155636)) ;
#64358=CARTESIAN_POINT('Ctrl Pts',(28.7468176421506,616.710565160562,-38.3620742445524)) ;
#64359=CARTESIAN_POINT('Ctrl Pts',(28.6903533001159,616.710565160562,-38.3238550492814)) ;
#64360=CARTESIAN_POINT('Ctrl Pts',(28.6360632941515,616.710565160562,-38.2825441451409)) ;
#64361=CARTESIAN_POINT('Ctrl Pts',(28.5842118032974,616.710565160562,-38.2383730315202)) ;
#64362=CARTESIAN_POINT('Ctrl Pts',(28.5410521825941,616.710565160562,-38.2016063257127)) ;
#64363=CARTESIAN_POINT('Ctrl Pts',(28.4995819204966,616.710565160562,-38.162856848819)) ;
#64364=CARTESIAN_POINT('Ctrl Pts',(28.4599650517436,616.710565160562,-38.1222331755884)) ;
#64365=CARTESIAN_POINT('Ctrl Pts',(28.4415739837682,616.710565160562,-38.1033747256578)) ;
#64366=CARTESIAN_POINT('Ctrl Pts',(28.4235825196302,616.710565160562,-38.084112082613)) ;
#64367=CARTESIAN_POINT('Ctrl Pts',(28.4060082484722,616.710565160562,-38.0644546500545)) ;
#64368=CARTESIAN_POINT('Ctrl Pts',(28.3984388547211,616.710565160562,-38.0559880202961)) ;
#64369=CARTESIAN_POINT('Ctrl Pts',(28.3909473261853,616.710565160562,-38.0474485305842)) ;
#64370=CARTESIAN_POINT('Ctrl Pts',(28.3835437024959,616.710565160562,-38.0388472958062)) ;
#64371=CARTESIAN_POINT('Ctrl Pts',(28.3377233367417,616.710565160562,-37.9856150219903)) ;
#64372=CARTESIAN_POINT('Ctrl Pts',(28.2951791805688,616.710565160562,-37.9299229619158)) ;
#64373=CARTESIAN_POINT('Ctrl Pts',(28.2561786153644,616.710565160562,-37.872022688255)) ;
#64374=CARTESIAN_POINT('Ctrl Pts',(28.2211117359888,616.710565160562,-37.8199623680613)) ;
#64375=CARTESIAN_POINT('Ctrl Pts',(28.1889093151112,616.710565160562,-37.7661158567172)) ;
#64376=CARTESIAN_POINT('Ctrl Pts',(28.1597844471134,616.710565160562,-37.710635294839)) ;
#64377=CARTESIAN_POINT('Ctrl Pts',(28.1281437015729,616.710565160562,-37.6503621859286)) ;
#64378=CARTESIAN_POINT('Ctrl Pts',(28.1001337962876,616.710565160562,-37.5881605235266)) ;
#64379=CARTESIAN_POINT('Ctrl Pts',(28.0756957976418,616.710565160562,-37.5243505776644)) ;
#64380=CARTESIAN_POINT('Ctrl Pts',(28.0664447763215,616.710565160562,-37.5001952784449)) ;
#64381=CARTESIAN_POINT('Ctrl Pts',(28.0577060649063,616.710565160562,-37.4758092124162)) ;
#64382=CARTESIAN_POINT('Ctrl Pts',(28.0494781473923,616.710565160562,-37.4512088109423)) ;
#64383=CARTESIAN_POINT('Ctrl Pts',(28.0458324122321,616.710565160562,-37.4403085377617)) ;
#64384=CARTESIAN_POINT('Ctrl Pts',(28.0422873762234,616.710565160562,-37.4293671270742)) ;
#64385=CARTESIAN_POINT('Ctrl Pts',(28.0388465277051,616.710565160562,-37.418398332039)) ;
#64386=CARTESIAN_POINT('Ctrl Pts',(28.018086867898,616.710565160562,-37.3522203377988)) ;
#64387=CARTESIAN_POINT('Ctrl Pts',(28.001076777631,616.710565160562,-37.2849317662674)) ;
#64388=CARTESIAN_POINT('Ctrl Pts',(27.987710553931,616.710565160562,-37.2168874703652)) ;
#64389=CARTESIAN_POINT('Ctrl Pts',(27.9739057996822,616.710565160562,-37.1466107187521)) ;
#64390=CARTESIAN_POINT('Ctrl Pts',(27.9639875930527,616.710565160562,-37.0755270717528)) ;
#64391=CARTESIAN_POINT('Ctrl Pts',(27.9578856891573,616.710565160562,-37.0039955050982)) ;
#64392=CARTESIAN_POINT('Ctrl Pts',(27.9532315299756,616.710565160562,-36.9494355999537)) ;
#64393=CARTESIAN_POINT('Ctrl Pts',(27.9507985212582,616.710565160562,-36.894614327456)) ;
#64394=CARTESIAN_POINT('Ctrl Pts',(27.950574430833,616.710565160562,-36.8396836324218)) ;
#64395=CARTESIAN_POINT('Ctrl Pts',(27.9504369704838,616.710565160562,-36.8059883394654)) ;
#64396=CARTESIAN_POINT('Ctrl Pts',(27.9511309993669,616.710565160562,-36.7722517715414)) ;
#64397=CARTESIAN_POINT('Ctrl Pts',(27.9526568263021,616.710565160562,-36.7385085318701)) ;
#64398=CARTESIAN_POINT('Ctrl Pts',(27.9532401980609,616.710565160562,-36.7256074271509)) ;
#64399=CARTESIAN_POINT('Ctrl Pts',(27.9539453351246,616.710565160562,-36.7127030614827)) ;
#64400=CARTESIAN_POINT('Ctrl Pts',(27.9547718594983,616.710565160562,-36.6998048208729)) ;
#64401=CARTESIAN_POINT('Ctrl Pts',(27.9595493423161,616.710565160562,-36.6252503069937)) ;
#64402=CARTESIAN_POINT('Ctrl Pts',(27.96836558868,616.710565160562,-36.5510772905987)) ;
#64403=CARTESIAN_POINT('Ctrl Pts',(27.9811572181665,616.710565160562,-36.4776677315349)) ;
#64404=CARTESIAN_POINT('Ctrl Pts',(27.9913560767737,616.710565160562,-36.4191377597205)) ;
#64405=CARTESIAN_POINT('Ctrl Pts',(28.0040830323133,616.710565160563,-36.3610924409845)) ;
#64406=CARTESIAN_POINT('Ctrl Pts',(28.0193293617847,616.710565160563,-36.3037215267236)) ;
#64407=CARTESIAN_POINT('Ctrl Pts',(28.0245563318108,616.710565160563,-36.2840527894203)) ;
#64408=CARTESIAN_POINT('Ctrl Pts',(28.0300795996869,616.710565160562,-36.2644633173544)) ;
#64409=CARTESIAN_POINT('Ctrl Pts',(28.0358993862355,616.710565160562,-36.244960793289)) ;
#64410=CARTESIAN_POINT('Ctrl Pts',(28.0403069622081,616.710565160562,-36.2301906886194)) ;
#64411=CARTESIAN_POINT('Ctrl Pts',(28.0448832231379,616.710565160563,-36.2154753485809)) ;
#64412=CARTESIAN_POINT('Ctrl Pts',(28.049625372632,616.710565160563,-36.2008256626758)) ;
#64413=CARTESIAN_POINT('Ctrl Pts',(28.0728186318987,616.710565160563,-36.1291758836473)) ;
#64414=CARTESIAN_POINT('Ctrl Pts',(28.0999924465964,616.710565160563,-36.0590410222514)) ;
#64415=CARTESIAN_POINT('Ctrl Pts',(28.1311148021221,616.710565160563,-35.9908000485429)) ;
#64416=CARTESIAN_POINT('Ctrl Pts',(28.1562581569131,616.710565160563,-35.9356690347023)) ;
#64417=CARTESIAN_POINT('Ctrl Pts',(28.1839795933006,616.710565160563,-35.8817737322274)) ;
#64418=CARTESIAN_POINT('Ctrl Pts',(28.2142868426508,616.710565160563,-35.8293178017528)) ;
#64419=CARTESIAN_POINT('Ctrl Pts',(28.2202628586927,616.710565160563,-35.8189744849317)) ;
#64420=CARTESIAN_POINT('Ctrl Pts',(28.2263394813903,616.710565160563,-35.8086871540485)) ;
#64421=CARTESIAN_POINT('Ctrl Pts',(28.2325153683705,616.710565160563,-35.7984563440547)) ;
#64422=CARTESIAN_POINT('',(181.555506994667,616.709677724475,-37.0754500573667)) ;
#64423=CARTESIAN_POINT('Ctrl Pts',(179.065295445318,616.710565160536,-35.1395326620961)) ;
#64424=CARTESIAN_POINT('Ctrl Pts',(179.135760309488,616.710565160536,-35.1162917818011)) ;
#64425=CARTESIAN_POINT('Ctrl Pts',(179.207358091158,616.710565160536,-35.097280708745)) ;
#64426=CARTESIAN_POINT('Ctrl Pts',(179.279742381724,616.710565160536,-35.082379713154)) ;
#64427=CARTESIAN_POINT('Ctrl Pts',(179.35212667229,616.710565160536,-35.067478717563)) ;
#64428=CARTESIAN_POINT('Ctrl Pts',(179.42529849312,616.710565160536,-35.05668810083)) ;
#64429=CARTESIAN_POINT('Ctrl Pts',(179.49891473763,616.710565160536,-35.0499403314768)) ;
#64430=CARTESIAN_POINT('Ctrl Pts',(179.573357338759,616.710565160536,-35.0431168171042)) ;
#64431=CARTESIAN_POINT('Ctrl Pts',(179.648255450353,616.710565160536,-35.0404276243099)) ;
#64432=CARTESIAN_POINT('Ctrl Pts',(179.723241986661,616.710565160536,-35.0418526440978)) ;
#64433=CARTESIAN_POINT('Ctrl Pts',(179.740096938686,616.710565160536,-35.0421729501333)) ;
#64434=CARTESIAN_POINT('Ctrl Pts',(179.756956273047,616.710565160536,-35.0427013079803)) ;
#64435=CARTESIAN_POINT('Ctrl Pts',(179.773815652038,616.710565160536,-35.0434378135935)) ;
#64436=CARTESIAN_POINT('Ctrl Pts',(179.789278957467,616.710565160536,-35.0441133314317)) ;
#64437=CARTESIAN_POINT('Ctrl Pts',(179.804742299989,616.710565160536,-35.0449639535352)) ;
#64438=CARTESIAN_POINT('Ctrl Pts',(179.820202273595,616.710565160536,-35.0459898383144)) ;
#64439=CARTESIAN_POINT('Ctrl Pts',(179.83457385404,616.710565160536,-35.046943500074)) ;
#64440=CARTESIAN_POINT('Ctrl Pts',(179.848944705152,616.710565160536,-35.0480489188537)) ;
#64441=CARTESIAN_POINT('Ctrl Pts',(179.863289748568,616.710565160536,-35.0493039991915)) ;
#64442=CARTESIAN_POINT('Ctrl Pts',(179.936267392455,616.710565160536,-35.0556889785383)) ;
#64443=CARTESIAN_POINT('Ctrl Pts',(180.008703721566,616.710565160536,-35.0659500945493)) ;
#64444=CARTESIAN_POINT('Ctrl Pts',(180.080264148198,616.710565160536,-35.0800175215934)) ;
#64445=CARTESIAN_POINT('Ctrl Pts',(180.151287993452,616.710565160536,-35.0939794668824)) ;
#64446=CARTESIAN_POINT('Ctrl Pts',(180.221449976707,616.710565160536,-35.1116912348591)) ;
#64447=CARTESIAN_POINT('Ctrl Pts',(180.290403053554,616.710565160536,-35.1331314491422)) ;
#64448=CARTESIAN_POINT('Ctrl Pts',(180.347810086237,616.710565160536,-35.1509815457351)) ;
#64449=CARTESIAN_POINT('Ctrl Pts',(180.404379083585,616.710565160536,-35.1714168999107)) ;
#64450=CARTESIAN_POINT('Ctrl Pts',(180.459892061383,616.710565160536,-35.1944475435978)) ;
#64451=CARTESIAN_POINT('Ctrl Pts',(180.482945306168,616.710565160536,-35.2040116327092)) ;
#64452=CARTESIAN_POINT('Ctrl Pts',(180.505816207519,616.710565160536,-35.2140235218046)) ;
#64453=CARTESIAN_POINT('Ctrl Pts',(180.528488085772,616.710565160536,-35.2244848788825)) ;
#64454=CARTESIAN_POINT('Ctrl Pts',(180.539061091979,616.710565160536,-35.229363521582)) ;
#64455=CARTESIAN_POINT('Ctrl Pts',(180.549590804644,616.710565160536,-35.2343399228102)) ;
#64456=CARTESIAN_POINT('Ctrl Pts',(180.560075478962,616.710565160536,-35.2394142911207)) ;
#64457=CARTESIAN_POINT('Ctrl Pts',(180.570894238498,616.710565160536,-35.2446503498554)) ;
#64458=CARTESIAN_POINT('Ctrl Pts',(180.581657404697,616.710565160536,-35.2499870499363)) ;
#64459=CARTESIAN_POINT('Ctrl Pts',(180.59235974437,616.710565160536,-35.2554223495306)) ;
#64460=CARTESIAN_POINT('Ctrl Pts',(180.653713401841,616.710565160536,-35.2865814717173)) ;
#64461=CARTESIAN_POINT('Ctrl Pts',(180.713109614463,616.710565160536,-35.3209966878714)) ;
#64462=CARTESIAN_POINT('Ctrl Pts',(180.770244363422,616.710565160536,-35.358644552309)) ;
#64463=CARTESIAN_POINT('Ctrl Pts',(180.822393082669,616.710565160536,-35.3930069665766)) ;
#64464=CARTESIAN_POINT('Ctrl Pts',(180.872657983207,616.710565160536,-35.4300630865994)) ;
#64465=CARTESIAN_POINT('Ctrl Pts',(180.920781439408,616.710565160535,-35.4698223282051)) ;
#64466=CARTESIAN_POINT('Ctrl Pts',(180.977342516551,616.710565160535,-35.5165526694802)) ;
#64467=CARTESIAN_POINT('Ctrl Pts',(181.030946757108,616.710565160536,-35.5670179744961)) ;
#64468=CARTESIAN_POINT('Ctrl Pts',(181.081390104837,616.710565160535,-35.6208420838424)) ;
#64469=CARTESIAN_POINT('Ctrl Pts',(181.092579707588,616.710565160535,-35.6327816245176)) ;
#64470=CARTESIAN_POINT('Ctrl Pts',(181.103613543871,616.710565160535,-35.6448865160113)) ;
#64471=CARTESIAN_POINT('Ctrl Pts',(181.114488983632,616.710565160535,-35.6571527556512)) ;
#64472=CARTESIAN_POINT('Ctrl Pts',(181.125135943949,616.710565160535,-35.6691612968745)) ;
#64473=CARTESIAN_POINT('Ctrl Pts',(181.135634394718,616.710565160535,-35.6813286224832)) ;
#64474=CARTESIAN_POINT('Ctrl Pts',(181.145961995009,616.710565160535,-35.6936268588133)) ;
#64475=CARTESIAN_POINT('Ctrl Pts',(181.190055697178,616.710565160536,-35.7461341939821)) ;
#64476=CARTESIAN_POINT('Ctrl Pts',(181.23110279425,616.710565160536,-35.8010940082152)) ;
#64477=CARTESIAN_POINT('Ctrl Pts',(181.268988309028,616.710565160536,-35.8581685016228)) ;
#64478=CARTESIAN_POINT('Ctrl Pts',(181.306869165289,616.710565160535,-35.9152359769777)) ;
#64479=CARTESIAN_POINT('Ctrl Pts',(181.341589526853,616.710565160535,-35.9744187271591)) ;
#64480=CARTESIAN_POINT('Ctrl Pts',(181.372986267054,616.710565160536,-36.0353982117686)) ;
#64481=CARTESIAN_POINT('Ctrl Pts',(181.39593969148,616.710565160536,-36.0799788906067)) ;
#64482=CARTESIAN_POINT('Ctrl Pts',(181.41711574832,616.710565160536,-36.12552033319)) ;
#64483=CARTESIAN_POINT('Ctrl Pts',(181.436432961007,616.710565160536,-36.1718994265542)) ;
#64484=CARTESIAN_POINT('Ctrl Pts',(181.444420861294,616.710565160536,-36.1910777406913)) ;
#64485=CARTESIAN_POINT('Ctrl Pts',(181.452090730016,616.710565160535,-36.21039927642)) ;
#64486=CARTESIAN_POINT('Ctrl Pts',(181.459436013036,616.710565160535,-36.2298552288666)) ;
#64487=CARTESIAN_POINT('Ctrl Pts',(181.464888066979,616.710565160535,-36.2442964562457)) ;
#64488=CARTESIAN_POINT('Ctrl Pts',(181.470161284513,616.710565160535,-36.2588117376376)) ;
#64489=CARTESIAN_POINT('Ctrl Pts',(181.475252814629,616.710565160535,-36.2733974322528)) ;
#64490=CARTESIAN_POINT('Ctrl Pts',(181.479536714035,616.710565160535,-36.2856695090322)) ;
#64491=CARTESIAN_POINT('Ctrl Pts',(181.483689186601,616.710565160535,-36.2979834742669)) ;
#64492=CARTESIAN_POINT('Ctrl Pts',(181.487707944483,616.710565160535,-36.3103335862059)) ;
#64493=CARTESIAN_POINT('Ctrl Pts',(181.508083347335,616.710565160536,-36.3729495768764)) ;
#64494=CARTESIAN_POINT('Ctrl Pts',(181.525035664371,616.710565160536,-36.4365238783295)) ;
#64495=CARTESIAN_POINT('Ctrl Pts',(181.538397094034,616.710565160536,-36.5007655742198)) ;
#64496=CARTESIAN_POINT('Ctrl Pts',(181.547857457299,616.710565160535,-36.5462509597779)) ;
#64497=CARTESIAN_POINT('Ctrl Pts',(181.555516660982,616.710565160535,-36.5920710450797)) ;
#64498=CARTESIAN_POINT('Ctrl Pts',(181.56129958931,616.710565160536,-36.6381201422034)) ;
#64499=CARTESIAN_POINT('Ctrl Pts',(181.563146895243,616.710565160536,-36.6528301239732)) ;
#64500=CARTESIAN_POINT('Ctrl Pts',(181.564802857695,616.710565160536,-36.6675656946417)) ;
#64501=CARTESIAN_POINT('Ctrl Pts',(181.566264035161,616.710565160536,-36.6823160803653)) ;
#64502=CARTESIAN_POINT('Ctrl Pts',(181.572480068538,616.710565160535,-36.7450660830706)) ;
#64503=CARTESIAN_POINT('Ctrl Pts',(181.575164374536,616.710565160536,-36.807968384507)) ;
#64504=CARTESIAN_POINT('Ctrl Pts',(181.574148237453,616.710565160536,-36.8707565192832)) ;
#64505=CARTESIAN_POINT('Ctrl Pts',(181.573201640889,616.710565160536,-36.9292476752771)) ;
#64506=CARTESIAN_POINT('Ctrl Pts',(181.569043416825,616.710565160536,-36.9876402348526)) ;
#64507=CARTESIAN_POINT('Ctrl Pts',(181.56149847437,616.710565160536,-37.0457059401061)) ;
#64508=CARTESIAN_POINT('Ctrl Pts',(181.56021018879,616.710565160535,-37.0556205565811)) ;
#64509=CARTESIAN_POINT('Ctrl Pts',(181.558823072082,616.710565160535,-37.065525602202)) ;
#64510=CARTESIAN_POINT('Ctrl Pts',(181.557337766069,616.710565160536,-37.0754199028953)) ;
#64511=CARTESIAN_POINT('Ctrl Pts',(181.553676994016,616.709677724475,-37.0753915560276)) ;
#64512=CARTESIAN_POINT('Ctrl Pts',(181.553428681374,616.709973536495,-37.0831591097797)) ;
#64513=CARTESIAN_POINT('Ctrl Pts',(181.553126016963,616.710269348516,-37.0909249260131)) ;
#64514=CARTESIAN_POINT('Ctrl Pts',(181.55276903042,616.710565160536,-37.0986882443158)) ;
#64515=CARTESIAN_POINT('Ctrl Pts',(179.569297170793,616.710565160536,-38.6572894990112)) ;
#64516=CARTESIAN_POINT('Ctrl Pts',(179.507575048679,616.710565160536,-38.652496700609)) ;
#64517=CARTESIAN_POINT('Ctrl Pts',(179.446384992941,616.710565160536,-38.6439866958335)) ;
#64518=CARTESIAN_POINT('Ctrl Pts',(179.385939827787,616.710565160536,-38.6320324698614)) ;
#64519=CARTESIAN_POINT('Ctrl Pts',(179.321346845425,616.710565160536,-38.6192579310643)) ;
#64520=CARTESIAN_POINT('Ctrl Pts',(179.257603783352,616.710565160536,-38.6025505502925)) ;
#64521=CARTESIAN_POINT('Ctrl Pts',(179.194958758116,616.710565160536,-38.5821821676965)) ;
#64522=CARTESIAN_POINT('Ctrl Pts',(179.132933456879,616.710565160536,-38.5620152819549)) ;
#64523=CARTESIAN_POINT('Ctrl Pts',(179.071983667288,616.710565160536,-38.5382589733736)) ;
#64524=CARTESIAN_POINT('Ctrl Pts',(179.012351808975,616.710565160536,-38.5111217596247)) ;
#64525=CARTESIAN_POINT('Ctrl Pts',(178.99280394022,616.710565160536,-38.5022259326666)) ;
#64526=CARTESIAN_POINT('Ctrl Pts',(178.97339776577,616.710565160536,-38.4929663833965)) ;
#64527=CARTESIAN_POINT('Ctrl Pts',(178.954142117937,616.710565160536,-38.4833492830115)) ;
#64528=CARTESIAN_POINT('Ctrl Pts',(178.942337688862,616.710565160536,-38.4774536423981)) ;
#64529=CARTESIAN_POINT('Ctrl Pts',(178.930588497952,616.710565160536,-38.4714227769235)) ;
#64530=CARTESIAN_POINT('Ctrl Pts',(178.918915261483,616.710565160536,-38.4652682451263)) ;
#64531=CARTESIAN_POINT('Ctrl Pts',(178.859687972246,616.710565160536,-38.4340415809661)) ;
#64532=CARTESIAN_POINT('Ctrl Pts',(178.802305834108,616.710565160536,-38.3995820670162)) ;
#64533=CARTESIAN_POINT('Ctrl Pts',(178.747009323128,616.710565160536,-38.3621576925695)) ;
#64534=CARTESIAN_POINT('Ctrl Pts',(178.690706061567,616.710565160536,-38.3240519548677)) ;
#64535=CARTESIAN_POINT('Ctrl Pts',(178.6365641045,616.710565160536,-38.2828721018293)) ;
#64536=CARTESIAN_POINT('Ctrl Pts',(178.58484526323,616.710565160536,-38.2388479055619)) ;
#64537=CARTESIAN_POINT('Ctrl Pts',(178.541462842338,616.710565160536,-38.2019198506213)) ;
#64538=CARTESIAN_POINT('Ctrl Pts',(178.499785181819,616.710565160536,-38.1629894148874)) ;
#64539=CARTESIAN_POINT('Ctrl Pts',(178.459978643299,616.710565160536,-38.1221668939241)) ;
#64540=CARTESIAN_POINT('Ctrl Pts',(178.441589914141,616.710565160536,-38.1033088291572)) ;
#64541=CARTESIAN_POINT('Ctrl Pts',(178.4236006766,616.710565160536,-38.0840466916977)) ;
#64542=CARTESIAN_POINT('Ctrl Pts',(178.406028512192,616.710565160536,-38.0643898917392)) ;
#64543=CARTESIAN_POINT('Ctrl Pts',(178.398456975362,616.710565160536,-38.0559201220854)) ;
#64544=CARTESIAN_POINT('Ctrl Pts',(178.390963333105,616.710565160536,-38.0473774447142)) ;
#64545=CARTESIAN_POINT('Ctrl Pts',(178.383557642961,616.710565160536,-38.0387729957834)) ;
#64546=CARTESIAN_POINT('Ctrl Pts',(178.337737205006,616.710565160536,-37.9855356052508)) ;
#64547=CARTESIAN_POINT('Ctrl Pts',(178.295192883898,616.710565160536,-37.9298386851746)) ;
#64548=CARTESIAN_POINT('Ctrl Pts',(178.256192046795,616.710565160536,-37.8719339906431)) ;
#64549=CARTESIAN_POINT('Ctrl Pts',(178.221120823221,616.710565160536,-37.8198636086029)) ;
#64550=CARTESIAN_POINT('Ctrl Pts',(178.188914641014,616.710565160536,-37.7660069730285)) ;
#64551=CARTESIAN_POINT('Ctrl Pts',(178.159786658629,616.710565160536,-37.7105164081319)) ;
#64552=CARTESIAN_POINT('Ctrl Pts',(178.128218081803,616.710565160536,-37.6503763634864)) ;
#64553=CARTESIAN_POINT('Ctrl Pts',(178.100263805153,616.710565160536,-37.5883170941831)) ;
#64554=CARTESIAN_POINT('Ctrl Pts',(178.075865254137,616.710565160536,-37.5246566438292)) ;
#64555=CARTESIAN_POINT('Ctrl Pts',(178.066552311063,616.710565160536,-37.5003574077897)) ;
#64556=CARTESIAN_POINT('Ctrl Pts',(178.057757876326,616.710565160536,-37.4758245865156)) ;
#64557=CARTESIAN_POINT('Ctrl Pts',(178.049480403893,616.710565160536,-37.4510749075307)) ;
#64558=CARTESIAN_POINT('Ctrl Pts',(178.045834737263,616.710565160536,-37.4401743482714)) ;
#64559=CARTESIAN_POINT('Ctrl Pts',(178.042289765575,616.710565160536,-37.4292326659532)) ;
#64560=CARTESIAN_POINT('Ctrl Pts',(178.038848977129,616.710565160536,-37.4182636134829)) ;
#64561=CARTESIAN_POINT('Ctrl Pts',(178.017905664152,616.710565160536,-37.3514974339986)) ;
#64562=CARTESIAN_POINT('Ctrl Pts',(178.00077847231,616.710565160536,-37.2836014755171)) ;
#64563=CARTESIAN_POINT('Ctrl Pts',(177.987359061536,616.710565160536,-37.2149398559529)) ;
#64564=CARTESIAN_POINT('Ctrl Pts',(177.973632227832,616.710565160536,-37.1447052793803)) ;
#64565=CARTESIAN_POINT('Ctrl Pts',(177.96378473025,616.710565160536,-37.0736687309019)) ;
#64566=CARTESIAN_POINT('Ctrl Pts',(177.95774689361,616.710565160536,-37.0021880127456)) ;
#64567=CARTESIAN_POINT('Ctrl Pts',(177.95318461716,616.710565160536,-36.9481761511335)) ;
#64568=CARTESIAN_POINT('Ctrl Pts',(177.950798421621,616.710565160536,-36.8939099228487)) ;
#64569=CARTESIAN_POINT('Ctrl Pts',(177.95057652878,616.710565160536,-36.8395366347886)) ;
#64570=CARTESIAN_POINT('Ctrl Pts',(177.950439026467,616.710565160536,-36.8058426551063)) ;
#64571=CARTESIAN_POINT('Ctrl Pts',(177.951132932983,616.710565160536,-36.7721074653787)) ;
#64572=CARTESIAN_POINT('Ctrl Pts',(177.952658557802,616.710565160536,-36.7383656561305)) ;
#64573=CARTESIAN_POINT('Ctrl Pts',(177.953241924976,616.710565160536,-36.7254634906293)) ;
#64574=CARTESIAN_POINT('Ctrl Pts',(177.953947076004,616.710565160536,-36.7125580728955)) ;
#64575=CARTESIAN_POINT('Ctrl Pts',(177.95477363332,616.710565160536,-36.6996587838914)) ;
#64576=CARTESIAN_POINT('Ctrl Pts',(177.959680119899,616.710565160536,-36.6230879433847)) ;
#64577=CARTESIAN_POINT('Ctrl Pts',(177.96884650041,616.710565160536,-36.5469198339896)) ;
#64578=CARTESIAN_POINT('Ctrl Pts',(177.982204867157,616.710565160536,-36.4715679483824)) ;
#64579=CARTESIAN_POINT('Ctrl Pts',(177.992223642217,616.710565160536,-36.4150540341769)) ;
#64580=CARTESIAN_POINT('Ctrl Pts',(178.004601543926,616.710565160536,-36.3589985786665)) ;
#64581=CARTESIAN_POINT('Ctrl Pts',(178.01933103088,616.710565160536,-36.3035726335972)) ;
#64582=CARTESIAN_POINT('Ctrl Pts',(178.024555445297,616.710565160536,-36.2839135573912)) ;
#64583=CARTESIAN_POINT('Ctrl Pts',(178.030075870223,616.710565160536,-36.2643336763624)) ;
#64584=CARTESIAN_POINT('Ctrl Pts',(178.035892526252,616.710565160536,-36.2448406603716)) ;
#64585=CARTESIAN_POINT('Ctrl Pts',(178.040298354069,616.710565160536,-36.2300756696835)) ;
#64586=CARTESIAN_POINT('Ctrl Pts',(178.044872758394,616.710565160536,-36.215365382693)) ;
#64587=CARTESIAN_POINT('Ctrl Pts',(178.049612935484,616.710565160536,-36.2007207121868)) ;
#64588=CARTESIAN_POINT('Ctrl Pts',(178.072804589896,616.710565160536,-36.1290706174879)) ;
#64589=CARTESIAN_POINT('Ctrl Pts',(178.099976840661,616.710565160536,-36.0589354223635)) ;
#64590=CARTESIAN_POINT('Ctrl Pts',(178.131097670835,616.710565160536,-35.9906940138396)) ;
#64591=CARTESIAN_POINT('Ctrl Pts',(178.156246568811,616.710565160536,-35.9355477914836)) ;
#64592=CARTESIAN_POINT('Ctrl Pts',(178.183974962278,616.710565160536,-35.8816378803032)) ;
#64593=CARTESIAN_POINT('Ctrl Pts',(178.21429059059,616.710565160536,-35.8291680617348)) ;
#64594=CARTESIAN_POINT('Ctrl Pts',(178.220263208248,616.710565160536,-35.8188307478686)) ;
#64595=CARTESIAN_POINT('Ctrl Pts',(178.226336317829,616.710565160493,-35.8085493533407)) ;
#64596=CARTESIAN_POINT('Ctrl Pts',(178.232508579458,616.710565160534,-35.798324412355)) ;
#64597=CARTESIAN_POINT('',(87.3885276254219,616.710565160552,-31.1471601717549)) ;
#64598=CARTESIAN_POINT('',(87.3885276254219,616.710565160552,-39.8971601717549)) ;
#64599=CARTESIAN_POINT('',(87.3885276254219,616.710565160552,-44.7721601717581)) ;
#64600=CARTESIAN_POINT('',(87.2635276254219,616.710565160552,-40.0221601717549)) ;
#64601=CARTESIAN_POINT('Origin',(87.2635276254219,616.710565160552,-39.8971601717549)) ;
#64602=CARTESIAN_POINT('',(73.5135276254219,616.710565160554,-40.0221601717549)) ;
#64603=CARTESIAN_POINT('',(142.888527625421,616.710565160542,-40.0221601717549)) ;
#64604=CARTESIAN_POINT('',(73.3885276254219,616.710565160554,-39.8971601717549)) ;
#64605=CARTESIAN_POINT('Origin',(73.5135276254219,616.710565160555,-39.8971601717549)) ;
#64606=CARTESIAN_POINT('',(73.3885276254219,616.710565160554,-31.1471601717549)) ;
#64607=CARTESIAN_POINT('',(73.3885276254219,616.710565160554,-40.272160171758)) ;
#64608=CARTESIAN_POINT('',(73.5135276254219,616.710565160554,-31.0221601717549)) ;
#64609=CARTESIAN_POINT('Origin',(73.5135276254219,616.710565160555,-31.1471601717549)) ;
#64610=CARTESIAN_POINT('',(87.2635276254219,616.710565160552,-31.0221601717549)) ;
#64611=CARTESIAN_POINT('',(149.888527625421,616.710565160541,-31.0221601717549)) ;
#64612=CARTESIAN_POINT('Origin',(87.2635276254219,616.710565160552,-31.1471601717549)) ;
#64613=CARTESIAN_POINT('',(94.6885276254222,616.710565160551,-25.7721601717558)) ;
#64614=CARTESIAN_POINT('',(97.4385276254221,616.71056516055,-25.772160171756)) ;
#64615=CARTESIAN_POINT('',(156.063527625422,616.71056516054,-25.7721601717586)) ;
#64616=CARTESIAN_POINT('',(97.4385276254222,616.71056516055,-24.122160171756)) ;
#64617=CARTESIAN_POINT('',(97.4385276254242,616.71056516055,19.910655277814)) ;
#64618=CARTESIAN_POINT('',(124.938527625422,616.710565160545,-24.1221601717572)) ;
#64619=CARTESIAN_POINT('',(97.4385276254222,616.71056516055,-24.122160171756)) ;
#64620=CARTESIAN_POINT('',(124.938527625422,616.710565160545,-25.7721601717572)) ;
#64621=CARTESIAN_POINT('',(124.938527625422,616.710565160545,-38.6663657544472)) ;
#64622=CARTESIAN_POINT('',(127.688527625422,616.710565160545,-25.7721601717573)) ;
#64623=CARTESIAN_POINT('',(156.063527625422,616.71056516054,-25.7721601717586)) ;
#64624=CARTESIAN_POINT('',(127.688527625422,616.710565160545,-38.1221601717573)) ;
#64625=CARTESIAN_POINT('',(127.688527625422,616.710565160545,-36.8221601717574)) ;
#64626=CARTESIAN_POINT('',(122.688527625421,616.710564962099,-43.1221604682021)) ;
#64627=CARTESIAN_POINT('Origin',(122.688527625422,616.710565160546,-38.1221601717571)) ;
#64628=CARTESIAN_POINT('',(99.6885276254214,616.710565358997,-43.122160473101)) ;
#64629=CARTESIAN_POINT('',(158.688527625421,616.710565160539,-43.1221607670988)) ;
#64630=CARTESIAN_POINT('',(94.6885276254216,616.710565160551,-38.1221601717558)) ;
#64631=CARTESIAN_POINT('Origin',(99.6885276254216,616.71056516055,-38.1221601717561)) ;
#64632=CARTESIAN_POINT('',(94.6885276254213,616.710565160551,-45.8221601717558)) ;
#64633=CARTESIAN_POINT('Origin',(212.388527625403,503.71056516053,0.477839828238782)) ;
#64634=CARTESIAN_POINT('',(-2.61147237459854,503.710565160568,-43.4900362557631)) ;
#64635=CARTESIAN_POINT('',(-2.61147237459654,503.710565160568,0.477839828248549)) ;
#64636=CARTESIAN_POINT('',(0.388527634349634,503.710565160567,-43.4900362557631)) ;
#64637=CARTESIAN_POINT('',(103.388527625413,503.710565160549,-43.4900362557631)) ;
#64638=CARTESIAN_POINT('',(0.38852763376135,503.710565160567,-47.5221601717516)) ;
#64639=CARTESIAN_POINT('',(0.388527634349642,503.710565160567,-24.0060982137622)) ;
#64640=CARTESIAN_POINT('',(193.688527625401,503.710565160533,-47.5221601717604)) ;
#64641=CARTESIAN_POINT('',(-2.61147237459866,503.710565160568,-47.5221601717515)) ;
#64642=CARTESIAN_POINT('',(193.688527625402,503.710565160533,-28.5221601717604)) ;
#64643=CARTESIAN_POINT('',(193.688527625401,503.710565160533,-47.5221601717604)) ;
#64644=CARTESIAN_POINT('',(197.688527625402,503.710565160533,-28.5221601717606)) ;
#64645=CARTESIAN_POINT('Origin',(195.688527625402,503.710565160533,-28.5221601717605)) ;
#64646=CARTESIAN_POINT('',(197.688527625401,503.710565160533,-47.5221601717606)) ;
#64647=CARTESIAN_POINT('',(197.688527625401,503.710565160533,-47.5221601717606)) ;
#64648=CARTESIAN_POINT('',(201.668527625401,503.710565160532,-47.5221601717608)) ;
#64649=CARTESIAN_POINT('',(201.668527625401,503.710565160532,-47.5221601717608)) ;
#64650=CARTESIAN_POINT('',(201.668527625402,503.710565160532,-28.5221601717607)) ;
#64651=CARTESIAN_POINT('',(201.668527625401,503.710565160532,-47.5221601717608)) ;
#64652=CARTESIAN_POINT('',(205.668527625402,503.710565160531,-28.5221601717609)) ;
#64653=CARTESIAN_POINT('Origin',(203.668527625402,503.710565160532,-28.5221601717608)) ;
#64654=CARTESIAN_POINT('',(205.668527625401,503.710565160531,-47.5221601717609)) ;
#64655=CARTESIAN_POINT('',(205.668527625402,503.710565160531,-28.5221601717609)) ;
#64656=CARTESIAN_POINT('',(-2.61147237459866,503.710565160568,-47.5221601717515)) ;
#64657=CARTESIAN_POINT('',(104.888527625403,503.710565160549,-19.5221601717563)) ;
#64658=CARTESIAN_POINT('',(3.73852762540217,503.710565160567,-24.0221601717537)) ;
#64659=CARTESIAN_POINT('Origin',(6.48852762540217,503.710565160566,-24.0221601717538)) ;
#64660=CARTESIAN_POINT('',(21.3885276254017,503.710565160564,-37.2221601717525)) ;
#64661=CARTESIAN_POINT('',(23.3885276254017,503.710565160563,-37.2221601717526)) ;
#64662=CARTESIAN_POINT('',(21.3885276254017,503.710565160564,-37.2221601717525)) ;
#64663=CARTESIAN_POINT('',(21.3885276254021,503.710565160564,-30.2221601717525)) ;
#64664=CARTESIAN_POINT('',(21.3885276254021,503.710565160564,-30.2221601717525)) ;
#64665=CARTESIAN_POINT('',(23.3885276254021,503.710565160563,-30.2221601717526)) ;
#64666=CARTESIAN_POINT('',(23.3885276254021,503.710565160563,-30.2221601717526)) ;
#64667=CARTESIAN_POINT('',(23.3885276254017,503.710565160563,-37.2221601717526)) ;
#64668=CARTESIAN_POINT('',(36.3885276254017,503.710565160561,-37.2221601717532)) ;
#64669=CARTESIAN_POINT('',(38.3885276254017,503.710565160561,-37.2221601717533)) ;
#64670=CARTESIAN_POINT('',(36.3885276254017,503.710565160561,-37.2221601717532)) ;
#64671=CARTESIAN_POINT('',(36.3885276254021,503.710565160561,-30.2221601717532)) ;
#64672=CARTESIAN_POINT('',(36.3885276254021,503.710565160561,-30.2221601717532)) ;
#64673=CARTESIAN_POINT('',(38.3885276254021,503.710565160561,-30.2221601717533)) ;
#64674=CARTESIAN_POINT('',(38.3885276254021,503.710565160561,-30.2221601717533)) ;
#64675=CARTESIAN_POINT('',(38.3885276254017,503.710565160561,-37.2221601717533)) ;
#64676=CARTESIAN_POINT('',(186.388527625402,503.710565160535,-37.22216017176)) ;
#64677=CARTESIAN_POINT('',(188.388527625402,503.710565160534,-37.2221601717601)) ;
#64678=CARTESIAN_POINT('',(186.388527625402,503.710565160535,-37.22216017176)) ;
#64679=CARTESIAN_POINT('',(186.388527625402,503.710565160535,-30.22216017176)) ;
#64680=CARTESIAN_POINT('',(186.388527625402,503.710565160535,-30.22216017176)) ;
#64681=CARTESIAN_POINT('',(188.388527625402,503.710565160534,-30.2221601717601)) ;
#64682=CARTESIAN_POINT('',(188.388527625402,503.710565160534,-30.2221601717601)) ;
#64683=CARTESIAN_POINT('',(188.388527625402,503.710565160534,-37.2221601717601)) ;
#64684=CARTESIAN_POINT('',(174.638527625402,503.710565160537,-38.1221601717595)) ;
#64685=CARTESIAN_POINT('',(169.388527626231,503.710565160538,-43.3721601717593)) ;
#64686=CARTESIAN_POINT('Origin',(169.388527625402,503.710565160538,-38.1221601717593)) ;
#64687=CARTESIAN_POINT('',(89.9885276254015,503.710565160552,-43.3721601717557)) ;
#64688=CARTESIAN_POINT('',(89.9885276254015,503.710565160552,-43.3721601717557)) ;
#64689=CARTESIAN_POINT('',(84.7385276254017,503.710565160553,-38.122160172492)) ;
#64690=CARTESIAN_POINT('Origin',(89.9885276254017,503.710565160551,-38.1221601717557)) ;
#64691=CARTESIAN_POINT('',(84.7385276254024,503.710565160553,-24.1221601717554)) ;
#64692=CARTESIAN_POINT('',(84.7385276254024,503.710565160553,-24.1221601717554)) ;
#64693=CARTESIAN_POINT('',(174.638527625402,503.710565160537,-24.1221601717595)) ;
#64694=CARTESIAN_POINT('',(174.638527625402,503.710565160537,-24.1221601717595)) ;
#64695=CARTESIAN_POINT('',(174.638527625402,503.710565160537,-38.1221601717595)) ;
#64696=CARTESIAN_POINT('',(184.638264665915,503.710565160535,-24.0197428787721)) ;
#64697=CARTESIAN_POINT('Origin',(187.388264603402,503.710565160534,-24.0203292412001)) ;
#64698=CARTESIAN_POINT('Ctrl Pts',(180.967886278451,503.710565160535,-38.2912310516114)) ;
#64699=CARTESIAN_POINT('Ctrl Pts',(180.92565375431,503.710565160535,-38.3365015005273)) ;
#64700=CARTESIAN_POINT('Ctrl Pts',(180.88084697963,503.710565160535,-38.3790384629369)) ;
#64701=CARTESIAN_POINT('Ctrl Pts',(180.833812038503,503.710565160535,-38.4188456718954)) ;
#64702=CARTESIAN_POINT('Ctrl Pts',(180.783552496009,503.710565160535,-38.4613819664522)) ;
#64703=CARTESIAN_POINT('Ctrl Pts',(180.730748583964,503.710565160535,-38.5008021215736)) ;
#64704=CARTESIAN_POINT('Ctrl Pts',(180.6757674221,503.710565160535,-38.5370815538523)) ;
#64705=CARTESIAN_POINT('Ctrl Pts',(180.621328160552,503.710565160535,-38.5730034120977)) ;
#64706=CARTESIAN_POINT('Ctrl Pts',(180.564753402286,503.710565160535,-38.6058465535098)) ;
#64707=CARTESIAN_POINT('Ctrl Pts',(180.506357253569,503.710565160535,-38.635551369466)) ;
#64708=CARTESIAN_POINT('Ctrl Pts',(180.487215433648,503.710565160535,-38.6452883855246)) ;
#64709=CARTESIAN_POINT('Ctrl Pts',(180.467877629559,503.710565160535,-38.6546878813455)) ;
#64710=CARTESIAN_POINT('Ctrl Pts',(180.448354169154,503.710565160535,-38.6637467966359)) ;
#64711=CARTESIAN_POINT('Ctrl Pts',(180.436388189703,503.710565160535,-38.669299029281)) ;
#64712=CARTESIAN_POINT('Ctrl Pts',(180.424350978305,503.710565160535,-38.6747238305229)) ;
#64713=CARTESIAN_POINT('Ctrl Pts',(180.412264471211,503.710565160535,-38.680012215594)) ;
#64714=CARTESIAN_POINT('Ctrl Pts',(180.350923190186,503.710565160535,-38.7068517575963)) ;
#64715=CARTESIAN_POINT('Ctrl Pts',(180.288204921529,503.710565160536,-38.7302329640473)) ;
#64716=CARTESIAN_POINT('Ctrl Pts',(180.224469064525,503.710565160536,-38.7501348242744)) ;
#64717=CARTESIAN_POINT('Ctrl Pts',(180.159384674807,503.710565160536,-38.770457771012)) ;
#64718=CARTESIAN_POINT('Ctrl Pts',(180.093238347601,503.710565160536,-38.7871531590327)) ;
#64719=CARTESIAN_POINT('Ctrl Pts',(180.02637585154,503.710565160536,-38.8001588616604)) ;
#64720=CARTESIAN_POINT('Ctrl Pts',(179.970650823328,503.710565160536,-38.8109981690234)) ;
#64721=CARTESIAN_POINT('Ctrl Pts',(179.914427390569,503.710565160536,-38.8192740427725)) ;
#64722=CARTESIAN_POINT('Ctrl Pts',(179.857893451262,503.710565160536,-38.8249257343172)) ;
#64723=CARTESIAN_POINT('Ctrl Pts',(179.831683152833,503.710565160536,-38.8275459748988)) ;
#64724=CARTESIAN_POINT('Ctrl Pts',(179.805405999129,503.710565160536,-38.8296018263968)) ;
#64725=CARTESIAN_POINT('Ctrl Pts',(179.779080308959,503.710565160536,-38.8310854028428)) ;
#64726=CARTESIAN_POINT('Ctrl Pts',(179.767740376304,503.710565160536,-38.8317244613776)) ;
#64727=CARTESIAN_POINT('Ctrl Pts',(179.756392022526,503.710565160536,-38.8322572009363)) ;
#64728=CARTESIAN_POINT('Ctrl Pts',(179.745050204682,503.710565160536,-38.8326827020381)) ;
#64729=CARTESIAN_POINT('Ctrl Pts',(179.674861914567,503.710565160536,-38.8353158949874)) ;
#64730=CARTESIAN_POINT('Ctrl Pts',(179.604793209435,503.710565160536,-38.8338540559347)) ;
#64731=CARTESIAN_POINT('Ctrl Pts',(179.535207522758,503.710565160536,-38.828245024526)) ;
#64732=CARTESIAN_POINT('Ctrl Pts',(179.472638445,503.710565160536,-38.8232015746569)) ;
#64733=CARTESIAN_POINT('Ctrl Pts',(179.41045891369,503.710565160536,-38.8148047974643)) ;
#64734=CARTESIAN_POINT('Ctrl Pts',(179.34892078897,503.710565160536,-38.8029829646867)) ;
#64735=CARTESIAN_POINT('Ctrl Pts',(179.282222053105,503.710565160536,-38.7901697484007)) ;
#64736=CARTESIAN_POINT('Ctrl Pts',(179.216275960956,503.710565160536,-38.7733339808827)) ;
#64737=CARTESIAN_POINT('Ctrl Pts',(179.151294678068,503.710565160536,-38.7527197824229)) ;
#64738=CARTESIAN_POINT('Ctrl Pts',(179.126490124642,503.710565160536,-38.744850962906)) ;
#64739=CARTESIAN_POINT('Ctrl Pts',(179.10182620156,503.710565160536,-38.7364310486033)) ;
#64740=CARTESIAN_POINT('Ctrl Pts',(179.077315026189,503.710565160536,-38.7274716808344)) ;
#64741=CARTESIAN_POINT('Ctrl Pts',(179.066519724691,503.710565160536,-38.7235257633161)) ;
#64742=CARTESIAN_POINT('Ctrl Pts',(179.055755047888,503.710565160536,-38.7194754705714)) ;
#64743=CARTESIAN_POINT('Ctrl Pts',(179.045033923296,503.710565160536,-38.7153266502158)) ;
#64744=CARTESIAN_POINT('Ctrl Pts',(178.979778672122,503.710565160536,-38.6900744192535)) ;
#64745=CARTESIAN_POINT('Ctrl Pts',(178.916019125604,503.710565160536,-38.6611341011757)) ;
#64746=CARTESIAN_POINT('Ctrl Pts',(178.853972447146,503.710565160536,-38.6288174516854)) ;
#64747=CARTESIAN_POINT('Ctrl Pts',(178.790503950737,503.710565160536,-38.5957602566335)) ;
#64748=CARTESIAN_POINT('Ctrl Pts',(178.728826906058,503.710565160536,-38.5591699147713)) ;
#64749=CARTESIAN_POINT('Ctrl Pts',(178.669177648379,503.710565160536,-38.519324021345)) ;
#64750=CARTESIAN_POINT('Ctrl Pts',(178.624103739663,503.710565160536,-38.4892145072808)) ;
#64751=CARTESIAN_POINT('Ctrl Pts',(178.580187697085,503.710565160536,-38.4572448398469)) ;
#64752=CARTESIAN_POINT('Ctrl Pts',(178.537537375342,503.710565160536,-38.4235161002359)) ;
#64753=CARTESIAN_POINT('Ctrl Pts',(178.511107918117,503.710565160536,-38.4026151493317)) ;
#64754=CARTESIAN_POINT('Ctrl Pts',(178.485164615864,503.710565160536,-38.3810384077748)) ;
#64755=CARTESIAN_POINT('Ctrl Pts',(178.459734712388,503.710565160536,-38.3588072065482)) ;
#64756=CARTESIAN_POINT('Ctrl Pts',(178.450011722904,503.710565160536,-38.3503072240003)) ;
#64757=CARTESIAN_POINT('Ctrl Pts',(178.440362108393,503.710565160536,-38.3417100057849)) ;
#64758=CARTESIAN_POINT('Ctrl Pts',(178.430792970441,503.710565160536,-38.3330216985486)) ;
#64759=CARTESIAN_POINT('Ctrl Pts',(178.373987234065,503.710565160536,-38.2814448801484)) ;
#64760=CARTESIAN_POINT('Ctrl Pts',(178.320152186293,503.710565160536,-38.226788560022)) ;
#64761=CARTESIAN_POINT('Ctrl Pts',(178.269568813303,503.710565160536,-38.1693636809231)) ;
#64762=CARTESIAN_POINT('Ctrl Pts',(178.23163128356,503.710565160536,-38.1262950215989)) ;
#64763=CARTESIAN_POINT('Ctrl Pts',(178.195523006449,503.710565160536,-38.0816677449143)) ;
#64764=CARTESIAN_POINT('Ctrl Pts',(178.161373031284,503.710565160536,-38.0355944133095)) ;
#64765=CARTESIAN_POINT('Ctrl Pts',(178.149255999991,503.710565160536,-38.019246758644)) ;
#64766=CARTESIAN_POINT('Ctrl Pts',(178.137385615073,503.710565160536,-38.0027169197252)) ;
#64767=CARTESIAN_POINT('Ctrl Pts',(178.125768018023,503.710565160536,-37.9860095118681)) ;
#64768=CARTESIAN_POINT('Ctrl Pts',(178.116969171299,503.710565160536,-37.9733557831959)) ;
#64769=CARTESIAN_POINT('Ctrl Pts',(178.108318282793,503.710565160536,-37.9606043293897)) ;
#64770=CARTESIAN_POINT('Ctrl Pts',(178.099822126482,503.710565160536,-37.9477641318199)) ;
#64771=CARTESIAN_POINT('Ctrl Pts',(178.058264513485,503.710565160536,-37.8849583238938)) ;
#64772=CARTESIAN_POINT('Ctrl Pts',(178.020373148467,503.710565160536,-37.8199849150515)) ;
#64773=CARTESIAN_POINT('Ctrl Pts',(177.986424343053,503.710565160536,-37.7531052054847)) ;
#64774=CARTESIAN_POINT('Ctrl Pts',(177.958995501856,503.710565160536,-37.6990699335321)) ;
#64775=CARTESIAN_POINT('Ctrl Pts',(177.934140557017,503.710565160536,-37.6437892876456)) ;
#64776=CARTESIAN_POINT('Ctrl Pts',(177.91202358458,503.710565160536,-37.5873842224957)) ;
#64777=CARTESIAN_POINT('Ctrl Pts',(177.907910233637,503.710565160536,-37.5768939156241)) ;
#64778=CARTESIAN_POINT('Ctrl Pts',(177.903891641335,503.710565160536,-37.5663646802333)) ;
#64779=CARTESIAN_POINT('Ctrl Pts',(177.899967455474,503.710565160536,-37.5557976775097)) ;
#64780=CARTESIAN_POINT('',(180.969462539582,503.709690117684,-35.7520600489767)) ;
#64781=CARTESIAN_POINT('Ctrl Pts',(177.903353299729,503.710565160537,-36.4919899545743)) ;
#64782=CARTESIAN_POINT('Ctrl Pts',(177.92875366093,503.710565160537,-36.4233890781418)) ;
#64783=CARTESIAN_POINT('Ctrl Pts',(177.958054337873,503.710565160536,-36.3564906321787)) ;
#64784=CARTESIAN_POINT('Ctrl Pts',(177.990958463266,503.710565160536,-36.2914824522412)) ;
#64785=CARTESIAN_POINT('Ctrl Pts',(178.024805498497,503.710565160536,-36.2246113796841)) ;
#64786=CARTESIAN_POINT('Ctrl Pts',(178.062466153447,503.710565160536,-36.1597396883479)) ;
#64787=CARTESIAN_POINT('Ctrl Pts',(178.103662086193,503.710565160536,-36.0971030288243)) ;
#64788=CARTESIAN_POINT('Ctrl Pts',(178.138514153112,503.710565160536,-36.0441119468471)) ;
#64789=CARTESIAN_POINT('Ctrl Pts',(178.175897575913,503.710565160536,-35.9927208717011)) ;
#64790=CARTESIAN_POINT('Ctrl Pts',(178.21566192862,503.710565160536,-35.943095316901)) ;
#64791=CARTESIAN_POINT('Ctrl Pts',(178.233297088326,503.710565160536,-35.921086796082)) ;
#64792=CARTESIAN_POINT('Ctrl Pts',(178.251400720061,503.710565160536,-35.8994258300726)) ;
#64793=CARTESIAN_POINT('Ctrl Pts',(178.269960423474,503.710565160536,-35.8781284061811)) ;
#64794=CARTESIAN_POINT('Ctrl Pts',(178.280129763591,503.710565160536,-35.8664589984135)) ;
#64795=CARTESIAN_POINT('Ctrl Pts',(178.290436033294,503.710565160536,-35.8548987517908)) ;
#64796=CARTESIAN_POINT('Ctrl Pts',(178.300877233601,503.710565160536,-35.8434504287225)) ;
#64797=CARTESIAN_POINT('Ctrl Pts',(178.31058164402,503.710565160536,-35.8328099637962)) ;
#64798=CARTESIAN_POINT('Ctrl Pts',(178.320404209226,503.710565160536,-35.822264668811)) ;
#64799=CARTESIAN_POINT('Ctrl Pts',(178.330327661833,503.710565160536,-35.8118328392013)) ;
#64800=CARTESIAN_POINT('Ctrl Pts',(178.380816949237,503.710565160536,-35.758756993108)) ;
#64801=CARTESIAN_POINT('Ctrl Pts',(178.433998984568,503.710565160536,-35.7085211059001)) ;
#64802=CARTESIAN_POINT('Ctrl Pts',(178.489610693573,503.710565160536,-35.6613432501725)) ;
#64803=CARTESIAN_POINT('Ctrl Pts',(178.54480483254,503.710565160536,-35.6145196374518)) ;
#64804=CARTESIAN_POINT('Ctrl Pts',(178.602393186154,503.710565160536,-35.5707077956924)) ;
#64805=CARTESIAN_POINT('Ctrl Pts',(178.662142797171,503.710565160536,-35.5301657365235)) ;
#64806=CARTESIAN_POINT('Ctrl Pts',(178.711887595478,503.710565160536,-35.4964122689777)) ;
#64807=CARTESIAN_POINT('Ctrl Pts',(178.763131118042,503.710565160536,-35.4649258789429)) ;
#64808=CARTESIAN_POINT('Ctrl Pts',(178.815745375594,503.710565160536,-35.4358832546787)) ;
#64809=CARTESIAN_POINT('Ctrl Pts',(178.837595338189,503.710565160536,-35.4238222605043)) ;
#64810=CARTESIAN_POINT('Ctrl Pts',(178.8596817389,503.710565160536,-35.412183045738)) ;
#64811=CARTESIAN_POINT('Ctrl Pts',(178.881995487401,503.710565160536,-35.4009796924745)) ;
#64812=CARTESIAN_POINT('Ctrl Pts',(178.892403669081,503.710565160536,-35.3957539216374)) ;
#64813=CARTESIAN_POINT('Ctrl Pts',(178.902861315364,503.710565160536,-35.3906229947982)) ;
#64814=CARTESIAN_POINT('Ctrl Pts',(178.913367501389,503.710565160536,-35.3855884072292)) ;
#64815=CARTESIAN_POINT('Ctrl Pts',(178.924203481469,503.710565160536,-35.38039578162)) ;
#64816=CARTESIAN_POINT('Ctrl Pts',(178.935083458973,503.710565160536,-35.3753093268688)) ;
#64817=CARTESIAN_POINT('Ctrl Pts',(178.946002593126,503.710565160536,-35.3703318526568)) ;
#64818=CARTESIAN_POINT('Ctrl Pts',(179.008613014799,503.710565160536,-35.3417909670061)) ;
#64819=CARTESIAN_POINT('Ctrl Pts',(179.072548898588,503.710565160536,-35.3168105966183)) ;
#64820=CARTESIAN_POINT('Ctrl Pts',(179.137602482649,503.710565160536,-35.2956138225865)) ;
#64821=CARTESIAN_POINT('Ctrl Pts',(179.196978933428,503.710565160536,-35.2762668607217)) ;
#64822=CARTESIAN_POINT('Ctrl Pts',(179.257287126168,503.710565160536,-35.2600722124355)) ;
#64823=CARTESIAN_POINT('Ctrl Pts',(179.318373891923,503.710565160536,-35.2472371731657)) ;
#64824=CARTESIAN_POINT('Ctrl Pts',(179.390171666925,503.710565160536,-35.2321516263986)) ;
#64825=CARTESIAN_POINT('Ctrl Pts',(179.463046503792,503.710565160536,-35.2217065918144)) ;
#64826=CARTESIAN_POINT('Ctrl Pts',(179.536577016775,503.710565160536,-35.2158270641581)) ;
#64827=CARTESIAN_POINT('Ctrl Pts',(179.552888295767,503.710565160536,-35.2145228081146)) ;
#64828=CARTESIAN_POINT('Ctrl Pts',(179.569231755604,503.710565160536,-35.2134434417709)) ;
#64829=CARTESIAN_POINT('Ctrl Pts',(179.585602626049,503.710565160536,-35.2125885256099)) ;
#64830=CARTESIAN_POINT('Ctrl Pts',(179.601628939277,503.710565160536,-35.2117516028435)) ;
#64831=CARTESIAN_POINT('Ctrl Pts',(179.617686819584,503.710565160536,-35.2111297845562)) ;
#64832=CARTESIAN_POINT('Ctrl Pts',(179.633740546289,503.710565160536,-35.2107231585423)) ;
#64833=CARTESIAN_POINT('Ctrl Pts',(179.702365296106,503.710565160536,-35.2089849572519)) ;
#64834=CARTESIAN_POINT('Ctrl Pts',(179.771008351008,503.710565160536,-35.2111671895507)) ;
#64835=CARTESIAN_POINT('Ctrl Pts',(179.839332646661,503.710565160536,-35.2171487203655)) ;
#64836=CARTESIAN_POINT('Ctrl Pts',(179.907485468652,503.710565160536,-35.2231152393167)) ;
#64837=CARTESIAN_POINT('Ctrl Pts',(179.975322186611,503.710565160536,-35.2328624822925)) ;
#64838=CARTESIAN_POINT('Ctrl Pts',(180.04249323035,503.710565160536,-35.2463196524421)) ;
#64839=CARTESIAN_POINT('Ctrl Pts',(180.091658875707,503.710565160536,-35.2561695880431)) ;
#64840=CARTESIAN_POINT('Ctrl Pts',(180.140467636658,503.710565160536,-35.2680081514718)) ;
#64841=CARTESIAN_POINT('Ctrl Pts',(180.188772438976,503.710565160536,-35.2818222804086)) ;
#64842=CARTESIAN_POINT('Ctrl Pts',(180.208747209415,503.710565160536,-35.2875346328267)) ;
#64843=CARTESIAN_POINT('Ctrl Pts',(180.228635683059,503.710565160536,-35.2935849339919)) ;
#64844=CARTESIAN_POINT('Ctrl Pts',(180.248426887822,503.710565160536,-35.299972818117)) ;
#64845=CARTESIAN_POINT('Ctrl Pts',(180.263114163255,503.710565160536,-35.3047133387022)) ;
#64846=CARTESIAN_POINT('Ctrl Pts',(180.277747862838,503.710565160535,-35.3096397827144)) ;
#64847=CARTESIAN_POINT('Ctrl Pts',(180.292323364453,503.710565160535,-35.3147521090727)) ;
#64848=CARTESIAN_POINT('Ctrl Pts',(180.30459079341,503.710565160535,-35.3190548838288)) ;
#64849=CARTESIAN_POINT('Ctrl Pts',(180.316809027902,503.710565160536,-35.3234865664285)) ;
#64850=CARTESIAN_POINT('Ctrl Pts',(180.32897214156,503.710565160536,-35.3280453620711)) ;
#64851=CARTESIAN_POINT('Ctrl Pts',(180.390631696042,503.710565160535,-35.3511556705168)) ;
#64852=CARTESIAN_POINT('Ctrl Pts',(180.450906378727,503.710565160535,-35.3775397554398)) ;
#64853=CARTESIAN_POINT('Ctrl Pts',(180.509464067445,503.710565160535,-35.4071474167633)) ;
#64854=CARTESIAN_POINT('Ctrl Pts',(180.550924650743,503.710565160536,-35.4281105205919)) ;
#64855=CARTESIAN_POINT('Ctrl Pts',(180.591523970704,503.710565160535,-35.4506904812246)) ;
#64856=CARTESIAN_POINT('Ctrl Pts',(180.631132547835,503.710565160535,-35.4748801279865)) ;
#64857=CARTESIAN_POINT('Ctrl Pts',(180.643785109954,503.710565160535,-35.4826072676732)) ;
#64858=CARTESIAN_POINT('Ctrl Pts',(180.656338382547,503.710565160535,-35.4904999551133)) ;
#64859=CARTESIAN_POINT('Ctrl Pts',(180.668781798428,503.710565160535,-35.4985541650934)) ;
#64860=CARTESIAN_POINT('Ctrl Pts',(180.721718073743,503.710565160535,-35.5328180586265)) ;
#64861=CARTESIAN_POINT('Ctrl Pts',(180.772571486636,503.710565160536,-35.5699380877714)) ;
#64862=CARTESIAN_POINT('Ctrl Pts',(180.821028469939,503.710565160536,-35.6098800128957)) ;
#64863=CARTESIAN_POINT('Ctrl Pts',(180.866170170906,503.710565160536,-35.64708923058)) ;
#64864=CARTESIAN_POINT('Ctrl Pts',(180.909232299481,503.710565160536,-35.6867479872827)) ;
#64865=CARTESIAN_POINT('Ctrl Pts',(180.949927175311,503.710565160536,-35.7288508505215)) ;
#64866=CARTESIAN_POINT('Ctrl Pts',(180.956875633919,503.710565160536,-35.7360397163559)) ;
#64867=CARTESIAN_POINT('Ctrl Pts',(180.963754988301,503.710565160536,-35.7432998832669)) ;
#64868=CARTESIAN_POINT('Ctrl Pts',(180.970564720765,503.710565160536,-35.7506301174499)) ;
#64869=CARTESIAN_POINT('Ctrl Pts',(180.968292474022,503.709690117684,-35.7534348777401)) ;
#64870=CARTESIAN_POINT('Ctrl Pts',(180.974127456679,503.709981798635,-35.7584008141771)) ;
#64871=CARTESIAN_POINT('Ctrl Pts',(180.979928180602,503.710273479585,-35.7634070046711)) ;
#64872=CARTESIAN_POINT('Ctrl Pts',(180.985694093679,503.710565160536,-35.7684529727346)) ;
#64873=CARTESIAN_POINT('Ctrl Pts',(30.9678862784492,503.710565160562,-38.2912310516066)) ;
#64874=CARTESIAN_POINT('Ctrl Pts',(30.9254422200844,503.710565160562,-38.3367282510996)) ;
#64875=CARTESIAN_POINT('Ctrl Pts',(30.880398964238,503.710565160562,-38.37946524855)) ;
#64876=CARTESIAN_POINT('Ctrl Pts',(30.8331075426913,503.710565160562,-38.4194456475178)) ;
#64877=CARTESIAN_POINT('Ctrl Pts',(30.7840703595289,503.710565160562,-38.4609019218898)) ;
#64878=CARTESIAN_POINT('Ctrl Pts',(30.7326155242731,503.710565160562,-38.4993948706189)) ;
#64879=CARTESIAN_POINT('Ctrl Pts',(30.6790837502068,503.710565160562,-38.5349018025089)) ;
#64880=CARTESIAN_POINT('Ctrl Pts',(30.6299497827742,503.710565160562,-38.5674917262607)) ;
#64881=CARTESIAN_POINT('Ctrl Pts',(30.5790650716403,503.710565160562,-38.5975660462198)) ;
#64882=CARTESIAN_POINT('Ctrl Pts',(30.5266633462617,503.710565160562,-38.6250826007819)) ;
#64883=CARTESIAN_POINT('Ctrl Pts',(30.5009196669565,503.710565160562,-38.6386008075034)) ;
#64884=CARTESIAN_POINT('Ctrl Pts',(30.4748094721683,503.710565160562,-38.651501306899)) ;
#64885=CARTESIAN_POINT('Ctrl Pts',(30.4483585771217,503.710565160562,-38.6637766953976)) ;
#64886=CARTESIAN_POINT('Ctrl Pts',(30.4363981919332,503.710565160562,-38.6693272967865)) ;
#64887=CARTESIAN_POINT('Ctrl Pts',(30.4243666589546,503.710565160562,-38.6747505776815)) ;
#64888=CARTESIAN_POINT('Ctrl Pts',(30.4122858861223,503.710565160562,-38.680037562082)) ;
#64889=CARTESIAN_POINT('Ctrl Pts',(30.3508796463339,503.710565160562,-38.7069111600186)) ;
#64890=CARTESIAN_POINT('Ctrl Pts',(30.2880936832432,503.710565160562,-38.7303188817798)) ;
#64891=CARTESIAN_POINT('Ctrl Pts',(30.2242884283509,503.710565160562,-38.7502394834274)) ;
#64892=CARTESIAN_POINT('Ctrl Pts',(30.1592053579717,503.710565160562,-38.7705590311074)) ;
#64893=CARTESIAN_POINT('Ctrl Pts',(30.0930609196203,503.710565160562,-38.78725096046)) ;
#64894=CARTESIAN_POINT('Ctrl Pts',(30.0262007044099,503.710565160562,-38.8002529480405)) ;
#64895=CARTESIAN_POINT('Ctrl Pts',(29.9705502048792,503.710565160562,-38.8110750356074)) ;
#64896=CARTESIAN_POINT('Ctrl Pts',(29.9144028696759,503.710565160562,-38.8193401845523)) ;
#64897=CARTESIAN_POINT('Ctrl Pts',(29.8579457755199,503.710565160562,-38.8249877807562)) ;
#64898=CARTESIAN_POINT('Ctrl Pts',(29.8317333455311,503.710565160562,-38.8276098997708)) ;
#64899=CARTESIAN_POINT('Ctrl Pts',(29.8054540290931,503.710565160562,-38.8296674312635)) ;
#64900=CARTESIAN_POINT('Ctrl Pts',(29.7791261443209,503.710565160562,-38.8311524769637)) ;
#64901=CARTESIAN_POINT('Ctrl Pts',(29.7677907216731,503.710565160562,-38.8317918606745)) ;
#64902=CARTESIAN_POINT('Ctrl Pts',(29.7564469004184,503.710565160562,-38.8323249875451)) ;
#64903=CARTESIAN_POINT('Ctrl Pts',(29.7451096041583,503.710565160562,-38.8327509389944)) ;
#64904=CARTESIAN_POINT('Ctrl Pts',(29.6749262076145,503.710565160562,-38.8353877863331)) ;
#64905=CARTESIAN_POINT('Ctrl Pts',(29.6048622076397,503.710565160562,-38.8339293126068)) ;
#64906=CARTESIAN_POINT('Ctrl Pts',(29.5352808719665,503.710565160562,-38.8283232046894)) ;
#64907=CARTESIAN_POINT('Ctrl Pts',(29.472724443851,503.710565160562,-38.8232830874862)) ;
#64908=CARTESIAN_POINT('Ctrl Pts',(29.4105571672994,503.710565160562,-38.8148902218149)) ;
#64909=CARTESIAN_POINT('Ctrl Pts',(29.3490306789795,503.710565160562,-38.803072799948)) ;
#64910=CARTESIAN_POINT('Ctrl Pts',(29.2823373784577,503.710565160562,-38.7902629860047)) ;
#64911=CARTESIAN_POINT('Ctrl Pts',(29.2163961579544,503.710565160562,-38.7734303424986)) ;
#64912=CARTESIAN_POINT('Ctrl Pts',(29.1514192353771,503.710565160562,-38.7528190391024)) ;
#64913=CARTESIAN_POINT('Ctrl Pts',(29.1266144198082,503.710565160562,-38.7449507135631)) ;
#64914=CARTESIAN_POINT('Ctrl Pts',(29.1019501818377,503.710565160562,-38.7365311742612)) ;
#64915=CARTESIAN_POINT('Ctrl Pts',(29.0774386443169,503.710565160562,-38.7275720679129)) ;
#64916=CARTESIAN_POINT('Ctrl Pts',(29.0666435317903,503.710565160562,-38.7236263928982)) ;
#64917=CARTESIAN_POINT('Ctrl Pts',(29.0558790328607,503.710565160562,-38.7195763273467)) ;
#64918=CARTESIAN_POINT('Ctrl Pts',(29.045158075543,503.710565160562,-38.7154277191505)) ;
#64919=CARTESIAN_POINT('Ctrl Pts',(28.9791589808581,503.710565160562,-38.6898885460116)) ;
#64920=CARTESIAN_POINT('Ctrl Pts',(28.9146895319876,503.710565160562,-38.660576147959)) ;
#64921=CARTESIAN_POINT('Ctrl Pts',(28.8519745023136,503.710565160562,-38.6278128528298)) ;
#64922=CARTESIAN_POINT('Ctrl Pts',(28.7892594726396,503.710565160562,-38.5950495577006)) ;
#64923=CARTESIAN_POINT('Ctrl Pts',(28.7282980769725,503.710565160562,-38.5588348642162)) ;
#64924=CARTESIAN_POINT('Ctrl Pts',(28.6693189033772,503.710565160562,-38.5194369089193)) ;
#64925=CARTESIAN_POINT('Ctrl Pts',(28.6242424962455,503.710565160562,-38.4893259703478)) ;
#64926=CARTESIAN_POINT('Ctrl Pts',(28.5803239211359,503.710565160562,-38.4573544700511)) ;
#64927=CARTESIAN_POINT('Ctrl Pts',(28.5376710848583,503.710565160562,-38.4236235398199)) ;
#64928=CARTESIAN_POINT('Ctrl Pts',(28.5112402242038,503.710565160562,-38.4027213538343)) ;
#64929=CARTESIAN_POINT('Ctrl Pts',(28.4852955197386,503.710565160562,-38.3811432476202)) ;
#64930=CARTESIAN_POINT('Ctrl Pts',(28.4598642273998,503.710565160562,-38.3589105629124)) ;
#64931=CARTESIAN_POINT('Ctrl Pts',(28.4501422583436,503.710565160562,-38.3504113694824)) ;
#64932=CARTESIAN_POINT('Ctrl Pts',(28.4404936410195,503.710565160562,-38.3418149523954)) ;
#64933=CARTESIAN_POINT('Ctrl Pts',(28.4309254817057,503.710565160562,-38.3331274627464)) ;
#64934=CARTESIAN_POINT('Ctrl Pts',(28.3756155014068,503.710565160562,-38.2829083071518)) ;
#64935=CARTESIAN_POINT('Ctrl Pts',(28.3231217092647,503.710565160562,-38.22976926723)) ;
#64936=CARTESIAN_POINT('Ctrl Pts',(28.2737032752297,503.710565160562,-38.1739980997431)) ;
#64937=CARTESIAN_POINT('Ctrl Pts',(28.2343018407941,503.710565160562,-38.1295316158888)) ;
#64938=CARTESIAN_POINT('Ctrl Pts',(28.196855448234,503.710565160562,-38.0833907473793)) ;
#64939=CARTESIAN_POINT('Ctrl Pts',(28.1615070381898,503.710565160562,-38.0357006475321)) ;
#64940=CARTESIAN_POINT('Ctrl Pts',(28.1493824195391,503.710565160562,-38.0193427894744)) ;
#64941=CARTESIAN_POINT('Ctrl Pts',(28.1375047434509,503.710565160562,-38.0028025194573)) ;
#64942=CARTESIAN_POINT('Ctrl Pts',(28.1258801643615,503.710565160562,-37.986084462753)) ;
#64943=CARTESIAN_POINT('Ctrl Pts',(28.1170775594472,503.710565160562,-37.9734248690617)) ;
#64944=CARTESIAN_POINT('Ctrl Pts',(28.1084230601432,503.710565160562,-37.9606674908369)) ;
#64945=CARTESIAN_POINT('Ctrl Pts',(28.0999234232508,503.710565160562,-37.947821283878)) ;
#64946=CARTESIAN_POINT('Ctrl Pts',(28.0583671615653,503.710565160562,-37.885013855183)) ;
#64947=CARTESIAN_POINT('Ctrl Pts',(28.0204771462595,503.710565160562,-37.820038892815)) ;
#64948=CARTESIAN_POINT('Ctrl Pts',(27.9865297735914,503.710565160562,-37.7531577608557)) ;
#64949=CARTESIAN_POINT('Ctrl Pts',(27.9591114444449,503.710565160562,-37.6991397693109)) ;
#64950=CARTESIAN_POINT('Ctrl Pts',(27.9342653114978,503.710565160562,-37.6438773379502)) ;
#64951=CARTESIAN_POINT('Ctrl Pts',(27.9121553253602,503.710565160562,-37.5874913344463)) ;
#64952=CARTESIAN_POINT('Ctrl Pts',(27.9080344254389,503.710565160562,-37.5769820073054)) ;
#64953=CARTESIAN_POINT('Ctrl Pts',(27.9040086289005,503.710565160562,-37.5664336134156)) ;
#64954=CARTESIAN_POINT('Ctrl Pts',(27.9000775815771,503.710565160562,-37.5558473201923)) ;
#64955=CARTESIAN_POINT('',(30.9693502314749,503.709709629953,-35.752017413352)) ;
#64956=CARTESIAN_POINT('Ctrl Pts',(27.9033532997302,503.710565160562,-36.4919899545636)) ;
#64957=CARTESIAN_POINT('Ctrl Pts',(27.9291186323697,503.710565160562,-36.4224033692924)) ;
#64958=CARTESIAN_POINT('Ctrl Pts',(27.9588957600935,503.710565160562,-36.3545683136294)) ;
#64959=CARTESIAN_POINT('Ctrl Pts',(27.9923754132967,503.710565160562,-36.2886810453698)) ;
#64960=CARTESIAN_POINT('Ctrl Pts',(28.0258550664998,503.710565160562,-36.2227937771102)) ;
#64961=CARTESIAN_POINT('Ctrl Pts',(28.063038117047,503.710565160562,-36.1588536853544)) ;
#64962=CARTESIAN_POINT('Ctrl Pts',(28.1036581552326,503.710565160562,-36.0970869979891)) ;
#64963=CARTESIAN_POINT('Ctrl Pts',(28.138506638453,503.710565160562,-36.0440965168282)) ;
#64964=CARTESIAN_POINT('Ctrl Pts',(28.175885788979,503.710565160562,-35.9927059676394)) ;
#64965=CARTESIAN_POINT('Ctrl Pts',(28.2156453273487,503.710565160562,-35.9430808735254)) ;
#64966=CARTESIAN_POINT('Ctrl Pts',(28.233276288535,503.710565160562,-35.9210751324112)) ;
#64967=CARTESIAN_POINT('Ctrl Pts',(28.2513755055103,503.710565160562,-35.8994168519458)) ;
#64968=CARTESIAN_POINT('Ctrl Pts',(28.2699305950182,503.710565160562,-35.8781220145597)) ;
#64969=CARTESIAN_POINT('Ctrl Pts',(28.2800999139146,503.710565160562,-35.866451146999)) ;
#64970=CARTESIAN_POINT('Ctrl Pts',(28.2904061701111,503.710565160562,-35.8548894646611)) ;
#64971=CARTESIAN_POINT('Ctrl Pts',(28.3008473659548,503.710565160562,-35.8434397311424)) ;
#64972=CARTESIAN_POINT('Ctrl Pts',(28.3105489342056,503.710565160562,-35.8328010674446)) ;
#64973=CARTESIAN_POINT('Ctrl Pts',(28.320368593542,503.710565160562,-35.82225754226)) ;
#64974=CARTESIAN_POINT('Ctrl Pts',(28.3302890881604,503.710565160562,-35.8118274425855)) ;
#64975=CARTESIAN_POINT('Ctrl Pts',(28.3807743786878,503.710565160562,-35.7587487774032)) ;
#64976=CARTESIAN_POINT('Ctrl Pts',(28.4339522312143,503.710565160562,-35.7085102932475)) ;
#64977=CARTESIAN_POINT('Ctrl Pts',(28.4895597627111,503.710565160562,-35.6613301145146)) ;
#64978=CARTESIAN_POINT('Ctrl Pts',(28.5443167148798,503.710565160562,-35.6148716093329)) ;
#64979=CARTESIAN_POINT('Ctrl Pts',(28.6014304833919,503.710565160562,-35.5713781267935)) ;
#64980=CARTESIAN_POINT('Ctrl Pts',(28.6606736741946,503.710565160562,-35.5311015201684)) ;
#64981=CARTESIAN_POINT('Ctrl Pts',(28.7108477173343,503.710565160562,-35.496990592466)) ;
#64982=CARTESIAN_POINT('Ctrl Pts',(28.7625497744598,503.710565160562,-35.4651875878731)) ;
#64983=CARTESIAN_POINT('Ctrl Pts',(28.8156483638411,503.710565160562,-35.4358740627275)) ;
#64984=CARTESIAN_POINT('Ctrl Pts',(28.8374967095457,503.710565160562,-35.4238124987826)) ;
#64985=CARTESIAN_POINT('Ctrl Pts',(28.8595815347472,503.710565160562,-35.4121727463269)) ;
#64986=CARTESIAN_POINT('Ctrl Pts',(28.8818937578735,503.710565160562,-35.4009688898361)) ;
#64987=CARTESIAN_POINT('Ctrl Pts',(28.8923047118028,503.710565160562,-35.3957411349371)) ;
#64988=CARTESIAN_POINT('Ctrl Pts',(28.9027651743749,503.710565160562,-35.3906082950447)) ;
#64989=CARTESIAN_POINT('Ctrl Pts',(28.9132742207043,503.710565160562,-35.3855718671928)) ;
#64990=CARTESIAN_POINT('Ctrl Pts',(28.9241052156119,503.710565160562,-35.3803811464836)) ;
#64991=CARTESIAN_POINT('Ctrl Pts',(28.9349801687178,503.710565160562,-35.3752965290426)) ;
#64992=CARTESIAN_POINT('Ctrl Pts',(28.9458942687065,503.710565160562,-35.3703208106301)) ;
#64993=CARTESIAN_POINT('Ctrl Pts',(29.008497953578,503.710565160562,-35.3417799041121)) ;
#64994=CARTESIAN_POINT('Ctrl Pts',(29.0724274399235,503.710565160562,-35.3167994837945)) ;
#64995=CARTESIAN_POINT('Ctrl Pts',(29.137475170634,503.710565160562,-35.2956026432451)) ;
#64996=CARTESIAN_POINT('Ctrl Pts',(29.1968462968923,503.710565160562,-35.2762556147971)) ;
#64997=CARTESIAN_POINT('Ctrl Pts',(29.257149618713,503.710565160562,-35.2600608879941)) ;
#64998=CARTESIAN_POINT('Ctrl Pts',(29.3182321292239,503.710565160562,-35.2472257671074)) ;
#64999=CARTESIAN_POINT('Ctrl Pts',(29.3900256430099,503.710565160562,-35.2321399688877)) ;
#65000=CARTESIAN_POINT('Ctrl Pts',(29.4628970918069,503.710565160562,-35.2216947742465)) ;
#65001=CARTESIAN_POINT('Ctrl Pts',(29.5364249740576,503.710565160562,-35.2158151578688)) ;
#65002=CARTESIAN_POINT('Ctrl Pts',(29.5527362121146,503.710565160562,-35.2145108387523)) ;
#65003=CARTESIAN_POINT('Ctrl Pts',(29.5690796704536,503.710565160562,-35.2134314278103)) ;
#65004=CARTESIAN_POINT('Ctrl Pts',(29.5854505771297,503.710565160562,-35.2125764852655)) ;
#65005=CARTESIAN_POINT('Ctrl Pts',(29.6014759873991,503.710565160562,-35.2117395856784)) ;
#65006=CARTESIAN_POINT('Ctrl Pts',(29.6175329970076,503.710565160562,-35.2111177828552)) ;
#65007=CARTESIAN_POINT('Ctrl Pts',(29.6335858867968,503.710565160562,-35.2107111643659)) ;
#65008=CARTESIAN_POINT('Ctrl Pts',(29.7019240276124,503.710565160562,-35.2089801644062)) ;
#65009=CARTESIAN_POINT('Ctrl Pts',(29.7702809286704,503.710565160562,-35.2111372171644)) ;
#65010=CARTESIAN_POINT('Ctrl Pts',(29.8383236179072,503.710565160562,-35.2170625644197)) ;
#65011=CARTESIAN_POINT('Ctrl Pts',(29.9064660399472,503.710565160562,-35.2229965966859)) ;
#65012=CARTESIAN_POINT('Ctrl Pts',(29.9742943886661,503.710565160562,-35.2327104142748)) ;
#65013=CARTESIAN_POINT('Ctrl Pts',(30.041459281945,503.710565160562,-35.2461330463219)) ;
#65014=CARTESIAN_POINT('Ctrl Pts',(30.0909216190662,503.710565160562,-35.2560178941786)) ;
#65015=CARTESIAN_POINT('Ctrl Pts',(30.1400239014881,503.710565160562,-35.2679151962761)) ;
#65016=CARTESIAN_POINT('Ctrl Pts',(30.1886164081109,503.710565160562,-35.2818116137659)) ;
#65017=CARTESIAN_POINT('Ctrl Pts',(30.208591560155,503.710565160562,-35.2875240799777)) ;
#65018=CARTESIAN_POINT('Ctrl Pts',(30.2284804448505,503.710565160562,-35.2935745008466)) ;
#65019=CARTESIAN_POINT('Ctrl Pts',(30.2482720871462,503.710565160562,-35.2999625101028)) ;
#65020=CARTESIAN_POINT('Ctrl Pts',(30.2629556614958,503.710565160562,-35.3047018241757)) ;
#65021=CARTESIAN_POINT('Ctrl Pts',(30.2775857039317,503.710565160562,-35.3096269627605)) ;
#65022=CARTESIAN_POINT('Ctrl Pts',(30.292157594932,503.710565160562,-35.314737884601)) ;
#65023=CARTESIAN_POINT('Ctrl Pts',(30.304427653017,503.710565160562,-35.3190414652309)) ;
#65024=CARTESIAN_POINT('Ctrl Pts',(30.3166485167175,503.710565160562,-35.3234740071886)) ;
#65025=CARTESIAN_POINT('Ctrl Pts',(30.3288142437168,503.710565160562,-35.328033710417)) ;
#65026=CARTESIAN_POINT('Ctrl Pts',(30.3904749935855,503.710565160562,-35.3511441024435)) ;
#65027=CARTESIAN_POINT('Ctrl Pts',(30.4507511168733,503.710565160562,-35.3775282676525)) ;
#65028=CARTESIAN_POINT('Ctrl Pts',(30.5093104003278,503.710565160562,-35.4071359897249)) ;
#65029=CARTESIAN_POINT('Ctrl Pts',(30.5507715572228,503.710565160562,-35.4280988556914)) ;
#65030=CARTESIAN_POINT('Ctrl Pts',(30.5913715511612,503.710565160562,-35.4506785253586)) ;
#65031=CARTESIAN_POINT('Ctrl Pts',(30.6309808754795,503.710565160562,-35.4748678223483)) ;
#65032=CARTESIAN_POINT('Ctrl Pts',(30.6436335721306,503.710565160562,-35.4825947867002)) ;
#65033=CARTESIAN_POINT('Ctrl Pts',(30.6561869871989,503.710565160562,-35.4904872892693)) ;
#65034=CARTESIAN_POINT('Ctrl Pts',(30.6686305569726,503.710565160562,-35.4985413075622)) ;
#65035=CARTESIAN_POINT('Ctrl Pts',(30.7215682446495,503.710565160562,-35.5328048760309)) ;
#65036=CARTESIAN_POINT('Ctrl Pts',(30.7724231620797,503.710565160562,-35.5699245066469)) ;
#65037=CARTESIAN_POINT('Ctrl Pts',(30.8208816659006,503.710565160562,-35.6098659448696)) ;
#65038=CARTESIAN_POINT('Ctrl Pts',(30.8660265554225,503.710565160562,-35.6470761695718)) ;
#65039=CARTESIAN_POINT('Ctrl Pts',(30.9090917235183,503.710565160561,-35.6867360487803)) ;
#65040=CARTESIAN_POINT('Ctrl Pts',(30.949789392883,503.710565160561,-35.7288401364669)) ;
#65041=CARTESIAN_POINT('Ctrl Pts',(30.956738104198,503.710565160561,-35.7360289793437)) ;
#65042=CARTESIAN_POINT('Ctrl Pts',(30.9636177085578,503.710565160561,-35.7432891216704)) ;
#65043=CARTESIAN_POINT('Ctrl Pts',(30.9704276883881,503.710565160561,-35.750619329669)) ;
#65044=CARTESIAN_POINT('Ctrl Pts',(30.968206386886,503.709709629953,-35.753361617214)) ;
#65045=CARTESIAN_POINT('Ctrl Pts',(30.9739106697334,503.709994806822,-35.7582156525672)) ;
#65046=CARTESIAN_POINT('Ctrl Pts',(30.9795822178181,503.710279983692,-35.7631081565965)) ;
#65047=CARTESIAN_POINT('Ctrl Pts',(30.9852205152954,503.710565160562,-35.7680386843137)) ;
#65048=CARTESIAN_POINT('Origin',(212.388527625421,618.71056516053,-49.5221601717612)) ;
#65049=CARTESIAN_POINT('',(205.668527625422,618.710565160531,-47.5221601717609)) ;
#65050=CARTESIAN_POINT('',(-2.61147237457848,618.710565160568,-47.5221601717514)) ;
#65051=CARTESIAN_POINT('',(205.668527625422,618.710565160531,-28.5221601717609)) ;
#65052=CARTESIAN_POINT('',(205.668527625422,618.710565160531,-47.5221601717609)) ;
#65053=CARTESIAN_POINT('',(201.668527625422,618.710565160532,-28.5221601717607)) ;
#65054=CARTESIAN_POINT('Origin',(203.668527625422,618.710565160532,-28.5221601717608)) ;
#65055=CARTESIAN_POINT('',(201.668527625421,618.710565160532,-47.5221601717607)) ;
#65056=CARTESIAN_POINT('',(201.668527625422,618.710565160532,-28.5221601717607)) ;
#65057=CARTESIAN_POINT('',(197.688527625422,618.710565160533,-47.5221601717605)) ;
#65058=CARTESIAN_POINT('',(201.668527625421,618.710565160532,-47.5221601717607)) ;
#65059=CARTESIAN_POINT('',(197.688527625422,618.710565160533,-28.5221601717605)) ;
#65060=CARTESIAN_POINT('',(197.688527625422,618.710565160533,-47.5221601717605)) ;
#65061=CARTESIAN_POINT('',(193.688527625422,618.710565160533,-28.5221601717604)) ;
#65062=CARTESIAN_POINT('Origin',(195.688527625422,618.710565160533,-28.5221601717604)) ;
#65063=CARTESIAN_POINT('',(193.688527625422,618.710565160533,-47.5221601717603)) ;
#65064=CARTESIAN_POINT('',(193.688527625422,618.710565160533,-47.5221601717603)) ;
#65065=CARTESIAN_POINT('',(152.388527625422,618.710565160541,-47.5221601717584)) ;
#65066=CARTESIAN_POINT('',(152.388527625422,618.710565160541,-47.5221601717584)) ;
#65067=CARTESIAN_POINT('',(152.388527625422,618.710565160541,-28.5221601717585)) ;
#65068=CARTESIAN_POINT('',(152.388527625422,618.710565160541,-47.5221601717584)) ;
#65069=CARTESIAN_POINT('',(148.388527625422,618.710565160541,-28.5221601717583)) ;
#65070=CARTESIAN_POINT('Origin',(150.388527625422,618.710565160541,-28.5221601717584)) ;
#65071=CARTESIAN_POINT('',(148.388527625422,618.710565160541,-47.5221601717583)) ;
#65072=CARTESIAN_POINT('',(148.388527625422,618.710565160541,-28.5221601717583)) ;
#65073=CARTESIAN_POINT('',(144.388527625422,618.710565160542,-47.5221601717581)) ;
#65074=CARTESIAN_POINT('',(144.388527625422,618.710565160542,-47.5221601717581)) ;
#65075=CARTESIAN_POINT('',(144.388527625422,618.710565160542,-28.5221601717581)) ;
#65076=CARTESIAN_POINT('',(144.388527625422,618.710565160542,-47.5221601717581)) ;
#65077=CARTESIAN_POINT('',(140.388527625422,618.710565160543,-28.5221601717579)) ;
#65078=CARTESIAN_POINT('Origin',(142.388527625422,618.710565160542,-28.522160171758)) ;
#65079=CARTESIAN_POINT('',(140.388527625421,618.710565160543,-47.5221601717579)) ;
#65080=CARTESIAN_POINT('',(140.388527625422,618.710565160543,-28.5221601717579)) ;
#65081=CARTESIAN_POINT('',(0.388527633780582,618.710565160567,-47.5221601717516)) ;
#65082=CARTESIAN_POINT('',(-2.61147237457848,618.710565160568,-47.5221601717514)) ;
#65083=CARTESIAN_POINT('',(0.3885276343684,618.710565160567,-43.4900362557631)) ;
#65084=CARTESIAN_POINT('',(0.388527634368422,618.710565160567,-49.0060982137622)) ;
#65085=CARTESIAN_POINT('',(-2.61147237457834,618.710565160568,-43.4900362557631)) ;
#65086=CARTESIAN_POINT('',(103.388527625432,618.710565160549,-43.4900362557631)) ;
#65087=CARTESIAN_POINT('',(-2.61147237457749,618.710565160568,-24.5221601717514)) ;
#65088=CARTESIAN_POINT('',(104.888527625423,618.710565160549,-19.5221601717563)) ;
#65089=CARTESIAN_POINT('',(87.2635276254222,618.710565160552,-30.8971601717549)) ;
#65090=CARTESIAN_POINT('',(87.5135276254222,618.710565160552,-31.1471601717549)) ;
#65091=CARTESIAN_POINT('Origin',(87.2635276254222,618.710565160552,-31.1471601717549)) ;
#65092=CARTESIAN_POINT('',(73.5135276254222,618.710565160554,-30.8971601717549)) ;
#65093=CARTESIAN_POINT('',(149.888527625422,618.710565160541,-30.8971601717549)) ;
#65094=CARTESIAN_POINT('',(73.2635276254222,618.710565160554,-31.1471601717549)) ;
#65095=CARTESIAN_POINT('Origin',(73.5135276254222,618.710565160554,-31.1471601717549)) ;
#65096=CARTESIAN_POINT('',(73.2635276254222,618.710565160554,-39.8971601717549)) ;
#65097=CARTESIAN_POINT('',(73.2635276254222,618.710565160554,-40.272160171758)) ;
#65098=CARTESIAN_POINT('',(73.5135276254222,618.710565160554,-40.1471601717549)) ;
#65099=CARTESIAN_POINT('Origin',(73.5135276254222,618.710565160554,-39.8971601717549)) ;
#65100=CARTESIAN_POINT('',(87.2635276254222,618.710565160552,-40.1471601717549)) ;
#65101=CARTESIAN_POINT('',(142.888527625422,618.710565160542,-40.1471601717549)) ;
#65102=CARTESIAN_POINT('',(87.5135276254222,618.710565160552,-39.8971601717549)) ;
#65103=CARTESIAN_POINT('Origin',(87.2635276254222,618.710565160552,-39.8971601717549)) ;
#65104=CARTESIAN_POINT('',(87.5135276254222,618.710565160552,-44.772160171758)) ;
#65105=CARTESIAN_POINT('Ctrl Pts',(30.9678862784723,618.710565160562,-35.7530892919022)) ;
#65106=CARTESIAN_POINT('Ctrl Pts',(30.9246614854188,618.710565160562,-35.7067551968985)) ;
#65107=CARTESIAN_POINT('Ctrl Pts',(30.8787404524756,618.710565160562,-35.6632842920493)) ;
#65108=CARTESIAN_POINT('Ctrl Pts',(30.830493598688,618.710565160562,-35.6226728706452)) ;
#65109=CARTESIAN_POINT('Ctrl Pts',(30.7822467449005,618.710565160562,-35.5820614492412)) ;
#65110=CARTESIAN_POINT('Ctrl Pts',(30.7316733549856,618.710565160562,-35.5443091349957)) ;
#65111=CARTESIAN_POINT('Ctrl Pts',(30.679095936171,618.710565160562,-35.5094375726184)) ;
#65112=CARTESIAN_POINT('Ctrl Pts',(30.6299565110526,618.710565160562,-35.476846232708)) ;
#65113=CARTESIAN_POINT('Ctrl Pts',(30.5790656467369,618.710565160562,-35.4467712038711)) ;
#65114=CARTESIAN_POINT('Ctrl Pts',(30.5266572192249,618.710565160562,-35.4192545791151)) ;
#65115=CARTESIAN_POINT('Ctrl Pts',(30.5009144572275,618.710565160562,-35.405738548284)) ;
#65116=CARTESIAN_POINT('Ctrl Pts',(30.4748051669133,618.710565160562,-35.3928401771113)) ;
#65117=CARTESIAN_POINT('Ctrl Pts',(30.4483551673175,618.710565160562,-35.3805668582694)) ;
#65118=CARTESIAN_POINT('Ctrl Pts',(30.4363904345703,618.710565160562,-35.3750149874902)) ;
#65119=CARTESIAN_POINT('Ctrl Pts',(30.4243544886558,618.710565160562,-35.3695905233535)) ;
#65120=CARTESIAN_POINT('Ctrl Pts',(30.412269259522,618.710565160562,-35.3643024486773)) ;
#65121=CARTESIAN_POINT('Ctrl Pts',(30.3509280970973,618.710565160562,-35.3374616958843)) ;
#65122=CARTESIAN_POINT('Ctrl Pts',(30.2882099920363,618.710565160562,-35.3140793129021)) ;
#65123=CARTESIAN_POINT('Ctrl Pts',(30.2244743219518,618.710565160562,-35.294176343009)) ;
#65124=CARTESIAN_POINT('Ctrl Pts',(30.1593907420887,618.710565160562,-35.2738524564187)) ;
#65125=CARTESIAN_POINT('Ctrl Pts',(30.0932452692249,618.710565160562,-35.2571561292323)) ;
#65126=CARTESIAN_POINT('Ctrl Pts',(30.026383639428,618.710565160562,-35.2441495216079)) ;
#65127=CARTESIAN_POINT('Ctrl Pts',(29.9706599072117,618.710565160562,-35.233309571662)) ;
#65128=CARTESIAN_POINT('Ctrl Pts',(29.9144377890335,618.710565160562,-35.2250330262529)) ;
#65129=CARTESIAN_POINT('Ctrl Pts',(29.8579051586923,618.710565160562,-35.2193806515948)) ;
#65130=CARTESIAN_POINT('Ctrl Pts',(29.8316943845793,618.710565160562,-35.2167599860699)) ;
#65131=CARTESIAN_POINT('Ctrl Pts',(29.8054167484692,618.710565160562,-35.2147037537742)) ;
#65132=CARTESIAN_POINT('Ctrl Pts',(29.7790905690437,618.710565160562,-35.2132198434095)) ;
#65133=CARTESIAN_POINT('Ctrl Pts',(29.7677516535389,618.710565160562,-35.2125807102497)) ;
#65134=CARTESIAN_POINT('Ctrl Pts',(29.7564043220059,618.710565160562,-35.2120478819763)) ;
#65135=CARTESIAN_POINT('Ctrl Pts',(29.745063524007,618.710565160562,-35.2116222778698)) ;
#65136=CARTESIAN_POINT('Ctrl Pts',(29.6748763277332,618.710565160562,-35.2089882516788)) ;
#65137=CARTESIAN_POINT('Ctrl Pts',(29.6048086763084,618.710565160562,-35.2104493210499)) ;
#65138=CARTESIAN_POINT('Ctrl Pts',(29.5352239666675,618.710565160562,-35.2160576802378)) ;
#65139=CARTESIAN_POINT('Ctrl Pts',(29.4726577330004,618.710565160562,-35.2211003672482)) ;
#65140=CARTESIAN_POINT('Ctrl Pts',(29.4104809593564,618.710565160563,-35.2294962498139)) ;
#65141=CARTESIAN_POINT('Ctrl Pts',(29.3489454561395,618.710565160563,-35.2413170737421)) ;
#65142=CARTESIAN_POINT('Ctrl Pts',(29.2822479435602,618.710565160563,-35.2541295074014)) ;
#65143=CARTESIAN_POINT('Ctrl Pts',(29.2163029514434,618.710565160563,-35.2709645531108)) ;
#65144=CARTESIAN_POINT('Ctrl Pts',(29.1513226566763,618.710565160563,-35.2915780798982)) ;
#65145=CARTESIAN_POINT('Ctrl Pts',(29.1265180515532,618.710565160563,-35.2994467790783)) ;
#65146=CARTESIAN_POINT('Ctrl Pts',(29.1018540653138,618.710565160563,-35.3078665994065)) ;
#65147=CARTESIAN_POINT('Ctrl Pts',(29.0773428165287,618.710565160563,-35.3168258983797)) ;
#65148=CARTESIAN_POINT('Ctrl Pts',(29.0665475612047,618.710565160563,-35.3207717569031)) ;
#65149=CARTESIAN_POINT('Ctrl Pts',(29.055782928172,618.710565160563,-35.3248219940153)) ;
#65150=CARTESIAN_POINT('Ctrl Pts',(29.0450618450274,618.710565160563,-35.3289707620551)) ;
#65151=CARTESIAN_POINT('Ctrl Pts',(28.9798075371171,618.710565160563,-35.3542224071978)) ;
#65152=CARTESIAN_POINT('Ctrl Pts',(28.9160488162804,618.710565160563,-35.3831621836307)) ;
#65153=CARTESIAN_POINT('Ctrl Pts',(28.8540028587099,618.710565160563,-35.4154783248475)) ;
#65154=CARTESIAN_POINT('Ctrl Pts',(28.7905349461042,618.710565160563,-35.448535079982)) ;
#65155=CARTESIAN_POINT('Ctrl Pts',(28.7288583842423,618.710565160563,-35.4851250339393)) ;
#65156=CARTESIAN_POINT('Ctrl Pts',(28.6692095221533,618.710565160563,-35.5249705780916)) ;
#65157=CARTESIAN_POINT('Ctrl Pts',(28.6089722266453,618.710565160563,-35.5652091967965)) ;
#65158=CARTESIAN_POINT('Ctrl Pts',(28.5508019236201,618.710565160563,-35.6087684304393)) ;
#65159=CARTESIAN_POINT('Ctrl Pts',(28.4949591104778,618.710565160563,-35.6554128189863)) ;
#65160=CARTESIAN_POINT('Ctrl Pts',(28.4831219231459,618.710565160563,-35.6653001855809)) ;
#65161=CARTESIAN_POINT('Ctrl Pts',(28.4713894054236,618.710565160563,-35.6753263402784)) ;
#65162=CARTESIAN_POINT('Ctrl Pts',(28.4597641973492,618.710565160563,-35.68548929546)) ;
#65163=CARTESIAN_POINT('Ctrl Pts',(28.4500414342721,618.710565160563,-35.6939891007762)) ;
#65164=CARTESIAN_POINT('Ctrl Pts',(28.440392041099,618.710565160563,-35.702586139205)) ;
#65165=CARTESIAN_POINT('Ctrl Pts',(28.430823120432,618.710565160563,-35.7112742631367)) ;
#65166=CARTESIAN_POINT('Ctrl Pts',(28.3755127664173,618.710565160563,-35.7614934286106)) ;
#65167=CARTESIAN_POINT('Ctrl Pts',(28.3230188069169,618.710565160563,-35.8146323668433)) ;
#65168=CARTESIAN_POINT('Ctrl Pts',(28.2736003531469,618.710565160563,-35.870403376926)) ;
#65169=CARTESIAN_POINT('Ctrl Pts',(28.2341986630398,618.710565160563,-35.9148700060615)) ;
#65170=CARTESIAN_POINT('Ctrl Pts',(28.1967521325585,618.710565160563,-35.9610110047264)) ;
#65171=CARTESIAN_POINT('Ctrl Pts',(28.1614036766299,618.710565160563,-36.00870124493)) ;
#65172=CARTESIAN_POINT('Ctrl Pts',(28.1492849977504,618.710565160563,-36.0250511162762)) ;
#65173=CARTESIAN_POINT('Ctrl Pts',(28.1374130297479,618.710565160563,-36.0415832216434)) ;
#65174=CARTESIAN_POINT('Ctrl Pts',(28.1257939169347,618.710565160563,-36.0582929435484)) ;
#65175=CARTESIAN_POINT('Ctrl Pts',(28.1169942611476,618.710565160563,-36.070947937387)) ;
#65176=CARTESIAN_POINT('Ctrl Pts',(28.1083425954881,618.710565160563,-36.0837006692725)) ;
#65177=CARTESIAN_POINT('Ctrl Pts',(28.0998456901819,618.710565160563,-36.0965421634147)) ;
#65178=CARTESIAN_POINT('Ctrl Pts',(28.0582883984916,618.710565160563,-36.1593482908903)) ;
#65179=CARTESIAN_POINT('Ctrl Pts',(28.0203973528173,618.710565160563,-36.2243220061981)) ;
#65180=CARTESIAN_POINT('Ctrl Pts',(27.9864488831358,618.710565160563,-36.2912019953229)) ;
#65181=CARTESIAN_POINT('Ctrl Pts',(27.9590223508319,618.710565160563,-36.3452334789043)) ;
#65182=CARTESIAN_POINT('Ctrl Pts',(27.9341693434085,618.710565160563,-36.4005101339978)) ;
#65183=CARTESIAN_POINT('Ctrl Pts',(27.9120539095342,618.710565160563,-36.4569110249402)) ;
#65184=CARTESIAN_POINT('Ctrl Pts',(27.9079385582216,618.710565160563,-36.4674063867718)) ;
#65185=CARTESIAN_POINT('Ctrl Pts',(27.9039180571055,618.710565160563,-36.4779407140531)) ;
#65186=CARTESIAN_POINT('Ctrl Pts',(27.8999920534665,618.710565160563,-36.4885128439382)) ;
#65187=CARTESIAN_POINT('',(30.969436549502,618.711435750373,-38.2922703312628)) ;
#65188=CARTESIAN_POINT('Ctrl Pts',(27.9033532997491,618.710565160563,-37.5523303889371)) ;
#65189=CARTESIAN_POINT('Ctrl Pts',(27.9288862972234,618.710565160563,-37.6212894872279)) ;
#65190=CARTESIAN_POINT('Ctrl Pts',(27.9583601267478,618.710565160563,-37.6885283764075)) ;
#65191=CARTESIAN_POINT('Ctrl Pts',(27.9914734180815,618.710565160563,-37.7538561924087)) ;
#65192=CARTESIAN_POINT('Ctrl Pts',(28.0253525646813,618.710565160563,-37.8206949319665)) ;
#65193=CARTESIAN_POINT('Ctrl Pts',(28.0630422037844,618.710565160563,-37.8855339267015)) ;
#65194=CARTESIAN_POINT('Ctrl Pts',(28.1042643880468,618.710565160563,-37.9481374667155)) ;
#65195=CARTESIAN_POINT('Ctrl Pts',(28.1389437182194,618.710565160563,-38.0008044680635)) ;
#65196=CARTESIAN_POINT('Ctrl Pts',(28.1761242586142,618.710565160563,-38.0518889788485)) ;
#65197=CARTESIAN_POINT('Ctrl Pts',(28.2156582418674,618.710565160563,-38.1012282656295)) ;
#65198=CARTESIAN_POINT('Ctrl Pts',(28.233292464534,618.710565160563,-38.123236166117)) ;
#65199=CARTESIAN_POINT('Ctrl Pts',(28.2513951108522,618.710565160563,-38.1448965329139)) ;
#65200=CARTESIAN_POINT('Ctrl Pts',(28.2699537842564,618.710565160563,-38.1661933798041)) ;
#65201=CARTESIAN_POINT('Ctrl Pts',(28.2801231194327,618.710565160563,-38.177863113384)) ;
#65202=CARTESIAN_POINT('Ctrl Pts',(28.2904293858722,618.710565160563,-38.1894236804798)) ;
#65203=CARTESIAN_POINT('Ctrl Pts',(28.3008705848837,618.710565160563,-38.2008723184176)) ;
#65204=CARTESIAN_POINT('Ctrl Pts',(28.3105743611267,618.710565160563,-38.21151238195)) ;
#65205=CARTESIAN_POINT('Ctrl Pts',(28.3203962779074,618.710565160563,-38.2220572825773)) ;
#65206=CARTESIAN_POINT('Ctrl Pts',(28.3303190704187,618.710565160563,-38.232488726747)) ;
#65207=CARTESIAN_POINT('Ctrl Pts',(28.3808070646547,618.710565160563,-38.2855647829586)) ;
#65208=CARTESIAN_POINT('Ctrl Pts',(28.4339877215713,618.710565160563,-38.3358008763694)) ;
#65209=CARTESIAN_POINT('Ctrl Pts',(28.4895980151892,618.710565160563,-38.3829789282195)) ;
#65210=CARTESIAN_POINT('Ctrl Pts',(28.5443605121329,618.710565160563,-38.4294377356122)) ;
#65211=CARTESIAN_POINT('Ctrl Pts',(28.6014800276728,618.710565160563,-38.4729314705988)) ;
#65212=CARTESIAN_POINT('Ctrl Pts',(28.6607289931891,618.710565160563,-38.5132082911547)) ;
#65213=CARTESIAN_POINT('Ctrl Pts',(28.710909637196,618.710565160563,-38.5473205625916)) ;
#65214=CARTESIAN_POINT('Ctrl Pts',(28.7626184193456,618.710565160563,-38.5791247261134)) ;
#65215=CARTESIAN_POINT('Ctrl Pts',(28.8157237359714,618.710565160563,-38.6084392126371)) ;
#65216=CARTESIAN_POINT('Ctrl Pts',(28.8375733334271,618.710565160563,-38.6205003351548)) ;
#65217=CARTESIAN_POINT('Ctrl Pts',(28.8596593778976,618.710565160563,-38.6321396712192)) ;
#65218=CARTESIAN_POINT('Ctrl Pts',(28.8819727809855,618.710565160563,-38.6433431382079)) ;
#65219=CARTESIAN_POINT('Ctrl Pts',(28.8923815922453,618.710565160563,-38.6485693590977)) ;
#65220=CARTESIAN_POINT('Ctrl Pts',(28.9028398779815,618.710565160563,-38.6537007199305)) ;
#65221=CARTESIAN_POINT('Ctrl Pts',(28.913346713321,618.710565160563,-38.6587357250361)) ;
#65222=CARTESIAN_POINT('Ctrl Pts',(28.9241815639023,618.710565160563,-38.6639279190919)) ;
#65223=CARTESIAN_POINT('Ctrl Pts',(28.9350604028915,618.710565160563,-38.6690139576571)) ;
#65224=CARTESIAN_POINT('Ctrl Pts',(28.9459783961876,618.710565160563,-38.6739910342067)) ;
#65225=CARTESIAN_POINT('Ctrl Pts',(29.0085873058914,618.710565160563,-38.7025319325049)) ;
#65226=CARTESIAN_POINT('Ctrl Pts',(29.0725217509502,618.710565160562,-38.7275123221109)) ;
#65227=CARTESIAN_POINT('Ctrl Pts',(29.1375740146656,618.710565160562,-38.7487091191263)) ;
#65228=CARTESIAN_POINT('Ctrl Pts',(29.1969492541683,618.710565160562,-38.7680560999629)) ;
#65229=CARTESIAN_POINT('Ctrl Pts',(29.2572563340101,618.710565160563,-38.7842507710163)) ;
#65230=CARTESIAN_POINT('Ctrl Pts',(29.31834212105,618.710565160563,-38.7970858349689)) ;
#65231=CARTESIAN_POINT('Ctrl Pts',(29.3901389193237,618.710565160562,-38.8121714472215)) ;
#65232=CARTESIAN_POINT('Ctrl Pts',(29.4630129701239,618.710565160562,-38.8226165274978)) ;
#65233=CARTESIAN_POINT('Ctrl Pts',(29.5365428627453,618.710565160562,-38.8284960853624)) ;
#65234=CARTESIAN_POINT('Ctrl Pts',(29.5528541311509,618.710565160562,-38.8298003582644)) ;
#65235=CARTESIAN_POINT('Ctrl Pts',(29.5691975890634,618.710565160562,-38.8308797372017)) ;
#65236=CARTESIAN_POINT('Ctrl Pts',(29.5855684658677,618.710565160562,-38.8317346617483)) ;
#65237=CARTESIAN_POINT('Ctrl Pts',(29.6015945658302,618.710565160562,-38.8325715812613)) ;
#65238=CARTESIAN_POINT('Ctrl Pts',(29.6176522398986,618.710565160562,-38.8331933981503)) ;
#65239=CARTESIAN_POINT('Ctrl Pts',(29.6337057677761,618.710565160562,-38.833600024665)) ;
#65240=CARTESIAN_POINT('Ctrl Pts',(29.7023301789556,618.710565160562,-38.8353382410466)) ;
#65241=CARTESIAN_POINT('Ctrl Pts',(29.7709730308323,618.710565160562,-38.8331560000629)) ;
#65242=CARTESIAN_POINT('Ctrl Pts',(29.8392972346922,618.710565160562,-38.827174441035)) ;
#65243=CARTESIAN_POINT('Ctrl Pts',(29.9074499692971,618.710565160562,-38.8212078935756)) ;
#65244=CARTESIAN_POINT('Ctrl Pts',(29.9752867105702,618.710565160562,-38.8114606021859)) ;
#65245=CARTESIAN_POINT('Ctrl Pts',(30.0424578652503,618.710565160562,-38.7980033675824)) ;
#65246=CARTESIAN_POINT('Ctrl Pts',(30.0916234690244,618.710565160562,-38.7881534094038)) ;
#65247=CARTESIAN_POINT('Ctrl Pts',(30.140432237142,618.710565160562,-38.7763148247249)) ;
#65248=CARTESIAN_POINT('Ctrl Pts',(30.1887370875502,618.710565160562,-38.762500677227)) ;
#65249=CARTESIAN_POINT('Ctrl Pts',(30.2087119349343,618.710565160562,-38.7567883008159)) ;
#65250=CARTESIAN_POINT('Ctrl Pts',(30.2286004920296,618.710565160562,-38.750737974188)) ;
#65251=CARTESIAN_POINT('Ctrl Pts',(30.248391786102,618.710565160562,-38.744350063234)) ;
#65252=CARTESIAN_POINT('Ctrl Pts',(30.263078162565,618.710565160562,-38.7396098342859)) ;
#65253=CARTESIAN_POINT('Ctrl Pts',(30.2777109734449,618.710565160562,-38.7346837055941)) ;
#65254=CARTESIAN_POINT('Ctrl Pts',(30.292285597272,618.710565160562,-38.7295717182766)) ;
#65255=CARTESIAN_POINT('Ctrl Pts',(30.3045536459369,618.710565160562,-38.7252687523868)) ;
#65256=CARTESIAN_POINT('Ctrl Pts',(30.3167724999768,618.710565160562,-38.7208368658164)) ;
#65257=CARTESIAN_POINT('Ctrl Pts',(30.3289362292424,618.710565160562,-38.716277854615)) ;
#65258=CARTESIAN_POINT('Ctrl Pts',(30.3905960186477,618.710565160562,-38.6931675350383)) ;
#65259=CARTESIAN_POINT('Ctrl Pts',(30.4508709911739,618.710565160562,-38.666783438768)) ;
#65260=CARTESIAN_POINT('Ctrl Pts',(30.5094290049217,618.710565160562,-38.6371757693896)) ;
#65261=CARTESIAN_POINT('Ctrl Pts',(30.5508896963081,618.710565160562,-38.6162127215639)) ;
#65262=CARTESIAN_POINT('Ctrl Pts',(30.5914891470767,618.710565160562,-38.5936328280989)) ;
#65263=CARTESIAN_POINT('Ctrl Pts',(30.6310978718703,618.710565160562,-38.5694432608945)) ;
#65264=CARTESIAN_POINT('Ctrl Pts',(30.6437504598953,618.710565160562,-38.5617161596072)) ;
#65265=CARTESIAN_POINT('Ctrl Pts',(30.6563037601999,618.710565160562,-38.5538235125602)) ;
#65266=CARTESIAN_POINT('Ctrl Pts',(30.6687472063364,618.710565160562,-38.5457693443873)) ;
#65267=CARTESIAN_POINT('Ctrl Pts',(30.7216837718687,618.710565160562,-38.5115055241707)) ;
#65268=CARTESIAN_POINT('Ctrl Pts',(30.7725374966231,618.710565160562,-38.4743855832958)) ;
#65269=CARTESIAN_POINT('Ctrl Pts',(30.8209947969149,618.710565160562,-38.4344437646062)) ;
#65270=CARTESIAN_POINT('Ctrl Pts',(30.8661371617876,618.710565160562,-38.3972343422465)) ;
#65271=CARTESIAN_POINT('Ctrl Pts',(30.9091999248329,618.710565160562,-38.3575753566552)) ;
#65272=CARTESIAN_POINT('Ctrl Pts',(30.9498953849965,618.710565160562,-38.3154722432163)) ;
#65273=CARTESIAN_POINT('Ctrl Pts',(30.9568438963168,618.710565160562,-38.3082833833491)) ;
#65274=CARTESIAN_POINT('Ctrl Pts',(30.9637233028815,618.710565160562,-38.301023222749)) ;
#65275=CARTESIAN_POINT('Ctrl Pts',(30.9705330870232,618.710565160562,-38.2936929952148)) ;
#65276=CARTESIAN_POINT('Ctrl Pts',(30.9682724688976,618.711435750373,-38.2909024911338)) ;
#65277=CARTESIAN_POINT('Ctrl Pts',(30.9740776063841,618.711145553769,-38.2859621126416)) ;
#65278=CARTESIAN_POINT('Ctrl Pts',(30.9798488362412,618.710855357166,-38.2809818913689)) ;
#65279=CARTESIAN_POINT('Ctrl Pts',(30.9855856147846,618.710565160562,-38.2759622964822)) ;
#65280=CARTESIAN_POINT('Ctrl Pts',(180.967886278469,618.710565160535,-35.7530892919063)) ;
#65281=CARTESIAN_POINT('Ctrl Pts',(180.925656002869,618.710565160535,-35.7078212532777)) ;
#65282=CARTESIAN_POINT('Ctrl Pts',(180.880851236392,618.710565160535,-35.6652868410807)) ;
#65283=CARTESIAN_POINT('Ctrl Pts',(180.833818101144,618.710565160535,-35.6254822445482)) ;
#65284=CARTESIAN_POINT('Ctrl Pts',(180.783557499346,618.710565160535,-35.5829462119081)) ;
#65285=CARTESIAN_POINT('Ctrl Pts',(180.730751994801,618.710565160535,-35.5435267603272)) ;
#65286=CARTESIAN_POINT('Ctrl Pts',(180.675768818775,618.710565160535,-35.507248385621)) ;
#65287=CARTESIAN_POINT('Ctrl Pts',(180.627658539752,618.710565160535,-35.4755048077531)) ;
#65288=CARTESIAN_POINT('Ctrl Pts',(180.577879742994,618.710565160535,-35.4461663668647)) ;
#65289=CARTESIAN_POINT('Ctrl Pts',(180.5266506585,618.710565160535,-35.4192725627713)) ;
#65290=CARTESIAN_POINT('Ctrl Pts',(180.500908854801,618.710565160535,-35.4057588521023)) ;
#65291=CARTESIAN_POINT('Ctrl Pts',(180.474800508004,618.710565160535,-35.3928627527034)) ;
#65292=CARTESIAN_POINT('Ctrl Pts',(180.448351441031,618.710565160535,-35.3805916458249)) ;
#65293=CARTESIAN_POINT('Ctrl Pts',(180.436382104309,618.710565160535,-35.3750384438792)) ;
#65294=CARTESIAN_POINT('Ctrl Pts',(180.424341484995,618.710565160535,-35.3696127401546)) ;
#65295=CARTESIAN_POINT('Ctrl Pts',(180.412251536294,618.710565160535,-35.3643235246544)) ;
#65296=CARTESIAN_POINT('Ctrl Pts',(180.350909936507,618.710565160535,-35.3374872701404)) ;
#65297=CARTESIAN_POINT('Ctrl Pts',(180.288191225939,618.710565160536,-35.3141092617675)) ;
#65298=CARTESIAN_POINT('Ctrl Pts',(180.224454861394,618.710565160536,-35.2942104227471)) ;
#65299=CARTESIAN_POINT('Ctrl Pts',(180.159558087471,618.710565160536,-35.2739492976196)) ;
#65300=CARTESIAN_POINT('Ctrl Pts',(180.093605424765,618.710565160535,-35.257294627986)) ;
#65301=CARTESIAN_POINT('Ctrl Pts',(180.026939752979,618.710565160535,-35.2443078456473)) ;
#65302=CARTESIAN_POINT('Ctrl Pts',(179.971019742292,618.710565160535,-35.2334143679739)) ;
#65303=CARTESIAN_POINT('Ctrl Pts',(179.914597108006,618.710565160536,-35.2251021895574)) ;
#65304=CARTESIAN_POINT('Ctrl Pts',(179.857861807401,618.710565160536,-35.2194326090212)) ;
#65305=CARTESIAN_POINT('Ctrl Pts',(179.831652792875,618.710565160536,-35.2168135320613)) ;
#65306=CARTESIAN_POINT('Ctrl Pts',(179.805376940538,618.710565160536,-35.214758725493)) ;
#65307=CARTESIAN_POINT('Ctrl Pts',(179.779052569468,618.710565160536,-35.2132760679416)) ;
#65308=CARTESIAN_POINT('Ctrl Pts',(179.767709862447,618.710565160536,-35.2126372169631)) ;
#65309=CARTESIAN_POINT('Ctrl Pts',(179.756358720358,618.710565160536,-35.2121047236115)) ;
#65310=CARTESIAN_POINT('Ctrl Pts',(179.745014120561,618.710565160536,-35.2116795079059)) ;
#65311=CARTESIAN_POINT('Ctrl Pts',(179.674822878097,618.710565160536,-35.2090486157432)) ;
#65312=CARTESIAN_POINT('Ctrl Pts',(179.604751323395,618.710565160536,-35.2105125865917)) ;
#65313=CARTESIAN_POINT('Ctrl Pts',(179.535162987157,618.710565160536,-35.2161234898321)) ;
#65314=CARTESIAN_POINT('Ctrl Pts',(179.472586177512,618.710565160536,-35.2211690541175)) ;
#65315=CARTESIAN_POINT('Ctrl Pts',(179.410399142565,618.710565160536,-35.22956830857)) ;
#65316=CARTESIAN_POINT('Ctrl Pts',(179.34885387623,618.710565160536,-35.2413929346126)) ;
#65317=CARTESIAN_POINT('Ctrl Pts',(179.282151812096,618.710565160536,-35.254208330688)) ;
#65318=CARTESIAN_POINT('Ctrl Pts',(179.216202716827,618.710565160536,-35.2710461175169)) ;
#65319=CARTESIAN_POINT('Ctrl Pts',(179.151218726316,618.710565160536,-35.2916622027171)) ;
#65320=CARTESIAN_POINT('Ctrl Pts',(179.12641429349,618.710565160536,-35.2995313762851)) ;
#65321=CARTESIAN_POINT('Ctrl Pts',(179.101750521018,618.710565160536,-35.307951574045)) ;
#65322=CARTESIAN_POINT('Ctrl Pts',(179.07723952307,618.710565160536,-35.3169111578168)) ;
#65323=CARTESIAN_POINT('Ctrl Pts',(179.06644408674,618.710565160536,-35.3208572483169)) ;
#65324=CARTESIAN_POINT('Ctrl Pts',(179.055679281374,618.710565160536,-35.3249077051062)) ;
#65325=CARTESIAN_POINT('Ctrl Pts',(179.044958034348,618.710565160536,-35.3290566806503)) ;
#65326=CARTESIAN_POINT('Ctrl Pts',(178.979700192647,618.710565160536,-35.3543105702976)) ;
#65327=CARTESIAN_POINT('Ctrl Pts',(178.915938366599,618.710565160536,-35.3832524293362)) ;
#65328=CARTESIAN_POINT('Ctrl Pts',(178.853889686145,618.710565160536,-35.415570530269)) ;
#65329=CARTESIAN_POINT('Ctrl Pts',(178.790419543132,618.710565160536,-35.4486290010233)) ;
#65330=CARTESIAN_POINT('Ctrl Pts',(178.728741119599,618.710565160536,-35.485220480269)) ;
#65331=CARTESIAN_POINT('Ctrl Pts',(178.669090714849,618.710565160536,-35.525067407697)) ;
#65332=CARTESIAN_POINT('Ctrl Pts',(178.624018007635,618.710565160536,-35.5551763214728)) ;
#65333=CARTESIAN_POINT('Ctrl Pts',(178.580103192787,618.710565160536,-35.5871451589576)) ;
#65334=CARTESIAN_POINT('Ctrl Pts',(178.537454095892,618.710565160536,-35.6208728672108)) ;
#65335=CARTESIAN_POINT('Ctrl Pts',(178.511025350192,618.710565160536,-35.641773216559)) ;
#65336=CARTESIAN_POINT('Ctrl Pts',(178.485082760104,618.710565160536,-35.6633492815855)) ;
#65337=CARTESIAN_POINT('Ctrl Pts',(178.459653562549,618.710565160536,-35.6855797374052)) ;
#65338=CARTESIAN_POINT('Ctrl Pts',(178.449929967101,618.710565160536,-35.694080200644)) ;
#65339=CARTESIAN_POINT('Ctrl Pts',(178.440279759941,618.710565160536,-35.7026779060663)) ;
#65340=CARTESIAN_POINT('Ctrl Pts',(178.430710039992,618.710565160536,-35.7113667095423)) ;
#65341=CARTESIAN_POINT('Ctrl Pts',(178.373903690972,618.710565160536,-35.7629438931444)) ;
#65342=CARTESIAN_POINT('Ctrl Pts',(178.320068210137,618.710565160536,-35.8176004972375)) ;
#65343=CARTESIAN_POINT('Ctrl Pts',(178.26948453935,618.710565160536,-35.8750256209584)) ;
#65344=CARTESIAN_POINT('Ctrl Pts',(178.23154678626,618.710565160536,-35.918094463749)) ;
#65345=CARTESIAN_POINT('Ctrl Pts',(178.195438361975,618.710565160536,-35.9627219017164)) ;
#65346=CARTESIAN_POINT('Ctrl Pts',(178.161288298157,618.710565160536,-36.0087953897241)) ;
#65347=CARTESIAN_POINT('Ctrl Pts',(178.149175580158,618.710565160536,-36.025137238174)) ;
#65348=CARTESIAN_POINT('Ctrl Pts',(178.137309339071,618.710565160536,-36.0416611396476)) ;
#65349=CARTESIAN_POINT('Ctrl Pts',(178.125695708976,618.710565160536,-36.0583624845284)) ;
#65350=CARTESIAN_POINT('Ctrl Pts',(178.116898961978,618.710565160536,-36.0710129223538)) ;
#65351=CARTESIAN_POINT('Ctrl Pts',(178.108250089833,618.710565160536,-36.0837610514211)) ;
#65352=CARTESIAN_POINT('Ctrl Pts',(178.099755876389,618.710565160536,-36.0965978756731)) ;
#65353=CARTESIAN_POINT('Ctrl Pts',(178.058197337227,618.710565160536,-36.1594029449052)) ;
#65354=CARTESIAN_POINT('Ctrl Pts',(178.020305055465,618.710565160536,-36.2243756452309)) ;
#65355=CARTESIAN_POINT('Ctrl Pts',(177.986355294698,618.710565160536,-36.2912547125809)) ;
#65356=CARTESIAN_POINT('Ctrl Pts',(177.958920326772,618.710565160536,-36.3453000144096)) ;
#65357=CARTESIAN_POINT('Ctrl Pts',(177.934060234432,618.710565160536,-36.4005912193201)) ;
#65358=CARTESIAN_POINT('Ctrl Pts',(177.911939165789,618.710565160536,-36.457007322563)) ;
#65359=CARTESIAN_POINT('Ctrl Pts',(177.907831226466,618.710565160536,-36.4674839379868)) ;
#65360=CARTESIAN_POINT('Ctrl Pts',(177.903817797862,618.710565160574,-36.4779993817103)) ;
#65361=CARTESIAN_POINT('Ctrl Pts',(177.899898529339,618.710565160544,-36.4885524971287)) ;
#65362=CARTESIAN_POINT('',(180.969536013849,618.711452603529,-38.2922314065076)) ;
#65363=CARTESIAN_POINT('Ctrl Pts',(177.90335329975,618.710565160536,-37.552330388949)) ;
#65364=CARTESIAN_POINT('Ctrl Pts',(177.92875265027,618.710565160536,-37.6209285357504)) ;
#65365=CARTESIAN_POINT('Ctrl Pts',(177.958052767198,618.710565160537,-37.6878243168137)) ;
#65366=CARTESIAN_POINT('Ctrl Pts',(177.99095668214,618.710565160536,-37.7528299326183)) ;
#65367=CARTESIAN_POINT('Ctrl Pts',(178.024804526857,618.710565160536,-37.8197003944861)) ;
#65368=CARTESIAN_POINT('Ctrl Pts',(178.062466592364,618.710565160536,-37.8845714605626)) ;
#65369=CARTESIAN_POINT('Ctrl Pts',(178.10366440299,618.710565160536,-37.9472075021294)) ;
#65370=CARTESIAN_POINT('Ctrl Pts',(178.138518637012,618.710565160537,-38.0001989406988)) ;
#65371=CARTESIAN_POINT('Ctrl Pts',(178.17590464559,618.710565160537,-38.051590324619)) ;
#65372=CARTESIAN_POINT('Ctrl Pts',(178.215671915688,618.710565160536,-38.1012161461691)) ;
#65373=CARTESIAN_POINT('Ctrl Pts',(178.233309628192,618.710565160536,-38.1232263563529)) ;
#65374=CARTESIAN_POINT('Ctrl Pts',(178.251415944853,618.710565160536,-38.1448889538452)) ;
#65375=CARTESIAN_POINT('Ctrl Pts',(178.269978455095,618.710565160536,-38.1661879483558)) ;
#65376=CARTESIAN_POINT('Ctrl Pts',(178.280147809454,618.710565160536,-38.1778564683908)) ;
#65377=CARTESIAN_POINT('Ctrl Pts',(178.290454088964,618.710565160536,-38.1894158417102)) ;
#65378=CARTESIAN_POINT('Ctrl Pts',(178.300895293865,618.710565160536,-38.2008633066224)) ;
#65379=CARTESIAN_POINT('Ctrl Pts',(178.310601431425,618.710565160536,-38.211504862862)) ;
#65380=CARTESIAN_POINT('Ctrl Pts',(178.320425762691,618.710565160536,-38.222051229921)) ;
#65381=CARTESIAN_POINT('Ctrl Pts',(178.330351013256,618.710565160536,-38.2324841072426)) ;
#65382=CARTESIAN_POINT('Ctrl Pts',(178.380800128125,618.710565160536,-38.2855134411581)) ;
#65383=CARTESIAN_POINT('Ctrl Pts',(178.433937571481,618.710565160536,-38.3357077319362)) ;
#65384=CARTESIAN_POINT('Ctrl Pts',(178.489500808843,618.710565160536,-38.382849507741)) ;
#65385=CARTESIAN_POINT('Ctrl Pts',(178.544743275573,618.710565160536,-38.4297191306276)) ;
#65386=CARTESIAN_POINT('Ctrl Pts',(178.602384494608,618.710565160536,-38.4735719050078)) ;
#65387=CARTESIAN_POINT('Ctrl Pts',(178.662190756132,618.710565160536,-38.5141491743324)) ;
#65388=CARTESIAN_POINT('Ctrl Pts',(178.711939225079,618.710565160536,-38.5479024465072)) ;
#65389=CARTESIAN_POINT('Ctrl Pts',(178.763186423315,618.710565160536,-38.5793886345307)) ;
#65390=CARTESIAN_POINT('Ctrl Pts',(178.815804283139,618.710565160536,-38.6084310566786)) ;
#65391=CARTESIAN_POINT('Ctrl Pts',(178.837655252695,618.710565160536,-38.6204916970072)) ;
#65392=CARTESIAN_POINT('Ctrl Pts',(178.859742637093,618.710565160536,-38.632130576785)) ;
#65393=CARTESIAN_POINT('Ctrl Pts',(178.882057340823,618.710565160536,-38.6433336153461)) ;
#65394=CARTESIAN_POINT('Ctrl Pts',(178.892463777766,618.710565160536,-38.6485581397573)) ;
#65395=CARTESIAN_POINT('Ctrl Pts',(178.902919652307,618.710565160536,-38.6536878644943)) ;
#65396=CARTESIAN_POINT('Ctrl Pts',(178.913424039632,618.710565160536,-38.6587212953844)) ;
#65397=CARTESIAN_POINT('Ctrl Pts',(178.924263143256,618.710565160536,-38.6639151136734)) ;
#65398=CARTESIAN_POINT('Ctrl Pts',(178.93514626959,618.710565160536,-38.6690027184636)) ;
#65399=CARTESIAN_POINT('Ctrl Pts',(178.946068559414,618.710565160536,-38.6739812913392)) ;
#65400=CARTESIAN_POINT('Ctrl Pts',(179.008683124175,618.710565160536,-38.702522117372)) ;
#65401=CARTESIAN_POINT('Ctrl Pts',(179.072622958707,618.710565160536,-38.7275024100009)) ;
#65402=CARTESIAN_POINT('Ctrl Pts',(179.13768017974,618.710565160536,-38.7486990958925)) ;
#65403=CARTESIAN_POINT('Ctrl Pts',(179.197059993512,618.710565160536,-38.7680459914542)) ;
#65404=CARTESIAN_POINT('Ctrl Pts',(179.257371289354,618.710565160536,-38.7842405601685)) ;
#65405=CARTESIAN_POINT('Ctrl Pts',(179.318460801853,618.710565160536,-38.7970755115389)) ;
#65406=CARTESIAN_POINT('Ctrl Pts',(179.390261310164,618.710565160536,-38.8121608509833)) ;
#65407=CARTESIAN_POINT('Ctrl Pts',(179.46313837298,618.710565160536,-38.8226057307213)) ;
#65408=CARTESIAN_POINT('Ctrl Pts',(179.536670670084,618.710565160536,-38.82848514471)) ;
#65409=CARTESIAN_POINT('Ctrl Pts',(179.552981982092,618.710565160536,-38.8297893465338)) ;
#65410=CARTESIAN_POINT('Ctrl Pts',(179.569325451759,618.710565160536,-38.8308686706868)) ;
#65411=CARTESIAN_POINT('Ctrl Pts',(179.585696309858,618.710565160536,-38.8317235565352)) ;
#65412=CARTESIAN_POINT('Ctrl Pts',(179.601723236992,618.710565160536,-38.8325604823162)) ;
#65413=CARTESIAN_POINT('Ctrl Pts',(179.617781712558,618.710565160536,-38.8331822982082)) ;
#65414=CARTESIAN_POINT('Ctrl Pts',(179.633836014706,618.710565160536,-38.8335889163139)) ;
#65415=CARTESIAN_POINT('Ctrl Pts',(179.70246178681,618.710565160536,-38.835327047389)) ;
#65416=CARTESIAN_POINT('Ctrl Pts',(179.771105501388,618.710565160536,-38.8331448085213)) ;
#65417=CARTESIAN_POINT('Ctrl Pts',(179.839430158321,618.710565160536,-38.8271633236124)) ;
#65418=CARTESIAN_POINT('Ctrl Pts',(179.907568389827,618.710565160536,-38.8211981593254)) ;
#65419=CARTESIAN_POINT('Ctrl Pts',(179.975390358138,618.710565160536,-38.8114539801615)) ;
#65420=CARTESIAN_POINT('Ctrl Pts',(180.042546786254,618.710565160536,-38.7980015312525)) ;
#65421=CARTESIAN_POINT('Ctrl Pts',(180.091727522222,618.710565160536,-38.7881498855279)) ;
#65422=CARTESIAN_POINT('Ctrl Pts',(180.140551072165,618.710565160536,-38.7763084156596)) ;
#65423=CARTESIAN_POINT('Ctrl Pts',(180.18887025211,618.710565160536,-38.7624901938655)) ;
#65424=CARTESIAN_POINT('Ctrl Pts',(180.208844836146,618.710565160536,-38.7567779025399)) ;
#65425=CARTESIAN_POINT('Ctrl Pts',(180.228733105885,618.710565160536,-38.7507276669264)) ;
#65426=CARTESIAN_POINT('Ctrl Pts',(180.248524090962,618.710565160536,-38.7443398525418)) ;
#65427=CARTESIAN_POINT('Ctrl Pts',(180.263213998755,618.710565160536,-38.7395984814609)) ;
#65428=CARTESIAN_POINT('Ctrl Pts',(180.277850301612,618.710565160536,-38.7346711184834)) ;
#65429=CARTESIAN_POINT('Ctrl Pts',(180.292428375474,618.710565160536,-38.7295578045955)) ;
#65430=CARTESIAN_POINT('Ctrl Pts',(180.304694037984,618.710565160536,-38.7252555776313)) ;
#65431=CARTESIAN_POINT('Ctrl Pts',(180.316910506913,618.710565160536,-38.720824480024)) ;
#65432=CARTESIAN_POINT('Ctrl Pts',(180.329071866739,618.710565160536,-38.7162663029856)) ;
#65433=CARTESIAN_POINT('Ctrl Pts',(180.390730875172,618.710565160536,-38.6931560027825)) ;
#65434=CARTESIAN_POINT('Ctrl Pts',(180.451004861965,618.710565160536,-38.6667719293244)) ;
#65435=CARTESIAN_POINT('Ctrl Pts',(180.509561757029,618.710565160536,-38.6371642734416)) ;
#65436=CARTESIAN_POINT('Ctrl Pts',(180.551022103343,618.710565160536,-38.6162010091653)) ;
#65437=CARTESIAN_POINT('Ctrl Pts',(180.591621123789,618.710565160536,-38.5936208597328)) ;
#65438=CARTESIAN_POINT('Ctrl Pts',(180.631229354313,618.710565160536,-38.5694309926077)) ;
#65439=CARTESIAN_POINT('Ctrl Pts',(180.643881857526,618.710565160536,-38.5617037508834)) ;
#65440=CARTESIAN_POINT('Ctrl Pts',(180.656435066235,618.710565160536,-38.5538109563834)) ;
#65441=CARTESIAN_POINT('Ctrl Pts',(180.668878411365,618.710565160536,-38.545756635812)) ;
#65442=CARTESIAN_POINT('Ctrl Pts',(180.721813972028,618.710565160536,-38.511492539563)) ;
#65443=CARTESIAN_POINT('Ctrl Pts',(180.772666608596,618.710565160536,-38.474372270941)) ;
#65444=CARTESIAN_POINT('Ctrl Pts',(180.821122797544,618.710565160536,-38.434430061149)) ;
#65445=CARTESIAN_POINT('Ctrl Pts',(180.866262830651,618.710565160536,-38.3972213430987)) ;
#65446=CARTESIAN_POINT('Ctrl Pts',(180.909323361008,618.710565160536,-38.3575631474454)) ;
#65447=CARTESIAN_POINT('Ctrl Pts',(180.950016762044,618.710565160536,-38.3154608990898)) ;
#65448=CARTESIAN_POINT('Ctrl Pts',(180.956965088351,618.710565160536,-38.308272014593)) ;
#65449=CARTESIAN_POINT('Ctrl Pts',(180.963844311663,618.710565160536,-38.3010118281384)) ;
#65450=CARTESIAN_POINT('Ctrl Pts',(180.970653914223,618.710565160536,-38.2936815735458)) ;
#65451=CARTESIAN_POINT('Ctrl Pts',(180.968349279596,618.711452603529,-38.2908371184949)) ;
#65452=CARTESIAN_POINT('Ctrl Pts',(180.97426742378,618.711156789198,-38.2857999494516)) ;
#65453=CARTESIAN_POINT('Ctrl Pts',(180.980150321186,618.710860974867,-38.2807213691574)) ;
#65454=CARTESIAN_POINT('Ctrl Pts',(180.985997395766,618.710565160536,-38.2756018749041)) ;
#65455=CARTESIAN_POINT('',(94.4385276254219,618.710565160551,-38.1221601717558)) ;
#65456=CARTESIAN_POINT('',(99.688527624592,618.71056516055,-43.3721601717561)) ;
#65457=CARTESIAN_POINT('Origin',(99.6885276254219,618.71056516055,-38.1221601717561)) ;
#65458=CARTESIAN_POINT('',(122.688527625422,618.710565160546,-43.3721601717571)) ;
#65459=CARTESIAN_POINT('',(122.688527625422,618.710565160546,-43.3721601717571)) ;
#65460=CARTESIAN_POINT('',(127.938527625422,618.710565160545,-38.1221601724939)) ;
#65461=CARTESIAN_POINT('Origin',(122.688527625422,618.710565160546,-38.1221601717571)) ;
#65462=CARTESIAN_POINT('',(127.938527625423,618.710565160545,-24.1221601717574)) ;
#65463=CARTESIAN_POINT('',(127.938527625423,618.710565160545,-24.1221601717574)) ;
#65464=CARTESIAN_POINT('',(94.4385276254226,618.710565160551,-24.1221601717558)) ;
#65465=CARTESIAN_POINT('',(94.4385276254226,618.710565160551,-24.1221601717558)) ;
#65466=CARTESIAN_POINT('',(94.4385276254219,618.710565160551,-38.1221601717558)) ;
#65467=CARTESIAN_POINT('',(21.3885276254223,618.710565160564,-30.2221601717525)) ;
#65468=CARTESIAN_POINT('',(23.3885276254223,618.710565160563,-30.2221601717526)) ;
#65469=CARTESIAN_POINT('',(21.3885276254223,618.710565160564,-30.2221601717525)) ;
#65470=CARTESIAN_POINT('',(21.388527625422,618.710565160564,-37.2221601717525)) ;
#65471=CARTESIAN_POINT('',(21.388527625422,618.710565160564,-37.2221601717525)) ;
#65472=CARTESIAN_POINT('',(23.388527625422,618.710565160563,-37.2221601717526)) ;
#65473=CARTESIAN_POINT('',(23.388527625422,618.710565160563,-37.2221601717526)) ;
#65474=CARTESIAN_POINT('',(23.3885276254223,618.710565160563,-30.2221601717526)) ;
#65475=CARTESIAN_POINT('',(36.3885276254223,618.710565160561,-30.2221601717532)) ;
#65476=CARTESIAN_POINT('',(38.3885276254223,618.710565160561,-30.2221601717533)) ;
#65477=CARTESIAN_POINT('',(36.3885276254223,618.710565160561,-30.2221601717532)) ;
#65478=CARTESIAN_POINT('',(36.388527625422,618.710565160561,-37.2221601717532)) ;
#65479=CARTESIAN_POINT('',(36.388527625422,618.710565160561,-37.2221601717532)) ;
#65480=CARTESIAN_POINT('',(38.388527625422,618.710565160561,-37.2221601717533)) ;
#65481=CARTESIAN_POINT('',(38.388527625422,618.710565160561,-37.2221601717533)) ;
#65482=CARTESIAN_POINT('',(38.3885276254223,618.710565160561,-30.2221601717533)) ;
#65483=CARTESIAN_POINT('',(171.388527625422,618.710565160537,-30.2221601717593)) ;
#65484=CARTESIAN_POINT('',(173.388527625422,618.710565160537,-30.2221601717594)) ;
#65485=CARTESIAN_POINT('',(171.388527625422,618.710565160537,-30.2221601717593)) ;
#65486=CARTESIAN_POINT('',(171.388527625422,618.710565160537,-37.2221601717593)) ;
#65487=CARTESIAN_POINT('',(171.388527625422,618.710565160537,-37.2221601717593)) ;
#65488=CARTESIAN_POINT('',(173.388527625422,618.710565160537,-37.2221601717594)) ;
#65489=CARTESIAN_POINT('',(173.388527625422,618.710565160537,-37.2221601717594)) ;
#65490=CARTESIAN_POINT('',(173.388527625422,618.710565160537,-30.2221601717594)) ;
#65491=CARTESIAN_POINT('',(186.388527625422,618.710565160535,-30.22216017176)) ;
#65492=CARTESIAN_POINT('',(188.388527625422,618.710565160534,-30.2221601717601)) ;
#65493=CARTESIAN_POINT('',(186.388527625422,618.710565160535,-30.22216017176)) ;
#65494=CARTESIAN_POINT('',(186.388527625422,618.710565160535,-37.22216017176)) ;
#65495=CARTESIAN_POINT('',(186.388527625422,618.710565160535,-37.22216017176)) ;
#65496=CARTESIAN_POINT('',(188.388527625422,618.710565160534,-37.2221601717601)) ;
#65497=CARTESIAN_POINT('',(188.388527625422,618.710565160534,-37.2221601717601)) ;
#65498=CARTESIAN_POINT('',(188.388527625422,618.710565160534,-30.2221601717601)) ;
#65499=CARTESIAN_POINT('',(187.378265783355,618.710565160534,-26.7703110636122)) ;
#65500=CARTESIAN_POINT('Origin',(187.388264603423,618.710565160534,-24.0203292412001)) ;
#65501=CARTESIAN_POINT('',(6.47826578335511,618.710565160566,-26.770311063604)) ;
#65502=CARTESIAN_POINT('Origin',(6.48826460342255,618.710565160563,-24.0203292411918)) ;
#65503=CARTESIAN_POINT('Origin',(0.388527634368701,620.552123681176,-48.4900362557631)) ;
#65504=CARTESIAN_POINT('',(0.388527634368074,616.710565160567,-49.5221601717515)) ;
#65505=CARTESIAN_POINT('Origin',(0.388527634368074,616.710565160567,-47.5221601717516)) ;
#65506=CARTESIAN_POINT('',(0.388527634367972,616.077123681176,-49.5221601717516)) ;
#65507=CARTESIAN_POINT('',(0.38852763435921,562.381344420871,-49.5221601717516)) ;
#65508=CARTESIAN_POINT('',(0.38852763436797,616.077123681176,-48.4900362557631)) ;
#65509=CARTESIAN_POINT('',(0.388527625421941,503.131344420871,-47.5221601717516)) ;
#65510=CARTESIAN_POINT('',(0.388527634359032,561.302123681176,-43.4900362557631)) ;
#65511=CARTESIAN_POINT('Origin',(-0.611472374578195,502.052123681177,-48.4900362557631)) ;
#65512=CARTESIAN_POINT('',(-0.611472374577496,506.335123681177,-43.4900362557631)) ;
#65513=CARTESIAN_POINT('',(-0.611472374577496,506.335123681177,-48.4900362557631)) ;
#65514=CARTESIAN_POINT('',(-0.611472374559588,616.077123681177,-43.4900362557631)) ;
#65515=CARTESIAN_POINT('',(-0.611472374559588,616.077123681177,-48.4900362557631)) ;
#65516=CARTESIAN_POINT('',(-0.611472374559506,616.57735283115,-43.4900362557631)) ;
#65517=CARTESIAN_POINT('',(-0.611472374578195,502.052123681177,-43.4900362557631)) ;
#65518=CARTESIAN_POINT('',(-0.611472374559505,616.585559486892,-19.5221601717515)) ;
#65519=CARTESIAN_POINT('Ctrl Pts',(-0.611472374559507,616.577352831186,
-43.4900362559989)) ;
#65520=CARTESIAN_POINT('Ctrl Pts',(-0.611472374559485,616.580300554184,
-42.8711455790505)) ;
#65521=CARTESIAN_POINT('Ctrl Pts',(-0.611472374559468,616.578645899186,
-42.2555490188023)) ;
#65522=CARTESIAN_POINT('Ctrl Pts',(-0.611472374559405,616.576796842089,
-40.3433653577621)) ;
#65523=CARTESIAN_POINT('Ctrl Pts',(-0.611472374559349,616.580239054546,
-39.0434564517781)) ;
#65524=CARTESIAN_POINT('Ctrl Pts',(-0.61147237455923,616.584223500474,-36.4426213256376)) ;
#65525=CARTESIAN_POINT('Ctrl Pts',(-0.611472374559168,616.584762379478,
-35.1426809282471)) ;
#65526=CARTESIAN_POINT('Ctrl Pts',(-0.611472374558881,616.586580540637,
-29.0698861297919)) ;
#65527=CARTESIAN_POINT('Ctrl Pts',(-0.611472374558661,616.585990493313,
-24.2959347172062)) ;
#65528=CARTESIAN_POINT('Ctrl Pts',(-0.611472374558452,616.585559486892,
-19.5221601717825)) ;
#65529=CARTESIAN_POINT('',(-0.611472374577577,505.835569713225,-19.5221601717515)) ;
#65530=CARTESIAN_POINT('',(-0.611472374577774,504.632344420872,-19.5221601717515)) ;
#65531=CARTESIAN_POINT('',(-0.611472374577577,505.835569713225,-43.4900362557631)) ;
#65532=CARTESIAN_POINT('',(-0.611472374577577,505.835569713225,-47.7060982137573)) ;
#65533=CARTESIAN_POINT('',(-0.611472374578195,502.052123681177,-43.4900362557631)) ;
#65534=CARTESIAN_POINT('Origin',(-283.146192374579,616.710565160617,-47.5221601717387)) ;
#65535=CARTESIAN_POINT('',(140.388527625421,616.710565160543,-49.5221601717579)) ;
#65536=CARTESIAN_POINT('Origin',(140.388527625421,616.710565160543,-47.5221601717579)) ;
#65537=CARTESIAN_POINT('',(-0.611472374578952,616.710565160567,-49.5221601717515)) ;
#65538=CARTESIAN_POINT('Origin',(-283.146192374579,616.710565160617,-47.5221601717387)) ;
#65539=CARTESIAN_POINT('',(205.668527625421,616.710565160531,-49.5221601717609)) ;
#65540=CARTESIAN_POINT('',(-0.611472374578952,616.710565160567,-49.5221601717515)) ;
#65541=CARTESIAN_POINT('Origin',(205.668527625421,616.710565160531,-47.5221601717609)) ;
#65542=CARTESIAN_POINT('Origin',(-283.146192374598,505.710565160617,-47.5221601717387)) ;
#65543=CARTESIAN_POINT('',(205.668527625402,505.710565160531,-49.5221601717609)) ;
#65544=CARTESIAN_POINT('Origin',(205.668527625402,505.710565160531,-47.5221601717609)) ;
#65545=CARTESIAN_POINT('',(-0.611472374598421,505.710565160567,-49.5221601717515)) ;
#65546=CARTESIAN_POINT('Origin',(212.388527625402,506.21056516053,-47.0221601717613)) ;
#65547=CARTESIAN_POINT('',(193.688527625402,506.210565160533,-47.5221601717604)) ;
#65548=CARTESIAN_POINT('Origin',(193.688527625402,506.210565160533,-47.0221601717604)) ;
#65549=CARTESIAN_POINT('',(0.388527630175977,506.210565160568,-47.5221601717516)) ;
#65550=CARTESIAN_POINT('',(212.388527625402,506.210565160531,-47.5221601717613)) ;
#65551=CARTESIAN_POINT('Origin',(0.388527634348712,506.210565160567,-47.0221601717516)) ;
#65552=CARTESIAN_POINT('Origin',(-2.61147237459646,504.210565160568,0.477839828248552)) ;
#65553=CARTESIAN_POINT('',(-2.61147237459865,503.131344420872,-43.4900362557631)) ;
#65554=CARTESIAN_POINT('Origin',(-2.61147237459681,507.212565160568,-19.5221601717514)) ;
#65555=CARTESIAN_POINT('',(-2.61147237457763,616.585559486893,-19.5221601717514)) ;
#65556=CARTESIAN_POINT('',(-0.611472374559505,616.585559486893,-19.5221601717515)) ;
#65557=CARTESIAN_POINT('',(-2.61147237459708,505.835569713225,-19.5221601717514)) ;
#65558=CARTESIAN_POINT('',(-2.6114723745971,505.711565160568,-19.5221601717514)) ;
#65559=CARTESIAN_POINT('',(-1.31147237459708,505.835569713225,-19.5221601717515)) ;
#65560=CARTESIAN_POINT('Origin',(-0.0114723745983569,505.835569713225,-46.9221601717515)) ;
#65561=CARTESIAN_POINT('',(-2.61147237459817,505.835569713225,-43.4900362557631)) ;
#65562=CARTESIAN_POINT('',(-2.81147237458794,505.835569713225,-43.4900362557631)) ;
#65563=CARTESIAN_POINT('',(-2.61147237459725,505.835569713225,-23.2221601717514)) ;
#65564=CARTESIAN_POINT('Ctrl Pts',(-2.6427223745788,616.576179137963,-43.6993995739517)) ;
#65565=CARTESIAN_POINT('Ctrl Pts',(0.327277625449208,616.576179137963,-43.6993995739518)) ;
#65566=CARTESIAN_POINT('Ctrl Pts',(-2.6427223745788,616.576400591684,-43.6645773254828)) ;
#65567=CARTESIAN_POINT('Ctrl Pts',(0.327277625449208,616.576400591684,-43.6645773254829)) ;
#65568=CARTESIAN_POINT('Ctrl Pts',(-2.6427223745788,616.576612329461,-43.6297316873501)) ;
#65569=CARTESIAN_POINT('Ctrl Pts',(0.327277625449208,616.576612329461,-43.6297316873502)) ;
#65570=CARTESIAN_POINT('Ctrl Pts',(-2.6427223745788,616.576808621265,-43.5948637771549)) ;
#65571=CARTESIAN_POINT('Ctrl Pts',(0.327277625449208,616.576808621265,-43.594863777155)) ;
#65572=CARTESIAN_POINT('Ctrl Pts',(-2.6427223745788,616.577000756849,-43.5607341490021)) ;
#65573=CARTESIAN_POINT('Ctrl Pts',(0.327277625449208,616.577000756849,-43.5607341490022)) ;
#65574=CARTESIAN_POINT('Ctrl Pts',(-2.64272237457879,616.577177913241,-43.5266148439379)) ;
#65575=CARTESIAN_POINT('Ctrl Pts',(0.327277625449218,616.577177913241,-43.526614843938)) ;
#65576=CARTESIAN_POINT('Ctrl Pts',(-2.64272237457879,616.577341045865,-43.4925055365579)) ;
#65577=CARTESIAN_POINT('Ctrl Pts',(0.327277625449218,616.577341045865,-43.492505536558)) ;
#65578=CARTESIAN_POINT('Ctrl Pts',(-2.64272237457877,616.580304957246,-42.8727829948047)) ;
#65579=CARTESIAN_POINT('Ctrl Pts',(0.327277625449238,616.580304957246,-42.8727829948048)) ;
#65580=CARTESIAN_POINT('Ctrl Pts',(-2.64272237457875,616.578646689173,-42.2563659747035)) ;
#65581=CARTESIAN_POINT('Ctrl Pts',(0.327277625449258,616.578646689173,-42.2563659747036)) ;
#65582=CARTESIAN_POINT('Ctrl Pts',(-2.64272237457873,616.5780518982,-41.6412689173054)) ;
#65583=CARTESIAN_POINT('Ctrl Pts',(0.327277625449278,616.5780518982,-41.6412689173055)) ;
#65584=CARTESIAN_POINT('Ctrl Pts',(-2.64272237457869,616.576796842089,-40.343365357762)) ;
#65585=CARTESIAN_POINT('Ctrl Pts',(0.327277625449318,616.576796842089,-40.3433653577621)) ;
#65586=CARTESIAN_POINT('Ctrl Pts',(-2.64272237457863,616.580239054546,-39.043456451778)) ;
#65587=CARTESIAN_POINT('Ctrl Pts',(0.327277625449378,616.580239054546,-39.0434564517781)) ;
#65588=CARTESIAN_POINT('Ctrl Pts',(-2.64272237457858,616.58223127751,-37.7430388887073)) ;
#65589=CARTESIAN_POINT('Ctrl Pts',(0.327277625449428,616.58223127751,-37.7430388887074)) ;
#65590=CARTESIAN_POINT('Ctrl Pts',(-2.64272237457852,616.584223500474,-36.4426213256375)) ;
#65591=CARTESIAN_POINT('Ctrl Pts',(0.327277625449487,616.584223500474,-36.4426213256376)) ;
#65592=CARTESIAN_POINT('Ctrl Pts',(-2.64272237457845,616.584762379478,-35.1426809282471)) ;
#65593=CARTESIAN_POINT('Ctrl Pts',(0.327277625449558,616.584762379478,-35.1426809282472)) ;
#65594=CARTESIAN_POINT('Ctrl Pts',(-2.64272237457839,616.585151546832,-33.8428327434185)) ;
#65595=CARTESIAN_POINT('Ctrl Pts',(0.327277625449618,616.585151546832,-33.8428327434186)) ;
#65596=CARTESIAN_POINT('Ctrl Pts',(-2.64272237457817,616.586580545288,-29.0698705940761)) ;
#65597=CARTESIAN_POINT('Ctrl Pts',(0.327277625449838,616.586580545288,-29.0698705940762)) ;
#65598=CARTESIAN_POINT('Ctrl Pts',(-2.64272237457795,616.585990489473,-24.2959036392336)) ;
#65599=CARTESIAN_POINT('Ctrl Pts',(0.327277625450058,616.585990489473,-24.2959036392337)) ;
#65600=CARTESIAN_POINT('Ctrl Pts',(-2.64272237457774,616.585559482684,-19.5221135565507)) ;
#65601=CARTESIAN_POINT('Ctrl Pts',(0.327277625450268,616.585559482684,-19.5221135565508)) ;
#65602=CARTESIAN_POINT('Ctrl Pts',(-2.64272237457773,616.585553230033,-19.4528597904909)) ;
#65603=CARTESIAN_POINT('Ctrl Pts',(0.327277625450278,616.585553230033,-19.452859790491)) ;
#65604=CARTESIAN_POINT('Ctrl Pts',(-2.64272237457773,616.585547010851,-19.3836060616588)) ;
#65605=CARTESIAN_POINT('Ctrl Pts',(0.327277625450278,616.585547010851,-19.3836060616589)) ;
#65606=CARTESIAN_POINT('Ctrl Pts',(-2.64272237457773,616.585540831787,-19.3143523736628)) ;
#65607=CARTESIAN_POINT('Ctrl Pts',(0.327277625450278,616.585540831787,-19.3143523736629)) ;
#65608=CARTESIAN_POINT('',(-2.61147237457872,616.57735283115,-43.4900362557631)) ;
#65609=CARTESIAN_POINT('',(-0.611472374559506,616.57735283115,-43.4900362557633)) ;
#65610=CARTESIAN_POINT('Ctrl Pts',(-2.61147237457763,616.585559486893,-19.5221601717514)) ;
#65611=CARTESIAN_POINT('Ctrl Pts',(-2.61147237457784,616.585990493314,-24.2959347171855)) ;
#65612=CARTESIAN_POINT('Ctrl Pts',(-2.61147237457806,616.586580540637,-29.0698861297815)) ;
#65613=CARTESIAN_POINT('Ctrl Pts',(-2.61147237457834,616.584762379478,-35.1426809282471)) ;
#65614=CARTESIAN_POINT('Ctrl Pts',(-2.61147237457841,616.584223500474,-36.4426213256375)) ;
#65615=CARTESIAN_POINT('Ctrl Pts',(-2.61147237457852,616.580239054546,-39.043456451778)) ;
#65616=CARTESIAN_POINT('Ctrl Pts',(-2.61147237457858,616.576796842089,-40.343365357762)) ;
#65617=CARTESIAN_POINT('Ctrl Pts',(-2.61147237457864,616.578645899187,-42.2555490187243)) ;
#65618=CARTESIAN_POINT('Ctrl Pts',(-2.61147237457866,616.580300554185,-42.8711455788942)) ;
#65619=CARTESIAN_POINT('Ctrl Pts',(-2.61147237457868,616.577352831188,-43.4900362557634)) ;
#65620=CARTESIAN_POINT('Origin',(-5.6114723745782,502.052123681177,-43.4900362557631)) ;
#65621=CARTESIAN_POINT('',(-2.61147237459808,506.335123681177,-43.4900362557631)) ;
#65622=CARTESIAN_POINT('',(-5.61147237457748,506.335123681177,-43.4900362557631)) ;
#65623=CARTESIAN_POINT('',(-2.61147237459865,503.131344420872,-43.4900362557631)) ;
#65624=CARTESIAN_POINT('Origin',(-5.61147237457746,506.335123681177,-48.4900362557631)) ;
#65625=CARTESIAN_POINT('',(0.388527634350065,506.335123681176,-49.5221601717516)) ;
#65626=CARTESIAN_POINT('',(103.388527625412,506.33512368116,-49.5221601717563)) ;
#65627=CARTESIAN_POINT('',(0.388527634350062,506.335123681176,-48.4900362557631)) ;
#65628=CARTESIAN_POINT('',(-2.6114723745972,506.335123681177,-24.0060982137574)) ;
#65629=CARTESIAN_POINT('Origin',(0.388527634368701,620.552123681176,-48.4900362557631)) ;
#65630=CARTESIAN_POINT('',(0.388527625421941,503.131344420871,-47.5221601717516)) ;
#65631=CARTESIAN_POINT('',(0.388527634349961,505.710565160567,-49.5221601717516)) ;
#65632=CARTESIAN_POINT('',(0.38852763435921,562.381344420871,-49.5221601717516)) ;
#65633=CARTESIAN_POINT('Origin',(0.38852763434857,505.710565160567,-47.5221601717516)) ;
#65634=CARTESIAN_POINT('',(0.388527634359032,561.302123681176,-43.4900362557631)) ;
#65635=CARTESIAN_POINT('Origin',(-5.6114723745782,502.052123681177,-43.4900362557631)) ;
#65636=CARTESIAN_POINT('Origin',(-5.6114723745782,502.052123681177,-43.4900362557631)) ;
#65637=CARTESIAN_POINT('',(-2.61147237459865,503.131344420872,-43.4900362557631)) ;
#65638=CARTESIAN_POINT('Origin',(-5.61147237457896,616.077123681177,-48.4900362557631)) ;
#65639=CARTESIAN_POINT('',(103.38852762542,616.07712368116,-49.5221601717563)) ;
#65640=CARTESIAN_POINT('',(-2.61147237457881,616.077123681177,-43.4900362557631)) ;
#65641=CARTESIAN_POINT('',(-2.61147237457792,616.077123681177,-24.0060982137574)) ;
#65642=CARTESIAN_POINT('',(-5.61147237456928,616.077123681177,-43.4900362557631)) ;
#65643=CARTESIAN_POINT('Origin',(-5.6114723745782,502.052123681177,-43.4900362557631)) ;
#65644=CARTESIAN_POINT('',(-2.61147237459865,503.131344420872,-43.4900362557631)) ;
#65645=CARTESIAN_POINT('Origin',(174.388527625403,506.710565160537,-20.8221601717595)) ;
#65646=CARTESIAN_POINT('',(173.388527625403,506.710565160537,-30.2221601717594)) ;
#65647=CARTESIAN_POINT('Origin',(174.388527625403,506.710565160537,-30.2221601717595)) ;
#65648=CARTESIAN_POINT('',(173.388527625403,506.710565160537,-25.7721601717594)) ;
#65649=CARTESIAN_POINT('',(173.388527625403,506.710565160537,-20.8221601717595)) ;
#65650=CARTESIAN_POINT('Origin',(174.388527625403,506.710565160537,-25.7721601717595)) ;
#65651=CARTESIAN_POINT('Origin',(173.388527625402,504.210565160537,-42.1221601717595)) ;
#65652=CARTESIAN_POINT('',(173.388527625403,506.960565160537,-30.2221601717594)) ;
#65653=CARTESIAN_POINT('',(173.388527625403,506.210565160537,-30.2221601717594)) ;
#65654=CARTESIAN_POINT('',(173.388527625403,506.960565160537,-25.7721601717594)) ;
#65655=CARTESIAN_POINT('',(173.388527625402,506.960565160537,-45.8221601717595)) ;
#65656=CARTESIAN_POINT('',(173.388527625403,506.210565160537,-25.7721601717594)) ;
#65657=CARTESIAN_POINT('Origin',(84.9885276254035,506.710565160552,-11.8221601717554)) ;
#65658=CARTESIAN_POINT('',(85.9885276254023,506.710565160552,-38.1221601717554)) ;
#65659=CARTESIAN_POINT('Origin',(84.9885276254023,506.710565160552,-38.1221601717554)) ;
#65660=CARTESIAN_POINT('',(85.9885276254028,506.710565160552,-25.7721601717555)) ;
#65661=CARTESIAN_POINT('Origin',(84.9885276254028,506.710565160552,-25.7721601717554)) ;
#65662=CARTESIAN_POINT('',(85.9885276254035,506.710565160552,-11.8221601717555)) ;
#65663=CARTESIAN_POINT('Origin',(89.9885276254023,506.710565160552,-38.1221601717556)) ;
#65664=CARTESIAN_POINT('',(89.9885276254021,506.710565160552,-42.122160469427)) ;
#65665=CARTESIAN_POINT('Origin',(89.988527625402,506.710565160552,-43.1221601717556)) ;
#65666=CARTESIAN_POINT('Origin',(89.9885276254023,506.710565160552,-38.1221601717556)) ;
#65667=CARTESIAN_POINT('Origin',(158.688527625402,506.710565160539,-43.1221607671016)) ;
#65668=CARTESIAN_POINT('',(169.388527625402,506.710565160538,-42.1221604694307)) ;
#65669=CARTESIAN_POINT('Origin',(169.388527625402,506.710565160538,-43.122160767102)) ;
#65670=CARTESIAN_POINT('',(158.688527625402,506.710565160539,-42.1221607671016)) ;
#65671=CARTESIAN_POINT('Origin',(169.388527625402,506.710565160538,-38.1221601717593)) ;
#65672=CARTESIAN_POINT('',(173.388527625402,506.710565160537,-38.1221601717594)) ;
#65673=CARTESIAN_POINT('Origin',(174.388527625402,506.710565160537,-38.1221601717595)) ;
#65674=CARTESIAN_POINT('Origin',(169.388527625402,506.710565160538,-38.1221601717593)) ;
#65675=CARTESIAN_POINT('Origin',(174.388527625403,506.710565160537,-20.8221601717595)) ;
#65676=CARTESIAN_POINT('',(173.388527625402,506.710565160537,-37.2221601717594)) ;
#65677=CARTESIAN_POINT('Origin',(174.388527625402,506.710565160537,-37.2221601717595)) ;
#65678=CARTESIAN_POINT('',(173.388527625403,506.710565160537,-20.8221601717595)) ;
#65679=CARTESIAN_POINT('Origin',(173.388527625402,504.210565160537,-42.1221601717595)) ;
#65680=CARTESIAN_POINT('',(173.388527625402,506.960565160537,-38.1221601717594)) ;
#65681=CARTESIAN_POINT('',(173.388527625402,507.460565160537,-38.1221601717594)) ;
#65682=CARTESIAN_POINT('',(173.388527625402,506.960565160537,-37.2221601717594)) ;
#65683=CARTESIAN_POINT('',(173.388527625402,506.960565160537,-45.8221601717595)) ;
#65684=CARTESIAN_POINT('',(173.388527625402,507.460565160537,-37.2221601717594)) ;
#65685=CARTESIAN_POINT('Origin',(169.388527625376,354.701436995038,-38.1221601717593)) ;
#65686=CARTESIAN_POINT('',(169.388527625402,506.960565160538,-42.1221604694306)) ;
#65687=CARTESIAN_POINT('',(169.388527625402,506.210565160538,-42.1221601717592)) ;
#65688=CARTESIAN_POINT('Origin',(169.388527625402,506.960565160538,-38.1221601717593)) ;
#65689=CARTESIAN_POINT('Origin',(104.988527625411,561.210565160549,-42.1221607670991)) ;
#65690=CARTESIAN_POINT('',(89.9885276254021,506.960565160552,-42.1221604694269)) ;
#65691=CARTESIAN_POINT('',(89.9885276254479,767.719724046651,-42.1221607670984)) ;
#65692=CARTESIAN_POINT('',(158.688527625402,506.960565160539,-42.1221607671016)) ;
#65693=CARTESIAN_POINT('Origin',(89.9885276254481,767.719724046652,-38.1221601717556)) ;
#65694=CARTESIAN_POINT('',(85.9885276254023,506.960565160552,-38.1221601717554)) ;
#65695=CARTESIAN_POINT('',(85.9885276254022,506.210565160552,-38.1221601717555)) ;
#65696=CARTESIAN_POINT('Origin',(89.9885276254023,506.960565160551,-38.1221601717556)) ;
#65697=CARTESIAN_POINT('Origin',(85.9885276254025,504.210565160552,-24.1221601717555)) ;
#65698=CARTESIAN_POINT('',(85.9885276254028,506.960565160552,-25.7721601717555)) ;
#65699=CARTESIAN_POINT('',(85.9885276254027,506.210565160552,-25.7721601717555)) ;
#65700=CARTESIAN_POINT('',(85.9885276254024,506.960565160552,-36.8221601717555)) ;
#65701=CARTESIAN_POINT('Origin',(127.688527625422,615.710565160545,-36.8221601717574)) ;
#65702=CARTESIAN_POINT('',(126.688527625421,615.710565160545,-38.1221601717573)) ;
#65703=CARTESIAN_POINT('Origin',(127.688527625421,615.710565160545,-38.1221601717573)) ;
#65704=CARTESIAN_POINT('',(126.688527625422,615.710565160545,-25.7721601717573)) ;
#65705=CARTESIAN_POINT('Origin',(127.688527625422,615.710565160545,-25.7721601717573)) ;
#65706=CARTESIAN_POINT('',(126.688527625422,615.710565160545,-36.8221601717573)) ;
#65707=CARTESIAN_POINT('Origin',(122.688527625421,615.710565160546,-38.1221601717571)) ;
#65708=CARTESIAN_POINT('',(122.688527625421,615.710565160546,-42.1221604694271)) ;
#65709=CARTESIAN_POINT('Origin',(122.688527625421,615.710565160546,-43.1221601717571)) ;
#65710=CARTESIAN_POINT('Origin',(122.688527625421,615.710565160546,-38.1221601717571)) ;
#65711=CARTESIAN_POINT('Origin',(158.688527625421,615.710565160539,-43.1221607670988)) ;
#65712=CARTESIAN_POINT('',(99.6885276254213,615.71056516055,-42.1221604694261)) ;
#65713=CARTESIAN_POINT('Origin',(99.6885276254212,615.71056516055,-43.1221607670961)) ;
#65714=CARTESIAN_POINT('',(158.688527625421,615.710565160539,-42.1221607670988)) ;
#65715=CARTESIAN_POINT('Origin',(99.6885276254214,615.71056516055,-38.1221601717561)) ;
#65716=CARTESIAN_POINT('',(95.6885276254214,615.71056516055,-38.1221601717559)) ;
#65717=CARTESIAN_POINT('Origin',(94.6885276254214,615.710565160551,-38.1221601717558)) ;
#65718=CARTESIAN_POINT('Origin',(99.6885276254214,615.71056516055,-38.1221601717561)) ;
#65719=CARTESIAN_POINT('Origin',(94.6885276254211,615.710565160551,-45.8221601717558)) ;
#65720=CARTESIAN_POINT('',(95.688527625422,615.71056516055,-25.7721601717559)) ;
#65721=CARTESIAN_POINT('Origin',(94.688527625422,615.710565160551,-25.7721601717558)) ;
#65722=CARTESIAN_POINT('',(95.6885276254211,615.71056516055,-45.8221601717559)) ;
#65723=CARTESIAN_POINT('Origin',(95.6885276254217,618.21056516055,-42.1221601717559)) ;
#65724=CARTESIAN_POINT('',(95.6885276254213,615.460565160551,-38.1221601717559)) ;
#65725=CARTESIAN_POINT('',(95.6885276254212,614.960565160551,-38.1221601717559)) ;
#65726=CARTESIAN_POINT('',(95.6885276254219,615.460565160551,-25.7721601717559)) ;
#65727=CARTESIAN_POINT('',(95.688527625421,615.460565160551,-45.8221601717559)) ;
#65728=CARTESIAN_POINT('',(95.6885276254174,589.898065160551,-25.7721601717559)) ;
#65729=CARTESIAN_POINT('Origin',(99.6885276254481,767.71972404665,-38.122160171756)) ;
#65730=CARTESIAN_POINT('',(99.6885276254212,615.46056516055,-42.1221604694261)) ;
#65731=CARTESIAN_POINT('',(99.6885276254213,616.21056516055,-42.1221601717561)) ;
#65732=CARTESIAN_POINT('Origin',(99.6885276254213,615.46056516055,-38.1221601717561)) ;
#65733=CARTESIAN_POINT('Origin',(104.988527625411,561.210565160549,-42.1221607670963)) ;
#65734=CARTESIAN_POINT('',(122.688527625421,615.460565160546,-42.1221604694271)) ;
#65735=CARTESIAN_POINT('',(122.688527625375,354.701436995046,-42.1221607670972)) ;
#65736=CARTESIAN_POINT('',(158.688527625421,615.460565160539,-42.1221607670988)) ;
#65737=CARTESIAN_POINT('Origin',(122.688527625376,354.701436995046,-38.1221601717572)) ;
#65738=CARTESIAN_POINT('',(126.688527625421,615.460565160545,-38.1221601717573)) ;
#65739=CARTESIAN_POINT('',(126.688527625422,616.210565160545,-38.1221601717573)) ;
#65740=CARTESIAN_POINT('Origin',(122.688527625421,615.460565160546,-38.1221601717571)) ;
#65741=CARTESIAN_POINT('Origin',(126.688527625423,618.210565160545,-24.1221601717573)) ;
#65742=CARTESIAN_POINT('',(126.688527625422,615.460565160545,-25.7721601717573)) ;
#65743=CARTESIAN_POINT('',(126.688527625417,589.898065160545,-25.7721601717573)) ;
#65744=CARTESIAN_POINT('',(126.688527625421,615.460565160545,-36.8221601717573)) ;
#65745=CARTESIAN_POINT('Origin',(94.8885276254124,564.535138680008,-46.5221601717561)) ;
#65746=CARTESIAN_POINT('',(97.6385276254124,566.122851920279,-47.522160171756)) ;
#65747=CARTESIAN_POINT('',(94.8885276254124,564.535138680008,-47.5221601717559)) ;
#65748=CARTESIAN_POINT('',(125.890374340326,582.434063226238,-47.5221601717573)) ;
#65749=CARTESIAN_POINT('',(97.6385276254124,566.122851920279,-49.522160171756)) ;
#65750=CARTESIAN_POINT('',(97.6385276254124,566.122851920279,-46.772160171756)) ;
#65751=CARTESIAN_POINT('',(94.8885276254124,564.535138680008,-49.5221601717559)) ;
#65752=CARTESIAN_POINT('',(125.890374340326,582.434063226239,-49.5221601717573)) ;
#65753=CARTESIAN_POINT('',(94.8885276254124,564.535138680008,-46.5221601717561)) ;
#65754=CARTESIAN_POINT('Origin',(92.1385276254124,566.122851920279,-46.522160171756)) ;
#65755=CARTESIAN_POINT('',(92.1385276254124,566.122851920279,-47.5221601717558)) ;
#65756=CARTESIAN_POINT('',(150.636680910491,532.348927374043,-47.5221601717585)) ;
#65757=CARTESIAN_POINT('',(92.1385276254124,566.122851920279,-49.5221601717558)) ;
#65758=CARTESIAN_POINT('',(150.636680910491,532.348927374043,-49.5221601717584)) ;
#65759=CARTESIAN_POINT('',(92.1385276254124,566.122851920279,-46.772160171756)) ;
#65760=CARTESIAN_POINT('Origin',(92.1385276254124,569.298278400822,-46.5221601717557)) ;
#65761=CARTESIAN_POINT('',(92.1385276254124,569.298278400822,-47.5221601717558)) ;
#65762=CARTESIAN_POINT('',(92.1385276254124,536.754421780676,-47.5221601717558)) ;
#65763=CARTESIAN_POINT('',(92.1385276254124,569.298278400822,-49.5221601717558)) ;
#65764=CARTESIAN_POINT('',(92.1385276254124,536.754421780676,-49.5221601717558)) ;
#65765=CARTESIAN_POINT('',(92.1385276254124,569.298278400822,-46.7721601717557)) ;
#65766=CARTESIAN_POINT('Origin',(94.8885276254124,570.885991641093,-46.5221601717556)) ;
#65767=CARTESIAN_POINT('',(94.8885276254124,570.885991641094,-47.5221601717559)) ;
#65768=CARTESIAN_POINT('',(124.515374340326,587.991059567189,-47.5221601717573)) ;
#65769=CARTESIAN_POINT('',(94.8885276254124,570.885991641094,-49.5221601717559)) ;
#65770=CARTESIAN_POINT('',(124.515374340326,587.991059567189,-49.5221601717572)) ;
#65771=CARTESIAN_POINT('',(94.8885276254124,570.885991641093,-46.5221601717556)) ;
#65772=CARTESIAN_POINT('Origin',(97.6385276254124,566.122851920279,-46.522160171756)) ;
#65773=CARTESIAN_POINT('',(97.6385276254124,569.298278400822,-47.522160171756)) ;
#65774=CARTESIAN_POINT('',(97.6385276254125,535.166708540405,-47.522160171756)) ;
#65775=CARTESIAN_POINT('',(97.6385276254124,569.298278400822,-49.522160171756)) ;
#65776=CARTESIAN_POINT('',(97.6385276254124,569.298278400822,-46.7721601717557)) ;
#65777=CARTESIAN_POINT('',(97.6385276254125,535.166708540405,-49.522160171756)) ;
#65778=CARTESIAN_POINT('Origin',(97.6385276254124,569.298278400822,-46.5221601717557)) ;
#65779=CARTESIAN_POINT('',(154.761680910491,536.318210474722,-47.5221601717586)) ;
#65780=CARTESIAN_POINT('',(154.761680910491,536.318210474722,-49.5221601717586)) ;
#65781=CARTESIAN_POINT('Origin',(184.888527625403,510.035138679992,-46.5221601717602)) ;
#65782=CARTESIAN_POINT('',(187.638527625403,511.622851920263,-47.5221601717601)) ;
#65783=CARTESIAN_POINT('',(184.888527625403,510.035138679992,-47.52216017176)) ;
#65784=CARTESIAN_POINT('',(193.939970466886,515.260991641077,-47.5221601717604)) ;
#65785=CARTESIAN_POINT('',(187.638527625403,511.622851920264,-49.5221601717601)) ;
#65786=CARTESIAN_POINT('',(187.638527625403,511.622851920263,-46.7721601717601)) ;
#65787=CARTESIAN_POINT('',(184.888527625403,510.035138679992,-49.52216017176)) ;
#65788=CARTESIAN_POINT('',(193.939970466886,515.260991641077,-49.5221601717604)) ;
#65789=CARTESIAN_POINT('',(184.888527625403,510.035138679992,-46.5221601717602)) ;
#65790=CARTESIAN_POINT('Origin',(182.138527625403,511.622851920263,-46.5221601717601)) ;
#65791=CARTESIAN_POINT('',(182.138527625403,511.622851920263,-47.5221601717599)) ;
#65792=CARTESIAN_POINT('',(195.087084783918,504.146998959177,-47.5221601717605)) ;
#65793=CARTESIAN_POINT('',(182.138527625403,511.622851920264,-49.5221601717599)) ;
#65794=CARTESIAN_POINT('',(195.087084783918,504.146998959177,-49.5221601717605)) ;
#65795=CARTESIAN_POINT('',(182.138527625403,511.622851920263,-46.7721601717601)) ;
#65796=CARTESIAN_POINT('Origin',(182.138527625403,514.798278400806,-46.5221601717598)) ;
#65797=CARTESIAN_POINT('',(182.138527625403,514.798278400806,-47.5221601717599)) ;
#65798=CARTESIAN_POINT('',(182.138527625403,509.504421780668,-47.5221601717599)) ;
#65799=CARTESIAN_POINT('',(182.138527625403,514.798278400806,-49.5221601717599)) ;
#65800=CARTESIAN_POINT('',(182.138527625403,509.504421780668,-49.5221601717599)) ;
#65801=CARTESIAN_POINT('',(182.138527625403,514.798278400806,-46.7721601717598)) ;
#65802=CARTESIAN_POINT('Origin',(184.888527625403,516.385991641078,-46.5221601717597)) ;
#65803=CARTESIAN_POINT('',(184.888527625403,516.385991641078,-47.52216017176)) ;
#65804=CARTESIAN_POINT('',(192.564970466886,520.817987982027,-47.5221601717604)) ;
#65805=CARTESIAN_POINT('',(184.888527625403,516.385991641078,-49.52216017176)) ;
#65806=CARTESIAN_POINT('',(192.564970466886,520.817987982027,-49.5221601717603)) ;
#65807=CARTESIAN_POINT('',(184.888527625403,516.385991641078,-46.5221601717597)) ;
#65808=CARTESIAN_POINT('Origin',(187.638527625403,511.622851920263,-46.5221601717601)) ;
#65809=CARTESIAN_POINT('',(187.638527625403,514.798278400806,-47.5221601717601)) ;
#65810=CARTESIAN_POINT('',(187.638527625403,507.916708540397,-47.5221601717601)) ;
#65811=CARTESIAN_POINT('',(187.638527625403,514.798278400806,-49.5221601717601)) ;
#65812=CARTESIAN_POINT('',(187.638527625403,514.798278400806,-46.7721601717598)) ;
#65813=CARTESIAN_POINT('',(187.638527625403,507.916708540397,-49.5221601717601)) ;
#65814=CARTESIAN_POINT('Origin',(187.638527625403,514.798278400806,-46.5221601717598)) ;
#65815=CARTESIAN_POINT('',(199.212084783918,508.116282059856,-47.5221601717607)) ;
#65816=CARTESIAN_POINT('',(199.212084783918,508.116282059856,-49.5221601717607)) ;
#65817=CARTESIAN_POINT('Origin',(-2.61147237459646,504.210565160568,0.477839828248552)) ;
#65818=CARTESIAN_POINT('Origin',(-2.61147237459646,504.210565160568,0.477839828248552)) ;
#65819=CARTESIAN_POINT('Origin',(212.388527625421,616.21056516053,-47.0221601717612)) ;
#65820=CARTESIAN_POINT('',(148.388527625421,616.210565160541,-47.5221601717583)) ;
#65821=CARTESIAN_POINT('Origin',(148.388527625421,616.210565160541,-47.0221601717583)) ;
#65822=CARTESIAN_POINT('',(144.388527625421,616.210565160542,-47.5221601717581)) ;
#65823=CARTESIAN_POINT('Origin',(144.388527625421,616.210565160542,-47.0221601717582)) ;
#65824=CARTESIAN_POINT('',(212.388527625421,616.21056516053,-47.5221601717612)) ;
#65825=CARTESIAN_POINT('Origin',(212.388527625402,506.21056516053,-47.0221601717613)) ;
#65826=CARTESIAN_POINT('',(197.688527625402,506.210565160533,-47.5221601717606)) ;
#65827=CARTESIAN_POINT('Origin',(197.688527625402,506.210565160533,-47.0221601717606)) ;
#65828=CARTESIAN_POINT('',(201.668527625402,506.210565160532,-47.5221601717607)) ;
#65829=CARTESIAN_POINT('Origin',(201.668527625402,506.210565160532,-47.0221601717608)) ;
#65830=CARTESIAN_POINT('',(212.388527625402,506.21056516053,-47.5221601717613)) ;
#65831=CARTESIAN_POINT('Origin',(212.388527625402,506.21056516053,-47.0221601717613)) ;
#65832=CARTESIAN_POINT('',(205.668527625402,506.210565160531,-47.5221601717609)) ;
#65833=CARTESIAN_POINT('',(212.388527625402,506.21056516053,-47.5221601717613)) ;
#65834=CARTESIAN_POINT('Origin',(205.668527625402,506.210565160531,-47.022160171761)) ;
#65835=CARTESIAN_POINT('Origin',(212.388527625421,616.21056516053,-47.0221601717612)) ;
#65836=CARTESIAN_POINT('',(201.668527625421,616.210565160532,-47.5221601717607)) ;
#65837=CARTESIAN_POINT('Origin',(201.668527625421,616.210565160532,-47.0221601717608)) ;
#65838=CARTESIAN_POINT('',(197.688527625421,616.210565160533,-47.5221601717605)) ;
#65839=CARTESIAN_POINT('Origin',(197.688527625421,616.210565160533,-47.0221601717606)) ;
#65840=CARTESIAN_POINT('',(212.388527625421,616.21056516053,-47.5221601717612)) ;
#65841=CARTESIAN_POINT('Origin',(212.388527625421,616.21056516053,-47.0221601717612)) ;
#65842=CARTESIAN_POINT('',(152.388527625421,616.210565160541,-47.5221601717585)) ;
#65843=CARTESIAN_POINT('Origin',(152.388527625421,616.210565160541,-47.0221601717585)) ;
#65844=CARTESIAN_POINT('',(193.688527625421,616.210565160533,-47.5221601717603)) ;
#65845=CARTESIAN_POINT('',(212.388527625421,616.21056516053,-47.5221601717612)) ;
#65846=CARTESIAN_POINT('Origin',(193.688527625421,616.210565160533,-47.0221601717604)) ;
#65847=CARTESIAN_POINT('Origin',(140.388527625421,618.210565160543,-49.5221601717579)) ;
#65848=CARTESIAN_POINT('',(140.38852762542,612.710565160543,-47.5221601717579)) ;
#65849=CARTESIAN_POINT('',(140.38852762542,612.710565160543,-47.5221601717579)) ;
#65850=CARTESIAN_POINT('',(140.38852762542,612.710565160543,-49.5221601717579)) ;
#65851=CARTESIAN_POINT('',(140.38852762542,612.710565160543,-49.5221601717579)) ;
#65852=CARTESIAN_POINT('',(140.388527625421,616.710565160543,-49.5221601717579)) ;
#65853=CARTESIAN_POINT('',(140.388527625422,616.210565160543,-28.5221601717579)) ;
#65854=CARTESIAN_POINT('Origin',(187.388264603402,504.260565160534,-24.0203292412001)) ;
#65855=CARTESIAN_POINT('',(185.73826464091,504.810565160535,-24.0199774237433)) ;
#65856=CARTESIAN_POINT('Origin',(187.388264603403,504.810565160534,-24.0203292412001)) ;
#65857=CARTESIAN_POINT('',(185.188264653412,504.260565160534,-24.0198601512577)) ;
#65858=CARTESIAN_POINT('Origin',(187.388264603402,504.210565160534,-24.0203292412001)) ;
#65859=CARTESIAN_POINT('',(185.73826464091,504.210565160534,-24.0199774237433)) ;
#65860=CARTESIAN_POINT('Origin',(187.388264603422,618.160565160534,-24.0203292412001)) ;
#65861=CARTESIAN_POINT('',(187.382265311382,617.610565160534,-25.6703183346474)) ;
#65862=CARTESIAN_POINT('Origin',(187.388264603422,617.610565160534,-24.0203292412001)) ;
#65863=CARTESIAN_POINT('',(187.380265547368,618.160565160534,-26.2203146991298)) ;
#65864=CARTESIAN_POINT('Origin',(187.388264603422,618.210565160534,-24.0203292412001)) ;
#65865=CARTESIAN_POINT('',(187.382265311382,618.210565160534,-25.6703183346474)) ;
#65866=CARTESIAN_POINT('Origin',(6.48852762540227,504.260565160566,-24.0221601717538)) ;
#65867=CARTESIAN_POINT('',(4.83852762540237,504.810565160566,-24.0221601717538)) ;
#65868=CARTESIAN_POINT('Origin',(6.48852762540237,504.810565160566,-24.0221601717538)) ;
#65869=CARTESIAN_POINT('',(4.28852762540227,504.260565160566,-24.0221601717537)) ;
#65870=CARTESIAN_POINT('Origin',(6.48852762540226,504.210565160566,-24.0221601717538)) ;
#65871=CARTESIAN_POINT('',(4.83852762540226,504.210565160566,-24.0221601717537)) ;
#65872=CARTESIAN_POINT('Origin',(99.7385276254127,561.58556516055,-25.7721601717561)) ;
#65873=CARTESIAN_POINT('',(97.6885276254219,615.46056516055,-25.772160171756)) ;
#65874=CARTESIAN_POINT('',(149.488527625422,615.460565160541,-25.7721601717583)) ;
#65875=CARTESIAN_POINT('Origin',(94.4385276254219,615.460565160551,-25.7721601717558)) ;
#65876=CARTESIAN_POINT('Origin',(99.7385276254127,561.58556516055,-25.7721601717561)) ;
#65877=CARTESIAN_POINT('',(124.688527625422,615.460565160545,-25.7721601717572)) ;
#65878=CARTESIAN_POINT('',(149.488527625422,615.460565160541,-25.7721601717583)) ;
#65879=CARTESIAN_POINT('Origin',(127.938527625422,615.460565160545,-25.7721601717574)) ;
#65880=CARTESIAN_POINT('Origin',(111.188527625422,614.960565160548,-29.5221601717566)) ;
#65881=CARTESIAN_POINT('',(112.938527625421,613.460565160548,-29.5221601717567)) ;
#65882=CARTESIAN_POINT('Origin',(111.188527625421,613.460565160548,-29.5221601717566)) ;
#65883=CARTESIAN_POINT('',(112.938527625422,614.460565160548,-29.5221601717567)) ;
#65884=CARTESIAN_POINT('',(112.938527625422,614.960565160548,-29.5221601717567)) ;
#65885=CARTESIAN_POINT('',(111.188527625422,614.460565160548,-27.7721601717566)) ;
#65886=CARTESIAN_POINT('Origin',(111.188527625422,614.460565160548,-29.5221601717566)) ;
#65887=CARTESIAN_POINT('Origin',(111.188527625422,614.460565160548,-29.5221601717566)) ;
#65888=CARTESIAN_POINT('Origin',(111.188527625422,614.960565160548,-29.5221601717566)) ;
#65889=CARTESIAN_POINT('',(111.188527625422,615.460565160548,-26.7721601717566)) ;
#65890=CARTESIAN_POINT('',(111.188527625422,614.960565160548,-27.2721601717566)) ;
#65891=CARTESIAN_POINT('Origin',(111.188527625422,615.460565160548,-29.5221601717566)) ;
#65892=CARTESIAN_POINT('Origin',(195.688527625419,612.880565160533,-89.2041436556704)) ;
#65893=CARTESIAN_POINT('',(197.68852762542,612.880565160533,-47.5221601717605)) ;
#65894=CARTESIAN_POINT('',(193.68852762542,612.880565160533,-47.5221601717603)) ;
#65895=CARTESIAN_POINT('Origin',(195.68852762542,612.880565160533,-47.5221601717604)) ;
#65896=CARTESIAN_POINT('',(197.68852762542,612.880565160533,-49.5221601717605)) ;
#65897=CARTESIAN_POINT('',(197.68852762542,612.880565160533,-47.5221601717605)) ;
#65898=CARTESIAN_POINT('',(193.68852762542,612.880565160533,-49.5221601717603)) ;
#65899=CARTESIAN_POINT('Origin',(195.68852762542,612.880565160533,-49.5221601717604)) ;
#65900=CARTESIAN_POINT('',(193.68852762542,612.880565160533,-49.5221601717603)) ;
#65901=CARTESIAN_POINT('Origin',(203.668527625419,612.880565160532,-89.2041436556707)) ;
#65902=CARTESIAN_POINT('',(205.66852762542,612.880565160531,-47.5221601717609)) ;
#65903=CARTESIAN_POINT('',(201.66852762542,612.880565160532,-47.5221601717607)) ;
#65904=CARTESIAN_POINT('Origin',(203.66852762542,612.880565160532,-47.5221601717608)) ;
#65905=CARTESIAN_POINT('',(205.66852762542,612.880565160531,-49.5221601717609)) ;
#65906=CARTESIAN_POINT('',(205.66852762542,612.880565160531,-47.5221601717609)) ;
#65907=CARTESIAN_POINT('',(201.66852762542,612.880565160532,-49.5221601717607)) ;
#65908=CARTESIAN_POINT('Origin',(203.66852762542,612.880565160532,-49.5221601717608)) ;
#65909=CARTESIAN_POINT('',(201.66852762542,612.880565160532,-49.5221601717607)) ;
#65910=CARTESIAN_POINT('Origin',(203.668527625405,509.540565160532,19.9106552778092)) ;
#65911=CARTESIAN_POINT('',(205.668527625402,509.540565160531,-49.522160171761)) ;
#65912=CARTESIAN_POINT('',(201.668527625402,509.540565160532,-49.5221601717608)) ;
#65913=CARTESIAN_POINT('Origin',(203.668527625402,509.540565160532,-49.5221601717608)) ;
#65914=CARTESIAN_POINT('',(205.668527625402,509.540565160531,-47.5221601717609)) ;
#65915=CARTESIAN_POINT('',(205.668527625402,509.540565160531,-49.5221601717609)) ;
#65916=CARTESIAN_POINT('',(201.668527625402,509.540565160532,-47.5221601717607)) ;
#65917=CARTESIAN_POINT('Origin',(203.668527625402,509.540565160532,-47.5221601717608)) ;
#65918=CARTESIAN_POINT('',(201.668527625402,509.540565160532,-47.5221601717607)) ;
#65919=CARTESIAN_POINT('Origin',(195.688527625405,509.540565160533,19.9106552778095)) ;
#65920=CARTESIAN_POINT('',(197.688527625402,509.540565160533,-49.5221601717606)) ;
#65921=CARTESIAN_POINT('',(193.688527625402,509.540565160533,-49.5221601717604)) ;
#65922=CARTESIAN_POINT('Origin',(195.688527625402,509.540565160533,-49.5221601717605)) ;
#65923=CARTESIAN_POINT('',(197.688527625402,509.540565160533,-47.5221601717606)) ;
#65924=CARTESIAN_POINT('',(197.688527625402,509.540565160533,-49.5221601717606)) ;
#65925=CARTESIAN_POINT('',(193.688527625402,509.540565160533,-47.5221601717604)) ;
#65926=CARTESIAN_POINT('Origin',(195.688527625402,509.540565160533,-47.5221601717605)) ;
#65927=CARTESIAN_POINT('',(193.688527625402,509.540565160533,-47.5221601717604)) ;
#65928=CARTESIAN_POINT('Origin',(142.388527625419,612.710565160542,-88.630160171758)) ;
#65929=CARTESIAN_POINT('',(144.38852762542,612.710565160542,-49.5221601717581)) ;
#65930=CARTESIAN_POINT('Origin',(142.38852762542,612.710565160542,-49.522160171758)) ;
#65931=CARTESIAN_POINT('',(144.38852762542,612.710565160542,-47.5221601717581)) ;
#65932=CARTESIAN_POINT('Origin',(142.38852762542,612.710565160542,-47.522160171758)) ;
#65933=CARTESIAN_POINT('',(144.38852762542,612.710565160542,-47.5221601717581)) ;
#65934=CARTESIAN_POINT('Origin',(150.388527625419,612.710565160541,-88.6301601717583)) ;
#65935=CARTESIAN_POINT('',(152.38852762542,612.710565160541,-49.5221601717584)) ;
#65936=CARTESIAN_POINT('',(148.38852762542,612.710565160541,-49.5221601717583)) ;
#65937=CARTESIAN_POINT('Origin',(150.38852762542,612.710565160541,-49.5221601717583)) ;
#65938=CARTESIAN_POINT('',(148.38852762542,612.710565160541,-47.5221601717583)) ;
#65939=CARTESIAN_POINT('',(148.38852762542,612.710565160541,-49.5221601717583)) ;
#65940=CARTESIAN_POINT('',(152.38852762542,612.710565160541,-47.5221601717585)) ;
#65941=CARTESIAN_POINT('Origin',(150.38852762542,612.710565160541,-47.5221601717583)) ;
#65942=CARTESIAN_POINT('',(152.38852762542,612.710565160541,-47.5221601717585)) ;
#65943=CARTESIAN_POINT('Origin',(122.688527625421,615.460565160546,-38.1221601717571)) ;
#65944=CARTESIAN_POINT('',(124.688527625421,615.460565160545,-38.1221601717572)) ;
#65945=CARTESIAN_POINT('Origin',(127.938527625421,615.460565160545,-38.1221601717574)) ;
#65946=CARTESIAN_POINT('',(122.688527625421,615.460565160546,-40.1221601717571)) ;
#65947=CARTESIAN_POINT('Origin',(122.688527625421,615.460565160546,-43.3721601717571)) ;
#65948=CARTESIAN_POINT('Origin',(122.688527625421,615.460565160546,-38.1221601717571)) ;
#65949=CARTESIAN_POINT('Origin',(127.938527625421,615.460565160545,-38.6663657544474)) ;
#65950=CARTESIAN_POINT('Origin',(127.938527625422,615.460565160545,-24.1221601717574)) ;
#65951=CARTESIAN_POINT('',(124.688527625421,615.460565160545,-38.1221601726072)) ;
#65952=CARTESIAN_POINT('Origin',(150.388527625448,766.820965161141,-28.5221601717584)) ;
#65953=CARTESIAN_POINT('',(148.388527625422,616.210565160541,-28.5221601717583)) ;
#65954=CARTESIAN_POINT('',(152.388527625422,618.710565160541,-28.5221601717585)) ;
#65955=CARTESIAN_POINT('Origin',(195.688527625376,354.701436995033,-28.5221601717605)) ;
#65956=CARTESIAN_POINT('',(197.688527625422,618.710565160533,-28.5221601717605)) ;
#65957=CARTESIAN_POINT('',(193.688527625422,616.210565160533,-28.5221601717604)) ;
#65958=CARTESIAN_POINT('Origin',(203.668527625376,354.701436995032,-28.5221601717608)) ;
#65959=CARTESIAN_POINT('',(205.668527625422,618.710565160531,-28.5221601717609)) ;
#65960=CARTESIAN_POINT('',(201.668527625422,616.210565160532,-28.5221601717607)) ;
#65961=CARTESIAN_POINT('Origin',(-2.61147237459681,507.212565160568,-19.5221601717514)) ;
#65962=CARTESIAN_POINT('Origin',(142.388527625448,766.820965161142,-28.522160171758)) ;
#65963=CARTESIAN_POINT('',(144.388527625422,618.710565160542,-28.5221601717581)) ;
#65964=CARTESIAN_POINT('Origin',(188.388527625422,618.210565160534,-30.2221601717601)) ;
#65965=CARTESIAN_POINT('',(188.388527625422,618.710565160534,-30.2221601717601)) ;
#65966=CARTESIAN_POINT('',(188.388527625422,616.210565160534,-37.2221601717601)) ;
#65967=CARTESIAN_POINT('Origin',(188.388527625422,618.210565160534,-37.2221601717601)) ;
#65968=CARTESIAN_POINT('',(186.388527625422,616.210565160535,-37.22216017176)) ;
#65969=CARTESIAN_POINT('Origin',(186.388527625422,618.210565160535,-37.22216017176)) ;
#65970=CARTESIAN_POINT('',(186.388527625422,616.210565160535,-30.22216017176)) ;
#65971=CARTESIAN_POINT('Origin',(186.388527625422,618.210565160535,-30.22216017176)) ;
#65972=CARTESIAN_POINT('Origin',(173.388527625422,618.210565160537,-30.2221601717594)) ;
#65973=CARTESIAN_POINT('',(173.388527625422,618.710565160537,-30.2221601717594)) ;
#65974=CARTESIAN_POINT('',(173.388527625422,616.210565160537,-37.2221601717594)) ;
#65975=CARTESIAN_POINT('Origin',(173.388527625422,618.210565160537,-37.2221601717594)) ;
#65976=CARTESIAN_POINT('',(171.388527625422,616.210565160537,-37.2221601717593)) ;
#65977=CARTESIAN_POINT('Origin',(171.388527625422,618.210565160537,-37.2221601717593)) ;
#65978=CARTESIAN_POINT('',(171.388527625422,616.210565160537,-30.2221601717593)) ;
#65979=CARTESIAN_POINT('Origin',(171.388527625422,618.210565160537,-30.2221601717593)) ;
#65980=CARTESIAN_POINT('Origin',(38.3885276254222,618.210565160561,-30.2221601717533)) ;
#65981=CARTESIAN_POINT('',(38.3885276254223,618.710565160561,-30.2221601717533)) ;
#65982=CARTESIAN_POINT('',(38.3885276254215,616.210565160561,-37.2221601717533)) ;
#65983=CARTESIAN_POINT('Origin',(38.3885276254219,618.210565160561,-37.2221601717533)) ;
#65984=CARTESIAN_POINT('',(36.3885276254215,616.210565160561,-37.2221601717532)) ;
#65985=CARTESIAN_POINT('Origin',(36.3885276254219,618.210565160561,-37.2221601717532)) ;
#65986=CARTESIAN_POINT('',(36.3885276254219,616.210565160561,-30.2221601717532)) ;
#65987=CARTESIAN_POINT('Origin',(36.3885276254222,618.210565160561,-30.2221601717532)) ;
#65988=CARTESIAN_POINT('Origin',(97.6885276254225,618.21056516055,-24.122160171756)) ;
#65989=CARTESIAN_POINT('Origin',(94.438527625422,615.460565160551,-24.1221601717558)) ;
#65990=CARTESIAN_POINT('Origin',(21.3885276254219,618.210565160564,-37.2221601717525)) ;
#65991=CARTESIAN_POINT('',(21.3885276254215,616.210565160564,-37.2221601717525)) ;
#65992=CARTESIAN_POINT('',(21.3885276254219,616.210565160564,-30.2221601717525)) ;
#65993=CARTESIAN_POINT('Origin',(21.3885276254222,618.210565160564,-30.2221601717525)) ;
#65994=CARTESIAN_POINT('',(23.3885276254223,618.710565160563,-30.2221601717526)) ;
#65995=CARTESIAN_POINT('Origin',(23.3885276254222,618.210565160563,-30.2221601717526)) ;
#65996=CARTESIAN_POINT('',(23.3885276254215,616.210565160563,-37.2221601717526)) ;
#65997=CARTESIAN_POINT('Origin',(23.3885276254219,618.210565160563,-37.2221601717526)) ;
#65998=CARTESIAN_POINT('Origin',(148.388527625421,618.210565160541,-49.5221601717583)) ;
#65999=CARTESIAN_POINT('',(148.38852762542,612.710565160541,-47.5221601717583)) ;
#66000=CARTESIAN_POINT('',(148.388527625421,616.710565160541,-49.5221601717583)) ;
#66001=CARTESIAN_POINT('',(148.388527625421,616.710565160541,-49.5221601717583)) ;
#66002=CARTESIAN_POINT('Origin',(148.388527625421,616.710565160541,-47.5221601717583)) ;
#66003=CARTESIAN_POINT('Origin',(201.668527625411,561.210565160532,-49.5221601717607)) ;
#66004=CARTESIAN_POINT('',(201.668527625421,615.210565160532,-47.5221601717607)) ;
#66005=CARTESIAN_POINT('',(201.668527625421,616.710565160532,-49.5221601717607)) ;
#66006=CARTESIAN_POINT('',(201.668527625421,616.710565160532,-49.5221601717607)) ;
#66007=CARTESIAN_POINT('Origin',(201.668527625421,616.710565160532,-47.5221601717607)) ;
#66008=CARTESIAN_POINT('Origin',(493.123247625421,616.710565160481,-47.522160171774)) ;
#66009=CARTESIAN_POINT('',(197.688527625421,616.710565160533,-49.5221601717605)) ;
#66010=CARTESIAN_POINT('Origin',(197.688527625421,616.710565160533,-47.5221601717605)) ;
#66011=CARTESIAN_POINT('',(201.668527625421,616.710565160532,-49.5221601717607)) ;
#66012=CARTESIAN_POINT('Origin',(-283.146192374579,616.710565160617,-47.5221601717387)) ;
#66013=CARTESIAN_POINT('',(144.388527625421,616.710565160542,-49.5221601717581)) ;
#66014=CARTESIAN_POINT('',(144.388527625421,616.710565160542,-49.5221601717581)) ;
#66015=CARTESIAN_POINT('Origin',(144.388527625421,616.710565160542,-47.5221601717581)) ;
#66016=CARTESIAN_POINT('Origin',(193.688527625411,561.210565160533,-49.5221601717604)) ;
#66017=CARTESIAN_POINT('',(193.68852762542,612.880565160533,-47.5221601717603)) ;
#66018=CARTESIAN_POINT('',(193.688527625421,616.710565160533,-49.5221601717603)) ;
#66019=CARTESIAN_POINT('',(193.688527625421,616.710565160533,-49.5221601717603)) ;
#66020=CARTESIAN_POINT('Origin',(193.688527625421,616.710565160533,-47.5221601717604)) ;
#66021=CARTESIAN_POINT('Origin',(-283.146192374579,616.710565160617,-47.5221601717387)) ;
#66022=CARTESIAN_POINT('',(152.388527625421,616.710565160541,-49.5221601717585)) ;
#66023=CARTESIAN_POINT('',(152.388527625421,616.710565160541,-49.5221601717585)) ;
#66024=CARTESIAN_POINT('Origin',(152.388527625421,616.710565160541,-47.5221601717585)) ;
#66025=CARTESIAN_POINT('Origin',(99.1443220427211,615.46056516055,-43.3721601717561)) ;
#66026=CARTESIAN_POINT('',(99.6885276246509,615.46056516055,-40.1221601717561)) ;
#66027=CARTESIAN_POINT('Origin',(99.6885276254211,615.46056516055,-43.3721601717561)) ;
#66028=CARTESIAN_POINT('',(99.6885276245213,615.46056516055,-40.1221601717561)) ;
#66029=CARTESIAN_POINT('Origin',(99.6885276254213,615.46056516055,-38.1221601717561)) ;
#66030=CARTESIAN_POINT('',(97.6885276254214,615.46056516055,-38.122160171756)) ;
#66031=CARTESIAN_POINT('Origin',(94.4385276254214,615.460565160551,-38.1221601717558)) ;
#66032=CARTESIAN_POINT('Origin',(99.6885276254213,615.46056516055,-38.1221601717561)) ;
#66033=CARTESIAN_POINT('Origin',(94.438527625424,615.460565160551,19.9106552778142)) ;
#66034=CARTESIAN_POINT('',(97.6885276254219,615.46056516055,-25.772160171756)) ;
#66035=CARTESIAN_POINT('Origin',(197.688527625411,561.210565160533,-49.5221601717606)) ;
#66036=CARTESIAN_POINT('',(197.68852762542,612.880565160533,-47.5221601717605)) ;
#66037=CARTESIAN_POINT('',(197.68852762542,612.880565160533,-49.5221601717605)) ;
#66038=CARTESIAN_POINT('Origin',(205.668527625411,561.210565160531,-49.5221601717609)) ;
#66039=CARTESIAN_POINT('',(205.66852762542,612.880565160531,-47.5221601717609)) ;
#66040=CARTESIAN_POINT('',(205.66852762542,612.880565160531,-49.5221601717609)) ;
#66041=CARTESIAN_POINT('Origin',(152.388527625422,618.210565160541,-26.5221601717585)) ;
#66042=CARTESIAN_POINT('',(152.38852762542,612.710565160541,-49.5221601717584)) ;
#66043=CARTESIAN_POINT('',(152.388527625421,615.210565160541,-47.5221601717585)) ;
#66044=CARTESIAN_POINT('Origin',(144.388527625422,618.210565160542,-26.5221601717581)) ;
#66045=CARTESIAN_POINT('',(144.38852762542,612.710565160542,-49.5221601717581)) ;
#66046=CARTESIAN_POINT('',(144.388527625421,615.210565160542,-47.5221601717581)) ;
#66047=CARTESIAN_POINT('Origin',(212.388527625402,506.96056516053,-49.5221601717612)) ;
#66048=CARTESIAN_POINT('',(171.388527625403,506.960565160537,-25.7721601717594)) ;
#66049=CARTESIAN_POINT('',(171.388527625403,506.960565160537,-30.2221601717593)) ;
#66050=CARTESIAN_POINT('',(171.388527625403,506.960565160537,-25.7721601717594)) ;
#66051=CARTESIAN_POINT('',(156.063527625403,506.96056516054,-25.7721601717587)) ;
#66052=CARTESIAN_POINT('',(173.388527625403,506.960565160537,-24.1221601717594)) ;
#66053=CARTESIAN_POINT('',(173.388527625401,506.960565160537,-55.8221601717594)) ;
#66054=CARTESIAN_POINT('',(85.9885276254029,506.960565160552,-24.1221601717555)) ;
#66055=CARTESIAN_POINT('',(173.388527625403,506.960565160537,-24.1221601717594)) ;
#66056=CARTESIAN_POINT('',(85.9885276254019,506.960565160552,-46.8221601717555)) ;
#66057=CARTESIAN_POINT('',(87.9885276254028,506.960565160552,-25.7721601717556)) ;
#66058=CARTESIAN_POINT('',(156.063527625403,506.96056516054,-25.7721601717587)) ;
#66059=CARTESIAN_POINT('',(87.9885276254023,506.960565160552,-38.1221601717556)) ;
#66060=CARTESIAN_POINT('',(87.9885276254023,506.960565160552,-38.1221601726056)) ;
#66061=CARTESIAN_POINT('',(89.9885276254022,506.960565160551,-40.1221601717556)) ;
#66062=CARTESIAN_POINT('Origin',(89.9885276254023,506.960565160551,-38.1221601717556)) ;
#66063=CARTESIAN_POINT('',(169.388527626173,506.960565160538,-40.1221601717593)) ;
#66064=CARTESIAN_POINT('',(169.388527626302,506.960565160538,-40.1221601717592)) ;
#66065=CARTESIAN_POINT('',(171.388527625402,506.960565160537,-38.1221601717593)) ;
#66066=CARTESIAN_POINT('Origin',(169.388527625402,506.960565160538,-38.1221601717593)) ;
#66067=CARTESIAN_POINT('',(171.388527625402,506.960565160537,-37.2221601717593)) ;
#66068=CARTESIAN_POINT('',(171.388527625402,506.960565160537,-37.2221601717593)) ;
#66069=CARTESIAN_POINT('',(171.388527625402,506.960565160537,-37.2221601717593)) ;
#66070=CARTESIAN_POINT('',(102.988527625403,506.960565160549,-26.7721601717562)) ;
#66071=CARTESIAN_POINT('Origin',(102.988527625403,506.960565160549,-29.5221601717562)) ;
#66072=CARTESIAN_POINT('',(119.388527625403,506.960565160546,-26.772160171757)) ;
#66073=CARTESIAN_POINT('Origin',(119.388527625403,506.960565160546,-29.522160171757)) ;
#66074=CARTESIAN_POINT('',(137.988527625403,506.960565160543,-26.7721601717578)) ;
#66075=CARTESIAN_POINT('Origin',(137.988527625403,506.960565160543,-29.5221601717578)) ;
#66076=CARTESIAN_POINT('',(156.988527625403,506.96056516054,-26.7721601717587)) ;
#66077=CARTESIAN_POINT('Origin',(156.988527625403,506.96056516054,-29.5221601717587)) ;
#66078=CARTESIAN_POINT('Origin',(173.388527625402,504.210565160537,-24.1221601717594)) ;
#66079=CARTESIAN_POINT('',(171.388527625403,508.960565160537,-24.1221601717594)) ;
#66080=CARTESIAN_POINT('Origin',(171.388527625403,506.960565160537,-24.1221601717593)) ;
#66081=CARTESIAN_POINT('',(87.9885276254033,508.960565160552,-24.1221601717556)) ;
#66082=CARTESIAN_POINT('',(192.888527625403,508.960565160534,-24.1221601717603)) ;
#66083=CARTESIAN_POINT('Origin',(87.9885276254029,506.960565160552,-24.1221601717556)) ;
#66084=CARTESIAN_POINT('Origin',(156.988527625403,507.46056516054,-29.5221601717587)) ;
#66085=CARTESIAN_POINT('',(155.238527625403,508.96056516054,-29.5221601717586)) ;
#66086=CARTESIAN_POINT('Origin',(156.988527625403,508.96056516054,-29.5221601717587)) ;
#66087=CARTESIAN_POINT('',(155.238527625403,507.96056516054,-29.5221601717586)) ;
#66088=CARTESIAN_POINT('',(155.238527625403,507.46056516054,-29.5221601717586)) ;
#66089=CARTESIAN_POINT('',(156.988527625403,507.96056516054,-27.7721601717587)) ;
#66090=CARTESIAN_POINT('Origin',(156.988527625403,507.96056516054,-29.5221601717587)) ;
#66091=CARTESIAN_POINT('Origin',(156.988527625403,507.96056516054,-29.5221601717587)) ;
#66092=CARTESIAN_POINT('Origin',(156.988527625403,507.46056516054,-29.5221601717587)) ;
#66093=CARTESIAN_POINT('',(156.988527625403,507.46056516054,-27.2721601717587)) ;
#66094=CARTESIAN_POINT('Origin',(137.988527625403,507.460565160543,-29.5221601717578)) ;
#66095=CARTESIAN_POINT('',(136.238527625403,508.960565160543,-29.5221601717578)) ;
#66096=CARTESIAN_POINT('Origin',(137.988527625403,508.960565160543,-29.5221601717578)) ;
#66097=CARTESIAN_POINT('',(136.238527625403,507.960565160543,-29.5221601717577)) ;
#66098=CARTESIAN_POINT('',(136.238527625403,507.460565160543,-29.5221601717577)) ;
#66099=CARTESIAN_POINT('',(137.988527625403,507.960565160543,-27.7721601717579)) ;
#66100=CARTESIAN_POINT('Origin',(137.988527625403,507.960565160543,-29.5221601717578)) ;
#66101=CARTESIAN_POINT('Origin',(137.988527625403,507.960565160543,-29.5221601717578)) ;
#66102=CARTESIAN_POINT('Origin',(137.988527625403,507.460565160543,-29.5221601717578)) ;
#66103=CARTESIAN_POINT('',(137.988527625403,507.460565160543,-27.2721601717578)) ;
#66104=CARTESIAN_POINT('Origin',(119.388527625403,507.460565160546,-29.522160171757)) ;
#66105=CARTESIAN_POINT('',(117.638527625403,508.960565160547,-29.5221601717569)) ;
#66106=CARTESIAN_POINT('Origin',(119.388527625403,508.960565160546,-29.522160171757)) ;
#66107=CARTESIAN_POINT('',(117.638527625403,507.960565160546,-29.5221601717569)) ;
#66108=CARTESIAN_POINT('',(117.638527625403,507.460565160546,-29.5221601717569)) ;
#66109=CARTESIAN_POINT('',(119.388527625403,507.960565160546,-27.772160171757)) ;
#66110=CARTESIAN_POINT('Origin',(119.388527625403,507.960565160546,-29.522160171757)) ;
#66111=CARTESIAN_POINT('Origin',(119.388527625403,507.960565160546,-29.522160171757)) ;
#66112=CARTESIAN_POINT('Origin',(119.388527625403,507.460565160546,-29.522160171757)) ;
#66113=CARTESIAN_POINT('',(119.388527625403,507.460565160546,-27.272160171757)) ;
#66114=CARTESIAN_POINT('Origin',(102.988527625403,507.460565160549,-29.5221601717562)) ;
#66115=CARTESIAN_POINT('',(101.238527625403,508.96056516055,-29.5221601717562)) ;
#66116=CARTESIAN_POINT('Origin',(102.988527625403,508.960565160549,-29.5221601717562)) ;
#66117=CARTESIAN_POINT('',(101.238527625403,507.960565160549,-29.5221601717561)) ;
#66118=CARTESIAN_POINT('',(101.238527625403,507.460565160549,-29.5221601717561)) ;
#66119=CARTESIAN_POINT('',(102.988527625403,507.960565160549,-27.7721601717563)) ;
#66120=CARTESIAN_POINT('Origin',(102.988527625403,507.960565160549,-29.5221601717563)) ;
#66121=CARTESIAN_POINT('Origin',(102.988527625403,507.960565160549,-29.5221601717563)) ;
#66122=CARTESIAN_POINT('Origin',(102.988527625403,507.460565160549,-29.5221601717562)) ;
#66123=CARTESIAN_POINT('',(102.988527625403,507.460565160549,-27.2721601717562)) ;
#66124=CARTESIAN_POINT('Origin',(171.388527625422,618.210565160537,-37.2221601717593)) ;
#66125=CARTESIAN_POINT('',(171.388527625403,508.960565160537,-37.2221601717594)) ;
#66126=CARTESIAN_POINT('',(171.388527625403,508.960565160537,-30.2221601717593)) ;
#66127=CARTESIAN_POINT('',(171.388527625402,508.960565160537,-43.3721601717594)) ;
#66128=CARTESIAN_POINT('',(171.388527625403,506.960565160537,-30.2221601717593)) ;
#66129=CARTESIAN_POINT('',(171.388527625403,509.460565160537,-37.2221601717594)) ;
#66130=CARTESIAN_POINT('Origin',(99.7385276254032,506.585565284346,-25.7721601717561)) ;
#66131=CARTESIAN_POINT('Origin',(174.638527625403,506.960565160537,-25.7721601717595)) ;
#66132=CARTESIAN_POINT('Origin',(99.7385276254032,506.585565284346,-25.7721601717561)) ;
#66133=CARTESIAN_POINT('Origin',(84.7385276254028,506.960565160553,-25.7721601717554)) ;
#66134=CARTESIAN_POINT('Origin',(201.668527625411,561.210565160532,-49.5221601717607)) ;
#66135=CARTESIAN_POINT('',(201.668527625402,503.710565160532,-28.5221601717607)) ;
#66136=CARTESIAN_POINT('',(201.668527625402,505.710565160532,-49.5221601717607)) ;
#66137=CARTESIAN_POINT('Origin',(201.668527625402,505.710565160532,-47.5221601717607)) ;
#66138=CARTESIAN_POINT('',(201.668527625402,509.540565160532,-49.5221601717607)) ;
#66139=CARTESIAN_POINT('',(201.668527625402,507.210565160532,-47.5221601717607)) ;
#66140=CARTESIAN_POINT('Origin',(205.668527625411,561.210565160531,-49.5221601717609)) ;
#66141=CARTESIAN_POINT('',(205.668527625402,509.540565160531,-47.5221601717609)) ;
#66142=CARTESIAN_POINT('',(205.668527625402,505.710565160531,-49.5221601717609)) ;
#66143=CARTESIAN_POINT('',(205.668527625403,506.210565160531,-28.5221601717609)) ;
#66144=CARTESIAN_POINT('Origin',(21.3885276254222,618.210565160564,-30.2221601717525)) ;
#66145=CARTESIAN_POINT('',(23.3885276254025,506.210565160563,-30.2221601717526)) ;
#66146=CARTESIAN_POINT('',(21.3885276254025,506.210565160564,-30.2221601717525)) ;
#66147=CARTESIAN_POINT('Origin',(23.3885276254222,618.210565160563,-30.2221601717526)) ;
#66148=CARTESIAN_POINT('',(23.3885276254017,503.710565160563,-37.2221601717526)) ;
#66149=CARTESIAN_POINT('Origin',(23.3885276254219,618.210565160563,-37.2221601717526)) ;
#66150=CARTESIAN_POINT('',(21.3885276254022,506.210565160564,-37.2221601717525)) ;
#66151=CARTESIAN_POINT('Origin',(21.3885276254219,618.210565160564,-37.2221601717525)) ;
#66152=CARTESIAN_POINT('Origin',(173.388527625422,618.210565160537,-30.2221601717594)) ;
#66153=CARTESIAN_POINT('',(173.388527625402,503.960565160537,-37.2221601717594)) ;
#66154=CARTESIAN_POINT('',(173.388527625402,506.210565160537,-37.2221601717594)) ;
#66155=CARTESIAN_POINT('',(173.388527625402,503.960565160537,-30.2221601717594)) ;
#66156=CARTESIAN_POINT('',(173.388527625402,503.960565160537,-30.2221601717594)) ;
#66157=CARTESIAN_POINT('',(173.388527625403,506.210565160537,-30.2221601717594)) ;
#66158=CARTESIAN_POINT('Origin',(195.688527625376,354.701436995033,-28.5221601717605)) ;
#66159=CARTESIAN_POINT('',(197.688527625403,506.210565160533,-28.5221601717605)) ;
#66160=CARTESIAN_POINT('',(193.688527625402,503.710565160533,-28.5221601717604)) ;
#66161=CARTESIAN_POINT('Origin',(203.668527625376,354.701436995032,-28.5221601717608)) ;
#66162=CARTESIAN_POINT('Origin',(-2.61147237459681,507.212565160568,-19.5221601717514)) ;
#66163=CARTESIAN_POINT('Origin',(171.388527625402,504.210565160537,-24.1221601717594)) ;
#66164=CARTESIAN_POINT('Origin',(174.638527625403,506.960565160537,-24.1221601717595)) ;
#66165=CARTESIAN_POINT('Origin',(84.7385276254029,506.960565160552,-24.1221601717554)) ;
#66166=CARTESIAN_POINT('Origin',(38.3885276254219,618.210565160561,-37.2221601717533)) ;
#66167=CARTESIAN_POINT('',(36.3885276254022,506.210565160561,-37.2221601717532)) ;
#66168=CARTESIAN_POINT('',(38.3885276254017,503.710565160561,-37.2221601717533)) ;
#66169=CARTESIAN_POINT('Origin',(36.3885276254219,618.210565160561,-37.2221601717532)) ;
#66170=CARTESIAN_POINT('',(36.3885276254025,506.210565160561,-30.2221601717532)) ;
#66171=CARTESIAN_POINT('Origin',(36.3885276254222,618.210565160561,-30.2221601717532)) ;
#66172=CARTESIAN_POINT('',(38.3885276254025,506.210565160561,-30.2221601717533)) ;
#66173=CARTESIAN_POINT('Origin',(38.3885276254222,618.210565160561,-30.2221601717533)) ;
#66174=CARTESIAN_POINT('Origin',(188.388527625422,618.210565160534,-37.2221601717601)) ;
#66175=CARTESIAN_POINT('',(186.388527625402,506.210565160535,-37.22216017176)) ;
#66176=CARTESIAN_POINT('',(188.388527625402,503.710565160534,-37.2221601717601)) ;
#66177=CARTESIAN_POINT('Origin',(186.388527625422,618.210565160535,-37.22216017176)) ;
#66178=CARTESIAN_POINT('',(186.388527625403,506.210565160535,-30.22216017176)) ;
#66179=CARTESIAN_POINT('Origin',(186.388527625422,618.210565160535,-30.22216017176)) ;
#66180=CARTESIAN_POINT('',(188.388527625403,506.210565160534,-30.2221601717601)) ;
#66181=CARTESIAN_POINT('Origin',(188.388527625422,618.210565160534,-30.2221601717601)) ;
#66182=CARTESIAN_POINT('Origin',(169.388527625402,506.960565160538,-38.1221601717593)) ;
#66183=CARTESIAN_POINT('Origin',(169.388527625402,506.960565160538,-43.3721601717593)) ;
#66184=CARTESIAN_POINT('Origin',(174.638527625402,506.960565160537,-38.1221601717595)) ;
#66185=CARTESIAN_POINT('Origin',(169.932733208102,506.960565160537,-43.3721601717593)) ;
#66186=CARTESIAN_POINT('Origin',(89.988527625402,506.960565160551,-43.3721601717557)) ;
#66187=CARTESIAN_POINT('Origin',(89.9885276254023,506.960565160551,-38.1221601717556)) ;
#66188=CARTESIAN_POINT('Origin',(84.7385276254023,506.960565160553,-38.1221601717554)) ;
#66189=CARTESIAN_POINT('Origin',(-283.146192374598,505.710565160617,-47.5221601717387)) ;
#66190=CARTESIAN_POINT('',(193.688527625402,505.710565160533,-49.5221601717604)) ;
#66191=CARTESIAN_POINT('',(-0.611472374598421,505.710565160567,-49.5221601717515)) ;
#66192=CARTESIAN_POINT('Origin',(193.688527625402,505.710565160533,-47.5221601717604)) ;
#66193=CARTESIAN_POINT('Origin',(193.688527625411,561.210565160533,-49.5221601717604)) ;
#66194=CARTESIAN_POINT('',(193.688527625402,509.540565160533,-49.5221601717604)) ;
#66195=CARTESIAN_POINT('',(193.688527625402,507.210565160533,-47.5221601717604)) ;
#66196=CARTESIAN_POINT('Origin',(493.123247625402,505.710565160481,-47.522160171774)) ;
#66197=CARTESIAN_POINT('',(197.688527625402,505.710565160533,-49.5221601717605)) ;
#66198=CARTESIAN_POINT('Origin',(197.688527625402,505.710565160533,-47.5221601717605)) ;
#66199=CARTESIAN_POINT('',(201.668527625402,505.710565160532,-49.5221601717607)) ;
#66200=CARTESIAN_POINT('Origin',(197.688527625411,561.210565160533,-49.5221601717606)) ;
#66201=CARTESIAN_POINT('',(197.688527625402,509.540565160533,-47.5221601717606)) ;
#66202=CARTESIAN_POINT('',(197.688527625402,505.710565160533,-49.5221601717605)) ;
#66203=CARTESIAN_POINT('Origin',(174.638527625405,506.960565160537,19.9106552778105)) ;
#66204=CARTESIAN_POINT('Origin',(174.638527625403,506.960565160537,-30.2221601717595)) ;
#66205=CARTESIAN_POINT('Origin',(174.638527625402,506.960565160537,-37.2221601717595)) ;
#66206=CARTESIAN_POINT('Origin',(84.7385276254022,506.960565160553,-38.6663657544454)) ;
#66207=CARTESIAN_POINT('Origin',(99.738527625422,615.46056516055,-22.6221601717603)) ;
#66208=CARTESIAN_POINT('',(95.688527625422,615.460565160551,-24.1221601717559)) ;
#66209=CARTESIAN_POINT('',(126.688527625422,615.460565160545,-24.1221601717573)) ;
#66210=CARTESIAN_POINT('',(95.688527625422,615.460565160551,-24.1221601717559)) ;
#66211=CARTESIAN_POINT('',(126.688527625422,615.460565160545,-24.1221601717573)) ;
#66212=CARTESIAN_POINT('',(95.688527625422,615.460565160551,-24.1221601717559)) ;
#66213=CARTESIAN_POINT('Origin',(6.48852762540226,504.210565160566,-24.0221601717538)) ;
#66214=CARTESIAN_POINT('',(4.83852769761494,617.610303266554,-24.0221601717537)) ;
#66215=CARTESIAN_POINT('',(6.48225865783948,617.612395100656,-25.6721482626337)) ;
#66216=CARTESIAN_POINT('Origin',(6.48852838553329,617.610565789223,-24.022160479896)) ;
#66217=CARTESIAN_POINT('',(4.83852762540226,504.210565160566,-24.0221601717537)) ;
#66218=CARTESIAN_POINT('Origin',(6.48852838553329,617.610565789223,-24.022160479896)) ;
#66219=CARTESIAN_POINT('Origin',(6.48826460342246,618.160565160566,-24.0203292411918)) ;
#66220=CARTESIAN_POINT('',(6.48026554736851,618.160565160566,-26.2203146991215)) ;
#66221=CARTESIAN_POINT('Ctrl Pts',(27.8977259437596,618.707397415445,-37.5528630721564)) ;
#66222=CARTESIAN_POINT('Ctrl Pts',(28.0743877192963,618.67030643865,-38.2156681467201)) ;
#66223=CARTESIAN_POINT('Ctrl Pts',(29.1421966155256,618.596141379903,-39.3386387111389)) ;
#66224=CARTESIAN_POINT('Ctrl Pts',(31.4346649598415,618.484902239203,-38.9068600918672)) ;
#66225=CARTESIAN_POINT('Ctrl Pts',(32.3091095046996,618.373679993346,-36.7435823810485)) ;
#66226=CARTESIAN_POINT('Ctrl Pts',(30.966253505222,618.262457747489,-34.8371854931543)) ;
#66227=CARTESIAN_POINT('Ctrl Pts',(28.6354820240381,618.151235501631,-34.9326680111136)) ;
#66228=CARTESIAN_POINT('Ctrl Pts',(27.4535163667976,618.040013255774,-36.9436582668131)) ;
#66229=CARTESIAN_POINT('Ctrl Pts',(28.5034276654628,617.928791009917,-39.0264313282299)) ;
#66230=CARTESIAN_POINT('Ctrl Pts',(30.8229580687087,617.817568764059,-39.2721846815949)) ;
#66231=CARTESIAN_POINT('Ctrl Pts',(32.2860034094053,617.706346518201,-37.4555666679615)) ;
#66232=CARTESIAN_POINT('Ctrl Pts',(31.5515705394677,617.595124272344,-35.2417057246827)) ;
#66233=CARTESIAN_POINT('Ctrl Pts',(29.2928260283501,617.483902026487,-34.659773469075)) ;
#66234=CARTESIAN_POINT('Ctrl Pts',(27.5800809010859,617.37267978063,-36.2431580734666)) ;
#66235=CARTESIAN_POINT('Ctrl Pts',(27.9832559996343,617.261457534773,-38.5405622264581)) ;
#66236=CARTESIAN_POINT('Ctrl Pts',(30.132705572695,617.150235288915,-39.446169146318)) ;
#66237=CARTESIAN_POINT('Ctrl Pts',(32.0585169830119,617.039013043057,-38.1299719592266)) ;
#66238=CARTESIAN_POINT('Ctrl Pts',(31.9950195758766,616.9277907972,-35.7981098946905)) ;
#66239=CARTESIAN_POINT('Ctrl Pts',(30.0015829148602,616.816568551343,-34.5882249381669)) ;
#66240=CARTESIAN_POINT('Ctrl Pts',(27.9028912368749,616.705346305486,-35.6079881248491)) ;
#66241=CARTESIAN_POINT('Ctrl Pts',(27.6282710239295,616.594109768654,-37.9244882573162)) ;
#66242=CARTESIAN_POINT('Ctrl Pts',(28.8212760718149,616.519947313775,-38.9133119870574)) ;
#66243=CARTESIAN_POINT('Ctrl Pts',(29.4945169267138,616.482858940849,-39.0444589860994)) ;
#66244=CARTESIAN_POINT('Ctrl Pts',(28.0258055392794,618.783926575113,-37.5187199360264)) ;
#66245=CARTESIAN_POINT('Ctrl Pts',(28.191101657974,618.746835598319,-38.1388829902218)) ;
#66246=CARTESIAN_POINT('Ctrl Pts',(29.1902123343951,618.672670539572,-39.1896064709675)) ;
#66247=CARTESIAN_POINT('Ctrl Pts',(31.3351931509543,618.561431398871,-38.7856066261564)) ;
#66248=CARTESIAN_POINT('Ctrl Pts',(32.1533797045511,618.450209153014,-36.7615048748273)) ;
#66249=CARTESIAN_POINT('Ctrl Pts',(30.8969172694545,618.338986907157,-34.9777573419897)) ;
#66250=CARTESIAN_POINT('Ctrl Pts',(28.7160975746836,618.2277646613,-35.0670969264808)) ;
#66251=CARTESIAN_POINT('Ctrl Pts',(27.6101744909914,618.116542415443,-36.9487087408633)) ;
#66252=CARTESIAN_POINT('Ctrl Pts',(28.5925390240981,618.005320169585,-38.897485164783)) ;
#66253=CARTESIAN_POINT('Ctrl Pts',(30.7628408434119,617.894097923727,-39.1274278071231)) ;
#66254=CARTESIAN_POINT('Ctrl Pts',(32.1317601557906,617.782875677869,-37.4276831629185)) ;
#66255=CARTESIAN_POINT('Ctrl Pts',(31.4445775297042,617.671653432013,-35.3562524861823)) ;
#66256=CARTESIAN_POINT('Ctrl Pts',(29.3311509003384,617.560431186156,-34.8117592425087)) ;
#66257=CARTESIAN_POINT('Ctrl Pts',(27.7285964089117,617.449208940298,-36.2932757092798)) ;
#66258=CARTESIAN_POINT('Ctrl Pts',(28.1058329601794,617.33798669444,-38.4428747858684)) ;
#66259=CARTESIAN_POINT('Ctrl Pts',(30.1169962165045,617.226764448583,-39.2902188616367)) ;
#66260=CARTESIAN_POINT('Ctrl Pts',(31.9189092251107,617.115542202726,-38.0587001258951)) ;
#66261=CARTESIAN_POINT('Ctrl Pts',(31.8594969673389,617.004319956867,-35.876860011202)) ;
#66262=CARTESIAN_POINT('Ctrl Pts',(29.9943094250516,616.893097711011,-34.7448138355498)) ;
#66263=CARTESIAN_POINT('Ctrl Pts',(28.0306385197095,616.781875465154,-35.6989698561946)) ;
#66264=CARTESIAN_POINT('Ctrl Pts',(27.7736861870555,616.670638928323,-37.8664363592844)) ;
#66265=CARTESIAN_POINT('Ctrl Pts',(28.8899384346023,616.596476473445,-38.7916434342315)) ;
#66266=CARTESIAN_POINT('Ctrl Pts',(29.5198658760269,616.559388100518,-38.9143530008837)) ;
#66267=CARTESIAN_POINT('Ctrl Pts',(28.1538851347994,618.860455734782,-37.4845767998963)) ;
#66268=CARTESIAN_POINT('Ctrl Pts',(28.3078155966519,618.823364757988,-38.0620978337234)) ;
#66269=CARTESIAN_POINT('Ctrl Pts',(29.2382280532645,618.749199699239,-39.0405742307961)) ;
#66270=CARTESIAN_POINT('Ctrl Pts',(31.2357213420671,618.637960558539,-38.6643531604454)) ;
#66271=CARTESIAN_POINT('Ctrl Pts',(31.9976499044024,618.526738312682,-36.779427368606)) ;
#66272=CARTESIAN_POINT('Ctrl Pts',(30.8275810336869,618.415516066825,-35.1183291908253)) ;
#66273=CARTESIAN_POINT('Ctrl Pts',(28.7967131253291,618.304293820967,-35.2015258418478)) ;
#66274=CARTESIAN_POINT('Ctrl Pts',(27.7668326151852,618.19307157511,-36.9537592149134)) ;
#66275=CARTESIAN_POINT('Ctrl Pts',(28.6816503827333,618.081849329253,-38.7685390013363)) ;
#66276=CARTESIAN_POINT('Ctrl Pts',(30.7027236181152,617.970627083395,-38.9826709326515)) ;
#66277=CARTESIAN_POINT('Ctrl Pts',(31.9775169021757,617.859404837538,-37.3997996578756)) ;
#66278=CARTESIAN_POINT('Ctrl Pts',(31.3375845199407,617.74818259168,-35.4707992476819)) ;
#66279=CARTESIAN_POINT('Ctrl Pts',(29.3694757723265,617.636960345823,-34.9637450159425)) ;
#66280=CARTESIAN_POINT('Ctrl Pts',(27.8771119167374,617.525738099966,-36.3433933450928)) ;
#66281=CARTESIAN_POINT('Ctrl Pts',(28.2284099207247,617.414515854109,-38.3451873452787)) ;
#66282=CARTESIAN_POINT('Ctrl Pts',(30.1012868603142,617.303293608251,-39.1342685769555)) ;
#66283=CARTESIAN_POINT('Ctrl Pts',(31.7793014672095,617.192071362394,-37.9874282925633)) ;
#66284=CARTESIAN_POINT('Ctrl Pts',(31.7239743588012,617.080849116536,-35.9556101277135)) ;
#66285=CARTESIAN_POINT('Ctrl Pts',(29.987035935243,616.969626870679,-34.9014027329326)) ;
#66286=CARTESIAN_POINT('Ctrl Pts',(28.158385802544,616.858404624822,-35.78995158754)) ;
#66287=CARTESIAN_POINT('Ctrl Pts',(27.9191013501814,616.747168087991,-37.8083844612528)) ;
#66288=CARTESIAN_POINT('Ctrl Pts',(28.9586007973896,616.673005633112,-38.6699748814058)) ;
#66289=CARTESIAN_POINT('Ctrl Pts',(29.5452148253402,616.635917260186,-38.7842470156678)) ;
#66290=CARTESIAN_POINT('Ctrl Pts',(28.2819647303194,618.93698489445,-37.4504336637662)) ;
#66291=CARTESIAN_POINT('Ctrl Pts',(28.4245295353296,618.899893917656,-37.9853126772251)) ;
#66292=CARTESIAN_POINT('Ctrl Pts',(29.286243772134,618.825728858908,-38.8915419906246)) ;
#66293=CARTESIAN_POINT('Ctrl Pts',(31.1362495331798,618.714489718209,-38.5430996947345)) ;
#66294=CARTESIAN_POINT('Ctrl Pts',(31.8419201042538,618.603267472351,-36.7973498623847)) ;
#66295=CARTESIAN_POINT('Ctrl Pts',(30.7582447979194,618.492045226494,-35.2589010396609)) ;
#66296=CARTESIAN_POINT('Ctrl Pts',(28.8773286759747,618.380822980637,-35.3359547572148)) ;
#66297=CARTESIAN_POINT('Ctrl Pts',(27.9234907393791,618.26960073478,-36.9588096889635)) ;
#66298=CARTESIAN_POINT('Ctrl Pts',(28.7707617413686,618.158378488922,-38.6395928378894)) ;
#66299=CARTESIAN_POINT('Ctrl Pts',(30.6426063928184,618.047156243065,-38.8379140581797)) ;
#66300=CARTESIAN_POINT('Ctrl Pts',(31.8232736485609,617.935933997207,-37.3719161528327)) ;
#66301=CARTESIAN_POINT('Ctrl Pts',(31.2305915101772,617.82471175135,-35.5853460091816)) ;
#66302=CARTESIAN_POINT('Ctrl Pts',(29.4078006443147,617.713489505493,-35.1157307893762)) ;
#66303=CARTESIAN_POINT('Ctrl Pts',(28.0256274245631,617.602267259635,-36.393510980906)) ;
#66304=CARTESIAN_POINT('Ctrl Pts',(28.35098688127,617.491045013778,-38.247499904689)) ;
#66305=CARTESIAN_POINT('Ctrl Pts',(30.0855775041238,617.37982276792,-38.9783182922743)) ;
#66306=CARTESIAN_POINT('Ctrl Pts',(31.6396937093084,617.268600522063,-37.9161564592317)) ;
#66307=CARTESIAN_POINT('Ctrl Pts',(31.5884517502634,617.157378276205,-36.034360244225)) ;
#66308=CARTESIAN_POINT('Ctrl Pts',(29.9797624454342,617.046156030348,-35.0579916303155)) ;
#66309=CARTESIAN_POINT('Ctrl Pts',(28.2861330853785,616.934933784491,-35.8809333188854)) ;
#66310=CARTESIAN_POINT('Ctrl Pts',(28.0645165133074,616.82369724766,-37.7503325632211)) ;
#66311=CARTESIAN_POINT('Ctrl Pts',(29.027263160177,616.749534792781,-38.54830632858)) ;
#66312=CARTESIAN_POINT('Ctrl Pts',(29.5705637746533,616.712446419854,-38.6541410304521)) ;
#66313=CARTESIAN_POINT('Ctrl Pts',(30.966214425925,618.708683906554,-35.756042592416)) ;
#66314=CARTESIAN_POINT('Ctrl Pts',(30.5447271292425,618.671595533668,-35.3972599237611)) ;
#66315=CARTESIAN_POINT('Ctrl Pts',(29.3205834535133,618.597433078829,-35.1420827411956)) ;
#66316=CARTESIAN_POINT('Ctrl Pts',(27.9972039226441,618.486196542039,-36.4809009401573)) ;
#66317=CARTESIAN_POINT('Ctrl Pts',(28.4097628334874,618.374974296181,-38.3181294473258)) ;
#66318=CARTESIAN_POINT('Ctrl Pts',(30.176119912037,618.263752050324,-38.9670975304033)) ;
#66319=CARTESIAN_POINT('Ctrl Pts',(31.6793162682317,618.152529804466,-37.8338793668858)) ;
#66320=CARTESIAN_POINT('Ctrl Pts',(31.5407722192233,618.041307558609,-35.9565753284643)) ;
#66321=CARTESIAN_POINT('Ctrl Pts',(29.8878958341303,617.930085312751,-35.0560755863368)) ;
#66322=CARTESIAN_POINT('Ctrl Pts',(28.2355306242915,617.818863066894,-35.9576425061243)) ;
#66323=CARTESIAN_POINT('Ctrl Pts',(28.0982927495265,617.707640821037,-37.8349519584651)) ;
#66324=CARTESIAN_POINT('Ctrl Pts',(29.6019442250164,617.596418575179,-38.9672669406877)) ;
#66325=CARTESIAN_POINT('Ctrl Pts',(31.3682722736937,617.485196329322,-38.3167362318318)) ;
#66326=CARTESIAN_POINT('Ctrl Pts',(31.7783015947118,617.373974083464,-36.4796186607374)) ;
#66327=CARTESIAN_POINT('Ctrl Pts',(30.4561717720678,617.262751837607,-35.1398028414488)) ;
#66328=CARTESIAN_POINT('Ctrl Pts',(28.6138177650868,617.15152959175,-35.5253308468272)) ;
#66329=CARTESIAN_POINT('Ctrl Pts',(27.9397269121408,617.040307345893,-37.2829048646609)) ;
#66330=CARTESIAN_POINT('Ctrl Pts',(29.0522159057932,616.929085100035,-38.801506501169)) ;
#66331=CARTESIAN_POINT('Ctrl Pts',(30.930684117803,616.817862854177,-38.6895508033932)) ;
#66332=CARTESIAN_POINT('Ctrl Pts',(31.8555878909266,616.70664060832,-37.049378113421)) ;
#66333=CARTESIAN_POINT('Ctrl Pts',(30.9745593872839,616.595402487695,-35.3857503772719)) ;
#66334=CARTESIAN_POINT('Ctrl Pts',(29.7287969659281,616.521238449023,-35.2770475901246)) ;
#66335=CARTESIAN_POINT('Ctrl Pts',(29.2217315764459,616.484148492302,-35.4990562403977)) ;
#66336=CARTESIAN_POINT('Ctrl Pts',(31.0526478907908,618.785673866071,-35.6544964574366)) ;
#66337=CARTESIAN_POINT('Ctrl Pts',(30.59735614607,618.748585493184,-35.2669384255025)) ;
#66338=CARTESIAN_POINT('Ctrl Pts',(29.2750327586311,618.674423038346,-34.9912953264635)) ;
#66339=CARTESIAN_POINT('Ctrl Pts',(27.8455145257457,618.563186501555,-36.4374904513627)) ;
#66340=CARTESIAN_POINT('Ctrl Pts',(28.2911618033656,618.451964255698,-38.4220697709847)) ;
#66341=CARTESIAN_POINT('Ctrl Pts',(30.1991856095934,618.34074200984,-39.1230868909266)) ;
#66342=CARTESIAN_POINT('Ctrl Pts',(31.8229424749996,618.229519763982,-37.8989814934968)) ;
#66343=CARTESIAN_POINT('Ctrl Pts',(31.6732868097158,618.118297518125,-35.8711124740704)) ;
#66344=CARTESIAN_POINT('Ctrl Pts',(29.8878451627196,618.007075272268,-34.898390159683)) ;
#66345=CARTESIAN_POINT('Ctrl Pts',(28.1029556886482,617.895853026411,-35.872265242333)) ;
#66346=CARTESIAN_POINT('Ctrl Pts',(27.9547109563982,617.784630780554,-37.9001401098902)) ;
#66347=CARTESIAN_POINT('Ctrl Pts',(29.5789594429271,617.673408534696,-39.1232698883848)) ;
#66348=CARTESIAN_POINT('Ctrl Pts',(31.4869518910064,617.562186288838,-38.4205648157511)) ;
#66349=CARTESIAN_POINT('Ctrl Pts',(31.9298666986942,617.450964042981,-36.4361053295835)) ;
#66350=CARTESIAN_POINT('Ctrl Pts',(30.5016984040935,617.339741797123,-34.9888325724452)) ;
#66351=CARTESIAN_POINT('Ctrl Pts',(28.5115825053845,617.228519551267,-35.4052809911498)) ;
#66352=CARTESIAN_POINT('Ctrl Pts',(27.7834276998808,617.117297305409,-37.303817310877)) ;
#66353=CARTESIAN_POINT('Ctrl Pts',(28.9851413906358,617.006075059552,-38.9442150027259)) ;
#66354=CARTESIAN_POINT('Ctrl Pts',(31.0142679535953,616.894852813694,-38.8232801480506)) ;
#66355=CARTESIAN_POINT('Ctrl Pts',(32.0133515698245,616.783630567837,-37.0515610676928)) ;
#66356=CARTESIAN_POINT('Ctrl Pts',(31.0616621411529,616.672392447211,-35.2545057815218)) ;
#66357=CARTESIAN_POINT('Ctrl Pts',(29.7159861248389,616.59822840854,-35.1370847299129)) ;
#66358=CARTESIAN_POINT('Ctrl Pts',(29.1682526873617,616.561138451819,-35.376899088546)) ;
#66359=CARTESIAN_POINT('Ctrl Pts',(31.1390813556564,618.862663825587,-35.5529503224572)) ;
#66360=CARTESIAN_POINT('Ctrl Pts',(30.6499851628975,618.825575452702,-35.1366169272439)) ;
#66361=CARTESIAN_POINT('Ctrl Pts',(29.2294820637489,618.751412997863,-34.8405079117313)) ;
#66362=CARTESIAN_POINT('Ctrl Pts',(27.6938251288474,618.640176461073,-36.3940799625681)) ;
#66363=CARTESIAN_POINT('Ctrl Pts',(28.1725607732438,618.528954215214,-38.5260100946437)) ;
#66364=CARTESIAN_POINT('Ctrl Pts',(30.2222513071496,618.417731969357,-39.2790762514498)) ;
#66365=CARTESIAN_POINT('Ctrl Pts',(31.9665686817676,618.306509723498,-37.9640836201077)) ;
#66366=CARTESIAN_POINT('Ctrl Pts',(31.8058014002084,618.195287477643,-35.7856496196763)) ;
#66367=CARTESIAN_POINT('Ctrl Pts',(29.887794491309,618.084065231784,-34.7407047330292)) ;
#66368=CARTESIAN_POINT('Ctrl Pts',(27.970380753005,617.972842985929,-35.7868879785417)) ;
#66369=CARTESIAN_POINT('Ctrl Pts',(27.8111291632698,617.861620740071,-37.9653282613151)) ;
#66370=CARTESIAN_POINT('Ctrl Pts',(29.555974660838,617.750398494213,-39.2792728360818)) ;
#66371=CARTESIAN_POINT('Ctrl Pts',(31.6056315083191,617.639176248354,-38.5243933996705)) ;
#66372=CARTESIAN_POINT('Ctrl Pts',(32.0814318026768,617.527954002496,-36.3925919984296)) ;
#66373=CARTESIAN_POINT('Ctrl Pts',(30.5472250361189,617.416731756641,-34.8378623034417)) ;
#66374=CARTESIAN_POINT('Ctrl Pts',(28.4093472456823,617.305509510783,-35.2852311354723)) ;
#66375=CARTESIAN_POINT('Ctrl Pts',(27.627128487621,617.194287264926,-37.3247297570932)) ;
#66376=CARTESIAN_POINT('Ctrl Pts',(28.9180668754785,617.083065019068,-39.0869235042828)) ;
#66377=CARTESIAN_POINT('Ctrl Pts',(31.0978517893876,616.971842773211,-38.9570094927081)) ;
#66378=CARTESIAN_POINT('Ctrl Pts',(32.1711152487225,616.860620527352,-37.0537440219648)) ;
#66379=CARTESIAN_POINT('Ctrl Pts',(31.1487648950217,616.749382406728,-35.123261185772)) ;
#66380=CARTESIAN_POINT('Ctrl Pts',(29.7031752837495,616.675218368056,-34.9971218697011)) ;
#66381=CARTESIAN_POINT('Ctrl Pts',(29.1147737982774,616.638128411336,-35.2547419366944)) ;
#66382=CARTESIAN_POINT('Ctrl Pts',(31.225514820522,618.939653785104,-35.4514041874778)) ;
#66383=CARTESIAN_POINT('Ctrl Pts',(30.7026141797248,618.902565412218,-35.0062954289854)) ;
#66384=CARTESIAN_POINT('Ctrl Pts',(29.1839313688666,618.828402957379,-34.6897204969993)) ;
#66385=CARTESIAN_POINT('Ctrl Pts',(27.542135731949,618.717166420589,-36.3506694737735)) ;
#66386=CARTESIAN_POINT('Ctrl Pts',(28.0539597431221,618.605944174731,-38.6299504183026)) ;
#66387=CARTESIAN_POINT('Ctrl Pts',(30.245317004706,618.494721928873,-39.4350656119731)) ;
#66388=CARTESIAN_POINT('Ctrl Pts',(32.1101948885357,618.383499683015,-38.0291857467188)) ;
#66389=CARTESIAN_POINT('Ctrl Pts',(31.9383159907009,618.272277437158,-35.7001867652823)) ;
#66390=CARTESIAN_POINT('Ctrl Pts',(29.8877438198984,618.161055191301,-34.5830193063753)) ;
#66391=CARTESIAN_POINT('Ctrl Pts',(27.8378058173618,618.049832945444,-35.7015107147504)) ;
#66392=CARTESIAN_POINT('Ctrl Pts',(27.6675473701414,617.938610699587,-38.0305164127401)) ;
#66393=CARTESIAN_POINT('Ctrl Pts',(29.5329898787488,617.827388453729,-39.435275783779)) ;
#66394=CARTESIAN_POINT('Ctrl Pts',(31.7243111256318,617.716166207871,-38.6282219835898)) ;
#66395=CARTESIAN_POINT('Ctrl Pts',(32.2329969066591,617.604943962014,-36.3490786672756)) ;
#66396=CARTESIAN_POINT('Ctrl Pts',(30.5927516681446,617.493721716156,-34.6868920344383)) ;
#66397=CARTESIAN_POINT('Ctrl Pts',(28.30711198598,617.3824994703,-35.1651812797949)) ;
#66398=CARTESIAN_POINT('Ctrl Pts',(27.4708292753611,617.271277224442,-37.3456422033094)) ;
#66399=CARTESIAN_POINT('Ctrl Pts',(28.850992360321,617.160054978585,-39.2296320058398)) ;
#66400=CARTESIAN_POINT('Ctrl Pts',(31.1814356251799,617.048832732727,-39.0907388373655)) ;
#66401=CARTESIAN_POINT('Ctrl Pts',(32.3288789276206,616.937610486869,-37.0559269762365)) ;
#66402=CARTESIAN_POINT('Ctrl Pts',(31.2358676488905,616.826372366244,-34.9920165900219)) ;
#66403=CARTESIAN_POINT('Ctrl Pts',(29.6903644426602,616.752208327571,-34.8571590094894)) ;
#66404=CARTESIAN_POINT('Ctrl Pts',(29.0612949091931,616.715118370851,-35.1325847848427)) ;
#66405=CARTESIAN_POINT('Ctrl Pts',(177.897694697021,618.70737979957,-37.5528661540161)) ;
#66406=CARTESIAN_POINT('Ctrl Pts',(178.074357719121,618.67028873138,-38.21568333661)) ;
#66407=CARTESIAN_POINT('Ctrl Pts',(179.142367773108,618.596123581238,-39.3386569433631)) ;
#66408=CARTESIAN_POINT('Ctrl Pts',(181.434831201881,618.484884349142,-38.9068792628014)) ;
#66409=CARTESIAN_POINT('Ctrl Pts',(182.309288473454,618.373662103284,-36.7435478468336)) ;
#66410=CARTESIAN_POINT('Ctrl Pts',(180.96634315944,618.262439857427,-34.8371019767222)) ;
#66411=CARTESIAN_POINT('Ctrl Pts',(178.635482469432,618.15121761157,-34.9325952570238)) ;
#66412=CARTESIAN_POINT('Ctrl Pts',(177.453462591305,618.039995365713,-36.9436498335109)) ;
#66413=CARTESIAN_POINT('Ctrl Pts',(178.503397865929,617.928773119855,-39.0264888319928)) ;
#66414=CARTESIAN_POINT('Ctrl Pts',(180.822992703844,617.817550873998,-39.2722505476327)) ;
#66415=CARTESIAN_POINT('Ctrl Pts',(182.286079804168,617.70632862814,-37.4555779132756)) ;
#66416=CARTESIAN_POINT('Ctrl Pts',(181.551623139311,617.595106382283,-35.2416494112721)) ;
#66417=CARTESIAN_POINT('Ctrl Pts',(179.292809605602,617.483884136426,-34.6596980177064)) ;
#66418=CARTESIAN_POINT('Ctrl Pts',(177.580012828887,617.372661890568,-36.24312800518)) ;
#66419=CARTESIAN_POINT('Ctrl Pts',(177.983200659197,617.261439644711,-38.5405958736053)) ;
#66420=CARTESIAN_POINT('Ctrl Pts',(180.132717649286,617.150217398854,-39.4462222224988)) ;
#66421=CARTESIAN_POINT('Ctrl Pts',(182.058589537804,617.038995152996,-38.1299665592977)) ;
#66422=CARTESIAN_POINT('Ctrl Pts',(181.995096791643,616.927772907139,-35.7980147600553)) ;
#66423=CARTESIAN_POINT('Ctrl Pts',(180.001605178594,616.816550661281,-34.5880440328019)) ;
#66424=CARTESIAN_POINT('Ctrl Pts',(177.902860787058,616.705328415424,-35.607823574719)) ;
#66425=CARTESIAN_POINT('Ctrl Pts',(177.628241205805,616.594091799347,-37.9243184862603)) ;
#66426=CARTESIAN_POINT('Ctrl Pts',(178.821262568672,616.519929265223,-38.913342614159)) ;
#66427=CARTESIAN_POINT('Ctrl Pts',(179.494515316492,616.482840813051,-39.0444902412825)) ;
#66428=CARTESIAN_POINT('Ctrl Pts',(178.025790309075,618.783918479111,-37.518719085898)) ;
#66429=CARTESIAN_POINT('Ctrl Pts',(178.191086351244,618.746827410922,-38.1388888059787)) ;
#66430=CARTESIAN_POINT('Ctrl Pts',(179.19037772995,618.672662260779,-39.1896072327892)) ;
#66431=CARTESIAN_POINT('Ctrl Pts',(181.335337818873,618.561423028684,-38.7856113040128)) ;
#66432=CARTESIAN_POINT('Ctrl Pts',(182.15353012827,618.450200782827,-36.761474522537)) ;
#66433=CARTESIAN_POINT('Ctrl Pts',(180.89699357287,618.338978536969,-34.9776945713462)) ;
#66434=CARTESIAN_POINT('Ctrl Pts',(178.716106807064,618.227756291112,-35.0670435539458)) ;
#66435=CARTESIAN_POINT('Ctrl Pts',(177.610141306776,618.116534045255,-36.9487014024733)) ;
#66436=CARTESIAN_POINT('Ctrl Pts',(178.592520886643,618.005311799398,-38.8975248678011)) ;
#66437=CARTESIAN_POINT('Ctrl Pts',(180.762866675961,617.89408955354,-39.127473605398)) ;
#66438=CARTESIAN_POINT('Ctrl Pts',(182.131814767968,617.782867307682,-37.4276906355025)) ;
#66439=CARTESIAN_POINT('Ctrl Pts',(181.444615045002,617.671645061825,-35.3562123222927)) ;
#66440=CARTESIAN_POINT('Ctrl Pts',(179.331139725258,617.560422815968,-34.8117052661604)) ;
#66441=CARTESIAN_POINT('Ctrl Pts',(177.728548957449,617.449200570111,-36.2932530562397)) ;
#66442=CARTESIAN_POINT('Ctrl Pts',(178.105794584794,617.337978324254,-38.4428955855411)) ;
#66443=CARTESIAN_POINT('Ctrl Pts',(180.117005798173,617.226756078396,-39.2902514689432)) ;
#66444=CARTESIAN_POINT('Ctrl Pts',(181.918961844844,617.115533832538,-38.0586872795428)) ;
#66445=CARTESIAN_POINT('Ctrl Pts',(181.859554394874,617.004311586681,-35.8767796094398)) ;
#66446=CARTESIAN_POINT('Ctrl Pts',(179.99432946089,616.893089340824,-34.7446616937728)) ;
#66447=CARTESIAN_POINT('Ctrl Pts',(178.030623998811,616.781867094967,-35.6988258428971)) ;
#66448=CARTESIAN_POINT('Ctrl Pts',(177.773674189261,616.67063047889,-37.8662711635459)) ;
#66449=CARTESIAN_POINT('Ctrl Pts',(178.889933308802,616.596467944766,-38.7916587857429)) ;
#66450=CARTESIAN_POINT('Ctrl Pts',(179.519867141423,616.559379492594,-38.9143680173957)) ;
#66451=CARTESIAN_POINT('Ctrl Pts',(178.153885921129,618.860457158654,-37.48457201778)) ;
#66452=CARTESIAN_POINT('Ctrl Pts',(178.307814983366,618.823366090463,-38.0620942753473)) ;
#66453=CARTESIAN_POINT('Ctrl Pts',(179.238387686792,618.749200940321,-39.0405575222152)) ;
#66454=CARTESIAN_POINT('Ctrl Pts',(181.235844435868,618.637961708226,-38.6643433452239)) ;
#66455=CARTESIAN_POINT('Ctrl Pts',(181.997771783088,618.526739462368,-36.7794011982405)) ;
#66456=CARTESIAN_POINT('Ctrl Pts',(180.827643986302,618.415517216512,-35.1182871659701)) ;
#66457=CARTESIAN_POINT('Ctrl Pts',(178.796731144695,618.304294970654,-35.2014918508676)) ;
#66458=CARTESIAN_POINT('Ctrl Pts',(177.766820022244,618.193072724797,-36.9537529714359)) ;
#66459=CARTESIAN_POINT('Ctrl Pts',(178.681643907358,618.081850478939,-38.7685609036097)) ;
#66460=CARTESIAN_POINT('Ctrl Pts',(180.702740648078,617.970628233082,-38.9826966631632)) ;
#66461=CARTESIAN_POINT('Ctrl Pts',(181.977549731769,617.859405987224,-37.3998033577292)) ;
#66462=CARTESIAN_POINT('Ctrl Pts',(181.337606950692,617.748183741368,-35.4707752333133)) ;
#66463=CARTESIAN_POINT('Ctrl Pts',(179.369469844914,617.636961495509,-34.9637125146143)) ;
#66464=CARTESIAN_POINT('Ctrl Pts',(177.877085086011,617.525739249652,-36.3433781072996)) ;
#66465=CARTESIAN_POINT('Ctrl Pts',(178.228388510391,617.414517003795,-38.3451952974769)) ;
#66466=CARTESIAN_POINT('Ctrl Pts',(180.101293947058,617.303294757937,-39.1342807153876)) ;
#66467=CARTESIAN_POINT('Ctrl Pts',(181.779334151885,617.19207251208,-37.9874079997878)) ;
#66468=CARTESIAN_POINT('Ctrl Pts',(181.724011998105,617.080850266222,-35.9555444588244)) ;
#66469=CARTESIAN_POINT('Ctrl Pts',(179.987053743187,616.969628020365,-34.9012793547438)) ;
#66470=CARTESIAN_POINT('Ctrl Pts',(178.158387210564,616.858405774508,-35.7898281110753)) ;
#66471=CARTESIAN_POINT('Ctrl Pts',(177.919107172716,616.747169158432,-37.8082238408314)) ;
#66472=CARTESIAN_POINT('Ctrl Pts',(178.958604048933,616.673006624308,-38.6699749573269)) ;
#66473=CARTESIAN_POINT('Ctrl Pts',(179.545218966355,616.635918172135,-38.784245793509)) ;
#66474=CARTESIAN_POINT('Ctrl Pts',(178.281981533183,618.936995838197,-37.4504249496618)) ;
#66475=CARTESIAN_POINT('Ctrl Pts',(178.42454361549,618.899904770007,-37.9852997447159)) ;
#66476=CARTESIAN_POINT('Ctrl Pts',(179.286397643634,618.825739619865,-38.891507811641)) ;
#66477=CARTESIAN_POINT('Ctrl Pts',(181.136351052861,618.714500387769,-38.5430753864352)) ;
#66478=CARTESIAN_POINT('Ctrl Pts',(181.842013437904,618.603278141912,-36.797327873944)) ;
#66479=CARTESIAN_POINT('Ctrl Pts',(180.758294399734,618.492055896054,-35.2588797605942)) ;
#66480=CARTESIAN_POINT('Ctrl Pts',(178.877355482327,618.380833650197,-35.3359401477894)) ;
#66481=CARTESIAN_POINT('Ctrl Pts',(177.923498737714,618.26961140434,-36.9588045403982)) ;
#66482=CARTESIAN_POINT('Ctrl Pts',(178.770766928071,618.158389158483,-38.6395969394181)) ;
#66483=CARTESIAN_POINT('Ctrl Pts',(180.642614620195,618.047166912625,-38.8379197209285)) ;
#66484=CARTESIAN_POINT('Ctrl Pts',(181.823284695569,617.935944666768,-37.3719160799559)) ;
#66485=CARTESIAN_POINT('Ctrl Pts',(181.230598856383,617.82472242091,-35.5853381443338)) ;
#66486=CARTESIAN_POINT('Ctrl Pts',(179.40779996457,617.713500175053,-35.1157197630681)) ;
#66487=CARTESIAN_POINT('Ctrl Pts',(178.025621214571,617.602277929196,-36.3935031583595)) ;
#66488=CARTESIAN_POINT('Ctrl Pts',(178.350982435989,617.491055683339,-38.2474950094128)) ;
#66489=CARTESIAN_POINT('Ctrl Pts',(180.085582095943,617.379833437481,-38.978309961832)) ;
#66490=CARTESIAN_POINT('Ctrl Pts',(181.639706458925,617.268611191623,-37.9161287200328)) ;
#66491=CARTESIAN_POINT('Ctrl Pts',(181.588469601338,617.157388945766,-36.0343093082089)) ;
#66492=CARTESIAN_POINT('Ctrl Pts',(179.979778025483,617.046166699909,-35.0578970157147)) ;
#66493=CARTESIAN_POINT('Ctrl Pts',(178.286150422316,616.934944454052,-35.8808303792533)) ;
#66494=CARTESIAN_POINT('Ctrl Pts',(178.064540156171,616.823707837974,-37.7501765181169)) ;
#66495=CARTESIAN_POINT('Ctrl Pts',(179.027274789061,616.74954530385,-38.5482911289107)) ;
#66496=CARTESIAN_POINT('Ctrl Pts',(179.570570791287,616.712456851679,-38.6541235696222)) ;
#66497=CARTESIAN_POINT('Ctrl Pts',(180.966205148325,618.708673473592,-35.7560589666014)) ;
#66498=CARTESIAN_POINT('Ctrl Pts',(180.544722495663,618.671585021452,-35.3972784943684)) ;
#66499=CARTESIAN_POINT('Ctrl Pts',(179.32047618186,618.59742248736,-35.1421985305261)) ;
#66500=CARTESIAN_POINT('Ctrl Pts',(177.997134246167,618.486185871316,-36.4809786807734)) ;
#66501=CARTESIAN_POINT('Ctrl Pts',(178.409698571325,618.374963625458,-38.3182006227404)) ;
#66502=CARTESIAN_POINT('Ctrl Pts',(180.176091219243,618.263741379601,-38.9671432459311)) ;
#66503=CARTESIAN_POINT('Ctrl Pts',(181.679302531611,618.152519133743,-37.8339066297847)) ;
#66504=CARTESIAN_POINT('Ctrl Pts',(181.540768571018,618.041296887886,-35.9565841108305)) ;
#66505=CARTESIAN_POINT('Ctrl Pts',(179.887889235789,617.930074642029,-35.0560751610428)) ;
#66506=CARTESIAN_POINT('Ctrl Pts',(178.235520635928,617.818852396172,-35.9576425269521)) ;
#66507=CARTESIAN_POINT('Ctrl Pts',(178.098283704118,617.707630150314,-37.8349583017894)) ;
#66508=CARTESIAN_POINT('Ctrl Pts',(179.601942656214,617.596407904457,-38.9672775885259)) ;
#66509=CARTESIAN_POINT('Ctrl Pts',(181.368279105258,617.485185658599,-38.3167449143955)) ;
#66510=CARTESIAN_POINT('Ctrl Pts',(181.778311152633,617.373963412741,-36.4796215614246)) ;
#66511=CARTESIAN_POINT('Ctrl Pts',(180.456178212682,617.262741166885,-35.1398043372561)) ;
#66512=CARTESIAN_POINT('Ctrl Pts',(178.613818725341,617.151518921027,-35.5253403081863)) ;
#66513=CARTESIAN_POINT('Ctrl Pts',(177.939732202149,617.04029667517,-37.2829349308624)) ;
#66514=CARTESIAN_POINT('Ctrl Pts',(179.052230194514,616.929074429313,-38.8015585494034)) ;
#66515=CARTESIAN_POINT('Ctrl Pts',(180.930725121544,616.817852183455,-38.6896374882165)) ;
#66516=CARTESIAN_POINT('Ctrl Pts',(181.855632185436,616.706629937598,-37.0494726460127)) ;
#66517=CARTESIAN_POINT('Ctrl Pts',(180.974626616194,616.595391473834,-35.38588823888)) ;
#66518=CARTESIAN_POINT('Ctrl Pts',(179.728787178078,616.521227092025,-35.2770659283329)) ;
#66519=CARTESIAN_POINT('Ctrl Pts',(179.221724915396,616.484136792166,-35.499079332989)) ;
#66520=CARTESIAN_POINT('Ctrl Pts',(181.052660894574,618.785683087004,-35.6544870935763)) ;
#66521=CARTESIAN_POINT('Ctrl Pts',(180.597365161011,618.748594634865,-35.2669237685818)) ;
#66522=CARTESIAN_POINT('Ctrl Pts',(179.274904746605,618.674432100772,-34.9913802354821)) ;
#66523=CARTESIAN_POINT('Ctrl Pts',(177.845398849837,618.563195484728,-36.4375628642004)) ;
#66524=CARTESIAN_POINT('Ctrl Pts',(178.291060790793,618.45197323887,-38.4221743458409)) ;
#66525=CARTESIAN_POINT('Ctrl Pts',(180.199160759592,618.340750993013,-39.1231778291386)) ;
#66526=CARTESIAN_POINT('Ctrl Pts',(181.822965898053,618.229528747155,-37.89902828659)) ;
#66527=CARTESIAN_POINT('Ctrl Pts',(181.673318170411,618.118306501298,-35.8710991938916)) ;
#66528=CARTESIAN_POINT('Ctrl Pts',(179.887838021533,618.00708425544,-34.8983476932453)) ;
#66529=CARTESIAN_POINT('Ctrl Pts',(178.102909581328,617.895862009583,-35.8722425205302)) ;
#66530=CARTESIAN_POINT('Ctrl Pts',(177.95466293548,617.784639763726,-37.9001643280707)) ;
#66531=CARTESIAN_POINT('Ctrl Pts',(179.578951625178,617.673417517868,-39.1233229492518)) ;
#66532=CARTESIAN_POINT('Ctrl Pts',(181.486990886596,617.562195272011,-38.4206018545543)) ;
#66533=CARTESIAN_POINT('Ctrl Pts',(181.929917399976,617.450973026154,-36.4360968711268)) ;
#66534=CARTESIAN_POINT('Ctrl Pts',(180.501717489587,617.339750780296,-34.9887939701297)) ;
#66535=CARTESIAN_POINT('Ctrl Pts',(178.511556307444,617.228528534439,-35.4052592305405)) ;
#66536=CARTESIAN_POINT('Ctrl Pts',(177.783391776534,617.117306288582,-37.3038553601391)) ;
#66537=CARTESIAN_POINT('Ctrl Pts',(178.985138957165,617.006084042724,-38.9443092436912)) ;
#66538=CARTESIAN_POINT('Ctrl Pts',(181.014334513363,616.894861796867,-38.823409412269)) ;
#66539=CARTESIAN_POINT('Ctrl Pts',(182.013441445692,616.78363955101,-37.0516637656131)) ;
#66540=CARTESIAN_POINT('Ctrl Pts',(181.061757967411,616.672401087247,-35.2546197397083)) ;
#66541=CARTESIAN_POINT('Ctrl Pts',(179.71597213899,616.598236705436,-35.137067253513)) ;
#66542=CARTESIAN_POINT('Ctrl Pts',(179.168231245286,616.561146405578,-35.3768914913441)) ;
#66543=CARTESIAN_POINT('Ctrl Pts',(181.139116640822,618.862692700416,-35.5529152205513)) ;
#66544=CARTESIAN_POINT('Ctrl Pts',(180.650007826359,618.825604248277,-35.1365690427952)) ;
#66545=CARTESIAN_POINT('Ctrl Pts',(179.22933331135,618.751441714185,-34.840561940438)) ;
#66546=CARTESIAN_POINT('Ctrl Pts',(177.693663453507,618.64020509814,-36.3941470476275)) ;
#66547=CARTESIAN_POINT('Ctrl Pts',(178.172423010261,618.528982852283,-38.5261480689413)) ;
#66548=CARTESIAN_POINT('Ctrl Pts',(180.222230299942,618.417760606425,-39.2792124123461)) ;
#66549=CARTESIAN_POINT('Ctrl Pts',(181.966629264493,618.306538360567,-37.9641499433951)) ;
#66550=CARTESIAN_POINT('Ctrl Pts',(181.805867769802,618.19531611471,-35.7856142769528)) ;
#66551=CARTESIAN_POINT('Ctrl Pts',(179.887786807278,618.084093868853,-34.740620225448)) ;
#66552=CARTESIAN_POINT('Ctrl Pts',(177.970298526728,617.972871622996,-35.7868425141084)) ;
#66553=CARTESIAN_POINT('Ctrl Pts',(177.811042166842,617.861649377138,-37.9653703543519)) ;
#66554=CARTESIAN_POINT('Ctrl Pts',(179.555960594141,617.750427131281,-39.2793683099778)) ;
#66555=CARTESIAN_POINT('Ctrl Pts',(181.605702667935,617.639204885423,-38.5244587947131)) ;
#66556=CARTESIAN_POINT('Ctrl Pts',(182.081523647319,617.527982639565,-36.3925721808291)) ;
#66557=CARTESIAN_POINT('Ctrl Pts',(180.547256766493,617.416760393708,-34.8377836030034)) ;
#66558=CARTESIAN_POINT('Ctrl Pts',(178.409293889545,617.305538147851,-35.2851781528945)) ;
#66559=CARTESIAN_POINT('Ctrl Pts',(177.627051350921,617.194315901994,-37.3247757894159)) ;
#66560=CARTESIAN_POINT('Ctrl Pts',(178.918047719815,617.083093656137,-39.0870599379789)) ;
#66561=CARTESIAN_POINT('Ctrl Pts',(181.097943905179,616.971871410279,-38.9571813363214)) ;
#66562=CARTESIAN_POINT('Ctrl Pts',(182.17125070595,616.860649164421,-37.0538548852137)) ;
#66563=CARTESIAN_POINT('Ctrl Pts',(181.148889318629,616.749410700658,-35.1233512405364)) ;
#66564=CARTESIAN_POINT('Ctrl Pts',(179.703157099901,616.675246318848,-34.9970685786932)) ;
#66565=CARTESIAN_POINT('Ctrl Pts',(179.114737575175,616.63815601899,-35.2547036496991)) ;
#66566=CARTESIAN_POINT('Ctrl Pts',(181.225572387071,618.939702313829,-35.4513433475264)) ;
#66567=CARTESIAN_POINT('Ctrl Pts',(180.702650491707,618.902613861688,-35.0062143170084)) ;
#66568=CARTESIAN_POINT('Ctrl Pts',(179.183761876095,618.828451327597,-34.6897436453939)) ;
#66569=CARTESIAN_POINT('Ctrl Pts',(177.541928057179,618.717214711552,-36.3507312310546)) ;
#66570=CARTESIAN_POINT('Ctrl Pts',(178.05378522973,618.605992465694,-38.6301217920418)) ;
#66571=CARTESIAN_POINT('Ctrl Pts',(180.24529984029,618.494770219836,-39.4352469955538)) ;
#66572=CARTESIAN_POINT('Ctrl Pts',(182.110292630934,618.383547973979,-38.0292716002004)) ;
#66573=CARTESIAN_POINT('Ctrl Pts',(181.938417369194,618.272325728121,-35.7001293600139)) ;
#66574=CARTESIAN_POINT('Ctrl Pts',(179.887735593022,618.161103482264,-34.5828927576505)) ;
#66575=CARTESIAN_POINT('Ctrl Pts',(177.837687472128,618.049881236407,-35.7014425076866)) ;
#66576=CARTESIAN_POINT('Ctrl Pts',(177.667421398203,617.93865899055,-38.0305763806333)) ;
#66577=CARTESIAN_POINT('Ctrl Pts',(179.532969563104,617.827436744692,-39.4354136707037)) ;
#66578=CARTESIAN_POINT('Ctrl Pts',(181.724414449273,617.716214498834,-38.6283157348719)) ;
#66579=CARTESIAN_POINT('Ctrl Pts',(182.233129894662,617.604992252977,-36.3490474905313)) ;
#66580=CARTESIAN_POINT('Ctrl Pts',(180.592796043397,617.49377000712,-34.6867732358772)) ;
#66581=CARTESIAN_POINT('Ctrl Pts',(178.307031471648,617.382547761263,-35.1650970752487)) ;
#66582=CARTESIAN_POINT('Ctrl Pts',(177.470710925308,617.271325515405,-37.3456962186925)) ;
#66583=CARTESIAN_POINT('Ctrl Pts',(178.850956482466,617.160103269548,-39.2298106322666)) ;
#66584=CARTESIAN_POINT('Ctrl Pts',(181.181553296997,617.04888102369,-39.090953260374)) ;
#66585=CARTESIAN_POINT('Ctrl Pts',(182.329059966206,616.937658777833,-37.0560460048141)) ;
#66586=CARTESIAN_POINT('Ctrl Pts',(181.236020669846,616.82642031407,-34.9920827413645)) ;
#66587=CARTESIAN_POINT('Ctrl Pts',(179.690342060812,616.752255932259,-34.8570699038733)) ;
#66588=CARTESIAN_POINT('Ctrl Pts',(179.061243905064,616.715165632402,-35.1325158080541)) ;
#66589=CARTESIAN_POINT('Ctrl Pts',(27.8977541328133,503.71371705854,-36.4914598282363)) ;
#66590=CARTESIAN_POINT('Ctrl Pts',(28.0744148476991,503.75080794899,-35.8286657489856)) ;
#66591=CARTESIAN_POINT('Ctrl Pts',(29.1420348524557,503.824972921393,-34.7056981288284)) ;
#66592=CARTESIAN_POINT('Ctrl Pts',(31.4345215740258,503.936211975746,-35.1374809470855)) ;
#66593=CARTESIAN_POINT('Ctrl Pts',(32.308955341866,504.047434221604,-37.300709716721)) ;
#66594=CARTESIAN_POINT('Ctrl Pts',(30.9661821194376,504.158656467462,-39.207060501706)) ;
#66595=CARTESIAN_POINT('Ctrl Pts',(28.6354901248007,504.269878713319,-39.1115873870729)) ;
#66596=CARTESIAN_POINT('Ctrl Pts',(27.4535723582629,504.381100959177,-37.1006559333751)) ;
#66597=CARTESIAN_POINT('Ctrl Pts',(28.5034591693879,504.492323205034,-35.017943588011)) ;
#66598=CARTESIAN_POINT('Ctrl Pts',(30.8229284125707,504.603545450891,-34.7721976604505)) ;
#66599=CARTESIAN_POINT('Ctrl Pts',(32.2859340628205,504.714767696748,-36.5887649780755)) ;
#66600=CARTESIAN_POINT('Ctrl Pts',(31.5515227471191,504.825989942606,-38.8025634523413)) ;
#66601=CARTESIAN_POINT('Ctrl Pts',(29.2928420280764,504.937212188463,-39.3844784587789)) ;
#66602=CARTESIAN_POINT('Ctrl Pts',(27.5801447756113,505.048434434321,-37.8011369057575)) ;
#66603=CARTESIAN_POINT('Ctrl Pts',(27.9833082997518,505.159656680178,-35.5037932649875)) ;
#66604=CARTESIAN_POINT('Ctrl Pts',(30.1326956298288,505.270878926035,-34.5982066401904)) ;
#66605=CARTESIAN_POINT('Ctrl Pts',(32.0584516367322,505.382101171892,-35.9143520425694)) ;
#66606=CARTESIAN_POINT('Ctrl Pts',(31.994950262249,505.49332341775,-38.2461341646642)) ;
#66607=CARTESIAN_POINT('Ctrl Pts',(30.0015652353422,505.604545663607,-39.455939676632)) ;
#66608=CARTESIAN_POINT('Ctrl Pts',(27.9029216508139,505.715767909465,-38.4361905755117)) ;
#66609=CARTESIAN_POINT('Ctrl Pts',(27.6282984704502,505.82700437211,-36.1196715697614)) ;
#66610=CARTESIAN_POINT('Ctrl Pts',(28.8212881368412,505.9011667528,-35.1310360076914)) ;
#66611=CARTESIAN_POINT('Ctrl Pts',(29.4945182216124,505.938255051539,-34.9998895262024)) ;
#66612=CARTESIAN_POINT('Ctrl Pts',(28.025819091536,503.637196597121,-36.5255993814499)) ;
#66613=CARTESIAN_POINT('Ctrl Pts',(28.1911153557476,503.67428748757,-35.9054423458996)) ;
#66614=CARTESIAN_POINT('Ctrl Pts',(29.1900561700542,503.748452459973,-34.8547143865864)) ;
#66615=CARTESIAN_POINT('Ctrl Pts',(31.3350689482234,503.859691514327,-35.2587209414953)) ;
#66616=CARTESIAN_POINT('Ctrl Pts',(32.1532510506677,503.970913760184,-37.2827908343813)) ;
#66617=CARTESIAN_POINT('Ctrl Pts',(30.8968574178533,504.082136006042,-39.066507509811)) ;
#66618=CARTESIAN_POINT('Ctrl Pts',(28.7160970830456,504.1933582519,-38.9771761087029)) ;
#66619=CARTESIAN_POINT('Ctrl Pts',(27.6102111958496,504.304580497757,-37.0956063601769)) ;
#66620=CARTESIAN_POINT('Ctrl Pts',(28.5925595795087,504.415802743614,-35.1468733306579)) ;
#66621=CARTESIAN_POINT('Ctrl Pts',(30.7628191140068,504.527024989472,-34.916936053447)) ;
#66622=CARTESIAN_POINT('Ctrl Pts',(32.1317107131565,504.638247235329,-36.6166449643197)) ;
#66623=CARTESIAN_POINT('Ctrl Pts',(31.4445435240122,504.749469481186,-38.6880314508418)) ;
#66624=CARTESIAN_POINT('Ctrl Pts',(29.331162033701,504.860691727044,-39.2325123033906)) ;
#66625=CARTESIAN_POINT('Ctrl Pts',(27.7286413049629,504.971913972901,-37.751025919421)) ;
#66626=CARTESIAN_POINT('Ctrl Pts',(28.1058696233806,505.083136218759,-35.6014686640044)) ;
#66627=CARTESIAN_POINT('Ctrl Pts',(30.1169884860854,505.194358464616,-34.7541377444173)) ;
#66628=CARTESIAN_POINT('Ctrl Pts',(31.9188620601296,505.305580710473,-35.985616504782)) ;
#66629=CARTESIAN_POINT('Ctrl Pts',(31.8594456812183,505.41680295633,-38.1673968399694)) ;
#66630=CARTESIAN_POINT('Ctrl Pts',(29.9942936110689,505.528025202188,-39.2993764749454)) ;
#66631=CARTESIAN_POINT('Ctrl Pts',(28.0306541869974,505.639247448046,-38.3452270651154)) ;
#66632=CARTESIAN_POINT('Ctrl Pts',(27.7736973088966,505.75048391069,-36.1777279814988)) ;
#66633=CARTESIAN_POINT('Ctrl Pts',(28.8899428489712,505.824646291381,-35.2526906001961)) ;
#66634=CARTESIAN_POINT('Ctrl Pts',(29.5198645496706,505.86173459012,-35.1299806730418)) ;
#66635=CARTESIAN_POINT('Ctrl Pts',(28.1538840502585,503.560676135701,-36.5597389346635)) ;
#66636=CARTESIAN_POINT('Ctrl Pts',(28.3078158637961,503.597767026151,-35.9822189428135)) ;
#66637=CARTESIAN_POINT('Ctrl Pts',(29.2380774876526,503.671931998554,-35.0037306443446)) ;
#66638=CARTESIAN_POINT('Ctrl Pts',(31.2356163224208,503.783171052908,-35.379960935905)) ;
#66639=CARTESIAN_POINT('Ctrl Pts',(31.9975467594692,503.894393298765,-37.2648719520417)) ;
#66640=CARTESIAN_POINT('Ctrl Pts',(30.8275327162687,504.005615544622,-38.9259545179161)) ;
#66641=CARTESIAN_POINT('Ctrl Pts',(28.7967040412908,504.11683779048,-38.842764830333)) ;
#66642=CARTESIAN_POINT('Ctrl Pts',(27.7668500334364,504.228060036338,-37.0905567869785)) ;
#66643=CARTESIAN_POINT('Ctrl Pts',(28.6816599896297,504.339282282195,-35.2758030733051)) ;
#66644=CARTESIAN_POINT('Ctrl Pts',(30.7027098154429,504.450504528052,-35.0616744464435)) ;
#66645=CARTESIAN_POINT('Ctrl Pts',(31.9774873634924,504.561726773909,-36.6445249505641)) ;
#66646=CARTESIAN_POINT('Ctrl Pts',(31.3375643009055,504.672949019767,-38.5734994493424)) ;
#66647=CARTESIAN_POINT('Ctrl Pts',(29.3694820393255,504.784171265625,-39.0805461480023)) ;
#66648=CARTESIAN_POINT('Ctrl Pts',(27.8771378343143,504.895393511482,-37.7009149330845)) ;
#66649=CARTESIAN_POINT('Ctrl Pts',(28.2284309470095,505.006615757339,-35.6991440630211)) ;
#66650=CARTESIAN_POINT('Ctrl Pts',(30.1012813423422,505.117838003197,-34.9100688486442)) ;
#66651=CARTESIAN_POINT('Ctrl Pts',(31.7792724835269,505.229060249053,-36.0568809669946)) ;
#66652=CARTESIAN_POINT('Ctrl Pts',(31.7239411001876,505.340282494911,-38.0886595152747)) ;
#66653=CARTESIAN_POINT('Ctrl Pts',(29.9870219867958,505.451504740768,-39.1428132732589)) ;
#66654=CARTESIAN_POINT('Ctrl Pts',(28.1583867231806,505.562726986626,-38.254263554719)) ;
#66655=CARTESIAN_POINT('Ctrl Pts',(27.9190961473432,505.673963449271,-36.2357843932362)) ;
#66656=CARTESIAN_POINT('Ctrl Pts',(28.9585975611013,505.748125829961,-35.3743451927006)) ;
#66657=CARTESIAN_POINT('Ctrl Pts',(29.5452108777287,505.7852141287,-35.2600718198812)) ;
#66658=CARTESIAN_POINT('Ctrl Pts',(28.2819490089811,503.484155674282,-36.5938784878771)) ;
#66659=CARTESIAN_POINT('Ctrl Pts',(28.4245163718447,503.521246564731,-36.0589955397274)) ;
#66660=CARTESIAN_POINT('Ctrl Pts',(29.2860988052509,503.595411537134,-35.1527469021027)) ;
#66661=CARTESIAN_POINT('Ctrl Pts',(31.1361636966183,503.706650591488,-35.5012009303147)) ;
#66662=CARTESIAN_POINT('Ctrl Pts',(31.8418424682708,503.817872837345,-37.2469530697021)) ;
#66663=CARTESIAN_POINT('Ctrl Pts',(30.7582080146843,503.929095083203,-38.7854015260211)) ;
#66664=CARTESIAN_POINT('Ctrl Pts',(28.8773109995357,504.040317329061,-38.708353551963)) ;
#66665=CARTESIAN_POINT('Ctrl Pts',(27.923488871023,504.151539574918,-37.0855072137802)) ;
#66666=CARTESIAN_POINT('Ctrl Pts',(28.7707603997505,504.262761820775,-35.4047328159522)) ;
#66667=CARTESIAN_POINT('Ctrl Pts',(30.6426005168789,504.373984066633,-35.20641283944)) ;
#66668=CARTESIAN_POINT('Ctrl Pts',(31.8232640138284,504.48520631249,-36.6724049368083)) ;
#66669=CARTESIAN_POINT('Ctrl Pts',(31.2305850777988,504.596428558347,-38.458967447843)) ;
#66670=CARTESIAN_POINT('Ctrl Pts',(29.4078020449499,504.707650804205,-38.9285799926139)) ;
#66671=CARTESIAN_POINT('Ctrl Pts',(28.0256343636658,504.818873050062,-37.650803946748)) ;
#66672=CARTESIAN_POINT('Ctrl Pts',(28.3509922706383,504.930095295921,-35.796819462038)) ;
#66673=CARTESIAN_POINT('Ctrl Pts',(30.085574198599,505.041317541777,-35.0659999528711)) ;
#66674=CARTESIAN_POINT('Ctrl Pts',(31.6396829069243,505.152539787634,-36.1281454292072)) ;
#66675=CARTESIAN_POINT('Ctrl Pts',(31.588436519157,505.263762033491,-38.0099221905798)) ;
#66676=CARTESIAN_POINT('Ctrl Pts',(29.9797503625226,505.374984279349,-38.9862500715725)) ;
#66677=CARTESIAN_POINT('Ctrl Pts',(28.2861192593641,505.486206525207,-38.1633000443226)) ;
#66678=CARTESIAN_POINT('Ctrl Pts',(28.0644949857897,505.597442987851,-36.2938408049737)) ;
#66679=CARTESIAN_POINT('Ctrl Pts',(29.0272522732312,505.671605368542,-35.4959997852053)) ;
#66680=CARTESIAN_POINT('Ctrl Pts',(29.5705572057869,505.70869366728,-35.3901629667207)) ;
#66681=CARTESIAN_POINT('Ctrl Pts',(30.9662230989071,503.71243666145,-38.2882930583653)) ;
#66682=CARTESIAN_POINT('Ctrl Pts',(30.5447314608486,503.749524960246,-38.6470777806288)) ;
#66683=CARTESIAN_POINT('Ctrl Pts',(29.3206848071998,503.823687340995,-38.9023459275938)) ;
#66684=CARTESIAN_POINT('Ctrl Pts',(27.9972632285561,503.934923803697,-37.5634843593214)) ;
#66685=CARTESIAN_POINT('Ctrl Pts',(28.4098167138482,504.046146049554,-35.7262492988704)) ;
#66686=CARTESIAN_POINT('Ctrl Pts',(30.1761400278415,504.157368295412,-35.0772583107157)) ;
#66687=CARTESIAN_POINT('Ctrl Pts',(31.6793239520214,504.268590541268,-36.2104609029163)) ;
#66688=CARTESIAN_POINT('Ctrl Pts',(31.5407717996218,504.379812787126,-38.0877489028456)) ;
#66689=CARTESIAN_POINT('Ctrl Pts',(29.8878999526904,504.491035032984,-38.9882411575102)) ;
#66690=CARTESIAN_POINT('Ctrl Pts',(28.2355391737867,504.602257278842,-38.0866757916757)) ;
#66691=CARTESIAN_POINT('Ctrl Pts',(28.0983010872981,504.713479524699,-36.2093732450915)) ;
#66692=CARTESIAN_POINT('Ctrl Pts',(29.6019455967526,504.824701770556,-35.0770627132181)) ;
#66693=CARTESIAN_POINT('Ctrl Pts',(31.3682656918741,504.935924016413,-35.7275911699162)) ;
#66694=CARTESIAN_POINT('Ctrl Pts',(31.7782928184681,505.04714626227,-37.5647021897656)) ;
#66695=CARTESIAN_POINT('Ctrl Pts',(30.4561667902946,505.158368508128,-38.9045152432018)) ;
#66696=CARTESIAN_POINT('Ctrl Pts',(28.6138192880979,505.269590753986,-38.5189930982623)) ;
#66697=CARTESIAN_POINT('Ctrl Pts',(27.9397253017718,505.380812999843,-36.7614367744957)) ;
#66698=CARTESIAN_POINT('Ctrl Pts',(29.0522068826185,505.4920352457,-35.2428536331562)) ;
#66699=CARTESIAN_POINT('Ctrl Pts',(30.9306493708943,505.603257491557,-35.3548410007556)) ;
#66700=CARTESIAN_POINT('Ctrl Pts',(31.855549839045,505.714479737415,-36.9950215303291)) ;
#66701=CARTESIAN_POINT('Ctrl Pts',(30.9744952911176,505.82571756818,-38.6586996936158)) ;
#66702=CARTESIAN_POINT('Ctrl Pts',(29.7288050765599,505.899881316993,-38.7672899890708)) ;
#66703=CARTESIAN_POINT('Ctrl Pts',(29.2217365356442,505.936970983854,-38.5452851357495)) ;
#66704=CARTESIAN_POINT('Ctrl Pts',(31.052637147478,503.635463816439,-38.3898167925285)) ;
#66705=CARTESIAN_POINT('Ctrl Pts',(30.5973485790445,503.672552115236,-38.7773703471557)) ;
#66706=CARTESIAN_POINT('Ctrl Pts',(29.2751528382168,503.746714495985,-39.0531069423909)) ;
#66707=CARTESIAN_POINT('Ctrl Pts',(27.8456138828295,503.857950958687,-37.6068899556027)) ;
#66708=CARTESIAN_POINT('Ctrl Pts',(28.2912476007037,503.969173204544,-35.6223378434861)) ;
#66709=CARTESIAN_POINT('Ctrl Pts',(30.1992019713357,504.080395450401,-34.9213080928504)) ;
#66710=CARTESIAN_POINT('Ctrl Pts',(31.82291735531,504.191617696258,-36.1453755223364)) ;
#66711=CARTESIAN_POINT('Ctrl Pts',(31.6732555223731,504.302839942116,-38.1731921830943)) ;
#66712=CARTESIAN_POINT('Ctrl Pts',(29.8878496233149,504.414062187973,-39.1458896045665)) ;
#66713=CARTESIAN_POINT('Ctrl Pts',(28.1029957718174,504.525284433831,-38.172033025464)) ;
#66714=CARTESIAN_POINT('Ctrl Pts',(27.9547533719926,504.636506679688,-36.1442006516409)) ;
#66715=CARTESIAN_POINT('Ctrl Pts',(29.57896627286,504.747728925545,-34.9210968115423)) ;
#66716=CARTESIAN_POINT('Ctrl Pts',(31.486917166518,504.858951171402,-35.6237873112628)) ;
#66717=CARTESIAN_POINT('Ctrl Pts',(31.9298219518792,504.97017341726,-37.6082054366929)) ;
#66718=CARTESIAN_POINT('Ctrl Pts',(30.5016824295189,505.081395663117,-39.0554502026324)) ;
#66719=CARTESIAN_POINT('Ctrl Pts',(28.5116079390836,505.192617908975,-38.6390153089833)) ;
#66720=CARTESIAN_POINT('Ctrl Pts',(27.7834623287988,505.303840154832,-36.7405309018553)) ;
#66721=CARTESIAN_POINT('Ctrl Pts',(28.9851472511506,505.41506240069,-35.1001815282536)) ;
#66722=CARTESIAN_POINT('Ctrl Pts',(31.0142109718713,505.526284646547,-35.221148502858)) ;
#66723=CARTESIAN_POINT('Ctrl Pts',(32.0132737576184,505.637506892404,-36.9928454426161)) ;
#66724=CARTESIAN_POINT('Ctrl Pts',(31.0615726380295,505.74874472317,-38.7899241528505)) ;
#66725=CARTESIAN_POINT('Ctrl Pts',(29.7159978667007,505.822908471983,-38.9072216641162)) ;
#66726=CARTESIAN_POINT('Ctrl Pts',(29.1682704879214,505.859998138843,-38.6674155500032)) ;
#66727=CARTESIAN_POINT('Ctrl Pts',(31.1390511960491,503.558490971429,-38.4913405266917)) ;
#66728=CARTESIAN_POINT('Ctrl Pts',(30.6499656972406,503.595579270226,-38.9076629136824)) ;
#66729=CARTESIAN_POINT('Ctrl Pts',(29.2296208692337,503.669741650975,-39.2038679571878)) ;
#66730=CARTESIAN_POINT('Ctrl Pts',(27.6939645371028,503.780978113676,-37.6502955518842)) ;
#66731=CARTESIAN_POINT('Ctrl Pts',(28.1726784875591,503.892200359534,-35.5184263881019)) ;
#66732=CARTESIAN_POINT('Ctrl Pts',(30.22226391483,504.003422605391,-34.7653578749853)) ;
#66733=CARTESIAN_POINT('Ctrl Pts',(31.9665107585986,504.114644851248,-36.0802901417566)) ;
#66734=CARTESIAN_POINT('Ctrl Pts',(31.8057392451245,504.225867097105,-38.2586354633428)) ;
#66735=CARTESIAN_POINT('Ctrl Pts',(29.8877992939395,504.337089342963,-39.3035380516228)) ;
#66736=CARTESIAN_POINT('Ctrl Pts',(27.9704523698482,504.448311588821,-38.2573902592525)) ;
#66737=CARTESIAN_POINT('Ctrl Pts',(27.811205656687,504.559533834678,-36.0790280581902)) ;
#66738=CARTESIAN_POINT('Ctrl Pts',(29.5559869489674,504.670756080535,-34.7651309098665)) ;
#66739=CARTESIAN_POINT('Ctrl Pts',(31.605568641162,504.781978326392,-35.5199834526092)) ;
#66740=CARTESIAN_POINT('Ctrl Pts',(32.0813510852903,504.893200572249,-37.6517086836202)) ;
#66741=CARTESIAN_POINT('Ctrl Pts',(30.5471980687433,505.004422818107,-39.206385162063)) ;
#66742=CARTESIAN_POINT('Ctrl Pts',(28.4093965900692,505.115645063965,-38.7590375197042)) ;
#66743=CARTESIAN_POINT('Ctrl Pts',(27.6271993558257,505.226867309822,-36.719625029215)) ;
#66744=CARTESIAN_POINT('Ctrl Pts',(28.9180876196827,505.338089555679,-34.957509423351)) ;
#66745=CARTESIAN_POINT('Ctrl Pts',(31.0977725728485,505.449311801536,-35.0874560049603)) ;
#66746=CARTESIAN_POINT('Ctrl Pts',(32.1709976761917,505.560534047393,-36.9906693549032)) ;
#66747=CARTESIAN_POINT('Ctrl Pts',(31.1486499849412,505.671771878159,-38.9211486120855)) ;
#66748=CARTESIAN_POINT('Ctrl Pts',(29.7031906568414,505.745935626972,-39.0471533391616)) ;
#66749=CARTESIAN_POINT('Ctrl Pts',(29.1148044401986,505.783025293834,-38.7895459642568)) ;
#66750=CARTESIAN_POINT('Ctrl Pts',(31.2254652446201,503.481518126418,-38.592864260855)) ;
#66751=CARTESIAN_POINT('Ctrl Pts',(30.7025828154366,503.518606425215,-39.0379554802091)) ;
#66752=CARTESIAN_POINT('Ctrl Pts',(29.1840889002507,503.592768805964,-39.3546289719847)) ;
#66753=CARTESIAN_POINT('Ctrl Pts',(27.5423151913762,503.704005268666,-37.6937011481655)) ;
#66754=CARTESIAN_POINT('Ctrl Pts',(28.0541093744144,503.815227514523,-35.4145149327176)) ;
#66755=CARTESIAN_POINT('Ctrl Pts',(30.2453258583243,503.92644976038,-34.60940765712)) ;
#66756=CARTESIAN_POINT('Ctrl Pts',(32.1101041618871,504.037672006237,-36.0152047611767)) ;
#66757=CARTESIAN_POINT('Ctrl Pts',(31.9382229678757,504.148894252095,-38.3440787435914)) ;
#66758=CARTESIAN_POINT('Ctrl Pts',(29.8877489645639,504.260116497952,-39.4611864986793)) ;
#66759=CARTESIAN_POINT('Ctrl Pts',(27.837908967879,504.37133874381,-38.3427474930407)) ;
#66760=CARTESIAN_POINT('Ctrl Pts',(27.6676579413815,504.482560989668,-36.0138554647395)) ;
#66761=CARTESIAN_POINT('Ctrl Pts',(29.5330076250747,504.593783235524,-34.6091650081907)) ;
#66762=CARTESIAN_POINT('Ctrl Pts',(31.7242201158058,504.705005481382,-35.4161795939558)) ;
#66763=CARTESIAN_POINT('Ctrl Pts',(32.2328802187016,504.81622772724,-37.6952119305476)) ;
#66764=CARTESIAN_POINT('Ctrl Pts',(30.5927137079678,504.927449973096,-39.3573201214937)) ;
#66765=CARTESIAN_POINT('Ctrl Pts',(28.3071852410547,505.038672218954,-38.8790597304251)) ;
#66766=CARTESIAN_POINT('Ctrl Pts',(27.4709363828527,505.149894464812,-36.6987191565747)) ;
#66767=CARTESIAN_POINT('Ctrl Pts',(28.8510279882148,505.261116710669,-34.8148373184484)) ;
#66768=CARTESIAN_POINT('Ctrl Pts',(31.1813341738256,505.372338956526,-34.9537635070626)) ;
#66769=CARTESIAN_POINT('Ctrl Pts',(32.328721594765,505.483561202383,-36.9884932671904)) ;
#66770=CARTESIAN_POINT('Ctrl Pts',(31.235727331853,505.59479903315,-39.0523730713204)) ;
#66771=CARTESIAN_POINT('Ctrl Pts',(29.6903834469821,505.668962781963,-39.1870850142069)) ;
#66772=CARTESIAN_POINT('Ctrl Pts',(29.0613383924757,505.706052448823,-38.9116763785105)) ;
#66773=CARTESIAN_POINT('Ctrl Pts',(177.897717671888,503.713737563885,-36.4914564811708)) ;
#66774=CARTESIAN_POINT('Ctrl Pts',(178.074379770071,503.750828565321,-35.8286481930038)) ;
#66775=CARTESIAN_POINT('Ctrl Pts',(179.142242773597,503.82499364871,-34.7056767914726)) ;
#66776=CARTESIAN_POINT('Ctrl Pts',(181.434708312697,503.936232814051,-35.1374547995427)) ;
#66777=CARTESIAN_POINT('Ctrl Pts',(182.309156092825,504.047455059908,-37.3007467834596)) ;
#66778=CARTESIAN_POINT('Ctrl Pts',(180.9662761525,504.158677305767,-39.2071568534577)) ;
#66779=CARTESIAN_POINT('Ctrl Pts',(178.635481119123,504.269899551625,-39.111671513941)) ;
#66780=CARTESIAN_POINT('Ctrl Pts',(177.453501211943,504.381121797482,-37.1006641248506)) ;
#66781=CARTESIAN_POINT('Ctrl Pts',(178.503419192989,504.492344043339,-35.0178734541952)) ;
#66782=CARTESIAN_POINT('Ctrl Pts',(180.822967024381,504.603566289197,-34.7721178983205)) ;
#66783=CARTESIAN_POINT('Ctrl Pts',(182.286023668365,504.714788535052,-36.5887505440602)) ;
#66784=CARTESIAN_POINT('Ctrl Pts',(181.551584491592,504.82601078091,-38.8026295560003)) ;
#66785=CARTESIAN_POINT('Ctrl Pts',(179.292821524194,504.937233026769,-39.3845668730687)) ;
#66786=CARTESIAN_POINT('Ctrl Pts',(177.580062568716,505.048455272626,-37.8011699949904)) ;
#66787=CARTESIAN_POINT('Ctrl Pts',(177.983241051759,505.159677518484,-35.503748604351)) ;
#66788=CARTESIAN_POINT('Ctrl Pts',(180.132708648325,505.270899764341,-34.5981362170648)) ;
#66789=CARTESIAN_POINT('Ctrl Pts',(182.058536181622,505.382122010198,-35.9143487880221)) ;
#66790=CARTESIAN_POINT('Ctrl Pts',(181.995039985258,505.493344256054,-38.24623454224)) ;
#66791=CARTESIAN_POINT('Ctrl Pts',(180.001588542046,505.604566501912,-39.4561424861251)) ;
#66792=CARTESIAN_POINT('Ctrl Pts',(177.902882844478,505.71578874777,-38.43637509949)) ;
#66793=CARTESIAN_POINT('Ctrl Pts',(177.628263058505,505.82702530589,-36.1198778771031)) ;
#66794=CARTESIAN_POINT('Ctrl Pts',(178.821272510594,505.901187782059,-35.1310002461774)) ;
#66795=CARTESIAN_POINT('Ctrl Pts',(179.494516518593,505.938276176274,-34.9998530865222)) ;
#66796=CARTESIAN_POINT('Ctrl Pts',(178.025801529032,503.637205871377,-36.5256006623227)) ;
#66797=CARTESIAN_POINT('Ctrl Pts',(178.191097618669,503.674296872814,-35.9054358429339)) ;
#66798=CARTESIAN_POINT('Ctrl Pts',(179.190256920894,503.748461956203,-34.854713682631)) ;
#66799=CARTESIAN_POINT('Ctrl Pts',(181.335230818161,503.859701121544,-35.2587121466989)) ;
#66800=CARTESIAN_POINT('Ctrl Pts',(182.153418760753,503.970923367401,-37.2828232002907)) ;
#66801=CARTESIAN_POINT('Ctrl Pts',(180.896936440721,504.082145613258,-39.0665794958116)) ;
#66802=CARTESIAN_POINT('Ctrl Pts',(178.716099075358,504.193367859116,-38.9772374501662)) ;
#66803=CARTESIAN_POINT('Ctrl Pts',(177.610164872749,504.304590104974,-37.0956133719672)) ;
#66804=CARTESIAN_POINT('Ctrl Pts',(178.592533691474,504.415812350831,-35.1468243734714)) ;
#66805=CARTESIAN_POINT('Ctrl Pts',(180.762847472397,504.527034596688,-34.9168801307035)) ;
#66806=CARTESIAN_POINT('Ctrl Pts',(182.131774620067,504.638256842545,-36.6166350624903)) ;
#66807=CARTESIAN_POINT('Ctrl Pts',(181.444587468748,504.749479088403,-38.6880784980957)) ;
#66808=CARTESIAN_POINT('Ctrl Pts',(179.331147801914,504.86070133426,-39.2325753874353)) ;
#66809=CARTESIAN_POINT('Ctrl Pts',(177.72858358049,504.971923580118,-37.751050402843)) ;
#66810=CARTESIAN_POINT('Ctrl Pts',(178.105822543221,505.083145825975,-35.6014395014372)) ;
#66811=CARTESIAN_POINT('Ctrl Pts',(180.116998636827,505.194368071832,-34.7540920065066)) ;
#66812=CARTESIAN_POINT('Ctrl Pts',(181.918923123416,505.305590317689,-35.9856226706786)) ;
#66813=CARTESIAN_POINT('Ctrl Pts',(181.859512117469,505.416812563547,-38.1674805825633)) ;
#66814=CARTESIAN_POINT('Ctrl Pts',(179.994314478408,505.528034809404,-39.2995460001091)) ;
#66815=CARTESIAN_POINT('Ctrl Pts',(178.030634387015,505.639257055262,-38.3453879600819)) ;
#66816=CARTESIAN_POINT('Ctrl Pts',(177.773682968319,505.750493613383,-36.1779285194202)) ;
#66817=CARTESIAN_POINT('Ctrl Pts',(178.889937101816,505.82465608955,-35.2526728635555)) ;
#66818=CARTESIAN_POINT('Ctrl Pts',(179.519866232276,505.861744483766,-35.1299633923057)) ;
#66819=CARTESIAN_POINT('Ctrl Pts',(178.153885386176,503.56067417887,-36.5597448434743)) ;
#66820=CARTESIAN_POINT('Ctrl Pts',(178.307815467267,503.597765180306,-35.9822234928638)) ;
#66821=CARTESIAN_POINT('Ctrl Pts',(179.238271068191,503.671930263695,-35.0037505737895)) ;
#66822=CARTESIAN_POINT('Ctrl Pts',(181.235753323625,503.783169429037,-35.379969493855)) ;
#66823=CARTESIAN_POINT('Ctrl Pts',(181.997681428681,503.894391674893,-37.2648996171217)) ;
#66824=CARTESIAN_POINT('Ctrl Pts',(180.827596728942,504.005613920752,-38.9260021381655)) ;
#66825=CARTESIAN_POINT('Ctrl Pts',(178.796717031594,504.116836166609,-38.8428033863913)) ;
#66826=CARTESIAN_POINT('Ctrl Pts',(177.766828533554,504.228058412467,-37.0905626190838)) ;
#66827=CARTESIAN_POINT('Ctrl Pts',(178.68164818996,504.339280658324,-35.2757752927476)) ;
#66828=CARTESIAN_POINT('Ctrl Pts',(180.702727920414,504.450502904182,-35.0616423630866)) ;
#66829=CARTESIAN_POINT('Ctrl Pts',(181.977525571768,504.561725150037,-36.6445195809203)) ;
#66830=CARTESIAN_POINT('Ctrl Pts',(181.337590445906,504.672947395896,-38.5735274401913)) ;
#66831=CARTESIAN_POINT('Ctrl Pts',(179.369474079635,504.784169641753,-39.0805839018018)) ;
#66832=CARTESIAN_POINT('Ctrl Pts',(177.877104592264,504.895391887611,-37.7009308106956)) ;
#66833=CARTESIAN_POINT('Ctrl Pts',(178.228404034682,505.006614133468,-35.6991303985234)) ;
#66834=CARTESIAN_POINT('Ctrl Pts',(180.101288625331,505.117836379325,-34.9100477959482)) ;
#66835=CARTESIAN_POINT('Ctrl Pts',(181.779310065209,505.229058625183,-36.0568965533351)) ;
#66836=CARTESIAN_POINT('Ctrl Pts',(181.72398424968,505.340280871041,-38.0887266228865)) ;
#66837=CARTESIAN_POINT('Ctrl Pts',(179.987040414768,505.451503116897,-39.1429495140928)) ;
#66838=CARTESIAN_POINT('Ctrl Pts',(178.158385929553,505.562725362755,-38.2544008206738)) ;
#66839=CARTESIAN_POINT('Ctrl Pts',(177.919102878132,505.673961920876,-36.2359791617375)) ;
#66840=CARTESIAN_POINT('Ctrl Pts',(178.958601693041,505.748124397043,-35.3743454809335)) ;
#66841=CARTESIAN_POINT('Ctrl Pts',(179.545215945959,505.785212791258,-35.2600736980892)) ;
#66842=CARTESIAN_POINT('Ctrl Pts',(178.281969243322,503.484142486362,-36.5938890246262)) ;
#66843=CARTESIAN_POINT('Ctrl Pts',(178.424533315865,503.521233487799,-36.0590111427939)) ;
#66844=CARTESIAN_POINT('Ctrl Pts',(179.286285215488,503.595398571188,-35.152787464948)) ;
#66845=CARTESIAN_POINT('Ctrl Pts',(181.136275829091,503.706637736529,-35.5012268410111)) ;
#66846=CARTESIAN_POINT('Ctrl Pts',(181.84194409661,503.817859982386,-37.2469760339526)) ;
#66847=CARTESIAN_POINT('Ctrl Pts',(180.758257017163,503.929082228244,-38.7854247805194)) ;
#66848=CARTESIAN_POINT('Ctrl Pts',(178.87733498783,504.040304474101,-38.7083693226163)) ;
#66849=CARTESIAN_POINT('Ctrl Pts',(177.923492194359,504.151526719959,-37.0855118662004)) ;
#66850=CARTESIAN_POINT('Ctrl Pts',(178.770762688445,504.262748965816,-35.4047262120238)) ;
#66851=CARTESIAN_POINT('Ctrl Pts',(180.64260836843,504.373971211673,-35.2064045954696)) ;
#66852=CARTESIAN_POINT('Ctrl Pts',(181.823276523471,504.48519345753,-36.6724040993504)) ;
#66853=CARTESIAN_POINT('Ctrl Pts',(181.230593423062,504.596415703388,-38.4589763822867)) ;
#66854=CARTESIAN_POINT('Ctrl Pts',(179.407800357355,504.707637949245,-38.9285924161684)) ;
#66855=CARTESIAN_POINT('Ctrl Pts',(178.025625604036,504.818860195103,-37.6508112185482)) ;
#66856=CARTESIAN_POINT('Ctrl Pts',(178.350985526144,504.93008244096,-35.7968212956097)) ;
#66857=CARTESIAN_POINT('Ctrl Pts',(180.085578613834,505.041304686817,-35.0660035853901)) ;
#66858=CARTESIAN_POINT('Ctrl Pts',(181.639697007003,505.152526932675,-36.1281704359915)) ;
#66859=CARTESIAN_POINT('Ctrl Pts',(181.588456381889,505.263749178532,-38.0099726632097)) ;
#66860=CARTESIAN_POINT('Ctrl Pts',(179.979766351128,505.37497142439,-38.9863530280767)) ;
#66861=CARTESIAN_POINT('Ctrl Pts',(178.286137472091,505.486193670247,-38.1634136812656)) ;
#66862=CARTESIAN_POINT('Ctrl Pts',(178.064522787946,505.597430228368,-36.2940298040548)) ;
#66863=CARTESIAN_POINT('Ctrl Pts',(179.027266284264,505.671592704535,-35.4960180983116)) ;
#66864=CARTESIAN_POINT('Ctrl Pts',(179.570565659642,505.708681098751,-35.3901840038727)) ;
#66865=CARTESIAN_POINT('Ctrl Pts',(180.966211923875,503.712449228157,-38.2882733352088)) ;
#66866=CARTESIAN_POINT('Ctrl Pts',(180.544725879619,503.749537622418,-38.6470554114846)) ;
#66867=CARTESIAN_POINT('Ctrl Pts',(179.320554395332,503.82370009863,-38.9022063717596)) ;
#66868=CARTESIAN_POINT('Ctrl Pts',(177.997185744815,503.934936656795,-37.5633992739045)) ;
#66869=CARTESIAN_POINT('Ctrl Pts',(178.409746192673,504.046158902652,-35.7261726101518)) ;
#66870=CARTESIAN_POINT('Ctrl Pts',(180.176112949347,504.157381148509,-35.0772113129443)) ;
#66871=CARTESIAN_POINT('Ctrl Pts',(181.679313189748,504.268603394366,-36.2104342869482)) ;
#66872=CARTESIAN_POINT('Ctrl Pts',(181.540771709607,504.379825640224,-38.087743183612)) ;
#66873=CARTESIAN_POINT('Ctrl Pts',(179.88789431332,504.491047886081,-38.9882452844909)) ;
#66874=CARTESIAN_POINT('Ctrl Pts',(178.235528027901,504.602270131939,-38.0866781045897)) ;
#66875=CARTESIAN_POINT('Ctrl Pts',(178.098290323385,504.713492377796,-36.2093668187347)) ;
#66876=CARTESIAN_POINT('Ctrl Pts',(179.601943814894,504.824714623653,-35.0770506193662)) ;
#66877=CARTESIAN_POINT('Ctrl Pts',(181.36827414496,504.93593686951,-35.7275819122057)) ;
#66878=CARTESIAN_POINT('Ctrl Pts',(181.778304157799,505.047159115368,-37.5647011898004)) ;
#66879=CARTESIAN_POINT('Ctrl Pts',(180.456173380299,505.158381361225,-38.9045175683596)) ;
#66880=CARTESIAN_POINT('Ctrl Pts',(178.613817724806,505.269603607083,-38.5189875961006)) ;
#66881=CARTESIAN_POINT('Ctrl Pts',(177.939727930398,505.380825852941,-36.761408185579)) ;
#66882=CARTESIAN_POINT('Ctrl Pts',(179.052219255809,505.492048098798,-35.2428008227509)) ;
#66883=CARTESIAN_POINT('Ctrl Pts',(180.930694777575,505.603270344655,-35.3547472317361)) ;
#66884=CARTESIAN_POINT('Ctrl Pts',(181.855599490743,505.714492590512,-36.9949177133331)) ;
#66885=CARTESIAN_POINT('Ctrl Pts',(180.974577666776,505.825730800284,-38.6585326954567)) ;
#66886=CARTESIAN_POINT('Ctrl Pts',(179.728794440342,505.899894928103,-38.7672677976822)) ;
#66887=CARTESIAN_POINT('Ctrl Pts',(179.221729919173,505.936984973969,-38.5452579363092)) ;
#66888=CARTESIAN_POINT('Ctrl Pts',(181.052651241069,503.635454107785,-38.3898262273626)) ;
#66889=CARTESIAN_POINT('Ctrl Pts',(180.597358481875,503.672542502045,-38.7773856345679)) ;
#66890=CARTESIAN_POINT('Ctrl Pts',(179.274998179785,503.746704978258,-39.0530018413153)) ;
#66891=CARTESIAN_POINT('Ctrl Pts',(177.845484266961,503.857941536421,-37.6068111882233)) ;
#66892=CARTESIAN_POINT('Ctrl Pts',(178.291135522085,503.96916378228,-35.6222235407668)) ;
#66893=CARTESIAN_POINT('Ctrl Pts',(180.19917970375,504.080386028136,-34.9212101059385)) ;
#66894=CARTESIAN_POINT('Ctrl Pts',(181.822949207867,504.191608273994,-36.1453270646094)) ;
#66895=CARTESIAN_POINT('Ctrl Pts',(181.673295539339,504.302830519851,-38.1732118761487)) ;
#66896=CARTESIAN_POINT('Ctrl Pts',(179.887843516382,504.414052765709,-39.1459417962898)) ;
#66897=CARTESIAN_POINT('Ctrl Pts',(178.102943599667,504.525275011566,-38.172061368858)) ;
#66898=CARTESIAN_POINT('Ctrl Pts',(177.954698280501,504.636497257424,-36.1441739764944)) ;
#66899=CARTESIAN_POINT('Ctrl Pts',(179.578957390265,504.747719503281,-34.921036523388)) ;
#66900=CARTESIAN_POINT('Ctrl Pts',(181.486962223605,504.858941749138,-35.6237458806624)) ;
#66901=CARTESIAN_POINT('Ctrl Pts',(181.929880081602,504.970163994995,-37.6082175286907)) ;
#66902=CARTESIAN_POINT('Ctrl Pts',(180.501703329591,505.081386240852,-39.0554984152621)) ;
#66903=CARTESIAN_POINT('Ctrl Pts',(178.511575302249,505.192608486711,-38.6390457065327)) ;
#66904=CARTESIAN_POINT('Ctrl Pts',(177.783417854041,505.303830732568,-36.7404936898641)) ;
#66905=CARTESIAN_POINT('Ctrl Pts',(178.985140312065,505.415052978424,-35.1000812829108)) ;
#66906=CARTESIAN_POINT('Ctrl Pts',(181.014285321822,505.526275224282,-35.221006732575)) ;
#66907=CARTESIAN_POINT('Ctrl Pts',(182.013375148374,505.63749747014,-36.9927326397374)) ;
#66908=CARTESIAN_POINT('Ctrl Pts',(181.061687986699,505.74873567991,-38.7897834929524)) ;
#66909=CARTESIAN_POINT('Ctrl Pts',(179.715982499526,505.822899807729,-38.9072400621277)) ;
#66910=CARTESIAN_POINT('Ctrl Pts',(179.168247151989,505.859989853596,-38.6674231483047)) ;
#66911=CARTESIAN_POINT('Ctrl Pts',(181.139090558262,503.558458987411,-38.4913791195165)) ;
#66912=CARTESIAN_POINT('Ctrl Pts',(180.64999108413,503.595547381672,-38.9077158576513)) ;
#66913=CARTESIAN_POINT('Ctrl Pts',(179.229441964241,503.669709857884,-39.2037973108709)) ;
#66914=CARTESIAN_POINT('Ctrl Pts',(177.693782789108,503.780946416049,-37.6502231025421)) ;
#66915=CARTESIAN_POINT('Ctrl Pts',(178.172524851497,503.892168661906,-35.5182744713817)) ;
#66916=CARTESIAN_POINT('Ctrl Pts',(180.222246458154,504.003390907763,-34.7652088989327)) ;
#66917=CARTESIAN_POINT('Ctrl Pts',(181.966585225987,504.11461315362,-36.0802198422706)) ;
#66918=CARTESIAN_POINT('Ctrl Pts',(181.805819369072,504.225835399478,-38.2586805686856)) ;
#66919=CARTESIAN_POINT('Ctrl Pts',(179.887792719443,504.337057645335,-39.3036383080886)) ;
#66920=CARTESIAN_POINT('Ctrl Pts',(177.970359171432,504.448279891193,-38.2574446331264)) ;
#66921=CARTESIAN_POINT('Ctrl Pts',(177.811106237618,504.55950213705,-36.0789811342541)) ;
#66922=CARTESIAN_POINT('Ctrl Pts',(179.555970965639,504.670724382908,-34.7650224274098)) ;
#66923=CARTESIAN_POINT('Ctrl Pts',(181.605650302248,504.781946628764,-35.5199098491192)) ;
#66924=CARTESIAN_POINT('Ctrl Pts',(182.081456005406,504.893168874622,-37.6517338675809)) ;
#66925=CARTESIAN_POINT('Ctrl Pts',(180.547233278882,505.00439112048,-39.2064792621645)) ;
#66926=CARTESIAN_POINT('Ctrl Pts',(178.409332879691,505.115613366337,-38.7591038169648)) ;
#66927=CARTESIAN_POINT('Ctrl Pts',(177.627107777683,505.226835612195,-36.7195791941492)) ;
#66928=CARTESIAN_POINT('Ctrl Pts',(178.918061368321,505.338057858052,-34.9573617430708)) ;
#66929=CARTESIAN_POINT('Ctrl Pts',(181.097875866069,505.449280103909,-35.0872662334139)) ;
#66930=CARTESIAN_POINT('Ctrl Pts',(182.171150806007,505.560502349766,-36.9905475661418)) ;
#66931=CARTESIAN_POINT('Ctrl Pts',(181.14879830662,505.671740559538,-38.9210342904481)) ;
#66932=CARTESIAN_POINT('Ctrl Pts',(179.703170558711,505.745904687357,-39.0472123265731)) ;
#66933=CARTESIAN_POINT('Ctrl Pts',(179.114764384806,505.782994733223,-38.7895883603002)) ;
#66934=CARTESIAN_POINT('Ctrl Pts',(181.225529875457,503.481463867038,-38.5929320116703)) ;
#66935=CARTESIAN_POINT('Ctrl Pts',(180.702623686385,503.518552261299,-39.0380460807347)) ;
#66936=CARTESIAN_POINT('Ctrl Pts',(179.183885748694,503.592714737512,-39.3545927804265)) ;
#66937=CARTESIAN_POINT('Ctrl Pts',(177.542081311253,503.703951295676,-37.6936350168609)) ;
#66938=CARTESIAN_POINT('Ctrl Pts',(178.053914180908,503.815173541534,-35.4143254019966)) ;
#66939=CARTESIAN_POINT('Ctrl Pts',(180.245313212556,503.926395787391,-34.6092076919268)) ;
#66940=CARTESIAN_POINT('Ctrl Pts',(182.110221244107,504.037618033248,-36.0151126199319)) ;
#66941=CARTESIAN_POINT('Ctrl Pts',(181.938343198804,504.148840279104,-38.3441492612223)) ;
#66942=CARTESIAN_POINT('Ctrl Pts',(179.887741922503,504.260062524963,-39.4613348198873)) ;
#66943=CARTESIAN_POINT('Ctrl Pts',(177.837774743198,504.371284770819,-38.3428278973948)) ;
#66944=CARTESIAN_POINT('Ctrl Pts',(177.667514194734,504.482507016678,-36.0137882920138)) ;
#66945=CARTESIAN_POINT('Ctrl Pts',(179.53298454101,504.593729262535,-34.6090083314316)) ;
#66946=CARTESIAN_POINT('Ctrl Pts',(181.724338380893,504.704951508392,-35.4160738175759)) ;
#66947=CARTESIAN_POINT('Ctrl Pts',(182.233031929209,504.816173754249,-37.6952502064713)) ;
#66948=CARTESIAN_POINT('Ctrl Pts',(180.592763228173,504.927396000106,-39.357460109067)) ;
#66949=CARTESIAN_POINT('Ctrl Pts',(178.307090457134,505.038618245965,-38.879161927397)) ;
#66950=CARTESIAN_POINT('Ctrl Pts',(177.470797701326,505.149840491822,-36.6986646984343)) ;
#66951=CARTESIAN_POINT('Ctrl Pts',(178.850982424577,505.261062737679,-34.8146422032309)) ;
#66952=CARTESIAN_POINT('Ctrl Pts',(181.181466410316,505.372284983536,-34.9535257342527)) ;
#66953=CARTESIAN_POINT('Ctrl Pts',(182.328926463639,505.483507229393,-36.9883624925461)) ;
#66954=CARTESIAN_POINT('Ctrl Pts',(181.235908626542,505.594745439164,-39.0522850879437)) ;
#66955=CARTESIAN_POINT('Ctrl Pts',(179.690358617895,505.668909566983,-39.1871845910186)) ;
#66956=CARTESIAN_POINT('Ctrl Pts',(179.061281617622,505.70599961285,-38.9117535722958)) ;
#66957=CARTESIAN_POINT('Origin',(87.3885276254222,618.710565160552,-31.0221601717549)) ;
#66958=CARTESIAN_POINT('',(87.2635276254222,618.585565160552,-31.0221601717549)) ;
#66959=CARTESIAN_POINT('',(87.2635276254222,618.710565160552,-31.0221601717549)) ;
#66960=CARTESIAN_POINT('',(73.5135276254222,618.585565160554,-31.0221601717549)) ;
#66961=CARTESIAN_POINT('',(73.5135276254222,618.710565160554,-31.0221601717549)) ;
#66962=CARTESIAN_POINT('',(149.888527625422,618.585565160541,-31.0221601717549)) ;
#66963=CARTESIAN_POINT('Origin',(73.3885276254222,618.710565160554,-31.0221601717549)) ;
#66964=CARTESIAN_POINT('',(73.3885276254222,618.585565160554,-31.1471601717549)) ;
#66965=CARTESIAN_POINT('',(73.3885276254222,618.710565160554,-31.1471601717549)) ;
#66966=CARTESIAN_POINT('',(73.3885276254222,618.585565160554,-39.8971601717549)) ;
#66967=CARTESIAN_POINT('',(73.3885276254222,618.710565160554,-39.8971601717549)) ;
#66968=CARTESIAN_POINT('',(73.3885276254222,618.585565160554,-40.272160171758)) ;
#66969=CARTESIAN_POINT('Origin',(73.3885276254222,618.710565160554,-40.0221601717549)) ;
#66970=CARTESIAN_POINT('',(87.2635276254222,618.585565160552,-40.0221601717549)) ;
#66971=CARTESIAN_POINT('',(87.2635276254222,618.710565160552,-40.0221601717549)) ;
#66972=CARTESIAN_POINT('',(73.5135276254222,618.585565160554,-40.0221601717549)) ;
#66973=CARTESIAN_POINT('',(142.888527625422,618.585565160542,-40.0221601717549)) ;
#66974=CARTESIAN_POINT('',(73.5135276254222,618.710565160554,-40.0221601717549)) ;
#66975=CARTESIAN_POINT('Origin',(87.3885276254222,618.710565160552,-40.0221601717549)) ;
#66976=CARTESIAN_POINT('',(87.3885276254222,618.585565160552,-31.1471601717549)) ;
#66977=CARTESIAN_POINT('',(87.3885276254222,618.710565160552,-31.1471601717549)) ;
#66978=CARTESIAN_POINT('',(87.3885276254222,618.585565160552,-39.8971601717549)) ;
#66979=CARTESIAN_POINT('',(87.3885276254222,618.585565160552,-44.772160171758)) ;
#66980=CARTESIAN_POINT('',(87.3885276254222,618.710565160552,-39.8971601717549)) ;
#66981=CARTESIAN_POINT('Origin',(73.5135276254222,618.710565160554,-39.8971601717549)) ;
#66982=CARTESIAN_POINT('Origin',(73.5135276254222,618.585565160554,-39.8971601717549)) ;
#66983=CARTESIAN_POINT('Origin',(87.2635276254222,618.710565160552,-39.8971601717549)) ;
#66984=CARTESIAN_POINT('Origin',(87.2635276254222,618.585565160552,-39.8971601717549)) ;
#66985=CARTESIAN_POINT('Origin',(142.888527625422,618.585565160542,-40.1471601717549)) ;
#66986=CARTESIAN_POINT('Origin',(87.2635276254222,618.585565160552,-40.1471601717549)) ;
#66987=CARTESIAN_POINT('Origin',(73.5135276254222,618.585565160554,-40.1471601717549)) ;
#66988=CARTESIAN_POINT('Origin',(73.5135276254222,618.710565160554,-31.1471601717549)) ;
#66989=CARTESIAN_POINT('Origin',(73.5135276254222,618.585565160554,-31.1471601717549)) ;
#66990=CARTESIAN_POINT('Origin',(149.888527625422,618.585565160541,-30.8971601717549)) ;
#66991=CARTESIAN_POINT('Origin',(73.5135276254222,618.585565160554,-30.8971601717549)) ;
#66992=CARTESIAN_POINT('Origin',(87.2635276254222,618.585565160552,-30.8971601717549)) ;
#66993=CARTESIAN_POINT('Origin',(87.2635276254222,618.710565160552,-31.1471601717549)) ;
#66994=CARTESIAN_POINT('Origin',(87.2635276254222,618.585565160552,-31.1471601717549)) ;
#66995=CARTESIAN_POINT('Origin',(87.5135276254222,618.585565160552,-44.772160171758)) ;
#66996=CARTESIAN_POINT('Origin',(87.5135276254222,618.585565160552,-31.1471601717549)) ;
#66997=CARTESIAN_POINT('Origin',(87.5135276254222,618.585565160552,-39.8971601717549)) ;
#66998=CARTESIAN_POINT('Origin',(87.2635276254222,618.585565160552,-31.1471601717549)) ;
#66999=CARTESIAN_POINT('Origin',(73.2635276254222,618.585565160554,-40.272160171758)) ;
#67000=CARTESIAN_POINT('Origin',(73.2635276254222,618.585565160554,-39.8971601717549)) ;
#67001=CARTESIAN_POINT('Origin',(73.2635276254222,618.585565160554,-31.1471601717549)) ;
#67002=CARTESIAN_POINT('Origin',(73.5135276254222,618.585565160554,-31.1471601717549)) ;
#67003=CARTESIAN_POINT('Origin',(87.2635276254222,618.585565160552,-39.8971601717549)) ;
#67004=CARTESIAN_POINT('Origin',(73.5135276254222,618.585565160554,-39.8971601717549)) ;
#67005=CARTESIAN_POINT('Origin',(95.6885276254225,618.21056516055,-24.1221601717559)) ;
#67006=CARTESIAN_POINT('',(97.6885276254217,613.46056516055,-24.122160171756)) ;
#67007=CARTESIAN_POINT('Origin',(97.688527625422,615.46056516055,-24.122160171756)) ;
#67008=CARTESIAN_POINT('',(124.688527625422,613.460565160546,-24.1221601717572)) ;
#67009=CARTESIAN_POINT('',(154.038527625422,613.46056516054,-24.1221601717586)) ;
#67010=CARTESIAN_POINT('Origin',(124.688527625422,615.460565160545,-24.1221601717572)) ;
#67011=CARTESIAN_POINT('Origin',(173.388527625422,618.210565160537,-37.2221601717594)) ;
#67012=CARTESIAN_POINT('Origin',(171.388527625402,506.960565160537,-37.2221601717594)) ;
#67013=CARTESIAN_POINT('Origin',(171.388527625402,506.960565160537,-45.8221601717594)) ;
#67014=CARTESIAN_POINT('',(171.388527625403,508.960565160537,-38.1221601717594)) ;
#67015=CARTESIAN_POINT('Origin',(171.388527625402,506.960565160537,-38.1221601717594)) ;
#67016=CARTESIAN_POINT('',(171.388527625402,508.960565160537,-45.8221601717594)) ;
#67017=CARTESIAN_POINT('Origin',(171.388527625422,618.210565160537,-30.2221601717593)) ;
#67018=CARTESIAN_POINT('Origin',(171.388527625403,506.960565160537,-30.2221601717594)) ;
#67019=CARTESIAN_POINT('Origin',(171.388527625402,506.960565160537,-45.8221601717594)) ;
#67020=CARTESIAN_POINT('',(171.388527625402,508.960565160537,-45.8221601717594)) ;
#67021=CARTESIAN_POINT('Origin',(124.688527625421,615.460565160545,-36.8221601717572)) ;
#67022=CARTESIAN_POINT('',(124.688527625421,613.460565160545,-38.1221601717572)) ;
#67023=CARTESIAN_POINT('Origin',(124.688527625421,615.460565160545,-38.1221601717572)) ;
#67024=CARTESIAN_POINT('',(124.688527625421,613.460565160545,-36.8221601717572)) ;
#67025=CARTESIAN_POINT('Origin',(87.9885276254024,506.960565160552,-36.8221601717556)) ;
#67026=CARTESIAN_POINT('',(87.9885276254026,508.960565160552,-38.1221601717555)) ;
#67027=CARTESIAN_POINT('Origin',(87.9885276254023,506.960565160552,-38.1221601717555)) ;
#67028=CARTESIAN_POINT('',(87.9885276254027,508.960565160552,-36.8221601717556)) ;
#67029=CARTESIAN_POINT('Origin',(212.388527625402,508.96056516053,-49.5221601717612)) ;
#67030=CARTESIAN_POINT('',(169.388527625402,508.960565160538,-40.1221604692946)) ;
#67031=CARTESIAN_POINT('Origin',(169.388527625403,508.960565160538,-38.1221601717593)) ;
#67032=CARTESIAN_POINT('',(89.9885276254026,508.960565160552,-40.1221604695632)) ;
#67033=CARTESIAN_POINT('',(158.688527625403,508.96056516054,-40.1221607671016)) ;
#67034=CARTESIAN_POINT('Origin',(89.9885276254027,508.960565160552,-38.1221601717556)) ;
#67035=CARTESIAN_POINT('Ctrl Pts',(87.9885276254048,508.960565160552,-38.122160171761)) ;
#67036=CARTESIAN_POINT('Ctrl Pts',(87.9885276253991,508.960565160552,-40.1221601717586)) ;
#67037=CARTESIAN_POINT('Ctrl Pts',(89.9885276253967,508.960565160552,-40.1221601717529)) ;
#67038=CARTESIAN_POINT('Ctrl Pts',(85.9885276254019,508.960565160554,-38.122160171761)) ;
#67039=CARTESIAN_POINT('Ctrl Pts',(85.9885276253905,508.960565160553,-42.1221601717673)) ;
#67040=CARTESIAN_POINT('Ctrl Pts',(89.9885276253967,508.960565160554,-42.1221601717558)) ;
#67041=CARTESIAN_POINT('Ctrl Pts',(85.9885276254023,506.960565160551,-38.1221601717605)) ;
#67042=CARTESIAN_POINT('Ctrl Pts',(85.9885276253908,506.96056516055,-42.1221601717667)) ;
#67043=CARTESIAN_POINT('Ctrl Pts',(89.988527625397,506.960565160551,-42.1221601717552)) ;
#67044=CARTESIAN_POINT('Origin',(89.9885276254022,506.960565160552,-40.1221607670984)) ;
#67045=CARTESIAN_POINT('Origin',(158.688527625402,506.960565160539,-40.1221607671016)) ;
#67046=CARTESIAN_POINT('Origin',(169.388527625402,506.960565160538,-40.1221601717593)) ;
#67047=CARTESIAN_POINT('Ctrl Pts',(173.388527625402,506.960565160537,-38.1221601717599)) ;
#67048=CARTESIAN_POINT('Ctrl Pts',(173.388527625405,506.960565160535,-42.1221601717625)) ;
#67049=CARTESIAN_POINT('Ctrl Pts',(169.388527625403,506.960565160538,-42.1221601717592)) ;
#67050=CARTESIAN_POINT('Ctrl Pts',(173.388527625403,508.960565160538,-38.1221601717607)) ;
#67051=CARTESIAN_POINT('Ctrl Pts',(173.388527625407,508.960565160536,-42.1221601717633)) ;
#67052=CARTESIAN_POINT('Ctrl Pts',(169.388527625404,508.960565160539,-42.12216017176)) ;
#67053=CARTESIAN_POINT('Ctrl Pts',(171.388527625402,508.960565160537,-38.1221601717607)) ;
#67054=CARTESIAN_POINT('Ctrl Pts',(171.388527625404,508.960565160537,-40.1221601717605)) ;
#67055=CARTESIAN_POINT('Ctrl Pts',(169.388527625404,508.960565160538,-40.1221601717589)) ;
#67056=CARTESIAN_POINT('Origin',(212.38852762542,613.46056516053,-49.5221601717612)) ;
#67057=CARTESIAN_POINT('',(122.688527625421,613.460565160546,-40.1221604695633)) ;
#67058=CARTESIAN_POINT('Origin',(122.688527625421,613.460565160546,-38.1221601717571)) ;
#67059=CARTESIAN_POINT('',(97.688527625421,613.46056516055,-38.122160171756)) ;
#67060=CARTESIAN_POINT('',(97.6885276254207,613.46056516055,-45.822160171756)) ;
#67061=CARTESIAN_POINT('',(99.6885276254209,613.46056516055,-40.12216046929)) ;
#67062=CARTESIAN_POINT('Origin',(99.688527625421,613.46056516055,-38.1221601717561)) ;
#67063=CARTESIAN_POINT('',(158.688527625421,613.46056516054,-40.1221607670988)) ;
#67064=CARTESIAN_POINT('Origin',(97.688527625421,615.46056516055,-45.822160171756)) ;
#67065=CARTESIAN_POINT('Origin',(97.6885276254213,615.46056516055,-38.122160171756)) ;
#67066=CARTESIAN_POINT('Ctrl Pts',(122.688527625423,615.460565160547,-42.1221601717572)) ;
#67067=CARTESIAN_POINT('Ctrl Pts',(126.688527625424,615.460565160546,-42.1221601717601)) ;
#67068=CARTESIAN_POINT('Ctrl Pts',(126.688527625421,615.460565160545,-38.1221601717583)) ;
#67069=CARTESIAN_POINT('Ctrl Pts',(122.688527625422,613.460565160545,-42.1221601717582)) ;
#67070=CARTESIAN_POINT('Ctrl Pts',(126.688527625425,613.460565160545,-42.1221601717611)) ;
#67071=CARTESIAN_POINT('Ctrl Pts',(126.688527625422,613.460565160544,-38.1221601717587)) ;
#67072=CARTESIAN_POINT('Ctrl Pts',(122.688527625422,613.460565160546,-40.1221601717567)) ;
#67073=CARTESIAN_POINT('Ctrl Pts',(124.688527625422,613.460565160546,-40.1221601717582)) ;
#67074=CARTESIAN_POINT('Ctrl Pts',(124.68852762542,613.460565160545,-38.1221601717587)) ;
#67075=CARTESIAN_POINT('Origin',(122.688527625421,615.460565160546,-40.1221607670971)) ;
#67076=CARTESIAN_POINT('Origin',(158.688527625421,615.460565160539,-40.1221607670988)) ;
#67077=CARTESIAN_POINT('Origin',(99.6885276254213,615.46056516055,-40.1221601717561)) ;
#67078=CARTESIAN_POINT('Ctrl Pts',(99.6885276254238,613.46056516055,-40.1221601717561)) ;
#67079=CARTESIAN_POINT('Ctrl Pts',(97.6885276254219,613.46056516055,-40.1221601717552)) ;
#67080=CARTESIAN_POINT('Ctrl Pts',(97.688527625421,613.46056516055,-38.1221601717534)) ;
#67081=CARTESIAN_POINT('Ctrl Pts',(99.6885276254238,613.46056516055,-42.122160171757)) ;
#67082=CARTESIAN_POINT('Ctrl Pts',(95.688527625422,613.460565160549,-42.1221601717552)) ;
#67083=CARTESIAN_POINT('Ctrl Pts',(95.6885276254202,613.46056516055,-38.1221601717534)) ;
#67084=CARTESIAN_POINT('Ctrl Pts',(99.6885276254231,615.460565160551,-42.1221601717564)) ;
#67085=CARTESIAN_POINT('Ctrl Pts',(95.6885276254227,615.46056516055,-42.1221601717546)) ;
#67086=CARTESIAN_POINT('Ctrl Pts',(95.6885276254209,615.460565160551,-38.1221601717541)) ;
#67087=CARTESIAN_POINT('Ctrl Pts',(180.41923219887,533.719746184936,-49.5189826834674)) ;
#67088=CARTESIAN_POINT('Ctrl Pts',(181.08204398532,533.89640864105,-49.4818916555201)) ;
#67089=CARTESIAN_POINT('Ctrl Pts',(182.205016276376,534.964329959553,-49.4077265456203)) ;
#67090=CARTESIAN_POINT('Ctrl Pts',(181.773238631581,537.25679369829,-49.296487353768)) ;
#67091=CARTESIAN_POINT('Ctrl Pts',(179.609931126086,538.131245101682,-49.1852651079104)) ;
#67092=CARTESIAN_POINT('Ctrl Pts',(177.703506856333,536.788339278838,-49.0740428620531)) ;
#67093=CARTESIAN_POINT('Ctrl Pts',(177.798995298387,534.457518489788,-48.9628206161957)) ;
#67094=CARTESIAN_POINT('Ctrl Pts',(179.810021293082,533.275522950702,-48.8515983703383)) ;
#67095=CARTESIAN_POINT('Ctrl Pts',(181.892831047736,534.325447947475,-48.7403761244811)) ;
#67096=CARTESIAN_POINT('Ctrl Pts',(182.138589015903,536.645014490742,-48.6291538786237)) ;
#67097=CARTESIAN_POINT('Ctrl Pts',(180.32194054985,538.108083264837,-48.5179316327663)) ;
#67098=CARTESIAN_POINT('Ctrl Pts',(178.1080419789,537.373637216578,-48.4067093869088)) ;
#67099=CARTESIAN_POINT('Ctrl Pts',(177.526099138551,535.114854267548,-48.2954871410515)) ;
#67100=CARTESIAN_POINT('Ctrl Pts',(179.109509196157,533.402080354734,-48.1842648951941)) ;
#67101=CARTESIAN_POINT('Ctrl Pts',(181.406949090904,533.805262519012,-48.0730426493369)) ;
#67102=CARTESIAN_POINT('Ctrl Pts',(182.31256717773,535.954749633126,-47.9618204034795)) ;
#67103=CARTESIAN_POINT('Ctrl Pts',(180.996337743865,537.880594664061,-47.850598157622)) ;
#67104=CARTESIAN_POINT('Ctrl Pts',(178.664426082464,537.817099808701,-47.7393759117645)) ;
#67105=CARTESIAN_POINT('Ctrl Pts',(177.454493283379,535.82363243575,-47.6281536659072)) ;
#67106=CARTESIAN_POINT('Ctrl Pts',(178.474265342102,533.724911499449,-47.5169314200499)) ;
#67107=CARTESIAN_POINT('Ctrl Pts',(180.790760669799,533.450291962028,-47.4056948389639)) ;
#67108=CARTESIAN_POINT('Ctrl Pts',(181.779696394841,534.643306150536,-47.3315323398303)) ;
#67109=CARTESIAN_POINT('Ctrl Pts',(181.910843734302,535.316553593751,-47.2944439226492)) ;
#67110=CARTESIAN_POINT('Ctrl Pts',(180.385086881284,533.847834672537,-49.5955171281681)) ;
#67111=CARTESIAN_POINT('Ctrl Pts',(181.005253625502,534.013130737684,-49.5584261002209)) ;
#67112=CARTESIAN_POINT('Ctrl Pts',(182.055974333595,535.012342430532,-49.484260990321)) ;
#67113=CARTESIAN_POINT('Ctrl Pts',(181.651977087812,537.157309979624,-49.3730217984687)) ;
#67114=CARTESIAN_POINT('Ctrl Pts',(179.62785591216,537.975499533435,-49.2617995526112)) ;
#67115=CARTESIAN_POINT('Ctrl Pts',(177.844090208774,536.718995728027,-49.1505773067538)) ;
#67116=CARTESIAN_POINT('Ctrl Pts',(177.933434963089,534.538139005725,-49.0393550608965)) ;
#67117=CARTESIAN_POINT('Ctrl Pts',(179.815072358748,533.432192581505,-48.9281328150392)) ;
#67118=CARTESIAN_POINT('Ctrl Pts',(181.763874976287,534.414565828681,-48.8169105691819)) ;
#67119=CARTESIAN_POINT('Ctrl Pts',(181.99382097619,536.584892398823,-48.7056883233245)) ;
#67120=CARTESIAN_POINT('Ctrl Pts',(180.294054937609,537.953827919806,-48.594466077467)) ;
#67121=CARTESIAN_POINT('Ctrl Pts',(178.222597705189,537.266635833207,-48.4832438316095)) ;
#67122=CARTESIAN_POINT('Ctrl Pts',(177.67809683179,535.153182065438,-48.3720215857521)) ;
#67123=CARTESIAN_POINT('Ctrl Pts',(179.159630926782,533.550607333357,-48.2607993398948)) ;
#67124=CARTESIAN_POINT('Ctrl Pts',(181.309254468017,533.927848920271,-48.1495770940376)) ;
#67125=CARTESIAN_POINT('Ctrl Pts',(182.15660545346,535.939038902933,-48.0383548481802)) ;
#67126=CARTESIAN_POINT('Ctrl Pts',(180.925061688953,537.740975843584,-47.9271326023229)) ;
#67127=CARTESIAN_POINT('Ctrl Pts',(178.743184280586,537.681566221535,-47.8159103564653)) ;
#67128=CARTESIAN_POINT('Ctrl Pts',(177.611098068376,535.816357732999,-47.704688110608)) ;
#67129=CARTESIAN_POINT('Ctrl Pts',(178.565258405338,533.852667652805,-47.5934658647506)) ;
#67130=CARTESIAN_POINT('Ctrl Pts',(180.732711360678,533.595717025337,-47.4822292836646)) ;
#67131=CARTESIAN_POINT('Ctrl Pts',(181.658019361195,534.711973163531,-47.4080667845311)) ;
#67132=CARTESIAN_POINT('Ctrl Pts',(181.780728733884,535.34190413858,-47.37097836735)) ;
#67133=CARTESIAN_POINT('Ctrl Pts',(180.350941563697,533.975923160139,-49.6720515728689)) ;
#67134=CARTESIAN_POINT('Ctrl Pts',(180.928463265684,534.129852834319,-49.6349605449215)) ;
#67135=CARTESIAN_POINT('Ctrl Pts',(181.906932390813,535.06035490151,-49.5607954350218)) ;
#67136=CARTESIAN_POINT('Ctrl Pts',(181.530715544042,537.057826260956,-49.4495562431695)) ;
#67137=CARTESIAN_POINT('Ctrl Pts',(179.645780698234,537.81975396519,-49.338333997312)) ;
#67138=CARTESIAN_POINT('Ctrl Pts',(177.984673561212,536.649652177216,-49.2271117514546)) ;
#67139=CARTESIAN_POINT('Ctrl Pts',(178.067874627792,534.618759521662,-49.1158895055972)) ;
#67140=CARTESIAN_POINT('Ctrl Pts',(179.820123424414,533.58886221231,-49.0046672597399)) ;
#67141=CARTESIAN_POINT('Ctrl Pts',(181.634918904837,534.503683709888,-48.8934450138826)) ;
#67142=CARTESIAN_POINT('Ctrl Pts',(181.849052936478,536.524770306902,-48.7822227680253)) ;
#67143=CARTESIAN_POINT('Ctrl Pts',(180.266169325365,537.799572574774,-48.6710005221678)) ;
#67144=CARTESIAN_POINT('Ctrl Pts',(178.337153431476,537.159634449835,-48.5597782763103)) ;
#67145=CARTESIAN_POINT('Ctrl Pts',(177.83009452503,535.191509863326,-48.4485560304529)) ;
#67146=CARTESIAN_POINT('Ctrl Pts',(179.209752657406,533.699134311977,-48.3373337845956)) ;
#67147=CARTESIAN_POINT('Ctrl Pts',(181.21155984513,534.05043532153,-48.2261115387384)) ;
#67148=CARTESIAN_POINT('Ctrl Pts',(182.000643729191,535.923328172739,-48.114889292881)) ;
#67149=CARTESIAN_POINT('Ctrl Pts',(180.853785634043,537.601357023106,-48.0036670470236)) ;
#67150=CARTESIAN_POINT('Ctrl Pts',(178.821942478709,537.546032634367,-47.8924448011661)) ;
#67151=CARTESIAN_POINT('Ctrl Pts',(177.767702853372,535.809083030247,-47.7812225553087)) ;
#67152=CARTESIAN_POINT('Ctrl Pts',(178.656251468576,533.980423806161,-47.6700003094514)) ;
#67153=CARTESIAN_POINT('Ctrl Pts',(180.674662051555,533.741142088646,-47.5587637283654)) ;
#67154=CARTESIAN_POINT('Ctrl Pts',(181.53634232755,534.780640176528,-47.4846012292319)) ;
#67155=CARTESIAN_POINT('Ctrl Pts',(181.650613733467,535.367254683408,-47.4475128120508)) ;
#67156=CARTESIAN_POINT('Ctrl Pts',(180.316796246111,534.104011647741,-49.7485860175697)) ;
#67157=CARTESIAN_POINT('Ctrl Pts',(180.851672905866,534.246574930955,-49.7114949896223)) ;
#67158=CARTESIAN_POINT('Ctrl Pts',(181.757890448032,535.108367372488,-49.6373298797226)) ;
#67159=CARTESIAN_POINT('Ctrl Pts',(181.409454000273,536.958342542287,-49.5260906878703)) ;
#67160=CARTESIAN_POINT('Ctrl Pts',(179.663705484307,537.664008396944,-49.4148684420128)) ;
#67161=CARTESIAN_POINT('Ctrl Pts',(178.125256913651,536.580308626405,-49.3036461961554)) ;
#67162=CARTESIAN_POINT('Ctrl Pts',(178.202314292494,534.699380037599,-49.192423950298)) ;
#67163=CARTESIAN_POINT('Ctrl Pts',(179.825174490079,533.745531843113,-49.0812017044407)) ;
#67164=CARTESIAN_POINT('Ctrl Pts',(181.505962833386,534.592801591096,-48.9699794585834)) ;
#67165=CARTESIAN_POINT('Ctrl Pts',(181.704284896765,536.464648214983,-48.858757212726)) ;
#67166=CARTESIAN_POINT('Ctrl Pts',(180.238283713123,537.645317229742,-48.7475349668686)) ;
#67167=CARTESIAN_POINT('Ctrl Pts',(178.451709157764,537.052633066464,-48.6363127210111)) ;
#67168=CARTESIAN_POINT('Ctrl Pts',(177.982092218269,535.229837661215,-48.5250904751537)) ;
#67169=CARTESIAN_POINT('Ctrl Pts',(179.25987438803,533.847661290597,-48.4138682292964)) ;
#67170=CARTESIAN_POINT('Ctrl Pts',(181.113865222243,534.173021722788,-48.3026459834391)) ;
#67171=CARTESIAN_POINT('Ctrl Pts',(181.844682004921,535.907617442545,-48.1914237375818)) ;
#67172=CARTESIAN_POINT('Ctrl Pts',(180.782509579131,537.461738202629,-48.0802014917245)) ;
#67173=CARTESIAN_POINT('Ctrl Pts',(178.900700676832,537.410499047199,-47.9689792458669)) ;
#67174=CARTESIAN_POINT('Ctrl Pts',(177.924307638369,535.801808327496,-47.8577570000095)) ;
#67175=CARTESIAN_POINT('Ctrl Pts',(178.747244531814,534.108179959515,-47.7465347541522)) ;
#67176=CARTESIAN_POINT('Ctrl Pts',(180.616612742433,533.886567151955,-47.6352981730662)) ;
#67177=CARTESIAN_POINT('Ctrl Pts',(181.414665293904,534.849307189524,-47.5611356739326)) ;
#67178=CARTESIAN_POINT('Ctrl Pts',(181.52049873305,535.392605228237,-47.5240472567515)) ;
#67179=CARTESIAN_POINT('Ctrl Pts',(181.523656952658,535.391334705907,-47.5221601717598)) ;
#67180=CARTESIAN_POINT('Ctrl Pts',(181.518699643216,535.327493994687,-47.5221601717599)) ;
#67181=CARTESIAN_POINT('Ctrl Pts',(181.509766310845,535.264222574159,-47.5221601717597)) ;
#67182=CARTESIAN_POINT('Ctrl Pts',(181.497157990989,535.201755695665,-47.5221601717597)) ;
#67183=CARTESIAN_POINT('Ctrl Pts',(181.484549671134,535.139288817172,-47.5221601717597)) ;
#67184=CARTESIAN_POINT('Ctrl Pts',(181.468266021405,535.077625700605,-47.5221601717599)) ;
#67185=CARTESIAN_POINT('Ctrl Pts',(181.448552578097,535.016991237747,-47.5221601717599)) ;
#67186=CARTESIAN_POINT('Ctrl Pts',(181.430731424601,534.962177065872,-47.5221601717599)) ;
#67187=CARTESIAN_POINT('Ctrl Pts',(181.410106447755,534.908202995365,-47.5221601717595)) ;
#67188=CARTESIAN_POINT('Ctrl Pts',(181.386823585982,534.855235972333,-47.5221601717596)) ;
#67189=CARTESIAN_POINT('Ctrl Pts',(181.375123803509,534.828619714685,-47.5221601717596)) ;
#67190=CARTESIAN_POINT('Ctrl Pts',(181.362752363877,534.802257809648,-47.5221601717599)) ;
#67191=CARTESIAN_POINT('Ctrl Pts',(181.349724849682,534.776172131308,-47.52216017176)) ;
#67192=CARTESIAN_POINT('Ctrl Pts',(181.343830429245,534.764369422577,-47.52216017176)) ;
#67193=CARTESIAN_POINT('Ctrl Pts',(181.337800833022,534.752621939525,-47.5221601717597)) ;
#67194=CARTESIAN_POINT('Ctrl Pts',(181.33164761352,534.74095038958,-47.5221601717597)) ;
#67195=CARTESIAN_POINT('Ctrl Pts',(181.300422339755,534.681721665141,-47.5221601717597)) ;
#67196=CARTESIAN_POINT('Ctrl Pts',(181.265964241246,534.624338180145,-47.5221601717599)) ;
#67197=CARTESIAN_POINT('Ctrl Pts',(181.228541247385,534.569040430327,-47.5221601717598)) ;
#67198=CARTESIAN_POINT('Ctrl Pts',(181.190437292971,534.51273646528,-47.5221601717597)) ;
#67199=CARTESIAN_POINT('Ctrl Pts',(181.149259248045,534.45859387379,-47.5221601717597)) ;
#67200=CARTESIAN_POINT('Ctrl Pts',(181.105236814465,534.406874481233,-47.5221601717596)) ;
#67201=CARTESIAN_POINT('Ctrl Pts',(181.068311305258,534.36349285167,-47.5221601717596)) ;
#67202=CARTESIAN_POINT('Ctrl Pts',(181.029383499007,534.321815942503,-47.5221601717598)) ;
#67203=CARTESIAN_POINT('Ctrl Pts',(180.988563640333,534.282010110072,-47.5221601717598)) ;
#67204=CARTESIAN_POINT('Ctrl Pts',(180.969705409454,534.263620345808,-47.5221601717598)) ;
#67205=CARTESIAN_POINT('Ctrl Pts',(180.950443053091,534.245630122635,-47.5221601717599)) ;
#67206=CARTESIAN_POINT('Ctrl Pts',(180.93078597856,534.228057025436,-47.5221601717598)) ;
#67207=CARTESIAN_POINT('Ctrl Pts',(180.92231760162,534.220486437511,-47.5221601717597)) ;
#67208=CARTESIAN_POINT('Ctrl Pts',(180.913776338193,534.212993731098,-47.5221601717599)) ;
#67209=CARTESIAN_POINT('Ctrl Pts',(180.905173315045,534.20558895583,-47.5221601717599)) ;
#67210=CARTESIAN_POINT('Ctrl Pts',(180.85193819082,534.159768536138,-47.5221601717599)) ;
#67211=CARTESIAN_POINT('Ctrl Pts',(180.796243425943,534.11722427461,-47.5221601717599)) ;
#67212=CARTESIAN_POINT('Ctrl Pts',(180.738340695584,534.078223544828,-47.5221601717599)) ;
#67213=CARTESIAN_POINT('Ctrl Pts',(180.686274773575,534.043154232163,-47.5221601717599)) ;
#67214=CARTESIAN_POINT('Ctrl Pts',(180.632422628309,534.010949703227,-47.5221601717598)) ;
#67215=CARTESIAN_POINT('Ctrl Pts',(180.576936503322,533.981823088212,-47.5221601717599)) ;
#67216=CARTESIAN_POINT('Ctrl Pts',(180.516798861993,533.950254728962,-47.52216017176)) ;
#67217=CARTESIAN_POINT('Ctrl Pts',(180.454741783477,533.922300623552,-47.5221601717598)) ;
#67218=CARTESIAN_POINT('Ctrl Pts',(180.391083335664,533.897902195449,-47.5221601717597)) ;
#67219=CARTESIAN_POINT('Ctrl Pts',(180.366784181766,533.888589037813,-47.5221601717597)) ;
#67220=CARTESIAN_POINT('Ctrl Pts',(180.34225140207,533.879794410572,-47.5221601717596)) ;
#67221=CARTESIAN_POINT('Ctrl Pts',(180.317501726775,533.871516767415,-47.5221601717599)) ;
#67222=CARTESIAN_POINT('Ctrl Pts',(180.306601299242,533.867871069106,-47.52216017176)) ;
#67223=CARTESIAN_POINT('Ctrl Pts',(180.295659742371,533.864326067602,-47.5221601717597)) ;
#67224=CARTESIAN_POINT('Ctrl Pts',(180.284690809148,533.860885251216,-47.5221601717597)) ;
#67225=CARTESIAN_POINT('Ctrl Pts',(180.217926491994,533.839942124679,-47.5221601717597)) ;
#67226=CARTESIAN_POINT('Ctrl Pts',(180.150032205707,533.82281505825,-47.5221601717595)) ;
#67227=CARTESIAN_POINT('Ctrl Pts',(180.081372094379,533.80939571116,-47.5221601717596)) ;
#67228=CARTESIAN_POINT('Ctrl Pts',(180.011138794992,533.795668890688,-47.5221601717597)) ;
#67229=CARTESIAN_POINT('Ctrl Pts',(179.940103346079,533.785821371076,-47.5221601717597)) ;
#67230=CARTESIAN_POINT('Ctrl Pts',(179.868623579727,533.779783474225,-47.5221601717596)) ;
#67231=CARTESIAN_POINT('Ctrl Pts',(179.814610960391,533.775221027523,-47.5221601717596)) ;
#67232=CARTESIAN_POINT('Ctrl Pts',(179.760343876057,533.772834758855,-47.5221601717598)) ;
#67233=CARTESIAN_POINT('Ctrl Pts',(179.705969657728,533.772612887654,-47.5221601717596)) ;
#67234=CARTESIAN_POINT('Ctrl Pts',(179.672275133079,533.77247539888,-47.5221601717595)) ;
#67235=CARTESIAN_POINT('Ctrl Pts',(179.638539369937,533.7731693538,-47.5221601717597)) ;
#67236=CARTESIAN_POINT('Ctrl Pts',(179.604796964325,533.774695061605,-47.5221601717595)) ;
#67237=CARTESIAN_POINT('Ctrl Pts',(179.59189526542,533.775278429102,-47.5221601717594)) ;
#67238=CARTESIAN_POINT('Ctrl Pts',(179.578990310459,533.775983572458,-47.5221601717595)) ;
#67239=CARTESIAN_POINT('Ctrl Pts',(179.566091482587,533.776810113921,-47.5221601717595)) ;
#67240=CARTESIAN_POINT('Ctrl Pts',(179.489521093383,533.781716652879,-47.5221601717596)) ;
#67241=CARTESIAN_POINT('Ctrl Pts',(179.413353319935,533.790883056781,-47.5221601717595)) ;
#67242=CARTESIAN_POINT('Ctrl Pts',(179.338001691281,533.80424141487,-47.5221601717595)) ;
#67243=CARTESIAN_POINT('Ctrl Pts',(179.281487969791,533.814260183437,-47.5221601717596)) ;
#67244=CARTESIAN_POINT('Ctrl Pts',(179.225432662501,533.826638060617,-47.5221601717597)) ;
#67245=CARTESIAN_POINT('Ctrl Pts',(179.170006835869,533.841367503496,-47.5221601717597)) ;
#67246=CARTESIAN_POINT('Ctrl Pts',(179.150343573577,533.846593025899,-47.5221601717597)) ;
#67247=CARTESIAN_POINT('Ctrl Pts',(179.130759536777,533.852114683679,-47.5221601717597)) ;
#67248=CARTESIAN_POINT('Ctrl Pts',(179.111262400932,533.857932697529,-47.5221601717595)) ;
#67249=CARTESIAN_POINT('Ctrl Pts',(179.096495204142,533.862339280944,-47.5221601717594)) ;
#67250=CARTESIAN_POINT('Ctrl Pts',(179.081782737386,533.866914487841,-47.5221601717595)) ;
#67251=CARTESIAN_POINT('Ctrl Pts',(179.067135903331,533.87165551767,-47.5221601717595)) ;
#67252=CARTESIAN_POINT('Ctrl Pts',(178.995485989662,533.894847859212,-47.5221601717595)) ;
#67253=CARTESIAN_POINT('Ctrl Pts',(178.925350981393,533.922020779554,-47.5221601717598)) ;
#67254=CARTESIAN_POINT('Ctrl Pts',(178.857109801498,533.95314226278,-47.5221601717595)) ;
#67255=CARTESIAN_POINT('Ctrl Pts',(178.801970214503,533.978288746683,-47.5221601717592)) ;
#67256=CARTESIAN_POINT('Ctrl Pts',(178.748066676868,534.0060141123,-47.5221601717596)) ;
#67257=CARTESIAN_POINT('Ctrl Pts',(178.695602917514,534.036326095524,-47.5221601717597)) ;
#67258=CARTESIAN_POINT('Ctrl Pts',(178.685262867438,534.042300265662,-47.5221601717597)) ;
#67259=CARTESIAN_POINT('Ctrl Pts',(178.674978767005,534.048374980139,-47.52216017176)) ;
#67260=CARTESIAN_POINT('Ctrl Pts',(178.66475115082,534.054548898047,-47.5221601717599)) ;
#67261=CARTESIAN_POINT('',(181.15861657589,536.79152871558,-49.5230400807548)) ;
#67262=CARTESIAN_POINT('Ctrl Pts',(181.157234110517,536.790352109262,-49.5230400807548)) ;
#67263=CARTESIAN_POINT('Ctrl Pts',(181.152240231553,536.796219717345,-49.5227467777565)) ;
#67264=CARTESIAN_POINT('Ctrl Pts',(181.147205646513,536.802052680774,-49.5224534747582)) ;
#67265=CARTESIAN_POINT('Ctrl Pts',(181.142130839976,536.807850438129,-49.5221601717599)) ;
#67266=CARTESIAN_POINT('Ctrl Pts',(180.418697842595,533.725390834864,-49.5221601717599)) ;
#67267=CARTESIAN_POINT('Ctrl Pts',(180.487297636394,533.750790795206,-49.5221601717598)) ;
#67268=CARTESIAN_POINT('Ctrl Pts',(180.554195025763,533.780091250273,-49.5221601717596)) ;
#67269=CARTESIAN_POINT('Ctrl Pts',(180.61920218942,533.812995292462,-49.5221601717597)) ;
#67270=CARTESIAN_POINT('Ctrl Pts',(180.686073023045,533.846842650308,-49.5221601717599)) ;
#67271=CARTESIAN_POINT('Ctrl Pts',(180.750944469885,533.88450386658,-49.5221601717598)) ;
#67272=CARTESIAN_POINT('Ctrl Pts',(180.813580887979,533.925700546046,-49.5221601717598)) ;
#67273=CARTESIAN_POINT('Ctrl Pts',(180.866572112173,533.960553472571,-49.5221601717597)) ;
#67274=CARTESIAN_POINT('Ctrl Pts',(180.917963310832,533.997937920844,-49.5221601717599)) ;
#67275=CARTESIAN_POINT('Ctrl Pts',(180.967588972733,534.037703430217,-49.5221601717599)) ;
#67276=CARTESIAN_POINT('Ctrl Pts',(180.989598162914,534.0553396012,-49.5221601717598)) ;
#67277=CARTESIAN_POINT('Ctrl Pts',(181.01125977542,534.073444296496,-49.5221601717595)) ;
#67278=CARTESIAN_POINT('Ctrl Pts',(181.03255782176,534.092005111688,-49.5221601717594)) ;
#67279=CARTESIAN_POINT('Ctrl Pts',(181.04422687788,534.1021744573,-49.5221601717594)) ;
#67280=CARTESIAN_POINT('Ctrl Pts',(181.055786778592,534.112480730719,-49.5221601717597)) ;
#67281=CARTESIAN_POINT('Ctrl Pts',(181.067234761772,534.12292193265,-49.5221601717597)) ;
#67282=CARTESIAN_POINT('Ctrl Pts',(181.077875659478,534.132627027419,-49.5221601717597)) ;
#67283=CARTESIAN_POINT('Ctrl Pts',(181.088421379634,534.142450292378,-49.5221601717595)) ;
#67284=CARTESIAN_POINT('Ctrl Pts',(181.098853624774,534.152374457357,-49.5221601717595)) ;
#67285=CARTESIAN_POINT('Ctrl Pts',(181.151929238903,534.202865137353,-49.5221601717596)) ;
#67286=CARTESIAN_POINT('Ctrl Pts',(181.202164898294,534.25604865759,-49.5221601717595)) ;
#67287=CARTESIAN_POINT('Ctrl Pts',(181.24934253704,534.311661892117,-49.5221601717596)) ;
#67288=CARTESIAN_POINT('Ctrl Pts',(181.296166128424,534.366857773857,-49.5221601717597)) ;
#67289=CARTESIAN_POINT('Ctrl Pts',(181.339977934579,534.424447930197,-49.5221601717597)) ;
#67290=CARTESIAN_POINT('Ctrl Pts',(181.380519947539,534.484199350413,-49.5221601717596)) ;
#67291=CARTESIAN_POINT('Ctrl Pts',(181.414273339383,534.533945600105,-49.5221601717595)) ;
#67292=CARTESIAN_POINT('Ctrl Pts',(181.445759651354,534.585190575276,-49.5221601717597)) ;
#67293=CARTESIAN_POINT('Ctrl Pts',(181.47480219779,534.637806255418,-49.5221601717596)) ;
#67294=CARTESIAN_POINT('Ctrl Pts',(181.486863052554,534.659656614784,-49.5221601717596)) ;
#67295=CARTESIAN_POINT('Ctrl Pts',(181.498502135439,534.681743402877,-49.5221601717599)) ;
#67296=CARTESIAN_POINT('Ctrl Pts',(181.509705364919,534.704057527305,-49.5221601717596)) ;
#67297=CARTESIAN_POINT('Ctrl Pts',(181.514930645526,534.714465022915,-49.5221601717594)) ;
#67298=CARTESIAN_POINT('Ctrl Pts',(181.520061099594,534.724921972449,-49.5221601717596)) ;
#67299=CARTESIAN_POINT('Ctrl Pts',(181.525095232284,534.735427451061,-49.5221601717597)) ;
#67300=CARTESIAN_POINT('Ctrl Pts',(181.530288327452,534.746264660481,-49.5221601717599)) ;
#67301=CARTESIAN_POINT('Ctrl Pts',(181.535375235005,534.757145877216,-49.5221601717596)) ;
#67302=CARTESIAN_POINT('Ctrl Pts',(181.540353141824,534.768066253231,-49.5221601717596)) ;
#67303=CARTESIAN_POINT('Ctrl Pts',(181.568894008366,534.830678312034,-49.52216017176)) ;
#67304=CARTESIAN_POINT('Ctrl Pts',(181.593874352498,534.894615755507,-49.5221601717597)) ;
#67305=CARTESIAN_POINT('Ctrl Pts',(181.615071096175,534.959670773429,-49.5221601717597)) ;
#67306=CARTESIAN_POINT('Ctrl Pts',(181.634418034443,535.019048545549,-49.5221601717597)) ;
#67307=CARTESIAN_POINT('Ctrl Pts',(181.650612654374,535.079357955261,-49.5221601717597)) ;
#67308=CARTESIAN_POINT('Ctrl Pts',(181.663447662517,535.140445795219,-49.5221601717599)) ;
#67309=CARTESIAN_POINT('Ctrl Pts',(181.678533132294,535.21224464047,-49.5221601717601)) ;
#67310=CARTESIAN_POINT('Ctrl Pts',(181.688978110915,535.285120344497,-49.5221601717598)) ;
#67311=CARTESIAN_POINT('Ctrl Pts',(181.694857599082,535.358651547933,-49.5221601717599)) ;
#67312=CARTESIAN_POINT('Ctrl Pts',(181.696161835107,535.374962839277,-49.5221601717599)) ;
#67313=CARTESIAN_POINT('Ctrl Pts',(181.697241186125,535.39130630221,-49.52216017176)) ;
#67314=CARTESIAN_POINT('Ctrl Pts',(181.698096091594,535.407677166896,-49.52216017176)) ;
#67315=CARTESIAN_POINT('Ctrl Pts',(181.698933016579,535.423703717419,-49.52216017176)) ;
#67316=CARTESIAN_POINT('Ctrl Pts',(181.699554835009,535.439761827546,-49.5221601717599)) ;
#67317=CARTESIAN_POINT('Ctrl Pts',(181.699961459045,535.455815776155,-49.5221601717599)) ;
#67318=CARTESIAN_POINT('Ctrl Pts',(181.701697562433,535.524358980973,-49.5221601717597)) ;
#67319=CARTESIAN_POINT('Ctrl Pts',(181.699522602882,535.592920300968,-49.5221601717599)) ;
#67320=CARTESIAN_POINT('Ctrl Pts',(181.693557308922,535.661163908554,-49.5221601717598)) ;
#67321=CARTESIAN_POINT('Ctrl Pts',(181.687592743364,535.72939918315,-49.5221601717597)) ;
#67322=CARTESIAN_POINT('Ctrl Pts',(181.677838315832,535.79731788866,-49.5221601717597)) ;
#67323=CARTESIAN_POINT('Ctrl Pts',(181.664365101627,535.864569235536,-49.5221601717598)) ;
#67324=CARTESIAN_POINT('Ctrl Pts',(181.654515187308,535.91373493531,-49.52216017176)) ;
#67325=CARTESIAN_POINT('Ctrl Pts',(181.642676644468,535.962543698494,-49.5221601717599)) ;
#67326=CARTESIAN_POINT('Ctrl Pts',(181.628862533981,536.010848459207,-49.5221601717601)) ;
#67327=CARTESIAN_POINT('Ctrl Pts',(181.623150206523,536.03082315184,-49.5221601717602)) ;
#67328=CARTESIAN_POINT('Ctrl Pts',(181.617099932002,536.050711540705,-49.52216017176)) ;
#67329=CARTESIAN_POINT('Ctrl Pts',(181.610712076097,536.070502654402,-49.5221601717599)) ;
#67330=CARTESIAN_POINT('Ctrl Pts',(181.605971227629,536.085190942998,-49.5221601717597)) ;
#67331=CARTESIAN_POINT('Ctrl Pts',(181.601044429239,536.099825644399,-49.52216017176)) ;
#67332=CARTESIAN_POINT('Ctrl Pts',(181.595931721971,536.114402135746,-49.5221601717599)) ;
#67333=CARTESIAN_POINT('Ctrl Pts',(181.591629159901,536.126668877315,-49.5221601717598)) ;
#67334=CARTESIAN_POINT('Ctrl Pts',(181.587197704363,536.138886424694,-49.5221601717601)) ;
#67335=CARTESIAN_POINT('Ctrl Pts',(181.582639148766,536.151048855726,-49.5221601717601)) ;
#67336=CARTESIAN_POINT('Ctrl Pts',(181.559528847451,536.212708177395,-49.52216017176)) ;
#67337=CARTESIAN_POINT('Ctrl Pts',(181.533144770481,536.272982567931,-49.52216017176)) ;
#67338=CARTESIAN_POINT('Ctrl Pts',(181.503537114218,536.331539926083,-49.5221601717599)) ;
#67339=CARTESIAN_POINT('Ctrl Pts',(181.482573948164,536.373000405483,-49.5221601717599)) ;
#67340=CARTESIAN_POINT('Ctrl Pts',(181.459993913709,536.413599596872,-49.5221601717601)) ;
#67341=CARTESIAN_POINT('Ctrl Pts',(181.435804180235,536.453208026963,-49.5221601717603)) ;
#67342=CARTESIAN_POINT('Ctrl Pts',(181.42807699997,536.465860563199,-49.5221601717603)) ;
#67343=CARTESIAN_POINT('Ctrl Pts',(181.420184269904,536.478413807954,-49.5221601717601)) ;
#67344=CARTESIAN_POINT('Ctrl Pts',(181.412130015855,536.490857193274,-49.5221601717601)) ;
#67345=CARTESIAN_POINT('Ctrl Pts',(181.377866042633,536.543793172047,-49.5221601717601)) ;
#67346=CARTESIAN_POINT('Ctrl Pts',(181.340745918553,536.594646264424,-49.5221601717597)) ;
#67347=CARTESIAN_POINT('Ctrl Pts',(181.300803879855,536.643102920757,-49.52216017176)) ;
#67348=CARTESIAN_POINT('Ctrl Pts',(181.263594869918,536.688243936733,-49.5221601717603)) ;
#67349=CARTESIAN_POINT('Ctrl Pts',(181.223936346045,536.731305409684,-49.5221601717598)) ;
#67350=CARTESIAN_POINT('Ctrl Pts',(181.181833737656,536.771999681009,-49.5221601717601)) ;
#67351=CARTESIAN_POINT('Ctrl Pts',(181.174644864848,536.7789480852,-49.5221601717601)) ;
#67352=CARTESIAN_POINT('Ctrl Pts',(181.167384690605,536.78582738569,-49.5221601717596)) ;
#67353=CARTESIAN_POINT('Ctrl Pts',(181.160054448737,536.792637064758,-49.5221601717595)) ;
#67354=CARTESIAN_POINT('Ctrl Pts',(178.622419190323,536.788246779922,-49.5202730914232)) ;
#67355=CARTESIAN_POINT('Ctrl Pts',(178.263637748317,536.36676207672,-49.4831846742774)) ;
#67356=CARTESIAN_POINT('Ctrl Pts',(178.008514861325,535.14256091782,-49.4090221751792)) ;
#67357=CARTESIAN_POINT('Ctrl Pts',(179.347310763183,533.819203307332,-49.2977855941286)) ;
#67358=CARTESIAN_POINT('Ctrl Pts',(181.184535504429,534.231765349117,-49.1865633482713)) ;
#67359=CARTESIAN_POINT('Ctrl Pts',(181.833489463951,535.998142408068,-49.075341102414)) ;
#67360=CARTESIAN_POINT('Ctrl Pts',(180.700261197456,537.501346936019,-48.9641188565566)) ;
#67361=CARTESIAN_POINT('Ctrl Pts',(178.822946992655,537.362808329003,-48.8528966106991)) ;
#67362=CARTESIAN_POINT('Ctrl Pts',(177.922442264761,535.709930020042,-48.7416743648417)) ;
#67363=CARTESIAN_POINT('Ctrl Pts',(178.824009613428,534.057562707726,-48.6304521189843)) ;
#67364=CARTESIAN_POINT('Ctrl Pts',(180.701322763348,533.920325250683,-48.519229873127)) ;
#67365=CARTESIAN_POINT('Ctrl Pts',(181.833640222805,535.42398090139,-48.4080076272697)) ;
#67366=CARTESIAN_POINT('Ctrl Pts',(181.183108346156,537.190313662327,-48.2967853814123)) ;
#67367=CARTESIAN_POINT('Ctrl Pts',(179.345987355079,537.600344449737,-48.1855631355549)) ;
#67368=CARTESIAN_POINT('Ctrl Pts',(178.00617051876,536.278212737651,-48.0743408896974)) ;
#67369=CARTESIAN_POINT('Ctrl Pts',(178.39170274318,534.435855450606,-47.9631186438401)) ;
#67370=CARTESIAN_POINT('Ctrl Pts',(180.149288064919,533.761766876316,-47.8518963979828)) ;
#67371=CARTESIAN_POINT('Ctrl Pts',(181.667901731917,534.874260780677,-47.7406741521255)) ;
#67372=CARTESIAN_POINT('Ctrl Pts',(181.555965320099,536.752744050679,-47.6294519062681)) ;
#67373=CARTESIAN_POINT('Ctrl Pts',(179.91579713902,537.677649735568,-47.5182296604107)) ;
#67374=CARTESIAN_POINT('Ctrl Pts',(178.252194934696,536.796634656889,-47.4069913524144)) ;
#67375=CARTESIAN_POINT('Ctrl Pts',(178.143425297585,535.55082917805,-47.3328271263707)) ;
#67376=CARTESIAN_POINT('Ctrl Pts',(178.365436513798,535.043765566178,-47.2957369822794)) ;
#67377=CARTESIAN_POINT('Ctrl Pts',(178.520858913152,536.874692490996,-49.597273851344)) ;
#67378=CARTESIAN_POINT('Ctrl Pts',(178.133297990902,536.419398595709,-49.5601854341982)) ;
#67379=CARTESIAN_POINT('Ctrl Pts',(177.857710544637,535.096998731576,-49.4860229350999)) ;
#67380=CARTESIAN_POINT('Ctrl Pts',(179.303897313739,533.667488628938,-49.3747863540493)) ;
#67381=CARTESIAN_POINT('Ctrl Pts',(181.288494151068,534.113144135825,-49.263564108192)) ;
#67382=CARTESIAN_POINT('Ctrl Pts',(181.989503639305,536.021210278212,-49.1523418623347)) ;
#67383=CARTESIAN_POINT('Ctrl Pts',(180.765374014243,537.644993632014,-49.0411196164771)) ;
#67384=CARTESIAN_POINT('Ctrl Pts',(178.737471956384,537.495342217487,-48.9298973706197)) ;
#67385=CARTESIAN_POINT('Ctrl Pts',(177.764733676274,535.709879072554,-48.8186751247623)) ;
#67386=CARTESIAN_POINT('Ctrl Pts',(178.73861981477,533.924967913615,-48.707452878905)) ;
#67387=CARTESIAN_POINT('Ctrl Pts',(180.76652073313,533.776722020178,-48.5962306330477)) ;
#67388=CARTESIAN_POINT('Ctrl Pts',(181.989666491209,535.400992683332,-48.4850083871904)) ;
#67389=CARTESIAN_POINT('Ctrl Pts',(181.286952513983,537.30901097436,-48.3737861413329)) ;
#67390=CARTESIAN_POINT('Ctrl Pts',(179.302467749094,537.751932183525,-48.2625638954756)) ;
#67391=CARTESIAN_POINT('Ctrl Pts',(177.855178151765,536.323746314136,-48.151341649618)) ;
#67392=CARTESIAN_POINT('Ctrl Pts',(178.271635657531,534.333605226323,-48.0401194037607)) ;
#67393=CARTESIAN_POINT('Ctrl Pts',(180.170204837748,533.605444962321,-47.9288971579034)) ;
#67394=CARTESIAN_POINT('Ctrl Pts',(181.810633367249,534.807177028397,-47.8176749120461)) ;
#67395=CARTESIAN_POINT('Ctrl Pts',(181.689718030172,536.836341927457,-47.7064526661887)) ;
#67396=CARTESIAN_POINT('Ctrl Pts',(179.917984549896,537.835438475557,-47.5952304203312)) ;
#67397=CARTESIAN_POINT('Ctrl Pts',(178.120937297508,536.883753197465,-47.483992112335)) ;
#67398=CARTESIAN_POINT('Ctrl Pts',(178.003442756441,535.538016033293,-47.4098278862913)) ;
#67399=CARTESIAN_POINT('Ctrl Pts',(178.243262495234,534.990278558474,-47.3727377422)) ;
#67400=CARTESIAN_POINT('Ctrl Pts',(178.419298635981,536.961138202069,-49.6742746112646)) ;
#67401=CARTESIAN_POINT('Ctrl Pts',(178.002958233487,536.4720351147,-49.6371861941188)) ;
#67402=CARTESIAN_POINT('Ctrl Pts',(177.706906227949,535.051436545331,-49.5630236950206)) ;
#67403=CARTESIAN_POINT('Ctrl Pts',(179.260483864295,533.515773950542,-49.45178711397)) ;
#67404=CARTESIAN_POINT('Ctrl Pts',(181.392452797707,533.994522922533,-49.3405648681127)) ;
#67405=CARTESIAN_POINT('Ctrl Pts',(182.14551781466,536.044278148355,-49.2293426222554)) ;
#67406=CARTESIAN_POINT('Ctrl Pts',(180.830486831031,537.788640328009,-49.1181203763979)) ;
#67407=CARTESIAN_POINT('Ctrl Pts',(178.651996920114,537.627876105971,-49.0068981305405)) ;
#67408=CARTESIAN_POINT('Ctrl Pts',(177.607025087785,535.709828125064,-48.895675884683)) ;
#67409=CARTESIAN_POINT('Ctrl Pts',(178.653230016112,533.792373119504,-48.7844536388257)) ;
#67410=CARTESIAN_POINT('Ctrl Pts',(180.831718702914,533.633118789673,-48.6732313929684)) ;
#67411=CARTESIAN_POINT('Ctrl Pts',(182.145692759613,535.378004465272,-48.5620091471111)) ;
#67412=CARTESIAN_POINT('Ctrl Pts',(181.390796681811,537.427708286391,-48.4507869012537)) ;
#67413=CARTESIAN_POINT('Ctrl Pts',(179.258948143106,537.903519917313,-48.3395646553962)) ;
#67414=CARTESIAN_POINT('Ctrl Pts',(177.704185784769,536.369279890622,-48.2283424095388)) ;
#67415=CARTESIAN_POINT('Ctrl Pts',(178.151568571882,534.231355002041,-48.1171201636814)) ;
#67416=CARTESIAN_POINT('Ctrl Pts',(180.191121610576,533.449123048327,-48.0058979178242)) ;
#67417=CARTESIAN_POINT('Ctrl Pts',(181.953365002583,534.740093276118,-47.8946756719669)) ;
#67418=CARTESIAN_POINT('Ctrl Pts',(181.823470740244,536.919939804236,-47.7834534261095)) ;
#67419=CARTESIAN_POINT('Ctrl Pts',(179.920171960771,537.993227215544,-47.672231180252)) ;
#67420=CARTESIAN_POINT('Ctrl Pts',(177.98967966032,536.970871738042,-47.5609928722558)) ;
#67421=CARTESIAN_POINT('Ctrl Pts',(177.863460215298,535.525202888537,-47.486828646212)) ;
#67422=CARTESIAN_POINT('Ctrl Pts',(178.12108847667,534.936791550772,-47.4497385021208)) ;
#67423=CARTESIAN_POINT('Ctrl Pts',(178.31773835881,537.047583913142,-49.7512753711853)) ;
#67424=CARTESIAN_POINT('Ctrl Pts',(177.872618476071,536.52467163369,-49.7141869540395)) ;
#67425=CARTESIAN_POINT('Ctrl Pts',(177.556101911261,535.005874359087,-49.6400244549413)) ;
#67426=CARTESIAN_POINT('Ctrl Pts',(179.217070414851,533.364059272146,-49.5287878738906)) ;
#67427=CARTESIAN_POINT('Ctrl Pts',(181.496411444346,533.875901709242,-49.4175656280333)) ;
#67428=CARTESIAN_POINT('Ctrl Pts',(182.301531990017,536.067346018498,-49.306343382176)) ;
#67429=CARTESIAN_POINT('Ctrl Pts',(180.895599647818,537.932287024005,-49.1951211363185)) ;
#67430=CARTESIAN_POINT('Ctrl Pts',(178.566521883845,537.760409994454,-49.0838988904611)) ;
#67431=CARTESIAN_POINT('Ctrl Pts',(177.449316499298,535.709777177576,-48.9726766446036)) ;
#67432=CARTESIAN_POINT('Ctrl Pts',(178.567840217455,533.659778325394,-48.8614543987463)) ;
#67433=CARTESIAN_POINT('Ctrl Pts',(180.896916672697,533.489515559168,-48.750232152889)) ;
#67434=CARTESIAN_POINT('Ctrl Pts',(182.301719028018,535.355016247213,-48.6390099070317)) ;
#67435=CARTESIAN_POINT('Ctrl Pts',(181.494640849637,537.546405598424,-48.5277876611743)) ;
#67436=CARTESIAN_POINT('Ctrl Pts',(179.215428537121,538.0551076511,-48.4165654153168)) ;
#67437=CARTESIAN_POINT('Ctrl Pts',(177.553193417773,536.414813467106,-48.3053431694594)) ;
#67438=CARTESIAN_POINT('Ctrl Pts',(178.031501486233,534.129104777759,-48.194120923602)) ;
#67439=CARTESIAN_POINT('Ctrl Pts',(180.212038383404,533.292801134333,-48.0828986777447)) ;
#67440=CARTESIAN_POINT('Ctrl Pts',(182.096096637916,534.673009523839,-47.9716764318875)) ;
#67441=CARTESIAN_POINT('Ctrl Pts',(181.957223450317,537.003537681016,-47.8604541860301)) ;
#67442=CARTESIAN_POINT('Ctrl Pts',(179.922359371647,538.151015955532,-47.7492319401726)) ;
#67443=CARTESIAN_POINT('Ctrl Pts',(177.858422023132,537.057990278619,-47.6379936321763)) ;
#67444=CARTESIAN_POINT('Ctrl Pts',(177.723477674154,535.512389743781,-47.5638294061326)) ;
#67445=CARTESIAN_POINT('Ctrl Pts',(177.998914458105,534.883304543068,-47.5267392620414)) ;
#67446=CARTESIAN_POINT('',(179.941771410307,537.377530426179,-47.5212802703069)) ;
#67447=CARTESIAN_POINT('Ctrl Pts',(178.005900115743,534.887332980433,-47.5221601717595)) ;
#67448=CARTESIAN_POINT('Ctrl Pts',(177.982987331993,534.956803076843,-47.5221601717592)) ;
#67449=CARTESIAN_POINT('Ctrl Pts',(177.964185509426,535.027374098354,-47.5221601717594)) ;
#67450=CARTESIAN_POINT('Ctrl Pts',(177.949379621047,535.098714081534,-47.5221601717595)) ;
#67451=CARTESIAN_POINT('Ctrl Pts',(177.934149267583,535.172099286938,-47.5221601717595)) ;
#67452=CARTESIAN_POINT('Ctrl Pts',(177.923147305685,535.246299210421,-47.5221601717596)) ;
#67453=CARTESIAN_POINT('Ctrl Pts',(177.916302997627,535.320956043131,-47.5221601717597)) ;
#67454=CARTESIAN_POINT('Ctrl Pts',(177.910512624069,535.384116693759,-47.5221601717597)) ;
#67455=CARTESIAN_POINT('Ctrl Pts',(177.907699073298,535.447604771906,-47.5221601717597)) ;
#67456=CARTESIAN_POINT('Ctrl Pts',(177.907847905046,535.511197065041,-47.5221601717597)) ;
#67457=CARTESIAN_POINT('Ctrl Pts',(177.907913912551,535.539400513806,-47.5221601717596)) ;
#67458=CARTESIAN_POINT('Ctrl Pts',(177.908562938165,535.567624335509,-47.5221601717597)) ;
#67459=CARTESIAN_POINT('Ctrl Pts',(177.909795252389,535.595848295825,-47.5221601717594)) ;
#67460=CARTESIAN_POINT('Ctrl Pts',(177.910470429113,535.61131201497,-47.5221601717592)) ;
#67461=CARTESIAN_POINT('Ctrl Pts',(177.911320717597,535.626775766067,-47.5221601717594)) ;
#67462=CARTESIAN_POINT('Ctrl Pts',(177.912346276888,535.64223614306,-47.5221601717594)) ;
#67463=CARTESIAN_POINT('Ctrl Pts',(177.913299533898,535.65660655817,-47.5221601717594)) ;
#67464=CARTESIAN_POINT('Ctrl Pts',(177.914404522285,535.670976238378,-47.5221601717596)) ;
#67465=CARTESIAN_POINT('Ctrl Pts',(177.915659147972,535.685320110379,-47.5221601717596)) ;
#67466=CARTESIAN_POINT('Ctrl Pts',(177.92204224511,535.75829671947,-47.5221601717597)) ;
#67467=CARTESIAN_POINT('Ctrl Pts',(177.932301372236,535.830731920874,-47.5221601717597)) ;
#67468=CARTESIAN_POINT('Ctrl Pts',(177.946366771134,535.902291167493,-47.5221601717596)) ;
#67469=CARTESIAN_POINT('Ctrl Pts',(177.960217864007,535.972760108906,-47.5221601717596)) ;
#67470=CARTESIAN_POINT('Ctrl Pts',(177.977760553777,536.04238048792,-47.5221601717593)) ;
#67471=CARTESIAN_POINT('Ctrl Pts',(177.998973857845,536.110813461122,-47.5221601717592)) ;
#67472=CARTESIAN_POINT('Ctrl Pts',(178.016940288639,536.168772196503,-47.5221601717591)) ;
#67473=CARTESIAN_POINT('Ctrl Pts',(178.037540545391,536.225879158725,-47.5221601717595)) ;
#67474=CARTESIAN_POINT('Ctrl Pts',(178.060784890946,536.281910303999,-47.5221601717594)) ;
#67475=CARTESIAN_POINT('Ctrl Pts',(178.070348369247,536.304963336004,-47.5221601717594)) ;
#67476=CARTESIAN_POINT('Ctrl Pts',(178.080359665454,536.327834024376,-47.5221601717598)) ;
#67477=CARTESIAN_POINT('Ctrl Pts',(178.090820450542,536.35050569072,-47.5221601717597)) ;
#67478=CARTESIAN_POINT('Ctrl Pts',(178.095699449288,536.361079947886,-47.5221601717597)) ;
#67479=CARTESIAN_POINT('Ctrl Pts',(178.100676236072,536.371610900689,-47.5221601717599)) ;
#67480=CARTESIAN_POINT('Ctrl Pts',(178.105751019838,536.382096803783,-47.5221601717599)) ;
#67481=CARTESIAN_POINT('Ctrl Pts',(178.110986048596,536.392913817235,-47.5221601717598)) ;
#67482=CARTESIAN_POINT('Ctrl Pts',(178.116321690533,536.403675247986,-47.5221601717598)) ;
#67483=CARTESIAN_POINT('Ctrl Pts',(178.121755909257,536.414375873961,-47.5221601717598)) ;
#67484=CARTESIAN_POINT('Ctrl Pts',(178.152913046783,536.475728000555,-47.5221601717598)) ;
#67485=CARTESIAN_POINT('Ctrl Pts',(178.18732636127,536.535122762543,-47.5221601717595)) ;
#67486=CARTESIAN_POINT('Ctrl Pts',(178.224972467088,536.592256182975,-47.5221601717596)) ;
#67487=CARTESIAN_POINT('Ctrl Pts',(178.259333258394,536.644403662598,-47.5221601717597)) ;
#67488=CARTESIAN_POINT('Ctrl Pts',(178.296387871761,536.694667427142,-47.5221601717599)) ;
#67489=CARTESIAN_POINT('Ctrl Pts',(178.336145770263,536.742789884874,-47.5221601717597)) ;
#67490=CARTESIAN_POINT('Ctrl Pts',(178.382874729947,536.799350026934,-47.5221601717594)) ;
#67491=CARTESIAN_POINT('Ctrl Pts',(178.433338910899,536.852953497548,-47.5221601717598)) ;
#67492=CARTESIAN_POINT('Ctrl Pts',(178.487162118891,536.903396221338,-47.5221601717598)) ;
#67493=CARTESIAN_POINT('Ctrl Pts',(178.499101622087,536.914585837943,-47.5221601717598)) ;
#67494=CARTESIAN_POINT('Ctrl Pts',(178.511206491567,536.925619691031,-47.52216017176)) ;
#67495=CARTESIAN_POINT('Ctrl Pts',(178.523472724127,536.936495150239,-47.5221601717599)) ;
#67496=CARTESIAN_POINT('Ctrl Pts',(178.535480971503,536.947141875209,-47.5221601717598)) ;
#67497=CARTESIAN_POINT('Ctrl Pts',(178.547648009925,536.957640100201,-47.5221601717596)) ;
#67498=CARTESIAN_POINT('Ctrl Pts',(178.55994596626,536.967967484784,-47.5221601717596)) ;
#67499=CARTESIAN_POINT('Ctrl Pts',(178.612452758427,537.012060813882,-47.5221601717597)) ;
#67500=CARTESIAN_POINT('Ctrl Pts',(178.66741222166,537.053107645582,-47.5221601717598)) ;
#67501=CARTESIAN_POINT('Ctrl Pts',(178.724486522341,537.090992984155,-47.5221601717597)) ;
#67502=CARTESIAN_POINT('Ctrl Pts',(178.781553853922,537.128873696712,-47.5221601717596)) ;
#67503=CARTESIAN_POINT('Ctrl Pts',(178.840736622279,537.163593998352,-47.5221601717598)) ;
#67504=CARTESIAN_POINT('Ctrl Pts',(178.901716254342,537.194990744259,-47.5221601717599)) ;
#67505=CARTESIAN_POINT('Ctrl Pts',(178.946296867578,537.217944083576,-47.52216017176)) ;
#67506=CARTESIAN_POINT('Ctrl Pts',(178.991838306226,537.239120104217,-47.5221601717598)) ;
#67507=CARTESIAN_POINT('Ctrl Pts',(179.038217446212,537.258437323501,-47.5221601717598)) ;
#67508=CARTESIAN_POINT('Ctrl Pts',(179.057395867761,537.266425263223,-47.5221601717598)) ;
#67509=CARTESIAN_POINT('Ctrl Pts',(179.076717520864,537.274095175778,-47.5221601717596)) ;
#67510=CARTESIAN_POINT('Ctrl Pts',(179.096173599739,537.28144050651,-47.5221601717598)) ;
#67511=CARTESIAN_POINT('Ctrl Pts',(179.110613234786,537.28689195928,-47.5221601717599)) ;
#67512=CARTESIAN_POINT('Ctrl Pts',(179.125126911539,537.292164619533,-47.5221601717598)) ;
#67513=CARTESIAN_POINT('Ctrl Pts',(179.139710990113,537.297255637053,-47.5221601717597)) ;
#67514=CARTESIAN_POINT('Ctrl Pts',(179.151984119639,537.301539947312,-47.5221601717596)) ;
#67515=CARTESIAN_POINT('Ctrl Pts',(179.164299151377,537.305692812503,-47.5221601717595)) ;
#67516=CARTESIAN_POINT('Ctrl Pts',(179.176650337018,537.309711942362,-47.5221601717596)) ;
#67517=CARTESIAN_POINT('Ctrl Pts',(179.239266573345,537.330087539685,-47.5221601717596)) ;
#67518=CARTESIAN_POINT('Ctrl Pts',(179.302841192719,537.347040105753,-47.5221601717595)) ;
#67519=CARTESIAN_POINT('Ctrl Pts',(179.367083250977,537.360401823903,-47.5221601717597)) ;
#67520=CARTESIAN_POINT('Ctrl Pts',(179.412568679346,537.369862346966,-47.5221601717598)) ;
#67521=CARTESIAN_POINT('Ctrl Pts',(179.45838882661,537.377521747157,-47.5221601717597)) ;
#67522=CARTESIAN_POINT('Ctrl Pts',(179.504437996434,537.383304904446,-47.5221601717596)) ;
#67523=CARTESIAN_POINT('Ctrl Pts',(179.519147966194,537.385152279093,-47.5221601717596)) ;
#67524=CARTESIAN_POINT('Ctrl Pts',(179.533883525363,537.386808314458,-47.5221601717597)) ;
#67525=CARTESIAN_POINT('Ctrl Pts',(179.548633901525,537.388269569041,-47.5221601717598)) ;
#67526=CARTESIAN_POINT('Ctrl Pts',(179.61138415443,537.394485959298,-47.52216017176)) ;
#67527=CARTESIAN_POINT('Ctrl Pts',(179.67428672212,537.397170662507,-47.5221601717597)) ;
#67528=CARTESIAN_POINT('Ctrl Pts',(179.737075115641,537.396154950622,-47.5221601717598)) ;
#67529=CARTESIAN_POINT('Ctrl Pts',(179.795567221839,537.395208738685,-47.52216017176)) ;
#67530=CARTESIAN_POINT('Ctrl Pts',(179.853960722779,537.39105084576,-47.5221601717601)) ;
#67531=CARTESIAN_POINT('Ctrl Pts',(179.912027332698,537.383506164524,-47.5221601717599)) ;
#67532=CARTESIAN_POINT('Ctrl Pts',(179.921942002788,537.382217936651,-47.5221601717599)) ;
#67533=CARTESIAN_POINT('Ctrl Pts',(179.931847101145,537.380830877618,-47.52216017176)) ;
#67534=CARTESIAN_POINT('Ctrl Pts',(179.94174145373,537.379345629264,-47.52216017176)) ;
#67535=CARTESIAN_POINT('Ctrl Pts',(178.619456745554,536.789923813584,-49.5221601717597)) ;
#67536=CARTESIAN_POINT('Ctrl Pts',(178.574187252732,536.747692181376,-49.5221601717596)) ;
#67537=CARTESIAN_POINT('Ctrl Pts',(178.531651301387,536.702886203401,-49.5221601717594)) ;
#67538=CARTESIAN_POINT('Ctrl Pts',(178.491845127613,536.655851978916,-49.5221601717595)) ;
#67539=CARTESIAN_POINT('Ctrl Pts',(178.449308935779,536.605592016557,-49.5221601717595)) ;
#67540=CARTESIAN_POINT('Ctrl Pts',(178.409889057913,536.552787473376,-49.5221601717596)) ;
#67541=CARTESIAN_POINT('Ctrl Pts',(178.373610042644,536.497805513443,-49.5221601717596)) ;
#67542=CARTESIAN_POINT('Ctrl Pts',(178.341865904283,536.449696298502,-49.5221601717596)) ;
#67543=CARTESIAN_POINT('Ctrl Pts',(178.31252673872,536.399918761028,-49.52216017176)) ;
#67544=CARTESIAN_POINT('Ctrl Pts',(178.285632078592,536.348691089427,-49.5221601717597)) ;
#67545=CARTESIAN_POINT('Ctrl Pts',(178.272117344439,536.322948865519,-49.5221601717596)) ;
#67546=CARTESIAN_POINT('Ctrl Pts',(178.259220242575,536.296840105165,-49.5221601717596)) ;
#67547=CARTESIAN_POINT('Ctrl Pts',(178.246948159264,536.270390629596,-49.5221601717598)) ;
#67548=CARTESIAN_POINT('Ctrl Pts',(178.241395541397,536.258423319165,-49.5221601717599)) ;
#67549=CARTESIAN_POINT('Ctrl Pts',(178.235970381399,536.246384756721,-49.5221601717596)) ;
#67550=CARTESIAN_POINT('Ctrl Pts',(178.230681666114,536.234296885241,-49.5221601717596)) ;
#67551=CARTESIAN_POINT('Ctrl Pts',(178.203843422477,536.17295547766,-49.5221601717596)) ;
#67552=CARTESIAN_POINT('Ctrl Pts',(178.180463478443,536.110237033969,-49.5221601717599)) ;
#67553=CARTESIAN_POINT('Ctrl Pts',(178.160562809962,536.046500976405,-49.5221601717598)) ;
#67554=CARTESIAN_POINT('Ctrl Pts',(178.140300022872,535.981605158178,-49.5221601717598)) ;
#67555=CARTESIAN_POINT('Ctrl Pts',(178.123643729798,535.915653513645,-49.5221601717599)) ;
#67556=CARTESIAN_POINT('Ctrl Pts',(178.110655417353,535.848988876354,-49.5221601717597)) ;
#67557=CARTESIAN_POINT('Ctrl Pts',(178.099760971122,535.793071349764,-49.5221601717596)) ;
#67558=CARTESIAN_POINT('Ctrl Pts',(178.091447740656,535.736651240133,-49.5221601717597)) ;
#67559=CARTESIAN_POINT('Ctrl Pts',(178.085777052212,535.679918461616,-49.5221601717597)) ;
#67560=CARTESIAN_POINT('Ctrl Pts',(178.083157269475,535.653708671526,-49.5221601717597)) ;
#67561=CARTESIAN_POINT('Ctrl Pts',(178.081101828741,535.627432033194,-49.52216017176)) ;
#67562=CARTESIAN_POINT('Ctrl Pts',(178.079618613066,535.601106865551,-49.5221601717599)) ;
#67563=CARTESIAN_POINT('Ctrl Pts',(178.078979635639,535.589765839312,-49.5221601717599)) ;
#67564=CARTESIAN_POINT('Ctrl Pts',(178.078446992385,535.578416386461,-49.5221601717598)) ;
#67565=CARTESIAN_POINT('Ctrl Pts',(178.078021602998,535.567073472083,-49.5221601717598)) ;
#67566=CARTESIAN_POINT('Ctrl Pts',(178.075389312044,535.496884013118,-49.52216017176)) ;
#67567=CARTESIAN_POINT('Ctrl Pts',(178.076851985684,535.4268141808,-49.5221601717599)) ;
#67568=CARTESIAN_POINT('Ctrl Pts',(178.082461748157,535.357227447347,-49.5221601717599)) ;
#67569=CARTESIAN_POINT('Ctrl Pts',(178.087506025577,535.294655317063,-49.5221601717599)) ;
#67570=CARTESIAN_POINT('Ctrl Pts',(178.095903772788,535.232472824493,-49.52216017176)) ;
#67571=CARTESIAN_POINT('Ctrl Pts',(178.107726699417,535.170931882839,-49.52216017176)) ;
#67572=CARTESIAN_POINT('Ctrl Pts',(178.120540767056,535.104231833544,-49.5221601717599)) ;
#67573=CARTESIAN_POINT('Ctrl Pts',(178.137377321743,535.038284558039,-49.52216017176)) ;
#67574=CARTESIAN_POINT('Ctrl Pts',(178.157992254397,534.97330220996,-49.5221601717597)) ;
#67575=CARTESIAN_POINT('Ctrl Pts',(178.165861208992,534.948497707562,-49.5221601717596)) ;
#67576=CARTESIAN_POINT('Ctrl Pts',(178.17428123032,534.923833847552,-49.5221601717598)) ;
#67577=CARTESIAN_POINT('Ctrl Pts',(178.183240678315,534.899322746024,-49.5221601717597)) ;
#67578=CARTESIAN_POINT('Ctrl Pts',(178.187186661782,534.888527393294,-49.5221601717596)) ;
#67579=CARTESIAN_POINT('Ctrl Pts',(178.191237016904,534.877762667777,-49.5221601717597)) ;
#67580=CARTESIAN_POINT('Ctrl Pts',(178.195385896106,534.867041496919,-49.5221601717597)) ;
#67581=CARTESIAN_POINT('Ctrl Pts',(178.220638770266,534.801785227622,-49.5221601717595)) ;
#67582=CARTESIAN_POINT('Ctrl Pts',(178.249579684661,534.73802478725,-49.5221601717595)) ;
#67583=CARTESIAN_POINT('Ctrl Pts',(178.281896894921,534.675977325775,-49.5221601717595)) ;
#67584=CARTESIAN_POINT('Ctrl Pts',(178.314954579631,534.612508189609,-49.5221601717596)) ;
#67585=CARTESIAN_POINT('Ctrl Pts',(178.351545356018,534.550830612049,-49.5221601717594)) ;
#67586=CARTESIAN_POINT('Ctrl Pts',(178.391391642872,534.491180913923,-49.5221601717596)) ;
#67587=CARTESIAN_POINT('Ctrl Pts',(178.421500896408,534.446107507438,-49.5221601717597)) ;
#67588=CARTESIAN_POINT('Ctrl Pts',(178.453470210955,534.402191977027,-49.5221601717595)) ;
#67589=CARTESIAN_POINT('Ctrl Pts',(178.487198516698,534.359542165663,-49.5221601717594)) ;
#67590=CARTESIAN_POINT('Ctrl Pts',(178.508099216798,534.333113001879,-49.5221601717593)) ;
#67591=CARTESIAN_POINT('Ctrl Pts',(178.529675677596,534.307169993219,-49.5221601717598)) ;
#67592=CARTESIAN_POINT('Ctrl Pts',(178.551906570558,534.281740380727,-49.5221601717596)) ;
#67593=CARTESIAN_POINT('Ctrl Pts',(178.560406742799,534.272017150689,-49.5221601717596)) ;
#67594=CARTESIAN_POINT('Ctrl Pts',(178.569004153348,534.262367300958,-49.5221601717594)) ;
#67595=CARTESIAN_POINT('Ctrl Pts',(178.57769265657,534.252797932049,-49.5221601717594)) ;
#67596=CARTESIAN_POINT('Ctrl Pts',(178.629269599752,534.19599196859,-49.5221601717595)) ;
#67597=CARTESIAN_POINT('Ctrl Pts',(178.683926012683,534.14215676504,-49.5221601717594)) ;
#67598=CARTESIAN_POINT('Ctrl Pts',(178.741350969432,534.091573289781,-49.5221601717595)) ;
#67599=CARTESIAN_POINT('Ctrl Pts',(178.784419686994,534.053635683337,-49.5221601717596)) ;
#67600=CARTESIAN_POINT('Ctrl Pts',(178.829047013371,534.017527359659,-49.5221601717598)) ;
#67601=CARTESIAN_POINT('Ctrl Pts',(178.875120393075,533.98337736097,-49.5221601717596)) ;
#67602=CARTESIAN_POINT('Ctrl Pts',(178.891465719858,533.971262059427,-49.5221601717596)) ;
#67603=CARTESIAN_POINT('Ctrl Pts',(178.907993178436,533.959393336413,-49.5221601717597)) ;
#67604=CARTESIAN_POINT('Ctrl Pts',(178.924698155776,533.947777330454,-49.5221601717595)) ;
#67605=CARTESIAN_POINT('Ctrl Pts',(178.937350560939,533.938979329069,-49.5221601717593)) ;
#67606=CARTESIAN_POINT('Ctrl Pts',(178.950100677659,533.930329252443,-49.5221601717598)) ;
#67607=CARTESIAN_POINT('Ctrl Pts',(178.962939518692,533.921833878502,-49.5221601717598)) ;
#67608=CARTESIAN_POINT('Ctrl Pts',(179.025745012568,533.880275909628,-49.5221601717594)) ;
#67609=CARTESIAN_POINT('Ctrl Pts',(179.090718120166,533.842384191777,-49.5221601717596)) ;
#67610=CARTESIAN_POINT('Ctrl Pts',(179.157597555806,533.808435017296,-49.5221601717596)) ;
#67611=CARTESIAN_POINT('Ctrl Pts',(179.211636829747,533.781003734088,-49.5221601717595)) ;
#67612=CARTESIAN_POINT('Ctrl Pts',(179.266921689961,533.756146738752,-49.5221601717597)) ;
#67613=CARTESIAN_POINT('Ctrl Pts',(179.323331161757,533.734028136155,-49.5221601717596)) ;
#67614=CARTESIAN_POINT('Ctrl Pts',(179.333816071531,533.729916919631,-49.5221601717596)) ;
#67615=CARTESIAN_POINT('Ctrl Pts',(179.344339870159,533.725900363626,-49.5221601717973)) ;
#67616=CARTESIAN_POINT('Ctrl Pts',(179.354901398821,533.721978117668,-49.5221601717672)) ;
#67617=CARTESIAN_POINT('Ctrl Pts',(179.941713456053,537.375715984761,-47.5212802703069)) ;
#67618=CARTESIAN_POINT('Ctrl Pts',(179.949414502833,537.375470009103,-47.5215735707912)) ;
#67619=CARTESIAN_POINT('Ctrl Pts',(179.957113843187,537.375170608489,-47.5218668712755)) ;
#67620=CARTESIAN_POINT('Ctrl Pts',(179.964810736065,537.374817811737,-47.5221601717598)) ;
#67621=CARTESIAN_POINT('Ctrl Pts',(30.4192289578182,533.719780492321,-49.5190019961068)) ;
#67622=CARTESIAN_POINT('Ctrl Pts',(31.0820274042068,533.896441620623,-49.4819110709933)) ;
#67623=CARTESIAN_POINT('Ctrl Pts',(32.2049962015177,534.964137330925,-49.4077460639272)) ;
#67624=CARTESIAN_POINT('Ctrl Pts',(31.7732154512908,537.256615082637,-49.2965069749086)) ;
#67625=CARTESIAN_POINT('Ctrl Pts',(29.6099672236945,538.131053118425,-49.1852847290511)) ;
#67626=CARTESIAN_POINT('Ctrl Pts',(27.7035979429832,536.788246892714,-49.0740624831937)) ;
#67627=CARTESIAN_POINT('Ctrl Pts',(27.7990747419387,534.457523563324,-48.9628402373363)) ;
#67628=CARTESIAN_POINT('Ctrl Pts',(29.8100295710541,533.275586941982,-48.851617991479)) ;
#67629=CARTESIAN_POINT('Ctrl Pts',(31.8927661072245,534.32548376863,-48.7403957456217)) ;
#67630=CARTESIAN_POINT('Ctrl Pts',(32.1385149627165,536.644977564754,-48.6291734997644)) ;
#67631=CARTESIAN_POINT('Ctrl Pts',(30.3219274024078,538.107999152117,-48.5179512539069)) ;
#67632=CARTESIAN_POINT('Ctrl Pts',(28.1081040068838,537.373579279037,-48.4067290080494)) ;
#67633=CARTESIAN_POINT('Ctrl Pts',(27.5261821604246,535.114873113739,-48.295506762192)) ;
#67634=CARTESIAN_POINT('Ctrl Pts',(29.1095409923539,533.402156751141,-48.1842845163347)) ;
#67635=CARTESIAN_POINT('Ctrl Pts',(31.4069089296102,533.805324868808,-48.0730622704775)) ;
#67636=CARTESIAN_POINT('Ctrl Pts',(32.3125038989418,535.954737015706,-47.9618400246202)) ;
#67637=CARTESIAN_POINT('Ctrl Pts',(30.9963380933565,537.880515059464,-47.8506177787627)) ;
#67638=CARTESIAN_POINT('Ctrl Pts',(28.664524458328,537.817015226414,-47.7393955329052)) ;
#67639=CARTESIAN_POINT('Ctrl Pts',(27.4546872795412,535.823609498753,-47.6281732870478)) ;
#67640=CARTESIAN_POINT('Ctrl Pts',(28.4744419640535,533.724946792159,-47.5169510411904)) ;
#67641=CARTESIAN_POINT('Ctrl Pts',(30.7909517769799,533.450325076242,-47.405714548837)) ;
#67642=CARTESIAN_POINT('Ctrl Pts',(31.7796627542034,534.643320901683,-47.3315521384358)) ;
#67643=CARTESIAN_POINT('Ctrl Pts',(31.9108094354616,535.316555260834,-47.2944638099872)) ;
#67644=CARTESIAN_POINT('Ctrl Pts',(30.3850879802084,533.847851274574,-49.5955259181223)) ;
#67645=CARTESIAN_POINT('Ctrl Pts',(31.005247402468,534.013147472626,-49.5584349930087)) ;
#67646=CARTESIAN_POINT('Ctrl Pts',(32.0559735837837,535.0121563847,-49.4842699859427)) ;
#67647=CARTESIAN_POINT('Ctrl Pts',(31.6519700710076,537.157154891849,-49.3730308969241)) ;
#67648=CARTESIAN_POINT('Ctrl Pts',(29.6278875187022,537.975338745523,-49.2618086510667)) ;
#67649=CARTESIAN_POINT('Ctrl Pts',(27.8441584255201,536.718917675618,-49.1505864052093)) ;
#67650=CARTESIAN_POINT('Ctrl Pts',(27.9334930291271,534.538133998049,-49.0393641593519)) ;
#67651=CARTESIAN_POINT('Ctrl Pts',(29.8150794930204,533.43223349959,-48.9281419134946)) ;
#67652=CARTESIAN_POINT('Ctrl Pts',(31.7638298167847,534.414588562422,-48.8169196676373)) ;
#67653=CARTESIAN_POINT('Ctrl Pts',(31.9937692034465,536.584865122932,-48.70569742178)) ;
#67654=CARTESIAN_POINT('Ctrl Pts',(30.2940460100332,537.95376788261,-48.5944751759224)) ;
#67655=CARTESIAN_POINT('Ctrl Pts',(28.2226418819252,537.266594569717,-48.483252930065)) ;
#67656=CARTESIAN_POINT('Ctrl Pts',(27.678156121485,535.153195061679,-48.3720306842076)) ;
#67657=CARTESIAN_POINT('Ctrl Pts',(29.1596546129031,533.550660843757,-48.2608084383503)) ;
#67658=CARTESIAN_POINT('Ctrl Pts',(31.3092287111068,533.927892426434,-48.149586192493)) ;
#67659=CARTESIAN_POINT('Ctrl Pts',(32.1565651163773,535.939028998164,-48.0383639466357)) ;
#67660=CARTESIAN_POINT('Ctrl Pts',(30.9250706401349,537.740918253523,-47.9271417007783)) ;
#67661=CARTESIAN_POINT('Ctrl Pts',(28.7432667982648,537.681503479708,-47.8159194549208)) ;
#67662=CARTESIAN_POINT('Ctrl Pts',(27.6112606357387,535.816337151797,-47.7046972090634)) ;
#67663=CARTESIAN_POINT('Ctrl Pts',(28.5654126550131,533.85268521699,-47.593474963206)) ;
#67664=CARTESIAN_POINT('Ctrl Pts',(30.7328971973664,533.595730413291,-47.4822384708525)) ;
#67665=CARTESIAN_POINT('Ctrl Pts',(31.6580026072502,534.711978657226,-47.4080760604514)) ;
#67666=CARTESIAN_POINT('Ctrl Pts',(31.7807123850468,535.341902631084,-47.3709877320027)) ;
#67667=CARTESIAN_POINT('Ctrl Pts',(30.3509470025985,533.975922056826,-49.6720498401378)) ;
#67668=CARTESIAN_POINT('Ctrl Pts',(30.9284674007291,534.12985332463,-49.6349589150241)) ;
#67669=CARTESIAN_POINT('Ctrl Pts',(31.9069509660495,535.060175438473,-49.5607939079581)) ;
#67670=CARTESIAN_POINT('Ctrl Pts',(31.5307246907242,537.057694701061,-49.4495548189396)) ;
#67671=CARTESIAN_POINT('Ctrl Pts',(29.6458078137101,537.819624372623,-49.3383325730821)) ;
#67672=CARTESIAN_POINT('Ctrl Pts',(27.984718908057,536.649588458522,-49.2271103272247)) ;
#67673=CARTESIAN_POINT('Ctrl Pts',(28.0679113163154,534.618744432776,-49.1158880813673)) ;
#67674=CARTESIAN_POINT('Ctrl Pts',(29.8201294149866,533.5888800572,-49.00466583551)) ;
#67675=CARTESIAN_POINT('Ctrl Pts',(31.6348935263451,534.503693356214,-48.8934435896527)) ;
#67676=CARTESIAN_POINT('Ctrl Pts',(31.8490234441765,536.524752681109,-48.7822213437953)) ;
#67677=CARTESIAN_POINT('Ctrl Pts',(30.2661646176585,537.799536613104,-48.6709990979379)) ;
#67678=CARTESIAN_POINT('Ctrl Pts',(28.3371797569666,537.159609860397,-48.5597768520804)) ;
#67679=CARTESIAN_POINT('Ctrl Pts',(27.8301300825456,535.191517009621,-48.448554606223)) ;
#67680=CARTESIAN_POINT('Ctrl Pts',(29.2097682334523,533.699164936375,-48.3373323603657)) ;
#67681=CARTESIAN_POINT('Ctrl Pts',(31.2115484926033,534.050459984059,-48.2261101145084)) ;
#67682=CARTESIAN_POINT('Ctrl Pts',(32.000626333813,535.92332098062,-48.1148878686511)) ;
#67683=CARTESIAN_POINT('Ctrl Pts',(30.8538031869134,537.601321447584,-48.0036656227937)) ;
#67684=CARTESIAN_POINT('Ctrl Pts',(28.8220091382015,537.545991733002,-47.8924433769362)) ;
#67685=CARTESIAN_POINT('Ctrl Pts',(27.7678339919361,535.809064804842,-47.7812211310788)) ;
#67686=CARTESIAN_POINT('Ctrl Pts',(28.6563833459727,533.980423641819,-47.6699988852214)) ;
#67687=CARTESIAN_POINT('Ctrl Pts',(30.674842617753,533.741135750339,-47.558762392868)) ;
#67688=CARTESIAN_POINT('Ctrl Pts',(31.536342460297,534.780636412768,-47.4845999824669)) ;
#67689=CARTESIAN_POINT('Ctrl Pts',(31.6506153346321,535.367250001332,-47.4475116540181)) ;
#67690=CARTESIAN_POINT('Ctrl Pts',(30.3168060249887,534.103992839079,-49.7485737621533)) ;
#67691=CARTESIAN_POINT('Ctrl Pts',(30.8516873989902,534.246559176633,-49.7114828370396)) ;
#67692=CARTESIAN_POINT('Ctrl Pts',(31.7579283483155,535.108194492247,-49.6373178299737)) ;
#67693=CARTESIAN_POINT('Ctrl Pts',(31.4094793104411,536.958234510272,-49.5260787409551)) ;
#67694=CARTESIAN_POINT('Ctrl Pts',(29.663728108718,537.663909999721,-49.4148564950976)) ;
#67695=CARTESIAN_POINT('Ctrl Pts',(28.1252793905938,536.580259241425,-49.3036342492401)) ;
#67696=CARTESIAN_POINT('Ctrl Pts',(28.2023296035037,534.699354867503,-49.1924120033828)) ;
#67697=CARTESIAN_POINT('Ctrl Pts',(29.825179336953,533.74552661481,-49.0811897575255)) ;
#67698=CARTESIAN_POINT('Ctrl Pts',(31.5059572359054,534.592798150006,-48.9699675116682)) ;
#67699=CARTESIAN_POINT('Ctrl Pts',(31.7042776849064,536.464640239286,-48.8587452658108)) ;
#67700=CARTESIAN_POINT('Ctrl Pts',(30.238283225284,537.645305343598,-48.7475230199534)) ;
#67701=CARTESIAN_POINT('Ctrl Pts',(28.451717632008,537.052625151078,-48.6363007740959)) ;
#67702=CARTESIAN_POINT('Ctrl Pts',(27.9821040436063,535.229838957562,-48.5250785282385)) ;
#67703=CARTESIAN_POINT('Ctrl Pts',(29.2598818540015,533.847669028992,-48.4138562823812)) ;
#67704=CARTESIAN_POINT('Ctrl Pts',(31.1138682740999,534.173027541684,-48.3026340365239)) ;
#67705=CARTESIAN_POINT('Ctrl Pts',(31.8446875512484,535.907612963078,-48.1914117906666)) ;
#67706=CARTESIAN_POINT('Ctrl Pts',(30.782535733692,537.461724641643,-48.0801895448092)) ;
#67707=CARTESIAN_POINT('Ctrl Pts',(28.9007514781382,537.410479986295,-47.9689672989517)) ;
#67708=CARTESIAN_POINT('Ctrl Pts',(27.9244073481337,535.801792457886,-47.8577450530943)) ;
#67709=CARTESIAN_POINT('Ctrl Pts',(28.7473540369323,534.108162066649,-47.7465228072369)) ;
#67710=CARTESIAN_POINT('Ctrl Pts',(30.6167880381395,533.886541087388,-47.6352863148834)) ;
#67711=CARTESIAN_POINT('Ctrl Pts',(31.4146823133438,534.84929416831,-47.5611239044823)) ;
#67712=CARTESIAN_POINT('Ctrl Pts',(31.5205182842175,535.392597371584,-47.5240355760335)) ;
#67713=CARTESIAN_POINT('Ctrl Pts',(31.5236569526584,535.391334705934,-47.522160171753)) ;
#67714=CARTESIAN_POINT('Ctrl Pts',(31.5186994705276,535.327491770809,-47.522160171753)) ;
#67715=CARTESIAN_POINT('Ctrl Pts',(31.5097667931575,535.264218142824,-47.522160171753)) ;
#67716=CARTESIAN_POINT('Ctrl Pts',(31.4971597796669,535.201749103154,-47.522160171753)) ;
#67717=CARTESIAN_POINT('Ctrl Pts',(31.4845527661763,535.139280063483,-47.522160171753)) ;
#67718=CARTESIAN_POINT('Ctrl Pts',(31.468271074477,535.077614831876,-47.522160171753)) ;
#67719=CARTESIAN_POINT('Ctrl Pts',(31.4485600751653,535.016978328503,-47.522160171753)) ;
#67720=CARTESIAN_POINT('Ctrl Pts',(31.4307419234247,534.962164749493,-47.522160171753)) ;
#67721=CARTESIAN_POINT('Ctrl Pts',(31.4101205948598,534.908191257982,-47.5221601717531)) ;
#67722=CARTESIAN_POINT('Ctrl Pts',(31.386841891083,534.855224799164,-47.522160171753)) ;
#67723=CARTESIAN_POINT('Ctrl Pts',(31.375142881693,534.828605829954,-47.5221601717529)) ;
#67724=CARTESIAN_POINT('Ctrl Pts',(31.3627721928826,534.802241266862,-47.522160171753)) ;
#67725=CARTESIAN_POINT('Ctrl Pts',(31.3497453957004,534.776152991293,-47.522160171753)) ;
#67726=CARTESIAN_POINT('Ctrl Pts',(31.3438540878375,534.764354691155,-47.5221601717529)) ;
#67727=CARTESIAN_POINT('Ctrl Pts',(31.337827729337,534.752611584923,-47.522160171753)) ;
#67728=CARTESIAN_POINT('Ctrl Pts',(31.3316778572707,534.740944357343,-47.522160171753)) ;
#67729=CARTESIAN_POINT('Ctrl Pts',(31.3004561004906,534.68171201269,-47.5221601717531)) ;
#67730=CARTESIAN_POINT('Ctrl Pts',(31.2660015749929,534.624325135799,-47.5221601717529)) ;
#67731=CARTESIAN_POINT('Ctrl Pts',(31.2285820548354,534.569024272131,-47.522160171753)) ;
#67732=CARTESIAN_POINT('Ctrl Pts',(31.1904826176123,534.51271858529,-47.5221601717531)) ;
#67733=CARTESIAN_POINT('Ctrl Pts',(31.1493091452131,534.458574448788,-47.5221601717529)) ;
#67734=CARTESIAN_POINT('Ctrl Pts',(31.1052911573092,534.406853723098,-47.522160171753)) ;
#67735=CARTESIAN_POINT('Ctrl Pts',(31.0683720694782,534.363474138857,-47.5221601717531)) ;
#67736=CARTESIAN_POINT('Ctrl Pts',(31.0294508873193,534.321799175608,-47.5221601717531)) ;
#67737=CARTESIAN_POINT('Ctrl Pts',(30.9886377240086,534.281995176134,-47.5221601717531)) ;
#67738=CARTESIAN_POINT('Ctrl Pts',(30.9697790441985,534.263602804155,-47.5221601717531)) ;
#67739=CARTESIAN_POINT('Ctrl Pts',(30.9505161023597,534.245610099233,-47.5221601717531)) ;
#67740=CARTESIAN_POINT('Ctrl Pts',(30.9308582982733,534.228034654789,-47.5221601717529)) ;
#67741=CARTESIAN_POINT('Ctrl Pts',(30.9223934077021,534.220466453717,-47.5221601717529)) ;
#67742=CARTESIAN_POINT('Ctrl Pts',(30.9138556834697,534.212976101739,-47.5221601717529)) ;
#67743=CARTESIAN_POINT('Ctrl Pts',(30.9052562285359,534.205573628438,-47.5221601717529)) ;
#67744=CARTESIAN_POINT('Ctrl Pts',(30.8520268008585,534.159753350261,-47.5221601717529)) ;
#67745=CARTESIAN_POINT('Ctrl Pts',(30.7963374348611,534.117209332328,-47.5221601717531)) ;
#67746=CARTESIAN_POINT('Ctrl Pts',(30.7384395986102,534.078208963547,-47.522160171753)) ;
#67747=CARTESIAN_POINT('Ctrl Pts',(30.6863848595582,534.043144544024,-47.5221601717529)) ;
#67748=CARTESIAN_POINT('Ctrl Pts',(30.6325439543738,534.010944257277,-47.522160171753)) ;
#67749=CARTESIAN_POINT('Ctrl Pts',(30.5770689192711,533.981821161704,-47.5221601717529)) ;
#67750=CARTESIAN_POINT('Ctrl Pts',(30.5169372524336,533.950253443414,-47.5221601717529)) ;
#67751=CARTESIAN_POINT('Ctrl Pts',(30.4548855870198,533.922299856533,-47.522160171753)) ;
#67752=CARTESIAN_POINT('Ctrl Pts',(30.3912320560275,533.897901819146,-47.5221601717529)) ;
#67753=CARTESIAN_POINT('Ctrl Pts',(30.3669330318675,533.88858814101,-47.5221601717528)) ;
#67754=CARTESIAN_POINT('Ctrl Pts',(30.3424002759375,533.879793049169,-47.5221601717531)) ;
#67755=CARTESIAN_POINT('Ctrl Pts',(30.3176505254538,533.871514996581,-47.522160171753)) ;
#67756=CARTESIAN_POINT('Ctrl Pts',(30.3067503928447,533.867869227667,-47.522160171753)) ;
#67757=CARTESIAN_POINT('Ctrl Pts',(30.2958091142617,533.864324160259,-47.5221601717527)) ;
#67758=CARTESIAN_POINT('Ctrl Pts',(30.2848404431185,533.86088328274,-47.5221601717527)) ;
#67759=CARTESIAN_POINT('Ctrl Pts',(30.2180806724344,533.839940709925,-47.5221601717528)) ;
#67760=CARTESIAN_POINT('Ctrl Pts',(30.1501904337754,533.822814034984,-47.5221601717527)) ;
#67761=CARTESIAN_POINT('Ctrl Pts',(30.081533941393,533.809394915133,-47.5221601717529)) ;
#67762=CARTESIAN_POINT('Ctrl Pts',(30.0113036312589,533.795668187825,-47.522160171753)) ;
#67763=CARTESIAN_POINT('Ctrl Pts',(29.940270706767,533.785820668202,-47.5221601717528)) ;
#67764=CARTESIAN_POINT('Ctrl Pts',(29.8687930800881,533.779782670237,-47.5221601717529)) ;
#67765=CARTESIAN_POINT('Ctrl Pts',(29.8147780369742,533.775219805806,-47.522160171753)) ;
#67766=CARTESIAN_POINT('Ctrl Pts',(29.7605082709567,533.772833387046,-47.5221601717526)) ;
#67767=CARTESIAN_POINT('Ctrl Pts',(29.7061311783795,533.772611627013,-47.5221601717528)) ;
#67768=CARTESIAN_POINT('Ctrl Pts',(29.6724350241176,533.772474207745,-47.522160171753)) ;
#67769=CARTESIAN_POINT('Ctrl Pts',(29.6386975577268,533.773168325095,-47.5221601717526)) ;
#67770=CARTESIAN_POINT('Ctrl Pts',(29.604953389941,533.774694287495,-47.522160171753)) ;
#67771=CARTESIAN_POINT('Ctrl Pts',(29.5920528858034,533.77527766784,-47.5221601717531)) ;
#67772=CARTESIAN_POINT('Ctrl Pts',(29.5791491157432,533.775982802408,-47.5221601717528)) ;
#67773=CARTESIAN_POINT('Ctrl Pts',(29.5662514687581,533.77680931295,-47.5221601717528)) ;
#67774=CARTESIAN_POINT('Ctrl Pts',(29.4896818934395,533.781716065419,-47.522160171753)) ;
#67775=CARTESIAN_POINT('Ctrl Pts',(29.413514639897,533.79088260525,-47.5221601717528)) ;
#67776=CARTESIAN_POINT('Ctrl Pts',(29.3381633346069,533.804241013433,-47.5221601717528)) ;
#67777=CARTESIAN_POINT('Ctrl Pts',(29.2816498556393,533.81425981957,-47.5221601717527)) ;
#67778=CARTESIAN_POINT('Ctrl Pts',(29.225594680158,533.826637686017,-47.5221601717529)) ;
#67779=CARTESIAN_POINT('Ctrl Pts',(29.1701689140933,533.8413670658,-47.5221601717527)) ;
#67780=CARTESIAN_POINT('Ctrl Pts',(29.1504944696968,533.846595543169,-47.5221601717526)) ;
#67781=CARTESIAN_POINT('Ctrl Pts',(29.1308993321089,533.852120486841,-47.5221601717527)) ;
#67782=CARTESIAN_POINT('Ctrl Pts',(29.1113911916752,533.857942117771,-47.5221601717528)) ;
#67783=CARTESIAN_POINT('Ctrl Pts',(29.0966180285685,533.862350733936,-47.5221601717529)) ;
#67784=CARTESIAN_POINT('Ctrl Pts',(29.0818996663657,533.86692809925,-47.5221601717528)) ;
#67785=CARTESIAN_POINT('Ctrl Pts',(29.0672469809268,533.871671421633,-47.5221601717528)) ;
#67786=CARTESIAN_POINT('Ctrl Pts',(28.9955972326579,533.894865658355,-47.522160171753)) ;
#67787=CARTESIAN_POINT('Ctrl Pts',(28.9254624202921,533.92204042568,-47.5221601717529)) ;
#67788=CARTESIAN_POINT('Ctrl Pts',(28.8572215630825,533.953163710321,-47.5221601717529)) ;
#67789=CARTESIAN_POINT('Ctrl Pts',(28.8020993751403,533.978303833343,-47.522160171753)) ;
#67790=CARTESIAN_POINT('Ctrl Pts',(28.7482125513535,534.00602120663,-47.5221601717529)) ;
#67791=CARTESIAN_POINT('Ctrl Pts',(28.6957646816156,534.036323556823,-47.5221601717531)) ;
#67792=CARTESIAN_POINT('Ctrl Pts',(28.6854183011059,534.042301295232,-47.5221601717531)) ;
#67793=CARTESIAN_POINT('Ctrl Pts',(28.6751279406135,534.048379698197,-47.5221601717528)) ;
#67794=CARTESIAN_POINT('Ctrl Pts',(28.6648941356016,534.054557422396,-47.5221601717531)) ;
#67795=CARTESIAN_POINT('',(31.1586577691864,536.791421537165,-49.5230216451333)) ;
#67796=CARTESIAN_POINT('Ctrl Pts',(31.1573042373964,536.790269707588,-49.5230216451333)) ;
#67797=CARTESIAN_POINT('Ctrl Pts',(31.1524161449685,536.796013776525,-49.5227344873399)) ;
#67798=CARTESIAN_POINT('Ctrl Pts',(31.1474890446894,536.801724650524,-49.5224473295465)) ;
#67799=CARTESIAN_POINT('Ctrl Pts',(31.1425233909828,536.807401802874,-49.5221601717531)) ;
#67800=CARTESIAN_POINT('Ctrl Pts',(30.4186978425951,533.72539083489,-49.5221601717531)) ;
#67801=CARTESIAN_POINT('Ctrl Pts',(30.4873018263811,533.750792346629,-49.522160171753)) ;
#67802=CARTESIAN_POINT('Ctrl Pts',(30.554203302766,533.780093658899,-49.5221601717531)) ;
#67803=CARTESIAN_POINT('Ctrl Pts',(30.6192143952837,533.812998021653,-49.5221601717532)) ;
#67804=CARTESIAN_POINT('Ctrl Pts',(30.6860861306996,533.84684412014,-49.5221601717532)) ;
#67805=CARTESIAN_POINT('Ctrl Pts',(30.7509584997066,533.884503151209,-49.5221601717529)) ;
#67806=CARTESIAN_POINT('Ctrl Pts',(30.8135958271794,533.925696927834,-49.522160171753)) ;
#67807=CARTESIAN_POINT('Ctrl Pts',(30.8665864966189,533.960546527715,-49.5221601717532)) ;
#67808=CARTESIAN_POINT('Ctrl Pts',(30.9179772112377,533.997927008956,-49.5221601717531)) ;
#67809=CARTESIAN_POINT('Ctrl Pts',(30.9676024509393,534.037688046095,-49.522160171753)) ;
#67810=CARTESIAN_POINT('Ctrl Pts',(30.9896090562751,534.055320312606,-49.522160171753)) ;
#67811=CARTESIAN_POINT('Ctrl Pts',(31.0112681718102,534.073420901991,-49.5221601717529)) ;
#67812=CARTESIAN_POINT('Ctrl Pts',(31.0325638136025,534.091977425642,-49.522160171753)) ;
#67813=CARTESIAN_POINT('Ctrl Pts',(31.0442342273179,534.102146750908,-49.5221601717531)) ;
#67814=CARTESIAN_POINT('Ctrl Pts',(31.0557954633371,534.112453011021,-49.5221601717531)) ;
#67815=CARTESIAN_POINT('Ctrl Pts',(31.0672447584333,534.122894207908,-49.5221601717531)) ;
#67816=CARTESIAN_POINT('Ctrl Pts',(31.0778839828076,534.132596659935,-49.5221601717531)) ;
#67817=CARTESIAN_POINT('Ctrl Pts',(31.0884280589244,534.142417222811,-49.5221601717532)) ;
#67818=CARTESIAN_POINT('Ctrl Pts',(31.0988586971619,534.152338637124,-49.5221601717532)) ;
#67819=CARTESIAN_POINT('Ctrl Pts',(31.1519351779608,534.202823923289,-49.5221601717531)) ;
#67820=CARTESIAN_POINT('Ctrl Pts',(31.2021716876196,534.256001695126,-49.5221601717531)) ;
#67821=CARTESIAN_POINT('Ctrl Pts',(31.2493501345782,534.311609028577,-49.5221601717531)) ;
#67822=CARTESIAN_POINT('Ctrl Pts',(31.2961737783185,534.366798169778,-49.5221601717531)) ;
#67823=CARTESIAN_POINT('Ctrl Pts',(31.3399856917906,534.424381358109,-49.5221601717529)) ;
#67824=CARTESIAN_POINT('Ctrl Pts',(31.3805278530913,534.484125791624,-49.5221601717529)) ;
#67825=CARTESIAN_POINT('Ctrl Pts',(31.4142815272287,534.533866458518,-49.5221601717529)) ;
#67826=CARTESIAN_POINT('Ctrl Pts',(31.4457681286474,534.585105851876,-49.5221601717531)) ;
#67827=CARTESIAN_POINT('Ctrl Pts',(31.4748109615605,534.63771607303,-49.522160171753)) ;
#67828=CARTESIAN_POINT('Ctrl Pts',(31.4868723497301,534.659564916114,-49.522160171753)) ;
#67829=CARTESIAN_POINT('Ctrl Pts',(31.498511936526,534.681650225412,-49.522160171753)) ;
#67830=CARTESIAN_POINT('Ctrl Pts',(31.5097156382178,534.703962916598,-49.522160171753)) ;
#67831=CARTESIAN_POINT('Ctrl Pts',(31.5149427851672,534.714373022015,-49.522160171753)) ;
#67832=CARTESIAN_POINT('Ctrl Pts',(31.5200750389261,534.724832622436,-49.5221601717529)) ;
#67833=CARTESIAN_POINT('Ctrl Pts',(31.5251109030024,534.735340792977,-49.522160171753)) ;
#67834=CARTESIAN_POINT('Ctrl Pts',(31.5303022079443,534.746173316816,-49.522160171753)) ;
#67835=CARTESIAN_POINT('Ctrl Pts',(31.5353873889545,534.757049810725,-49.5221601717531)) ;
#67836=CARTESIAN_POINT('Ctrl Pts',(31.5403636460063,534.767965454351,-49.5221601717531)) ;
#67837=CARTESIAN_POINT('Ctrl Pts',(31.5689045556854,534.830571223217,-49.522160171753)) ;
#67838=CARTESIAN_POINT('Ctrl Pts',(31.5938849702325,534.894502684949,-49.522160171753)) ;
#67839=CARTESIAN_POINT('Ctrl Pts',(31.6150817999401,534.959552218106,-49.5221601717531)) ;
#67840=CARTESIAN_POINT('Ctrl Pts',(31.6344288124596,535.018924971001,-49.5221601717531)) ;
#67841=CARTESIAN_POINT('Ctrl Pts',(31.6506235210653,535.079229774877,-49.5221601717531)) ;
#67842=CARTESIAN_POINT('Ctrl Pts',(31.6634586243526,535.140313572021,-49.5221601717531)) ;
#67843=CARTESIAN_POINT('Ctrl Pts',(31.6785443557651,535.212108378556,-49.522160171753)) ;
#67844=CARTESIAN_POINT('Ctrl Pts',(31.6889895128008,535.284980843413,-49.5221601717531)) ;
#67845=CARTESIAN_POINT('Ctrl Pts',(31.6948691143251,535.358509502156,-49.5221601717531)) ;
#67846=CARTESIAN_POINT('Ctrl Pts',(31.6961734172464,535.374820751141,-49.5221601717531)) ;
#67847=CARTESIAN_POINT('Ctrl Pts',(31.6972528175616,535.391164207973,-49.5221601717531)) ;
#67848=CARTESIAN_POINT('Ctrl Pts',(31.6981077549656,535.407535101245,-49.5221601717531)) ;
#67849=CARTESIAN_POINT('Ctrl Pts',(31.6989446641061,535.423560777691,-49.5221601717531)) ;
#67850=CARTESIAN_POINT('Ctrl Pts',(31.6995664742495,535.439618043232,-49.522160171753)) ;
#67851=CARTESIAN_POINT('Ctrl Pts',(31.6999730977482,535.455671178293,-49.522160171753)) ;
#67852=CARTESIAN_POINT('Ctrl Pts',(31.7017092506482,535.524212954849,-49.5221601717531)) ;
#67853=CARTESIAN_POINT('Ctrl Pts',(31.6995342482065,535.592773413081,-49.5221601717531)) ;
#67854=CARTESIAN_POINT('Ctrl Pts',(31.6935688364705,535.66101662413,-49.522160171753)) ;
#67855=CARTESIAN_POINT('Ctrl Pts',(31.6876125268821,535.729155708289,-49.522160171753)) ;
#67856=CARTESIAN_POINT('Ctrl Pts',(31.6778769035789,535.796979569927,-49.5221601717531)) ;
#67857=CARTESIAN_POINT('Ctrl Pts',(31.6644327909043,535.864138816221,-49.5221601717531)) ;
#67858=CARTESIAN_POINT('Ctrl Pts',(31.65457150191,535.913400284968,-49.5221601717531)) ;
#67859=CARTESIAN_POINT('Ctrl Pts',(31.6427139028012,535.962303925143,-49.522160171753)) ;
#67860=CARTESIAN_POINT('Ctrl Pts',(31.6288731470677,536.010701797538,-49.522160171753)) ;
#67861=CARTESIAN_POINT('Ctrl Pts',(31.6231607179449,536.030676820657,-49.522160171753)) ;
#67862=CARTESIAN_POINT('Ctrl Pts',(31.6171103358191,536.050565567194,-49.5221601717531)) ;
#67863=CARTESIAN_POINT('Ctrl Pts',(31.6107223668049,536.070357063039,-49.522160171753)) ;
#67864=CARTESIAN_POINT('Ctrl Pts',(31.605982706735,536.085041693219,-49.522160171753)) ;
#67865=CARTESIAN_POINT('Ctrl Pts',(31.6010571935044,536.099672778431,-49.5221601717531)) ;
#67866=CARTESIAN_POINT('Ctrl Pts',(31.5959458683123,536.114245698436,-49.5221601717531)) ;
#67867=CARTESIAN_POINT('Ctrl Pts',(31.5916425233631,536.12651498269,-49.5221601717531)) ;
#67868=CARTESIAN_POINT('Ctrl Pts',(31.5872102325381,536.138735072304,-49.5221601717531)) ;
#67869=CARTESIAN_POINT('Ctrl Pts',(31.5826507943598,536.150900029629,-49.5221601717531)) ;
#67870=CARTESIAN_POINT('Ctrl Pts',(31.5595404376064,536.212560368616,-49.5221601717531)) ;
#67871=CARTESIAN_POINT('Ctrl Pts',(31.5331563054528,536.272836005059,-49.5221601717531)) ;
#67872=CARTESIAN_POINT('Ctrl Pts',(31.5035486090204,536.331394754774,-49.5221601717531)) ;
#67873=CARTESIAN_POINT('Ctrl Pts',(31.4825856728236,536.372855708579,-49.5221601717531)) ;
#67874=CARTESIAN_POINT('Ctrl Pts',(31.4600059155797,536.413455468647,-49.5221601717531)) ;
#67875=CARTESIAN_POINT('Ctrl Pts',(31.4358165118334,536.453064537015,-49.5221601717531)) ;
#67876=CARTESIAN_POINT('Ctrl Pts',(31.4280894921966,536.465717186592,-49.5221601717531)) ;
#67877=CARTESIAN_POINT('Ctrl Pts',(31.4201969312163,536.478270552164,-49.5221601717531)) ;
#67878=CARTESIAN_POINT('Ctrl Pts',(31.4121428522646,536.490714068894,-49.5221601717531)) ;
#67879=CARTESIAN_POINT('Ctrl Pts',(31.3778791836545,536.543651286935,-49.5221601717531)) ;
#67880=CARTESIAN_POINT('Ctrl Pts',(31.3407594282531,536.594505707453,-49.5221601717532)) ;
#67881=CARTESIAN_POINT('Ctrl Pts',(31.300817835818,536.64296371139,-49.5221601717531)) ;
#67882=CARTESIAN_POINT('Ctrl Pts',(31.2636079488606,536.68810755115,-49.5221601717531)) ;
#67883=CARTESIAN_POINT('Ctrl Pts',(31.2239484452003,536.731171720598,-49.5221601717532)) ;
#67884=CARTESIAN_POINT('Ctrl Pts',(31.1818447665004,536.771868473735,-49.522160171753)) ;
#67885=CARTESIAN_POINT('Ctrl Pts',(31.1746559175354,536.778817101995,-49.522160171753)) ;
#67886=CARTESIAN_POINT('Ctrl Pts',(31.1673957685906,536.785696624249,-49.522160171753)) ;
#67887=CARTESIAN_POINT('Ctrl Pts',(31.1600655534529,536.792506522884,-49.5221601717531)) ;
#67888=CARTESIAN_POINT('Ctrl Pts',(28.6224008556909,536.788257168284,-49.5202847734518)) ;
#67889=CARTESIAN_POINT('Ctrl Pts',(28.2636169540964,536.366767265057,-49.4831964450485)) ;
#67890=CARTESIAN_POINT('Ctrl Pts',(28.0083851733653,535.142681732903,-49.4090340346928)) ;
#67891=CARTESIAN_POINT('Ctrl Pts',(29.3472284941806,533.81927777062,-49.2977975423846)) ;
#67892=CARTESIAN_POINT('Ctrl Pts',(31.1844609256909,534.231833414637,-49.1865752965273)) ;
#67893=CARTESIAN_POINT('Ctrl Pts',(31.8334428866778,535.998170240813,-49.07535305067)) ;
#67894=CARTESIAN_POINT('Ctrl Pts',(30.7002342883442,537.501358927502,-48.9641308048125)) ;
#67895=CARTESIAN_POINT('Ctrl Pts',(28.8229400342555,537.362809870203,-48.8529085589551)) ;
#67896=CARTESIAN_POINT('Ctrl Pts',(27.922444913608,535.709936033526,-48.7416863130977)) ;
#67897=CARTESIAN_POINT('Ctrl Pts',(28.8240110099946,534.0575733704,-48.6304640672403)) ;
#67898=CARTESIAN_POINT('Ctrl Pts',(30.7013164038052,533.92033530544,-48.519241821383)) ;
#67899=CARTESIAN_POINT('Ctrl Pts',(31.8336287497696,535.423982591803,-48.4080195755257)) ;
#67900=CARTESIAN_POINT('Ctrl Pts',(31.1830993569614,537.190305869038,-48.2967973296683)) ;
#67901=CARTESIAN_POINT('Ctrl Pts',(29.3459856170836,537.600333837421,-48.1855750838108)) ;
#67902=CARTESIAN_POINT('Ctrl Pts',(28.0061713207052,536.278206215794,-48.0743528379535)) ;
#67903=CARTESIAN_POINT('Ctrl Pts',(28.3916956359744,534.435855981822,-47.9631305920961)) ;
#67904=CARTESIAN_POINT('Ctrl Pts',(30.1492588407991,533.761763155306,-47.8519083462388)) ;
#67905=CARTESIAN_POINT('Ctrl Pts',(31.6678491066124,534.874247564052,-47.7406861003814)) ;
#67906=CARTESIAN_POINT('Ctrl Pts',(31.5558742796478,536.752700386808,-47.6294638545241)) ;
#67907=CARTESIAN_POINT('Ctrl Pts',(29.9156968899049,537.677602163744,-47.5182416086666)) ;
#67908=CARTESIAN_POINT('Ctrl Pts',(28.2520400432131,536.796558566173,-47.4070036656182)) ;
#67909=CARTESIAN_POINT('Ctrl Pts',(28.1434047061733,535.55083948989,-47.3328398045222)) ;
#67910=CARTESIAN_POINT('Ctrl Pts',(28.3654110025038,535.043772234511,-47.2957500253787)) ;
#67911=CARTESIAN_POINT('Ctrl Pts',(28.52086835799,536.874678815716,-49.5972643150057)) ;
#67912=CARTESIAN_POINT('Ctrl Pts',(28.1333130675147,536.419389040585,-49.5601759866023)) ;
#67913=CARTESIAN_POINT('Ctrl Pts',(27.8576138890395,535.097142357075,-49.4860135762466)) ;
#67914=CARTESIAN_POINT('Ctrl Pts',(29.3038209507092,533.667612757949,-49.3747770839385)) ;
#67915=CARTESIAN_POINT('Ctrl Pts',(31.2883836512653,534.113251822979,-49.2635548380812)) ;
#67916=CARTESIAN_POINT('Ctrl Pts',(31.9894083942532,536.021233699266,-49.1523325922239)) ;
#67917=CARTESIAN_POINT('Ctrl Pts',(30.7653261945102,537.644965214308,-49.0411103463664)) ;
#67918=CARTESIAN_POINT('Ctrl Pts',(28.7374890571207,537.495305712007,-48.929888100509)) ;
#67919=CARTESIAN_POINT('Ctrl Pts',(27.764781958215,535.709885582938,-48.8186658546515)) ;
#67920=CARTESIAN_POINT('Ctrl Pts',(28.7386459159201,533.925017619152,-48.7074436087942)) ;
#67921=CARTESIAN_POINT('Ctrl Pts',(30.7664950863416,533.77677423952,-48.5962213629369)) ;
#67922=CARTESIAN_POINT('Ctrl Pts',(31.9896091619694,535.401001129993,-48.4849991170796)) ;
#67923=CARTESIAN_POINT('Ctrl Pts',(31.2869128964124,537.308968370831,-48.3737768712222)) ;
#67924=CARTESIAN_POINT('Ctrl Pts',(29.3024784055384,537.75187706234,-48.2625546253647)) ;
#67925=CARTESIAN_POINT('Ctrl Pts',(27.8552225044011,536.323726155436,-48.1513323795073)) ;
#67926=CARTESIAN_POINT('Ctrl Pts',(28.2716625601711,534.333635248594,-48.04011013365)) ;
#67927=CARTESIAN_POINT('Ctrl Pts',(30.1701672459924,533.60548596423,-47.9288878877926)) ;
#67928=CARTESIAN_POINT('Ctrl Pts',(31.810535414588,534.80718207229,-47.8176656419354)) ;
#67929=CARTESIAN_POINT('Ctrl Pts',(31.6895811677632,536.836270685608,-47.706443396078)) ;
#67930=CARTESIAN_POINT('Ctrl Pts',(29.9178756316795,537.835341645114,-47.5952211502205)) ;
#67931=CARTESIAN_POINT('Ctrl Pts',(28.120807787762,536.883645914451,-47.4839832071721)) ;
#67932=CARTESIAN_POINT('Ctrl Pts',(28.0034608292857,535.538030862288,-47.409819346076)) ;
#67933=CARTESIAN_POINT('Ctrl Pts',(28.24327012474,534.990301166012,-47.3727295669326)) ;
#67934=CARTESIAN_POINT('Ctrl Pts',(28.419335860289,536.961100463147,-49.6742438565595)) ;
#67935=CARTESIAN_POINT('Ctrl Pts',(28.0030091809332,536.472010816113,-49.6371555281562)) ;
#67936=CARTESIAN_POINT('Ctrl Pts',(27.7068426047137,535.051602981246,-49.5629931178004)) ;
#67937=CARTESIAN_POINT('Ctrl Pts',(29.2604134072377,533.515947745279,-49.4517566254923)) ;
#67938=CARTESIAN_POINT('Ctrl Pts',(31.3923063768398,533.994670231322,-49.340534379635)) ;
#67939=CARTESIAN_POINT('Ctrl Pts',(32.1453739018286,536.044297157719,-49.2293121337776)) ;
#67940=CARTESIAN_POINT('Ctrl Pts',(30.8304181006761,537.788571501115,-49.1180898879202)) ;
#67941=CARTESIAN_POINT('Ctrl Pts',(28.652038079986,537.62780155381,-49.0068676420627)) ;
#67942=CARTESIAN_POINT('Ctrl Pts',(27.6071190028218,535.709835132352,-48.8956453962053)) ;
#67943=CARTESIAN_POINT('Ctrl Pts',(28.6532808218456,533.792461867905,-48.784423150348)) ;
#67944=CARTESIAN_POINT('Ctrl Pts',(30.8316737688779,533.633213173601,-48.6732009044907)) ;
#67945=CARTESIAN_POINT('Ctrl Pts',(32.1455895741691,535.378019668185,-48.5619786586334)) ;
#67946=CARTESIAN_POINT('Ctrl Pts',(31.3907264358632,537.427630872625,-48.450756412776)) ;
#67947=CARTESIAN_POINT('Ctrl Pts',(29.2589711939935,537.903420287258,-48.3395341669185)) ;
#67948=CARTESIAN_POINT('Ctrl Pts',(27.704273688097,536.369246095077,-48.2283119210611)) ;
#67949=CARTESIAN_POINT('Ctrl Pts',(28.151629484368,534.231414515366,-48.1170896752037)) ;
#67950=CARTESIAN_POINT('Ctrl Pts',(30.1910756511857,533.449208773154,-48.0058674293464)) ;
#67951=CARTESIAN_POINT('Ctrl Pts',(31.9532217225635,534.740116580527,-47.8946451834892)) ;
#67952=CARTESIAN_POINT('Ctrl Pts',(31.8232880558788,536.919840984407,-47.7834229376318)) ;
#67953=CARTESIAN_POINT('Ctrl Pts',(29.9200543734541,537.993081126484,-47.6722006917743)) ;
#67954=CARTESIAN_POINT('Ctrl Pts',(27.989575532311,536.97073326273,-47.5609627487258)) ;
#67955=CARTESIAN_POINT('Ctrl Pts',(27.8635169523983,535.525222234686,-47.4867988876299)) ;
#67956=CARTESIAN_POINT('Ctrl Pts',(28.1211292469763,534.936830097514,-47.4497091084864)) ;
#67957=CARTESIAN_POINT('Ctrl Pts',(28.3178033625881,537.047522110579,-49.7512233981133)) ;
#67958=CARTESIAN_POINT('Ctrl Pts',(27.8727052943514,536.524632591642,-49.71413506971)) ;
#67959=CARTESIAN_POINT('Ctrl Pts',(27.5560713203878,535.006063605417,-49.6399726593542)) ;
#67960=CARTESIAN_POINT('Ctrl Pts',(29.2170058637665,533.364282732609,-49.5287361670461)) ;
#67961=CARTESIAN_POINT('Ctrl Pts',(31.4962291024142,533.876088639664,-49.4175139211888)) ;
#67962=CARTESIAN_POINT('Ctrl Pts',(32.3013394094041,536.067360616172,-49.3062916753315)) ;
#67963=CARTESIAN_POINT('Ctrl Pts',(30.8955100068421,537.932177787921,-49.195069429474)) ;
#67964=CARTESIAN_POINT('Ctrl Pts',(28.5665871028512,537.760297395612,-49.0838471836165)) ;
#67965=CARTESIAN_POINT('Ctrl Pts',(27.4494560474289,535.709784681764,-48.9726249377591)) ;
#67966=CARTESIAN_POINT('Ctrl Pts',(28.5679157277713,533.659906116657,-48.8614026919018)) ;
#67967=CARTESIAN_POINT('Ctrl Pts',(30.8968524514142,533.489652107681,-48.7501804460445)) ;
#67968=CARTESIAN_POINT('Ctrl Pts',(32.3015699863689,535.355038206375,-48.6389582001872)) ;
#67969=CARTESIAN_POINT('Ctrl Pts',(31.4945399753143,537.546293374418,-48.5277359543298)) ;
#67970=CARTESIAN_POINT('Ctrl Pts',(29.2154639824486,538.054963512177,-48.4165137084723)) ;
#67971=CARTESIAN_POINT('Ctrl Pts',(27.553324871793,536.414766034718,-48.305291462615)) ;
#67972=CARTESIAN_POINT('Ctrl Pts',(28.0315964085647,534.129193782138,-48.1940692167575)) ;
#67973=CARTESIAN_POINT('Ctrl Pts',(30.2119840563792,533.292931582077,-48.0828469709002)) ;
#67974=CARTESIAN_POINT('Ctrl Pts',(32.0959080305391,534.673051088765,-47.971624725043)) ;
#67975=CARTESIAN_POINT('Ctrl Pts',(31.9569949439941,537.003411283205,-47.8604024791856)) ;
#67976=CARTESIAN_POINT('Ctrl Pts',(29.9222331152288,538.150820607853,-47.7491802333281)) ;
#67977=CARTESIAN_POINT('Ctrl Pts',(27.8583432768598,537.057820611007,-47.6379422902796)) ;
#67978=CARTESIAN_POINT('Ctrl Pts',(27.723573075511,535.512413607084,-47.5637784291836)) ;
#67979=CARTESIAN_POINT('Ctrl Pts',(27.9989883692128,534.883359029015,-47.5266886500402)) ;
#67980=CARTESIAN_POINT('',(29.9416619236741,537.377495804614,-47.5212987075501)) ;
#67981=CARTESIAN_POINT('Ctrl Pts',(28.0059001157431,534.88733298046,-47.522160171753)) ;
#67982=CARTESIAN_POINT('Ctrl Pts',(27.9829859323478,534.956807320503,-47.5221601717529)) ;
#67983=CARTESIAN_POINT('Ctrl Pts',(27.9641822315392,535.027382072257,-47.5221601717529)) ;
#67984=CARTESIAN_POINT('Ctrl Pts',(27.9493741439311,535.098725327386,-47.5221601717529)) ;
#67985=CARTESIAN_POINT('Ctrl Pts',(27.934145219614,535.172096113787,-47.5221601717529)) ;
#67986=CARTESIAN_POINT('Ctrl Pts',(27.9231422999915,535.246280738549,-47.5221601717529)) ;
#67987=CARTESIAN_POINT('Ctrl Pts',(27.9162948670505,535.320921706951,-47.5221601717529)) ;
#67988=CARTESIAN_POINT('Ctrl Pts',(27.9104995242757,535.384094285734,-47.5221601717529)) ;
#67989=CARTESIAN_POINT('Ctrl Pts',(27.9076818396783,535.447594149968,-47.5221601717529)) ;
#67990=CARTESIAN_POINT('Ctrl Pts',(27.9078274713952,535.511198010894,-47.5221601717529)) ;
#67991=CARTESIAN_POINT('Ctrl Pts',(27.9078920377234,535.539397003841,-47.5221601717529)) ;
#67992=CARTESIAN_POINT('Ctrl Pts',(27.9085394098575,535.567616312829,-47.5221601717528)) ;
#67993=CARTESIAN_POINT('Ctrl Pts',(27.9097698678232,535.595835716945,-47.5221601717528)) ;
#67994=CARTESIAN_POINT('Ctrl Pts',(27.9104441820957,535.611300484931,-47.5221601717528)) ;
#67995=CARTESIAN_POINT('Ctrl Pts',(27.9112936275329,535.62676527183,-47.5221601717528)) ;
#67996=CARTESIAN_POINT('Ctrl Pts',(27.912318364823,535.642226671488,-47.5221601717528)) ;
#67997=CARTESIAN_POINT('Ctrl Pts',(27.9132705988578,535.656594130466,-47.5221601717529)) ;
#67998=CARTESIAN_POINT('Ctrl Pts',(27.9143744996085,535.670960840443,-47.5221601717528)) ;
#67999=CARTESIAN_POINT('Ctrl Pts',(27.9156279765185,535.685301740957,-47.5221601717528)) ;
#68000=CARTESIAN_POINT('Ctrl Pts',(27.9220008875486,535.758213561142,-47.5221601717528)) ;
#68001=CARTESIAN_POINT('Ctrl Pts',(27.9322429746534,535.830584659191,-47.5221601717528)) ;
#68002=CARTESIAN_POINT('Ctrl Pts',(27.9462848097153,535.902081453107,-47.5221601717528)) ;
#68003=CARTESIAN_POINT('Ctrl Pts',(27.9601366899147,535.97261105409,-47.5221601717528)) ;
#68004=CARTESIAN_POINT('Ctrl Pts',(27.9776866254573,536.042290755737,-47.5221601717529)) ;
#68005=CARTESIAN_POINT('Ctrl Pts',(27.9989137274389,536.110780927498,-47.5221601717528)) ;
#68006=CARTESIAN_POINT('Ctrl Pts',(28.0168750590771,536.168733948594,-47.5221601717528)) ;
#68007=CARTESIAN_POINT('Ctrl Pts',(28.0374699981699,536.225835262571,-47.5221601717528)) ;
#68008=CARTESIAN_POINT('Ctrl Pts',(28.0607089111533,536.281860922513,-47.5221601717528)) ;
#68009=CARTESIAN_POINT('Ctrl Pts',(28.0702708712446,536.30491342608,-47.5221601717528)) ;
#68010=CARTESIAN_POINT('Ctrl Pts',(28.0802806969461,536.327783586327,-47.5221601717528)) ;
#68011=CARTESIAN_POINT('Ctrl Pts',(28.0907400669133,536.350454728169,-47.5221601717528)) ;
#68012=CARTESIAN_POINT('Ctrl Pts',(28.0956199427452,536.361032072454,-47.5221601717528)) ;
#68013=CARTESIAN_POINT('Ctrl Pts',(28.100597680306,536.371566085872,-47.5221601717528)) ;
#68014=CARTESIAN_POINT('Ctrl Pts',(28.1056734895392,536.382055021761,-47.5221601717528)) ;
#68015=CARTESIAN_POINT('Ctrl Pts',(28.1109059706895,536.392867713255,-47.5221601717529)) ;
#68016=CARTESIAN_POINT('Ctrl Pts',(28.1162389961769,536.403624848622,-47.5221601717528)) ;
#68017=CARTESIAN_POINT('Ctrl Pts',(28.1216705430934,536.414321233288,-47.5221601717528)) ;
#68018=CARTESIAN_POINT('Ctrl Pts',(28.1528227355498,536.475669471426,-47.5221601717529)) ;
#68019=CARTESIAN_POINT('Ctrl Pts',(28.1872313289458,536.535060558472,-47.5221601717528)) ;
#68020=CARTESIAN_POINT('Ctrl Pts',(28.2248730925408,536.592190626077,-47.5221601717528)) ;
#68021=CARTESIAN_POINT('Ctrl Pts',(28.2592299129734,536.64433503395,-47.5221601717528)) ;
#68022=CARTESIAN_POINT('Ctrl Pts',(28.2962808697179,536.694595995804,-47.5221601717528)) ;
#68023=CARTESIAN_POINT('Ctrl Pts',(28.3360355478087,536.742716006994,-47.5221601717528)) ;
#68024=CARTESIAN_POINT('Ctrl Pts',(28.3827611865145,536.799273835288,-47.5221601717527)) ;
#68025=CARTESIAN_POINT('Ctrl Pts',(28.4332227235773,536.852875425638,-47.5221601717527)) ;
#68026=CARTESIAN_POINT('Ctrl Pts',(28.4870438712866,536.903316651351,-47.5221601717528)) ;
#68027=CARTESIAN_POINT('Ctrl Pts',(28.4989832996611,536.914506293846,-47.5221601717528)) ;
#68028=CARTESIAN_POINT('Ctrl Pts',(28.5110881336462,536.925540181673,-47.522160171753)) ;
#68029=CARTESIAN_POINT('Ctrl Pts',(28.5233543686585,536.936415683673,-47.5221601717529)) ;
#68030=CARTESIAN_POINT('Ctrl Pts',(28.5353619424006,536.947061851149,-47.5221601717527)) ;
#68031=CARTESIAN_POINT('Ctrl Pts',(28.5475283255332,536.957559542949,-47.5221601717527)) ;
#68032=CARTESIAN_POINT('Ctrl Pts',(28.5598256460145,536.967886419756,-47.5221601717527)) ;
#68033=CARTESIAN_POINT('Ctrl Pts',(28.6123312906609,537.011978897036,-47.5221601717529)) ;
#68034=CARTESIAN_POINT('Ctrl Pts',(28.667290106961,537.053025157918,-47.5221601717527)) ;
#68035=CARTESIAN_POINT('Ctrl Pts',(28.7243641711787,537.090910157219,-47.5221601717528)) ;
#68036=CARTESIAN_POINT('Ctrl Pts',(28.7814313798004,537.128790605868,-47.5221601717528)) ;
#68037=CARTESIAN_POINT('Ctrl Pts',(28.8406144442193,537.163510862665,-47.5221601717531)) ;
#68038=CARTESIAN_POINT('Ctrl Pts',(28.9015947041635,537.194907734422,-47.5221601717529)) ;
#68039=CARTESIAN_POINT('Ctrl Pts',(28.9461752574605,537.217860898545,-47.5221601717528)) ;
#68040=CARTESIAN_POINT('Ctrl Pts',(28.9917167912542,537.239036876612,-47.5221601717527)) ;
#68041=CARTESIAN_POINT('Ctrl Pts',(29.0380961522282,537.258354169963,-47.522160171753)) ;
#68042=CARTESIAN_POINT('Ctrl Pts',(29.057274895643,537.266342236311,-47.522160171753)) ;
#68043=CARTESIAN_POINT('Ctrl Pts',(29.0765968955737,537.2740122878,-47.5221601717531)) ;
#68044=CARTESIAN_POINT('Ctrl Pts',(29.0960533438445,537.281357768422,-47.522160171753)) ;
#68045=CARTESIAN_POINT('Ctrl Pts',(29.110489377956,537.286807869456,-47.5221601717529)) ;
#68046=CARTESIAN_POINT('Ctrl Pts',(29.1249994264623,537.292079279947,-47.5221601717527)) ;
#68047=CARTESIAN_POINT('Ctrl Pts',(29.1395798514287,537.297169151436,-47.5221601717527)) ;
#68048=CARTESIAN_POINT('Ctrl Pts',(29.1518554570994,537.301454434989,-47.5221601717527)) ;
#68049=CARTESIAN_POINT('Ctrl Pts',(29.164172997307,537.30560823222,-47.5221601717528)) ;
#68050=CARTESIAN_POINT('Ctrl Pts',(29.1765267084414,537.309628247203,-47.5221601717528)) ;
#68051=CARTESIAN_POINT('Ctrl Pts',(29.239143774932,537.330004435599,-47.5221601717528)) ;
#68052=CARTESIAN_POINT('Ctrl Pts',(29.3027194030454,537.346957735481,-47.5221601717529)) ;
#68053=CARTESIAN_POINT('Ctrl Pts',(29.3669625745666,537.360320290012,-47.5221601717529)) ;
#68054=CARTESIAN_POINT('Ctrl Pts',(29.4124482306339,537.36978128867,-47.5221601717529)) ;
#68055=CARTESIAN_POINT('Ctrl Pts',(29.4582686497801,537.37744126027,-47.5221601717528)) ;
#68056=CARTESIAN_POINT('Ctrl Pts',(29.5043181131541,537.383225073432,-47.5221601717529)) ;
#68057=CARTESIAN_POINT('Ctrl Pts',(29.5190280710151,537.385072644319,-47.5221601717529)) ;
#68058=CARTESIAN_POINT('Ctrl Pts',(29.5337636188551,537.38672888721,-47.5221601717531)) ;
#68059=CARTESIAN_POINT('Ctrl Pts',(29.5485139882223,537.388190360635,-47.522160171753)) ;
#68060=CARTESIAN_POINT('Ctrl Pts',(29.6112650202864,537.39440776194,-47.5221601717527)) ;
#68061=CARTESIAN_POINT('Ctrl Pts',(29.674168396674,537.397093581716,-47.522160171753)) ;
#68062=CARTESIAN_POINT('Ctrl Pts',(29.7369575657226,537.396079059198,-47.522160171753)) ;
#68063=CARTESIAN_POINT('Ctrl Pts',(29.7954524273515,537.395133922397,-47.5221601717529)) ;
#68064=CARTESIAN_POINT('Ctrl Pts',(29.8538486482669,537.390976944829,-47.5221601717529)) ;
#68065=CARTESIAN_POINT('Ctrl Pts',(29.9119178667258,537.383432974238,-47.5221601717531)) ;
#68066=CARTESIAN_POINT('Ctrl Pts',(29.921832697167,537.382144904737,-47.5221601717531)) ;
#68067=CARTESIAN_POINT('Ctrl Pts',(29.9317379531658,537.380758003776,-47.5221601717528)) ;
#68068=CARTESIAN_POINT('Ctrl Pts',(29.941632460783,537.379272913244,-47.5221601717531)) ;
#68069=CARTESIAN_POINT('Ctrl Pts',(28.6194567455546,536.789923813611,-49.5221601717528)) ;
#68070=CARTESIAN_POINT('Ctrl Pts',(28.5741835241712,536.747688703051,-49.5221601717528)) ;
#68071=CARTESIAN_POINT('Ctrl Pts',(28.5316436333847,536.702879617092,-49.5221601717529)) ;
#68072=CARTESIAN_POINT('Ctrl Pts',(28.4918334298705,536.655842595265,-49.5221601717528)) ;
#68073=CARTESIAN_POINT('Ctrl Pts',(28.4492968452567,536.605584267442,-49.5221601717527)) ;
#68074=CARTESIAN_POINT('Ctrl Pts',(28.4098758983343,536.552782180805,-49.522160171753)) ;
#68075=CARTESIAN_POINT('Ctrl Pts',(28.3735952737005,536.497803325823,-49.522160171753)) ;
#68076=CARTESIAN_POINT('Ctrl Pts',(28.341849727146,536.449696827713,-49.522160171753)) ;
#68077=CARTESIAN_POINT('Ctrl Pts',(28.3125087393969,536.399922503953,-49.5221601717529)) ;
#68078=CARTESIAN_POINT('Ctrl Pts',(28.2856119276886,536.348698435406,-49.522160171753)) ;
#68079=CARTESIAN_POINT('Ctrl Pts',(28.2720945912425,536.322955125151,-49.522160171753)) ;
#68080=CARTESIAN_POINT('Ctrl Pts',(28.2591949428059,536.296845294405,-49.5221601717529)) ;
#68081=CARTESIAN_POINT('Ctrl Pts',(28.2469203815683,536.270394759938,-49.5221601717529)) ;
#68082=CARTESIAN_POINT('Ctrl Pts',(28.2413692702196,536.258432632802,-49.5221601717529)) ;
#68083=CARTESIAN_POINT('Ctrl Pts',(28.2359455138467,536.246399331703,-49.522160171753)) ;
#68084=CARTESIAN_POINT('Ctrl Pts',(28.2306580911855,536.234316773402,-49.522160171753)) ;
#68085=CARTESIAN_POINT('Ctrl Pts',(28.203570951268,536.172418573045,-49.522160171753)) ;
#68086=CARTESIAN_POINT('Ctrl Pts',(28.1800053268915,536.109118453109,-49.5221601717528)) ;
#68087=CARTESIAN_POINT('Ctrl Pts',(28.1599830712663,536.044785442915,-49.5221601717528)) ;
#68088=CARTESIAN_POINT('Ctrl Pts',(28.139960815641,535.98045243272,-49.5221601717528)) ;
#68089=CARTESIAN_POINT('Ctrl Pts',(28.1234814998453,535.915085598446,-49.5221601717529)) ;
#68090=CARTESIAN_POINT('Ctrl Pts',(28.1106053005632,535.849018425769,-49.5221601717529)) ;
#68091=CARTESIAN_POINT('Ctrl Pts',(28.0997084494549,535.793107195442,-49.5221601717529)) ;
#68092=CARTESIAN_POINT('Ctrl Pts',(28.0913926099977,535.73669347859,-49.5221601717529)) ;
#68093=CARTESIAN_POINT('Ctrl Pts',(28.0857191798105,535.679967078133,-49.5221601717529)) ;
#68094=CARTESIAN_POINT('Ctrl Pts',(28.0830976380087,535.65375531115,-49.5221601717529)) ;
#68095=CARTESIAN_POINT('Ctrl Pts',(28.0810406218419,535.627476667704,-49.5221601717529)) ;
#68096=CARTESIAN_POINT('Ctrl Pts',(28.0795560257393,535.60114946616,-49.5221601717529)) ;
#68097=CARTESIAN_POINT('Ctrl Pts',(28.0789167406597,535.589812654008,-49.5221601717529)) ;
#68098=CARTESIAN_POINT('Ctrl Pts',(28.0783837314708,535.578467436334,-49.5221601717529)) ;
#68099=CARTESIAN_POINT('Ctrl Pts',(28.0779579170341,535.567128747108,-49.5221601717529)) ;
#68100=CARTESIAN_POINT('Ctrl Pts',(28.0753221846355,535.496943830925,-49.5221601717529)) ;
#68101=CARTESIAN_POINT('Ctrl Pts',(28.0767816822343,535.426878372279,-49.5221601717529)) ;
#68102=CARTESIAN_POINT('Ctrl Pts',(28.0823886751965,535.357295690998,-49.5221601717529)) ;
#68103=CARTESIAN_POINT('Ctrl Pts',(28.0874298054729,535.294735355418,-49.5221601717529)) ;
#68104=CARTESIAN_POINT('Ctrl Pts',(28.0958238609977,535.232564296308,-49.5221601717529)) ;
#68105=CARTESIAN_POINT('Ctrl Pts',(28.107642624543,535.171034219996,-49.5221601717529)) ;
#68106=CARTESIAN_POINT('Ctrl Pts',(28.1204534679983,535.10433924193,-49.5221601717529)) ;
#68107=CARTESIAN_POINT('Ctrl Pts',(28.1372870528362,535.038396522335,-49.522160171753)) ;
#68108=CARTESIAN_POINT('Ctrl Pts',(28.1578992251687,534.973418262404,-49.522160171753)) ;
#68109=CARTESIAN_POINT('Ctrl Pts',(28.165767691918,534.948613536855,-49.5221601717529)) ;
#68110=CARTESIAN_POINT('Ctrl Pts',(28.1741873351911,534.92394940569,-49.5221601717529)) ;
#68111=CARTESIAN_POINT('Ctrl Pts',(28.1831465099758,534.899437990031,-49.5221601717529)) ;
#68112=CARTESIAN_POINT('Ctrl Pts',(28.1870922543454,534.888642823885,-49.5221601717529)) ;
#68113=CARTESIAN_POINT('Ctrl Pts',(28.1911423844193,534.877878274877,-49.5221601717529)) ;
#68114=CARTESIAN_POINT('Ctrl Pts',(28.1952910524112,534.867157270828,-49.5221601717529)) ;
#68115=CARTESIAN_POINT('Ctrl Pts',(28.2205415246478,534.801904901726,-49.522160171753)) ;
#68116=CARTESIAN_POINT('Ctrl Pts',(28.2494802213268,534.738147870322,-49.522160171753)) ;
#68117=CARTESIAN_POINT('Ctrl Pts',(28.2817953527524,534.676103380191,-49.522160171753)) ;
#68118=CARTESIAN_POINT('Ctrl Pts',(28.3148512464585,534.612636639368,-49.5221601717529)) ;
#68119=CARTESIAN_POINT('Ctrl Pts',(28.3514404488416,534.550961035581,-49.522160171753)) ;
#68120=CARTESIAN_POINT('Ctrl Pts',(28.3912853225522,534.491312947336,-49.522160171753)) ;
#68121=CARTESIAN_POINT('Ctrl Pts',(28.421395761063,534.446237384883,-49.522160171753)) ;
#68122=CARTESIAN_POINT('Ctrl Pts',(28.4533666306937,534.402319663736,-49.5221601717529)) ;
#68123=CARTESIAN_POINT('Ctrl Pts',(28.4870968158936,534.359667673985,-49.522160171753)) ;
#68124=CARTESIAN_POINT('Ctrl Pts',(28.5079985866382,534.333237279183,-49.522160171753)) ;
#68125=CARTESIAN_POINT('Ctrl Pts',(28.5295762366623,534.307293039875,-49.5221601717528)) ;
#68126=CARTESIAN_POINT('Ctrl Pts',(28.5518084276599,534.281862208131,-49.5221601717529)) ;
#68127=CARTESIAN_POINT('Ctrl Pts',(28.5603078651189,534.272139920122,-49.5221601717529)) ;
#68128=CARTESIAN_POINT('Ctrl Pts',(28.5689045301256,534.262490991216,-49.522160171753)) ;
#68129=CARTESIAN_POINT('Ctrl Pts',(28.5775922730039,534.252922526196,-49.522160171753)) ;
#68130=CARTESIAN_POINT('Ctrl Pts',(28.6291688757767,534.196117332211,-49.522160171753)) ;
#68131=CARTESIAN_POINT('Ctrl Pts',(28.683825070941,534.142282619883,-49.5221601717529)) ;
#68132=CARTESIAN_POINT('Ctrl Pts',(28.7412498653522,534.091699428638,-49.5221601717528)) ;
#68133=CARTESIAN_POINT('Ctrl Pts',(28.7843184611605,534.053762035204,-49.5221601717528)) ;
#68134=CARTESIAN_POINT('Ctrl Pts',(28.8289456970457,534.017653807843,-49.5221601717529)) ;
#68135=CARTESIAN_POINT('Ctrl Pts',(28.87501898973,533.983503817113,-49.5221601717528)) ;
#68136=CARTESIAN_POINT('Ctrl Pts',(28.8913736012136,533.971381613597,-49.5221601717528)) ;
#68137=CARTESIAN_POINT('Ctrl Pts',(28.9079105525739,533.959506258588,-49.5221601717527)) ;
#68138=CARTESIAN_POINT('Ctrl Pts',(28.9246252217011,533.947883902412,-49.5221601717529)) ;
#68139=CARTESIAN_POINT('Ctrl Pts',(28.9372829380326,533.939082502488,-49.5221601717531)) ;
#68140=CARTESIAN_POINT('Ctrl Pts',(28.9500384200079,533.930429161134,-49.522160171753)) ;
#68141=CARTESIAN_POINT('Ctrl Pts',(28.9628827037222,533.921930640592,-49.522160171753)) ;
#68142=CARTESIAN_POINT('Ctrl Pts',(29.0256895766991,533.880373983011,-49.522160171753)) ;
#68143=CARTESIAN_POINT('Ctrl Pts',(29.0906640066724,533.842483570269,-49.5221601717531)) ;
#68144=CARTESIAN_POINT('Ctrl Pts',(29.1575446499793,533.808535771635,-49.522160171753)) ;
#68145=CARTESIAN_POINT('Ctrl Pts',(29.2115680980119,533.781114128471,-49.522160171753)) ;
#68146=CARTESIAN_POINT('Ctrl Pts',(29.2668362837646,533.756265219817,-49.522160171753)) ;
#68147=CARTESIAN_POINT('Ctrl Pts',(29.3232283120257,533.734153036032,-49.5221601717528)) ;
#68148=CARTESIAN_POINT('Ctrl Pts',(29.3337310402553,533.730034754353,-49.5221601717528)) ;
#68149=CARTESIAN_POINT('Ctrl Pts',(29.3442727870821,533.726011456111,-49.5221601717526)) ;
#68150=CARTESIAN_POINT('Ctrl Pts',(29.3548523877517,533.722082788819,-49.5221601717526)) ;
#68151=CARTESIAN_POINT('Ctrl Pts',(29.9416053009762,537.375719435804,-47.5212987075501)) ;
#68152=CARTESIAN_POINT('Ctrl Pts',(29.9491437898387,537.375479142474,-47.5215858622844)) ;
#68153=CARTESIAN_POINT('Ctrl Pts',(29.9566806468873,537.37518765597,-47.5218730170187)) ;
#68154=CARTESIAN_POINT('Ctrl Pts',(29.9642151770171,537.374845003176,-47.522160171753)) ;
#68155=CARTESIAN_POINT('Ctrl Pts',(30.4192300785532,583.719768248152,-49.5189951107294)) ;
#68156=CARTESIAN_POINT('Ctrl Pts',(31.0820332975824,583.896429840045,-49.4819041482875)) ;
#68157=CARTESIAN_POINT('Ctrl Pts',(32.2050033717352,584.964207263547,-49.4077391038933)) ;
#68158=CARTESIAN_POINT('Ctrl Pts',(31.7732242756362,587.256677742684,-49.2964999775465)) ;
#68159=CARTESIAN_POINT('Ctrl Pts',(29.6099548125204,588.131120449431,-49.185277731689)) ;
#68160=CARTESIAN_POINT('Ctrl Pts',(27.7035655963549,586.788278335697,-49.0740554858316)) ;
#68161=CARTESIAN_POINT('Ctrl Pts',(27.7990464989561,584.45752039736,-48.9628332399742)) ;
#68162=CARTESIAN_POINT('Ctrl Pts',(29.8100268470855,583.275562917911,-48.8516109941169)) ;
#68163=CARTESIAN_POINT('Ctrl Pts',(31.8927897096346,584.325470257128,-48.7403887482596)) ;
#68164=CARTESIAN_POINT('Ctrl Pts',(32.1385417975513,586.644990498722,-48.6291665024023)) ;
#68165=CARTESIAN_POINT('Ctrl Pts',(30.3219322734697,588.10802924709,-48.5179442565448)) ;
#68166=CARTESIAN_POINT('Ctrl Pts',(28.1080818049476,587.373600016883,-48.4067220106873)) ;
#68167=CARTESIAN_POINT('Ctrl Pts',(27.5261524671424,585.114866204111,-48.2954997648299)) ;
#68168=CARTESIAN_POINT('Ctrl Pts',(29.1095299162611,583.402129097654,-48.1842775189726)) ;
#68169=CARTESIAN_POINT('Ctrl Pts',(31.4069240173951,583.805302241545,-48.0730552731154)) ;
#68170=CARTESIAN_POINT('Ctrl Pts',(32.312527681685,585.954741369732,-47.961833027258)) ;
#68171=CARTESIAN_POINT('Ctrl Pts',(30.9963393282325,587.880543452508,-47.8506107814006)) ;
#68172=CARTESIAN_POINT('Ctrl Pts',(28.66449088512,587.817045356221,-47.7393885355431)) ;
#68173=CARTESIAN_POINT('Ctrl Pts',(27.4546192595412,585.823617294928,-47.6281662896857)) ;
#68174=CARTESIAN_POINT('Ctrl Pts',(28.4743800506003,583.724933720291,-47.5169440438284)) ;
#68175=CARTESIAN_POINT('Ctrl Pts',(30.7908823865385,583.450313172167,-47.4057075193723)) ;
#68176=CARTESIAN_POINT('Ctrl Pts',(31.7796747638363,584.643315655865,-47.3315450768686)) ;
#68177=CARTESIAN_POINT('Ctrl Pts',(31.9108216721039,585.31655469127,-47.2944567163174)) ;
#68178=CARTESIAN_POINT('Ctrl Pts',(30.3850875462748,583.847845379583,-49.5955228059578)) ;
#68179=CARTESIAN_POINT('Ctrl Pts',(31.0052495825354,584.013141517883,-49.5584318435159)) ;
#68180=CARTESIAN_POINT('Ctrl Pts',(32.0559738214225,585.012223903455,-49.4842667991217)) ;
#68181=CARTESIAN_POINT('Ctrl Pts',(31.6519730625794,587.157209201643,-49.3730276727749)) ;
#68182=CARTESIAN_POINT('Ctrl Pts',(29.6278766841831,587.975394982943,-49.2618054269174)) ;
#68183=CARTESIAN_POINT('Ctrl Pts',(27.8441342637189,586.718944085118,-49.15058318106)) ;
#68184=CARTESIAN_POINT('Ctrl Pts',(27.9334724402411,584.538134536265,-49.0393609352026)) ;
#68185=CARTESIAN_POINT('Ctrl Pts',(29.8150771635899,583.432217823454,-48.9281386893453)) ;
#68186=CARTESIAN_POINT('Ctrl Pts',(31.7638463017036,584.41457978954,-48.8169164434881)) ;
#68187=CARTESIAN_POINT('Ctrl Pts',(31.9937880263092,586.584874614423,-48.7056941976306)) ;
#68188=CARTESIAN_POINT('Ctrl Pts',(30.2940493569722,587.953789343964,-48.5944719517732)) ;
#68189=CARTESIAN_POINT('Ctrl Pts',(28.2226260821331,587.266609327605,-48.4832497059157)) ;
#68190=CARTESIAN_POINT('Ctrl Pts',(27.6781349379567,585.153190260705,-48.3720274600584)) ;
#68191=CARTESIAN_POINT('Ctrl Pts',(29.1596464255638,583.550641418117,-48.260805214201)) ;
#68192=CARTESIAN_POINT('Ctrl Pts',(31.3092385864758,583.927876577365,-48.1495829683438)) ;
#68193=CARTESIAN_POINT('Ctrl Pts',(32.1565805974484,585.939032389956,-48.0383607224865)) ;
#68194=CARTESIAN_POINT('Ctrl Pts',(30.9250687007873,587.740938757941,-47.927138476629)) ;
#68195=CARTESIAN_POINT('Ctrl Pts',(28.7432388043513,587.681525786548,-47.8159162307715)) ;
#68196=CARTESIAN_POINT('Ctrl Pts',(27.6112037909547,585.816344130607,-47.7046939849141)) ;
#68197=CARTESIAN_POINT('Ctrl Pts',(28.5653586751273,583.852678533116,-47.5934717390568)) ;
#68198=CARTESIAN_POINT('Ctrl Pts',(30.7328297501203,583.595725589265,-47.4822352146008)) ;
#68199=CARTESIAN_POINT('Ctrl Pts',(31.658008561174,584.711976730347,-47.4080727720971)) ;
#68200=CARTESIAN_POINT('Ctrl Pts',(31.7807181850044,585.34190319887,-47.3709844115459)) ;
#68201=CARTESIAN_POINT('Ctrl Pts',(30.3509450139963,583.975922511015,-49.6720505011861)) ;
#68202=CARTESIAN_POINT('Ctrl Pts',(30.9284658674885,584.12985319572,-49.6349595387444)) ;
#68203=CARTESIAN_POINT('Ctrl Pts',(31.90694427111,585.060240543361,-49.56079449435)) ;
#68204=CARTESIAN_POINT('Ctrl Pts',(31.5307218495225,587.0577406606,-49.4495553680033)) ;
#68205=CARTESIAN_POINT('Ctrl Pts',(29.6457985558456,587.819669516452,-49.3383331221458)) ;
#68206=CARTESIAN_POINT('Ctrl Pts',(27.9847029310828,586.649609834538,-49.2271108762884)) ;
#68207=CARTESIAN_POINT('Ctrl Pts',(28.0678983815261,584.618748675169,-49.115888630431)) ;
#68208=CARTESIAN_POINT('Ctrl Pts',(29.8201274800944,583.588872728996,-49.0046663845737)) ;
#68209=CARTESIAN_POINT('Ctrl Pts',(31.6349028937727,584.503689321952,-48.8934441387164)) ;
#68210=CARTESIAN_POINT('Ctrl Pts',(31.8490342550673,586.524758730124,-48.782221892859)) ;
#68211=CARTESIAN_POINT('Ctrl Pts',(30.2661664404749,587.799549440838,-48.6709996470017)) ;
#68212=CARTESIAN_POINT('Ctrl Pts',(28.3371703593188,587.159618638329,-48.5597774011441)) ;
#68213=CARTESIAN_POINT('Ctrl Pts',(27.830117408771,585.191514317299,-48.4485551552867)) ;
#68214=CARTESIAN_POINT('Ctrl Pts',(29.2097629348664,583.699153738578,-48.3373329094294)) ;
#68215=CARTESIAN_POINT('Ctrl Pts',(31.2115531555567,584.050450913185,-48.2261106635721)) ;
#68216=CARTESIAN_POINT('Ctrl Pts',(32.0006335132117,585.92332341018,-48.1148884177148)) ;
#68217=CARTESIAN_POINT('Ctrl Pts',(30.8537980733421,587.601334063374,-48.0036661718574)) ;
#68218=CARTESIAN_POINT('Ctrl Pts',(28.8219867235824,587.546006216873,-47.892443926)) ;
#68219=CARTESIAN_POINT('Ctrl Pts',(27.7677883223683,585.809070966287,-47.7812216801425)) ;
#68220=CARTESIAN_POINT('Ctrl Pts',(28.6563372996543,583.980423345943,-47.6699994342852)) ;
#68221=CARTESIAN_POINT('Ctrl Pts',(30.6747771137021,583.741138006364,-47.5587629098291)) ;
#68222=CARTESIAN_POINT('Ctrl Pts',(31.5363423585119,584.78063780483,-47.4846004673254)) ;
#68223=CARTESIAN_POINT('Ctrl Pts',(31.6506146979047,585.367251706467,-47.4475121067741)) ;
#68224=CARTESIAN_POINT('Ctrl Pts',(30.3168024817179,584.103999642447,-49.7485781964146)) ;
#68225=CARTESIAN_POINT('Ctrl Pts',(30.8516821524416,584.246564873558,-49.7114872339728)) ;
#68226=CARTESIAN_POINT('Ctrl Pts',(31.7579147207974,585.108257183268,-49.6373221895785)) ;
#68227=CARTESIAN_POINT('Ctrl Pts',(31.4094706364656,586.958272119558,-49.5260830632317)) ;
#68228=CARTESIAN_POINT('Ctrl Pts',(29.6637204275083,587.663944049963,-49.4148608173743)) ;
#68229=CARTESIAN_POINT('Ctrl Pts',(28.1252715984466,586.580275583958,-49.3036385715168)) ;
#68230=CARTESIAN_POINT('Ctrl Pts',(28.2023243228111,584.699362814073,-49.1924163256595)) ;
#68231=CARTESIAN_POINT('Ctrl Pts',(29.8251777965987,583.745527634539,-49.0811940798022)) ;
#68232=CARTESIAN_POINT('Ctrl Pts',(31.5059594858419,584.592798854365,-48.9699718339449)) ;
#68233=CARTESIAN_POINT('Ctrl Pts',(31.7042804838254,586.464642845826,-48.8587495880875)) ;
#68234=CARTESIAN_POINT('Ctrl Pts',(30.2382835239775,587.645309537712,-48.7475273422301)) ;
#68235=CARTESIAN_POINT('Ctrl Pts',(28.4517146365045,587.052627949051,-48.6363050963726)) ;
#68236=CARTESIAN_POINT('Ctrl Pts',(27.9820998795853,585.229838373894,-48.5250828505152)) ;
#68237=CARTESIAN_POINT('Ctrl Pts',(29.2598794441691,583.84766605904,-48.4138606046579)) ;
#68238=CARTESIAN_POINT('Ctrl Pts',(31.1138677246376,584.173025249005,-48.3026383588006)) ;
#68239=CARTESIAN_POINT('Ctrl Pts',(31.844686428975,585.907614430404,-48.1914161129433)) ;
#68240=CARTESIAN_POINT('Ctrl Pts',(30.7825274458969,587.461729368807,-48.0801938670858)) ;
#68241=CARTESIAN_POINT('Ctrl Pts',(28.9007346428137,587.410486647199,-47.9689716212284)) ;
#68242=CARTESIAN_POINT('Ctrl Pts',(27.9243728537819,585.801797801967,-47.857749375371)) ;
#68243=CARTESIAN_POINT('Ctrl Pts',(28.7473159241813,584.108168158769,-47.7465271295137)) ;
#68244=CARTESIAN_POINT('Ctrl Pts',(30.616724477284,583.886550423464,-47.6352906050575)) ;
#68245=CARTESIAN_POINT('Ctrl Pts',(31.4146761558497,584.849298879313,-47.5611281625539)) ;
#68246=CARTESIAN_POINT('Ctrl Pts',(31.5205112108052,585.392600214065,-47.5240398020026)) ;
#68247=CARTESIAN_POINT('Ctrl Pts',(31.5236569526671,585.391334705933,-47.522160171753)) ;
#68248=CARTESIAN_POINT('Ctrl Pts',(31.5188401675311,585.329303680336,-47.522160171753)) ;
#68249=CARTESIAN_POINT('Ctrl Pts',(31.510269991655,585.26781004648,-47.522160171753)) ;
#68250=CARTESIAN_POINT('Ctrl Pts',(31.4982232071401,585.207069811533,-47.522160171753)) ;
#68251=CARTESIAN_POINT('Ctrl Pts',(31.4857315767339,585.144086650771,-47.522160171753)) ;
#68252=CARTESIAN_POINT('Ctrl Pts',(31.4695018364279,585.081912853305,-47.522160171753)) ;
#68253=CARTESIAN_POINT('Ctrl Pts',(31.449786324334,585.020778555998,-47.5221601717531)) ;
#68254=CARTESIAN_POINT('Ctrl Pts',(31.4316885056168,584.964660438202,-47.5221601717531)) ;
#68255=CARTESIAN_POINT('Ctrl Pts',(31.4106526261513,584.909417627139,-47.5221601717531)) ;
#68256=CARTESIAN_POINT('Ctrl Pts',(31.3868352669909,584.855228845485,-47.522160171753)) ;
#68257=CARTESIAN_POINT('Ctrl Pts',(31.3751359799049,584.828610860294,-47.5221601717529)) ;
#68258=CARTESIAN_POINT('Ctrl Pts',(31.3627650218181,584.80224726166,-47.5221601717531)) ;
#68259=CARTESIAN_POINT('Ctrl Pts',(31.3497379680007,584.776159928329,-47.5221601717531)) ;
#68260=CARTESIAN_POINT('Ctrl Pts',(31.3438455310544,584.764360025687,-47.5221601717531)) ;
#68261=CARTESIAN_POINT('Ctrl Pts',(31.3378179980786,584.752615328467,-47.5221601717531)) ;
#68262=CARTESIAN_POINT('Ctrl Pts',(31.3316669117536,584.740946529661,-47.5221601717531)) ;
#68263=CARTESIAN_POINT('Ctrl Pts',(31.3001600716856,584.681177090842,-47.522160171753)) ;
#68264=CARTESIAN_POINT('Ctrl Pts',(31.2653614871049,584.623286734142,-47.522160171753)) ;
#68265=CARTESIAN_POINT('Ctrl Pts',(31.2275461136954,584.567522616136,-47.5221601717531)) ;
#68266=CARTESIAN_POINT('Ctrl Pts',(31.1897307402858,584.51175849813,-47.5221601717532)) ;
#68267=CARTESIAN_POINT('Ctrl Pts',(31.1488981152621,584.45811970133,-47.5221601717531)) ;
#68268=CARTESIAN_POINT('Ctrl Pts',(31.1052715103391,584.406861182841,-47.5221601717531)) ;
#68269=CARTESIAN_POINT('Ctrl Pts',(31.0683501055194,584.363480852996,-47.5221601717531)) ;
#68270=CARTESIAN_POINT('Ctrl Pts',(31.0294265346734,584.321805179775,-47.5221601717531)) ;
#68271=CARTESIAN_POINT('Ctrl Pts',(30.988610958903,584.28200051088,-47.5221601717531)) ;
#68272=CARTESIAN_POINT('Ctrl Pts',(30.9697524459878,584.263609079465,-47.5221601717531)) ;
#68273=CARTESIAN_POINT('Ctrl Pts',(30.9504897208788,584.245617269463,-47.5221601717533)) ;
#68274=CARTESIAN_POINT('Ctrl Pts',(30.9308321861222,584.228042671206,-47.5221601717532)) ;
#68275=CARTESIAN_POINT('Ctrl Pts',(30.9223660422836,584.220473610355,-47.5221601717531)) ;
#68276=CARTESIAN_POINT('Ctrl Pts',(30.9138270458502,584.212982410202,-47.522160171753)) ;
#68277=CARTESIAN_POINT('Ctrl Pts',(30.9052263083889,584.205579107581,-47.522160171753)) ;
#68278=CARTESIAN_POINT('Ctrl Pts',(30.8519948284383,584.159758762896,-47.522160171753)) ;
#68279=CARTESIAN_POINT('Ctrl Pts',(30.7963035204994,584.117214641986,-47.5221601717532)) ;
#68280=CARTESIAN_POINT('Ctrl Pts',(30.7384039283002,584.078214128361,-47.5221601717532)) ;
#68281=CARTESIAN_POINT('Ctrl Pts',(30.6863451657001,584.043147931813,-47.5221601717533)) ;
#68282=CARTESIAN_POINT('Ctrl Pts',(30.6325002196233,584.010946103046,-47.5221601717531)) ;
#68283=CARTESIAN_POINT('Ctrl Pts',(30.5770212017373,583.981821726431,-47.5221601717531)) ;
#68284=CARTESIAN_POINT('Ctrl Pts',(30.5168873937906,583.950253761881,-47.5221601717532)) ;
#68285=CARTESIAN_POINT('Ctrl Pts',(30.4548337940956,583.922299973818,-47.5221601717531)) ;
#68286=CARTESIAN_POINT('Ctrl Pts',(30.3911785114919,583.897901782336,-47.522160171753)) ;
#68287=CARTESIAN_POINT('Ctrl Pts',(30.3668794535727,583.888588288723,-47.5221601717529)) ;
#68288=CARTESIAN_POINT('Ctrl Pts',(30.3423467027344,583.879793361185,-47.5221601717531)) ;
#68289=CARTESIAN_POINT('Ctrl Pts',(30.3175969936173,583.871515452949,-47.5221601717533)) ;
#68290=CARTESIAN_POINT('Ctrl Pts',(30.3066967610943,583.867869708098,-47.5221601717534)) ;
#68291=CARTESIAN_POINT('Ctrl Pts',(30.2957553887351,583.864324663052,-47.522160171753)) ;
#68292=CARTESIAN_POINT('Ctrl Pts',(30.2847866297612,583.860883806162,-47.522160171753)) ;
#68293=CARTESIAN_POINT('Ctrl Pts',(30.2180252438734,583.839941019909,-47.522160171753)) ;
#68294=CARTESIAN_POINT('Ctrl Pts',(30.150133573222,583.822814191443,-47.5221601717531)) ;
#68295=CARTESIAN_POINT('Ctrl Pts',(30.0814758060322,583.809394978751,-47.522160171753)) ;
#68296=CARTESIAN_POINT('Ctrl Pts',(30.0112444562779,583.795668208153,-47.522160171753)) ;
#68297=CARTESIAN_POINT('Ctrl Pts',(29.9402106626795,583.785820679544,-47.5221601717534)) ;
#68298=CARTESIAN_POINT('Ctrl Pts',(29.8687323076889,583.779782709858,-47.5221601717533)) ;
#68299=CARTESIAN_POINT('Ctrl Pts',(29.8147182254866,583.775219994459,-47.5221601717533)) ;
#68300=CARTESIAN_POINT('Ctrl Pts',(29.7604495150754,583.772833624314,-47.5221601717531)) ;
#68301=CARTESIAN_POINT('Ctrl Pts',(29.7060735484461,583.772611814858,-47.5221601717532)) ;
#68302=CARTESIAN_POINT('Ctrl Pts',(29.6723780247881,583.77247436469,-47.5221601717532)) ;
#68303=CARTESIAN_POINT('Ctrl Pts',(29.6386412158712,583.773168416777,-47.5221601717529)) ;
#68304=CARTESIAN_POINT('Ctrl Pts',(29.6048977269777,583.774694279834,-47.5221601717531)) ;
#68305=CARTESIAN_POINT('Ctrl Pts',(29.5919967889767,583.775277653555,-47.5221601717532)) ;
#68306=CARTESIAN_POINT('Ctrl Pts',(29.5790925886481,583.775982789546,-47.5221601717528)) ;
#68307=CARTESIAN_POINT('Ctrl Pts',(29.5661945128201,583.776809309743,-47.5221601717529)) ;
#68308=CARTESIAN_POINT('Ctrl Pts',(29.4896246981783,583.781715971724,-47.5221601717529)) ;
#68309=CARTESIAN_POINT('Ctrl Pts',(29.4134573117978,583.790882449776,-47.5221601717532)) ;
#68310=CARTESIAN_POINT('Ctrl Pts',(29.3381059440092,583.804240827962,-47.5221601717532)) ;
#68311=CARTESIAN_POINT('Ctrl Pts',(29.2815924181677,583.814259611602,-47.5221601717532)) ;
#68312=CARTESIAN_POINT('Ctrl Pts',(29.2255372354374,583.826637473437,-47.5221601717532)) ;
#68313=CARTESIAN_POINT('Ctrl Pts',(29.1701114870961,583.841366868005,-47.5221601717533)) ;
#68314=CARTESIAN_POINT('Ctrl Pts',(29.1504411817609,583.846594252339,-47.5221601717533)) ;
#68315=CARTESIAN_POINT('Ctrl Pts',(29.1308501530702,583.852117980893,-47.5221601717531)) ;
#68316=CARTESIAN_POINT('Ctrl Pts',(29.1113460858728,583.857938274527,-47.5221601717531)) ;
#68317=CARTESIAN_POINT('Ctrl Pts',(29.096575143476,583.862346135776,-47.5221601717531)) ;
#68318=CARTESIAN_POINT('Ctrl Pts',(29.0818589756558,583.86692269961,-47.5221601717531)) ;
#68319=CARTESIAN_POINT('Ctrl Pts',(29.0672084681585,583.871665170823,-47.5221601717531)) ;
#68320=CARTESIAN_POINT('Ctrl Pts',(28.9955587082349,583.894858696637,-47.5221601717532)) ;
#68321=CARTESIAN_POINT('Ctrl Pts',(28.9254238704092,583.922032771105,-47.5221601717531)) ;
#68322=CARTESIAN_POINT('Ctrl Pts',(28.8571829382313,583.953155379993,-47.522160171753)) ;
#68323=CARTESIAN_POINT('Ctrl Pts',(28.8020543600867,583.978297843927,-47.522160171753)) ;
#68324=CARTESIAN_POINT('Ctrl Pts',(28.7481613973935,584.006018160781,-47.5221601717531)) ;
#68325=CARTESIAN_POINT('Ctrl Pts',(28.6957076913023,584.036324060624,-47.5221601717529)) ;
#68326=CARTESIAN_POINT('Ctrl Pts',(28.6853634342856,584.042300607192,-47.5221601717529)) ;
#68327=CARTESIAN_POINT('Ctrl Pts',(28.6750751736428,584.048377778284,-47.522160171753)) ;
#68328=CARTESIAN_POINT('Ctrl Pts',(28.6648434444544,584.05455423117,-47.5221601717531)) ;
#68329=CARTESIAN_POINT('',(31.158643478419,586.791459225795,-49.5230281993293)) ;
#68330=CARTESIAN_POINT('Ctrl Pts',(31.1572796596168,586.790298588641,-49.5230281993293)) ;
#68331=CARTESIAN_POINT('Ctrl Pts',(31.1523539815153,586.796086558105,-49.5227388568039)) ;
#68332=CARTESIAN_POINT('Ctrl Pts',(31.1473886962525,586.801840821075,-49.5224495142784)) ;
#68333=CARTESIAN_POINT('Ctrl Pts',(31.1423842688183,586.807560838673,-49.5221601717531)) ;
#68334=CARTESIAN_POINT('Ctrl Pts',(30.4186978426039,583.72539083489,-49.5221601717529)) ;
#68335=CARTESIAN_POINT('Ctrl Pts',(30.4873003083186,583.750791784544,-49.5221601717532)) ;
#68336=CARTESIAN_POINT('Ctrl Pts',(30.554200304582,583.780092786686,-49.5221601717532)) ;
#68337=CARTESIAN_POINT('Ctrl Pts',(30.6192099749106,583.812997033709,-49.5221601717531)) ;
#68338=CARTESIAN_POINT('Ctrl Pts',(30.6860813906505,583.846843591785,-49.522160171753)) ;
#68339=CARTESIAN_POINT('Ctrl Pts',(30.7509534329247,583.884503418489,-49.5221601717532)) ;
#68340=CARTESIAN_POINT('Ctrl Pts',(30.8135904385567,583.925698250773,-49.5221601717532)) ;
#68341=CARTESIAN_POINT('Ctrl Pts',(30.8665813102266,583.960549055804,-49.5221601717531)) ;
#68342=CARTESIAN_POINT('Ctrl Pts',(30.9179722019561,583.997930973722,-49.5221601717531)) ;
#68343=CARTESIAN_POINT('Ctrl Pts',(30.9675975968691,584.037693629774,-49.5221601717531)) ;
#68344=CARTESIAN_POINT('Ctrl Pts',(30.9896051368742,584.05532730796,-49.5221601717531)) ;
#68345=CARTESIAN_POINT('Ctrl Pts',(31.0112651554311,584.073429381718,-49.522160171753)) ;
#68346=CARTESIAN_POINT('Ctrl Pts',(31.0325616669576,584.09198745669,-49.5221601717529)) ;
#68347=CARTESIAN_POINT('Ctrl Pts',(31.0442315898504,584.102156789056,-49.5221601717529)) ;
#68348=CARTESIAN_POINT('Ctrl Pts',(31.055792343147,584.112463053672,-49.5221601717529)) ;
#68349=CARTESIAN_POINT('Ctrl Pts',(31.0672411640197,584.122904252017,-49.5221601717529)) ;
#68350=CARTESIAN_POINT('Ctrl Pts',(31.0778809940872,584.132607659672,-49.522160171753)) ;
#68351=CARTESIAN_POINT('Ctrl Pts',(31.0884256653329,584.142429199591,-49.5221601717529)) ;
#68352=CARTESIAN_POINT('Ctrl Pts',(31.0988568852982,584.152351608469,-49.5221601717529)) ;
#68353=CARTESIAN_POINT('Ctrl Pts',(31.1519330615585,584.202838850063,-49.5221601717529)) ;
#68354=CARTESIAN_POINT('Ctrl Pts',(31.2021692727164,584.256018704938,-49.522160171753)) ;
#68355=CARTESIAN_POINT('Ctrl Pts',(31.2493474364414,584.311628175327,-49.522160171753)) ;
#68356=CARTESIAN_POINT('Ctrl Pts',(31.2961710704225,584.366819757232,-49.522160171753)) ;
#68357=CARTESIAN_POINT('Ctrl Pts',(31.339982954292,584.424405467255,-49.522160171753)) ;
#68358=CARTESIAN_POINT('Ctrl Pts',(31.3805250711276,584.484152427248,-49.522160171753)) ;
#68359=CARTESIAN_POINT('Ctrl Pts',(31.414278646109,584.533895106008,-49.5221601717531)) ;
#68360=CARTESIAN_POINT('Ctrl Pts',(31.4457651463981,584.585136509089,-49.5221601717531)) ;
#68361=CARTESIAN_POINT('Ctrl Pts',(31.474807879904,584.637748693389,-49.5221601717531)) ;
#68362=CARTESIAN_POINT('Ctrl Pts',(31.4868690766659,584.659598079804,-49.5221601717531)) ;
#68363=CARTESIAN_POINT('Ctrl Pts',(31.4985084828501,584.681683918493,-49.522160171753)) ;
#68364=CARTESIAN_POINT('Ctrl Pts',(31.5097120155267,584.703997122186,-49.522160171753)) ;
#68365=CARTESIAN_POINT('Ctrl Pts',(31.5149384960288,584.714406296454,-49.522160171753)) ;
#68366=CARTESIAN_POINT('Ctrl Pts',(31.5200701071974,584.724864950923,-49.522160171753)) ;
#68367=CARTESIAN_POINT('Ctrl Pts',(31.525105353132,584.735372160716,-49.522160171753)) ;
#68368=CARTESIAN_POINT('Ctrl Pts',(31.5302972980837,584.746206359393,-49.522160171753)) ;
#68369=CARTESIAN_POINT('Ctrl Pts',(31.5353830964004,584.757084541308,-49.5221601717531)) ;
#68370=CARTESIAN_POINT('Ctrl Pts',(31.5403599433786,584.768001876211,-49.5221601717531)) ;
#68371=CARTESIAN_POINT('Ctrl Pts',(31.5689008468457,584.830609909557,-49.522160171753)) ;
#68372=CARTESIAN_POINT('Ctrl Pts',(31.5938812454169,584.894543521471,-49.5221601717529)) ;
#68373=CARTESIAN_POINT('Ctrl Pts',(31.6150780535725,584.959595021631,-49.5221601717529)) ;
#68374=CARTESIAN_POINT('Ctrl Pts',(31.6344250442579,585.018969563233,-49.522160171753)) ;
#68375=CARTESIAN_POINT('Ctrl Pts',(31.6506197270796,585.079276003087,-49.5221601717531)) ;
#68376=CARTESIAN_POINT('Ctrl Pts',(31.6634548036038,585.140361228952,-49.522160171753)) ;
#68377=CARTESIAN_POINT('Ctrl Pts',(31.6785404513754,585.212157466372,-49.522160171753)) ;
#68378=CARTESIAN_POINT('Ctrl Pts',(31.6889855555218,585.285031068209,-49.522160171753)) ;
#68379=CARTESIAN_POINT('Ctrl Pts',(31.6948651281539,585.358560609028,-49.522160171753)) ;
#68380=CARTESIAN_POINT('Ctrl Pts',(31.6961694101108,585.374871871663,-49.522160171753)) ;
#68381=CARTESIAN_POINT('Ctrl Pts',(31.6972487956621,585.391215328875,-49.522160171753)) ;
#68382=CARTESIAN_POINT('Ctrl Pts',(31.698103724415,585.407586209828,-49.522160171753)) ;
#68383=CARTESIAN_POINT('Ctrl Pts',(31.6989406415282,585.423612189046,-49.522160171753)) ;
#68384=CARTESIAN_POINT('Ctrl Pts',(31.6995624570579,585.4396697465,-49.522160171753)) ;
#68385=CARTESIAN_POINT('Ctrl Pts',(31.6999690832809,585.455723162103,-49.522160171753)) ;
#68386=CARTESIAN_POINT('Ctrl Pts',(31.7017073058113,585.524347385327,-49.522160171753)) ;
#68387=CARTESIAN_POINT('Ctrl Pts',(31.6995250570887,585.592990128663,-49.522160171753)) ;
#68388=CARTESIAN_POINT('Ctrl Pts',(31.6935434789382,585.661314289035,-49.522160171753)) ;
#68389=CARTESIAN_POINT('Ctrl Pts',(31.6875769121955,585.729466982645,-49.522160171753)) ;
#68390=CARTESIAN_POINT('Ctrl Pts',(31.6778295899244,585.797303747662,-49.522160171753)) ;
#68391=CARTESIAN_POINT('Ctrl Pts',(31.6643723151243,585.864474977224,-49.522160171753)) ;
#68392=CARTESIAN_POINT('Ctrl Pts',(31.6545223425228,585.913640560942,-49.5221601717531)) ;
#68393=CARTESIAN_POINT('Ctrl Pts',(31.642683744479,585.9624493375,-49.522160171753)) ;
#68394=CARTESIAN_POINT('Ctrl Pts',(31.628869585479,586.01075422025,-49.522160171753)) ;
#68395=CARTESIAN_POINT('Ctrl Pts',(31.6231571947481,586.030729114449,-49.522160171753)) ;
#68396=CARTESIAN_POINT('Ctrl Pts',(31.617106852988,586.050617722158,-49.522160171753)) ;
#68397=CARTESIAN_POINT('Ctrl Pts',(31.6107189261506,586.070409070264,-49.522160171753)) ;
#68398=CARTESIAN_POINT('Ctrl Pts',(31.6059788613649,586.08509494169,-49.522160171753)) ;
#68399=CARTESIAN_POINT('Ctrl Pts',(31.6010529102216,586.099727253392,-49.5221601717529)) ;
#68400=CARTESIAN_POINT('Ctrl Pts',(31.5959411138607,586.11430138426,-49.522160171753)) ;
#68401=CARTESIAN_POINT('Ctrl Pts',(31.5916380395207,586.126569785451,-49.522160171753)) ;
#68402=CARTESIAN_POINT('Ctrl Pts',(31.5872060372536,586.138788991967,-49.522160171753)) ;
#68403=CARTESIAN_POINT('Ctrl Pts',(31.5826469038171,586.150953071513,-49.522160171753)) ;
#68404=CARTESIAN_POINT('Ctrl Pts',(31.5595365757891,586.212613005881,-49.522160171753)) ;
#68405=CARTESIAN_POINT('Ctrl Pts',(31.5331524711879,586.272888155243,-49.5221601717529)) ;
#68406=CARTESIAN_POINT('Ctrl Pts',(31.5035447956668,586.33144636608,-49.5221601717529)) ;
#68407=CARTESIAN_POINT('Ctrl Pts',(31.4825817796702,586.372907125458,-49.522160171753)) ;
#68408=CARTESIAN_POINT('Ctrl Pts',(31.4600019247098,586.413506657349,-49.5221601717529)) ;
#68409=CARTESIAN_POINT('Ctrl Pts',(31.4358124034094,586.453115472938,-49.5221601717529)) ;
#68410=CARTESIAN_POINT('Ctrl Pts',(31.4280853247628,586.465768076904,-49.5221601717529)) ;
#68411=CARTESIAN_POINT('Ctrl Pts',(31.4201927015562,586.478321394194,-49.5221601717531)) ;
#68412=CARTESIAN_POINT('Ctrl Pts',(31.4121385580784,586.490764858801,-49.5221601717531)) ;
#68413=CARTESIAN_POINT('Ctrl Pts',(31.3778747803058,586.543701599648,-49.522160171753)) ;
#68414=CARTESIAN_POINT('Ctrl Pts',(31.3407548909434,586.594555512031,-49.5221601717529)) ;
#68415=CARTESIAN_POINT('Ctrl Pts',(31.3008131347297,586.643013002544,-49.522160171753)) ;
#68416=CARTESIAN_POINT('Ctrl Pts',(31.2636035879197,586.688155766219,-49.522160171753)) ;
#68417=CARTESIAN_POINT('Ctrl Pts',(31.2239444633598,586.731218909947,-49.5221601717528)) ;
#68418=CARTESIAN_POINT('Ctrl Pts',(31.1818411981515,586.771914720393,-49.5221601717528)) ;
#68419=CARTESIAN_POINT('Ctrl Pts',(31.1746523415314,586.778863263336,-49.5221601717528)) ;
#68420=CARTESIAN_POINT('Ctrl Pts',(31.1673921843832,586.785742701195,-49.522160171753)) ;
#68421=CARTESIAN_POINT('Ctrl Pts',(31.1600619605025,586.792552516318,-49.522160171753)) ;
#68422=CARTESIAN_POINT('Ctrl Pts',(28.6224074890457,586.788253409867,-49.5202805469744)) ;
#68423=CARTESIAN_POINT('Ctrl Pts',(28.2636244773615,586.366765387965,-49.4831921864647)) ;
#68424=CARTESIAN_POINT('Ctrl Pts',(28.0084321078388,585.14263785445,-49.4090297440025)) ;
#68425=CARTESIAN_POINT('Ctrl Pts',(29.3472570216431,583.819251769591,-49.297793219588)) ;
#68426=CARTESIAN_POINT('Ctrl Pts',(31.1844866118933,584.231809776485,-49.1865709737307)) ;
#68427=CARTESIAN_POINT('Ctrl Pts',(31.8334585912461,585.998161231894,-49.0753487278734)) ;
#68428=CARTESIAN_POINT('Ctrl Pts',(30.7002431513819,587.50135539588,-48.9641264820159)) ;
#68429=CARTESIAN_POINT('Ctrl Pts',(28.822941880499,587.362809908455,-48.8529042361585)) ;
#68430=CARTESIAN_POINT('Ctrl Pts',(27.9224434628909,585.709934174676,-48.7416819903011)) ;
#68431=CARTESIAN_POINT('Ctrl Pts',(28.8240101900071,584.057569634295,-48.6304597444437)) ;
#68432=CARTESIAN_POINT('Ctrl Pts',(30.7013185437651,583.920331685552,-48.5192374985864)) ;
#68433=CARTESIAN_POINT('Ctrl Pts',(31.8336328053599,585.423981994271,-48.4080152527291)) ;
#68434=CARTESIAN_POINT('Ctrl Pts',(31.1831024500014,587.190308717922,-48.2967930068717)) ;
#68435=CARTESIAN_POINT('Ctrl Pts',(29.3459859094712,587.600337651261,-48.1855707610142)) ;
#68436=CARTESIAN_POINT('Ctrl Pts',(28.0061704677458,586.27820841406,-48.0743485151568)) ;
#68437=CARTESIAN_POINT('Ctrl Pts',(28.3916973927331,584.435855412722,-47.9631262692994)) ;
#68438=CARTESIAN_POINT('Ctrl Pts',(30.1492683457755,583.761763980669,-47.8519040234422)) ;
#68439=CARTESIAN_POINT('Ctrl Pts',(31.6678667421111,584.874251660798,-47.7406817775848)) ;
#68440=CARTESIAN_POINT('Ctrl Pts',(31.5559056918524,586.752715612336,-47.6294595317275)) ;
#68441=CARTESIAN_POINT('Ctrl Pts',(29.9157317041138,587.677618832294,-47.51823728587)) ;
#68442=CARTESIAN_POINT('Ctrl Pts',(28.2520962180047,586.796586291543,-47.4069992157278)) ;
#68443=CARTESIAN_POINT('Ctrl Pts',(28.1434121707751,585.550835925276,-47.3328352275381)) ;
#68444=CARTESIAN_POINT('Ctrl Pts',(28.3654201435781,585.043770024595,-47.2957453213009)) ;
#68445=CARTESIAN_POINT('Ctrl Pts',(28.5208652057457,586.874683537923,-49.5972675643953)) ;
#68446=CARTESIAN_POINT('Ctrl Pts',(28.1333079528429,586.419392360303,-49.5601792038856)) ;
#68447=CARTESIAN_POINT('Ctrl Pts',(27.8576492664693,585.09709033194,-49.4860167614234)) ;
#68448=CARTESIAN_POINT('Ctrl Pts',(29.3038473550471,583.667569259663,-49.3747802370089)) ;
#68449=CARTESIAN_POINT('Ctrl Pts',(31.2884219579716,584.113214238963,-49.2635579911516)) ;
#68450=CARTESIAN_POINT('Ctrl Pts',(31.9894412073173,586.021226311511,-49.1523357452942)) ;
#68451=CARTESIAN_POINT('Ctrl Pts',(30.7653423829074,587.644975992522,-49.0411134994368)) ;
#68452=CARTESIAN_POINT('Ctrl Pts',(28.7374823680225,587.49531921737,-48.9298912535793)) ;
#68453=CARTESIAN_POINT('Ctrl Pts',(27.7647643696611,585.709883569883,-48.8186690077219)) ;
#68454=CARTESIAN_POINT('Ctrl Pts',(28.7386363554878,583.925000113285,-48.7074467618646)) ;
#68455=CARTESIAN_POINT('Ctrl Pts',(30.7665040212914,583.776755740845,-48.5962245160073)) ;
#68456=CARTESIAN_POINT('Ctrl Pts',(31.9896293933272,585.400998149198,-48.48500227015)) ;
#68457=CARTESIAN_POINT('Ctrl Pts',(31.2869267868988,587.308983506512,-48.3737800242926)) ;
#68458=CARTESIAN_POINT('Ctrl Pts',(29.3024743002329,587.751896581659,-48.2625577784351)) ;
#68459=CARTESIAN_POINT('Ctrl Pts',(27.8552062438262,586.323733155674,-48.1513355325777)) ;
#68460=CARTESIAN_POINT('Ctrl Pts',(28.2716522602271,584.333624246324,-48.0401132867203)) ;
#68461=CARTESIAN_POINT('Ctrl Pts',(30.170179637946,583.605470975117,-47.9288910408631)) ;
#68462=CARTESIAN_POINT('Ctrl Pts',(31.8105689640286,584.807179682491,-47.8176687950058)) ;
#68463=CARTESIAN_POINT('Ctrl Pts',(31.6896286863195,586.836295624513,-47.7064465491484)) ;
#68464=CARTESIAN_POINT('Ctrl Pts',(29.9179134593728,587.83537567974,-47.5952243032909)) ;
#68465=CARTESIAN_POINT('Ctrl Pts',(28.1208551321083,586.883684713078,-47.4839862331486)) ;
#68466=CARTESIAN_POINT('Ctrl Pts',(28.0034546716436,585.538025710199,-47.409822244959)) ;
#68467=CARTESIAN_POINT('Ctrl Pts',(28.2432675871385,584.990293345207,-47.3727323387218)) ;
#68468=CARTESIAN_POINT('Ctrl Pts',(28.4193229224455,586.961113665978,-49.6742545818162)) ;
#68469=CARTESIAN_POINT('Ctrl Pts',(28.0029914283242,586.472019332639,-49.6371662213065)) ;
#68470=CARTESIAN_POINT('Ctrl Pts',(27.7068664251,585.051542809432,-49.5630037788443)) ;
#68471=CARTESIAN_POINT('Ctrl Pts',(29.2604376884511,583.515886749735,-49.4517672544297)) ;
#68472=CARTESIAN_POINT('Ctrl Pts',(31.3923573040497,583.99461870144,-49.3405450085725)) ;
#68473=CARTESIAN_POINT('Ctrl Pts',(32.1454238233885,586.044291391129,-49.2293227627151)) ;
#68474=CARTESIAN_POINT('Ctrl Pts',(30.8304416144329,587.788596589164,-49.1181005168577)) ;
#68475=CARTESIAN_POINT('Ctrl Pts',(28.652022855546,587.627828526282,-49.0068782710002)) ;
#68476=CARTESIAN_POINT('Ctrl Pts',(27.6070852764312,585.70983296509,-48.8956560251428)) ;
#68477=CARTESIAN_POINT('Ctrl Pts',(28.6532625209683,583.792430592273,-48.7844337792855)) ;
#68478=CARTESIAN_POINT('Ctrl Pts',(30.8316894988174,583.633179796137,-48.6732115334282)) ;
#68479=CARTESIAN_POINT('Ctrl Pts',(32.1456259812944,585.378014304122,-48.5619892875709)) ;
#68480=CARTESIAN_POINT('Ctrl Pts',(31.3907511237965,587.4276582951,-48.4507670417135)) ;
#68481=CARTESIAN_POINT('Ctrl Pts',(29.2589626909946,587.903455512057,-48.339544795856)) ;
#68482=CARTESIAN_POINT('Ctrl Pts',(27.7042420199065,586.369257897288,-48.2283225499986)) ;
#68483=CARTESIAN_POINT('Ctrl Pts',(28.1516071277209,584.231393079927,-48.1171003041412)) ;
#68484=CARTESIAN_POINT('Ctrl Pts',(30.1910909301166,583.449177969564,-48.0058780582839)) ;
#68485=CARTESIAN_POINT('Ctrl Pts',(31.9532711859459,584.740107704183,-47.8946558124267)) ;
#68486=CARTESIAN_POINT('Ctrl Pts',(31.8233516807864,586.91987563669,-47.7834335665693)) ;
#68487=CARTESIAN_POINT('Ctrl Pts',(29.9200952146318,587.993132527187,-47.6722113207118)) ;
#68488=CARTESIAN_POINT('Ctrl Pts',(27.9896140462121,586.970783134613,-47.5609732505695)) ;
#68489=CARTESIAN_POINT('Ctrl Pts',(27.863497172512,585.525215495121,-47.4868092623798)) ;
#68490=CARTESIAN_POINT('Ctrl Pts',(28.1211150306988,584.936816665818,-47.4497193561427)) ;
#68491=CARTESIAN_POINT('Ctrl Pts',(28.3177806391455,587.047543794034,-49.7512415992371)) ;
#68492=CARTESIAN_POINT('Ctrl Pts',(27.8726749038054,586.524646304977,-49.7141532387274)) ;
#68493=CARTESIAN_POINT('Ctrl Pts',(27.5560835837305,585.005995286921,-49.6399907962651)) ;
#68494=CARTESIAN_POINT('Ctrl Pts',(29.2170280218552,583.364204239807,-49.5287542718506)) ;
#68495=CARTESIAN_POINT('Ctrl Pts',(31.4962926501278,583.876023163918,-49.4175320259934)) ;
#68496=CARTESIAN_POINT('Ctrl Pts',(32.3014064394596,586.067356470747,-49.306309780136)) ;
#68497=CARTESIAN_POINT('Ctrl Pts',(30.8955408459586,587.932217185805,-49.1950875342786)) ;
#68498=CARTESIAN_POINT('Ctrl Pts',(28.5665633430695,587.760337835196,-49.0838652884211)) ;
#68499=CARTESIAN_POINT('Ctrl Pts',(27.4494061832013,585.709782360297,-48.9726430425637)) ;
#68500=CARTESIAN_POINT('Ctrl Pts',(28.567888686449,583.659861071261,-48.8614207967064)) ;
#68501=CARTESIAN_POINT('Ctrl Pts',(30.8968749763436,583.489603851428,-48.7501985508491)) ;
#68502=CARTESIAN_POINT('Ctrl Pts',(32.3016225692617,585.355030459046,-48.6389763049918)) ;
#68503=CARTESIAN_POINT('Ctrl Pts',(31.4945754606939,587.546333083691,-48.5277540591344)) ;
#68504=CARTESIAN_POINT('Ctrl Pts',(29.2154510817562,588.055014442455,-48.4165318132769)) ;
#68505=CARTESIAN_POINT('Ctrl Pts',(27.5532777959871,586.414782638902,-48.3053095674195)) ;
#68506=CARTESIAN_POINT('Ctrl Pts',(28.0315619952149,584.129161913529,-48.1940873215621)) ;
#68507=CARTESIAN_POINT('Ctrl Pts',(30.2120022222872,583.292884964012,-48.0828650757048)) ;
#68508=CARTESIAN_POINT('Ctrl Pts',(32.0959734078635,584.673035725876,-47.9716428298476)) ;
#68509=CARTESIAN_POINT('Ctrl Pts',(31.9570746752535,587.003455648867,-47.8604205839902)) ;
#68510=CARTESIAN_POINT('Ctrl Pts',(29.9222769698908,588.150889374633,-47.7491983381327)) ;
#68511=CARTESIAN_POINT('Ctrl Pts',(27.8583729603156,587.057881556148,-47.6379602679904)) ;
#68512=CARTESIAN_POINT('Ctrl Pts',(27.7235396733805,585.512405280044,-47.5637962798008)) ;
#68513=CARTESIAN_POINT('Ctrl Pts',(27.9989624742593,584.88333998643,-47.5267063735636)) ;
#68514=CARTESIAN_POINT('',(29.9417003027147,587.377508131277,-47.5212921527489)) ;
#68515=CARTESIAN_POINT('Ctrl Pts',(28.0059001157518,584.887332980459,-47.522160171753)) ;
#68516=CARTESIAN_POINT('Ctrl Pts',(27.982867140185,584.957167490777,-47.522160171753)) ;
#68517=CARTESIAN_POINT('Ctrl Pts',(27.9639876910789,585.028114081953,-47.5221601717529)) ;
#68518=CARTESIAN_POINT('Ctrl Pts',(27.9491451721318,585.099835637674,-47.5221601717529)) ;
#68519=CARTESIAN_POINT('Ctrl Pts',(27.9339594575577,585.173215572568,-47.5221601717529)) ;
#68520=CARTESIAN_POINT('Ctrl Pts',(27.9229996253534,585.247407769229,-47.5221601717529)) ;
#68521=CARTESIAN_POINT('Ctrl Pts',(27.9161953558799,585.32205465925,-47.5221601717529)) ;
#68522=CARTESIAN_POINT('Ctrl Pts',(27.9104710901557,585.384853264689,-47.5221601717529)) ;
#68523=CARTESIAN_POINT('Ctrl Pts',(27.9076889433615,585.447974061067,-47.5221601717529)) ;
#68524=CARTESIAN_POINT('Ctrl Pts',(27.9078348642577,585.511197697194,-47.5221601717529)) ;
#68525=CARTESIAN_POINT('Ctrl Pts',(27.9078999515837,585.539398301253,-47.5221601717529)) ;
#68526=CARTESIAN_POINT('Ctrl Pts',(27.9085479212935,585.567619241939,-47.5221601717529)) ;
#68527=CARTESIAN_POINT('Ctrl Pts',(27.9097790499397,585.59584029347,-47.5221601717529)) ;
#68528=CARTESIAN_POINT('Ctrl Pts',(27.9104536758238,585.6113046821,-47.5221601717529)) ;
#68529=CARTESIAN_POINT('Ctrl Pts',(27.9113034257906,585.626769094357,-47.5221601717528)) ;
#68530=CARTESIAN_POINT('Ctrl Pts',(27.9123284599295,585.64223012412,-47.5221601717529)) ;
#68531=CARTESIAN_POINT('Ctrl Pts',(27.9132810635077,585.656598652656,-47.5221601717529)) ;
#68532=CARTESIAN_POINT('Ctrl Pts',(27.914385357136,585.670966437285,-47.5221601717529)) ;
#68533=CARTESIAN_POINT('Ctrl Pts',(27.9156392489812,585.685308412897,-47.5221601717529)) ;
#68534=CARTESIAN_POINT('Ctrl Pts',(27.9220137363149,585.758219599158,-47.5221601717529)) ;
#68535=CARTESIAN_POINT('Ctrl Pts',(27.9322573244265,585.830590171318,-47.5221601717529)) ;
#68536=CARTESIAN_POINT('Ctrl Pts',(27.9463005260323,585.902086531053,-47.5221601717529)) ;
#68537=CARTESIAN_POINT('Ctrl Pts',(27.9602626500392,585.973170110758,-47.5221601717529)) ;
#68538=CARTESIAN_POINT('Ctrl Pts',(27.9779810064621,586.043390504702,-47.5221601717529)) ;
#68539=CARTESIAN_POINT('Ctrl Pts',(27.9994343190645,586.112399884924,-47.5221601717528)) ;
#68540=CARTESIAN_POINT('Ctrl Pts',(28.0172796994433,586.169803543864,-47.5221601717528)) ;
#68541=CARTESIAN_POINT('Ctrl Pts',(28.0377103276275,586.22636917177,-47.5221601717529)) ;
#68542=CARTESIAN_POINT('Ctrl Pts',(28.0607363394367,586.281878854015,-47.5221601717529)) ;
#68543=CARTESIAN_POINT('Ctrl Pts',(28.070298843717,586.304931546703,-47.5221601717529)) ;
#68544=CARTESIAN_POINT('Ctrl Pts',(28.0803091959749,586.32780189582,-47.5221601717529)) ;
#68545=CARTESIAN_POINT('Ctrl Pts',(28.0907690720635,586.35047322507,-47.5221601717529)) ;
#68546=CARTESIAN_POINT('Ctrl Pts',(28.0956486353482,586.36104946755,-47.5221601717529)) ;
#68547=CARTESIAN_POINT('Ctrl Pts',(28.1006260339097,586.371582388587,-47.5221601717529)) ;
#68548=CARTESIAN_POINT('Ctrl Pts',(28.1057014773282,586.382070241986,-47.5221601717529)) ;
#68549=CARTESIAN_POINT('Ctrl Pts',(28.1109348689906,586.392884478302,-47.522160171753)) ;
#68550=CARTESIAN_POINT('Ctrl Pts',(28.1162688294438,586.403643148949,-47.5221601717528)) ;
#68551=CARTESIAN_POINT('Ctrl Pts',(28.1217013309573,586.414341049525,-47.5221601717528)) ;
#68552=CARTESIAN_POINT('Ctrl Pts',(28.1528552979291,586.475690694877,-47.5221601717528)) ;
#68553=CARTESIAN_POINT('Ctrl Pts',(28.1872655825553,586.535083110227,-47.522160171753)) ;
#68554=CARTESIAN_POINT('Ctrl Pts',(28.2249088976231,586.592214387545,-47.522160171753)) ;
#68555=CARTESIAN_POINT('Ctrl Pts',(28.2592671302627,586.644359893688,-47.5221601717529)) ;
#68556=CARTESIAN_POINT('Ctrl Pts',(28.2963193822463,586.694621855483,-47.5221601717527)) ;
#68557=CARTESIAN_POINT('Ctrl Pts',(28.3360751941218,586.742742736611,-47.5221601717528)) ;
#68558=CARTESIAN_POINT('Ctrl Pts',(28.3828020037815,586.799301391738,-47.5221601717529)) ;
#68559=CARTESIAN_POINT('Ctrl Pts',(28.4332644628052,586.852903649694,-47.5221601717529)) ;
#68560=CARTESIAN_POINT('Ctrl Pts',(28.487086318189,586.903345402823,-47.5221601717529)) ;
#68561=CARTESIAN_POINT('Ctrl Pts',(28.4990257703044,586.914535037439,-47.5221601717529)) ;
#68562=CARTESIAN_POINT('Ctrl Pts',(28.511130613787,586.925568913959,-47.5221601717527)) ;
#68563=CARTESIAN_POINT('Ctrl Pts',(28.5233968445569,586.936444401515,-47.5221601717528)) ;
#68564=CARTESIAN_POINT('Ctrl Pts',(28.5354046498584,586.94709076384,-47.522160171753)) ;
#68565=CARTESIAN_POINT('Ctrl Pts',(28.5475712576655,586.957588641698,-47.5221601717528)) ;
#68566=CARTESIAN_POINT('Ctrl Pts',(28.5598687955868,586.967915695398,-47.5221601717528)) ;
#68567=CARTESIAN_POINT('Ctrl Pts',(28.6123748171967,587.012008464876,-47.5221601717527)) ;
#68568=CARTESIAN_POINT('Ctrl Pts',(28.6673338270958,587.053054915024,-47.5221601717528)) ;
#68569=CARTESIAN_POINT('Ctrl Pts',(28.7244079349294,587.090940018963,-47.5221601717528)) ;
#68570=CARTESIAN_POINT('Ctrl Pts',(28.7814751479459,587.128820546206,-47.5221601717527)) ;
#68571=CARTESIAN_POINT('Ctrl Pts',(28.8406580638171,587.163540801281,-47.5221601717531)) ;
#68572=CARTESIAN_POINT('Ctrl Pts',(28.9016380545588,587.194937608893,-47.5221601717529)) ;
#68573=CARTESIAN_POINT('Ctrl Pts',(28.9462186128203,587.217890830006,-47.5221601717528)) ;
#68574=CARTESIAN_POINT('Ctrl Pts',(28.9917600957509,587.23906681561,-47.5221601717529)) ;
#68575=CARTESIAN_POINT('Ctrl Pts',(29.038139360794,587.258384072901,-47.5221601717529)) ;
#68576=CARTESIAN_POINT('Ctrl Pts',(29.0573179795054,587.26637208892,-47.5221601717529)) ;
#68577=CARTESIAN_POINT('Ctrl Pts',(29.0766398457555,587.274042085443,-47.5221601717531)) ;
#68578=CARTESIAN_POINT('Ctrl Pts',(29.0960961522501,587.281387506957,-47.5221601717531)) ;
#68579=CARTESIAN_POINT('Ctrl Pts',(29.110533411056,587.286838066212,-47.5221601717531)) ;
#68580=CARTESIAN_POINT('Ctrl Pts',(29.125044693437,587.292109899721,-47.522160171753)) ;
#68581=CARTESIAN_POINT('Ctrl Pts',(29.1396263608139,587.297200158435,-47.522160171753)) ;
#68582=CARTESIAN_POINT('Ctrl Pts',(29.1519011062021,587.30148510254,-47.5221601717531)) ;
#68583=CARTESIAN_POINT('Ctrl Pts',(29.1642177748965,587.305638574356,-47.522160171753)) ;
#68584=CARTESIAN_POINT('Ctrl Pts',(29.1765706085811,587.309658279919,-47.522160171753)) ;
#68585=CARTESIAN_POINT('Ctrl Pts',(29.2391873407233,587.330034238421,-47.5221601717529)) ;
#68586=CARTESIAN_POINT('Ctrl Pts',(29.3027625707403,587.34698725607,-47.5221601717527)) ;
#68587=CARTESIAN_POINT('Ctrl Pts',(29.3670053078069,587.360349490877,-47.5221601717528)) ;
#68588=CARTESIAN_POINT('Ctrl Pts',(29.412490861665,587.369810305885,-47.5221601717529)) ;
#68589=CARTESIAN_POINT('Ctrl Pts',(29.4583111633863,587.377470058772,-47.522160171753)) ;
#68590=CARTESIAN_POINT('Ctrl Pts',(29.5043605024696,587.38325362236,-47.5221601717531)) ;
#68591=CARTESIAN_POINT('Ctrl Pts',(29.519070461532,587.385101118661,-47.5221601717531)) ;
#68592=CARTESIAN_POINT('Ctrl Pts',(29.533806010492,587.386757282783,-47.5221601717531)) ;
#68593=CARTESIAN_POINT('Ctrl Pts',(29.5485563794087,587.388218673244,-47.522160171753)) ;
#68594=CARTESIAN_POINT('Ctrl Pts',(29.6113071063726,587.394435691563,-47.5221601717528)) ;
#68595=CARTESIAN_POINT('Ctrl Pts',(29.6742101689315,587.397121089668,-47.5221601717529)) ;
#68596=CARTESIAN_POINT('Ctrl Pts',(29.7369990386124,587.396106118865,-47.5221601717529)) ;
#68597=CARTESIAN_POINT('Ctrl Pts',(29.7954928462785,587.395160576969,-47.5221601717529)) ;
#68598=CARTESIAN_POINT('Ctrl Pts',(29.8538880283258,587.391003256213,-47.522160171753)) ;
#68599=CARTESIAN_POINT('Ctrl Pts',(29.911956251404,587.383459021148,-47.5221601717529)) ;
#68600=CARTESIAN_POINT('Ctrl Pts',(29.9218710199011,587.382170892457,-47.5221601717529)) ;
#68601=CARTESIAN_POINT('Ctrl Pts',(29.9317762150191,587.380783932454,-47.5221601717531)) ;
#68602=CARTESIAN_POINT('Ctrl Pts',(29.9416706627822,587.379298783007,-47.5221601717529)) ;
#68603=CARTESIAN_POINT('Ctrl Pts',(28.6194567455633,586.789923813611,-49.522160171753)) ;
#68604=CARTESIAN_POINT('Ctrl Pts',(28.5741848796632,586.747689967573,-49.5221601717529)) ;
#68605=CARTESIAN_POINT('Ctrl Pts',(28.5316464199738,586.702882011821,-49.522160171753)) ;
#68606=CARTESIAN_POINT('Ctrl Pts',(28.4918376792449,586.655846007778,-49.5221601717529)) ;
#68607=CARTESIAN_POINT('Ctrl Pts',(28.4493012350658,586.605587086654,-49.5221601717528)) ;
#68608=CARTESIAN_POINT('Ctrl Pts',(28.4098806731104,586.552784108491,-49.5221601717529)) ;
#68609=CARTESIAN_POINT('Ctrl Pts',(28.373600628434,586.497804127081,-49.5221601717529)) ;
#68610=CARTESIAN_POINT('Ctrl Pts',(28.3418555893421,586.449696643347,-49.522160171753)) ;
#68611=CARTESIAN_POINT('Ctrl Pts',(28.312515258461,586.399921153953,-49.5221601717529)) ;
#68612=CARTESIAN_POINT('Ctrl Pts',(28.2856192221846,586.348695779004,-49.5221601717528)) ;
#68613=CARTESIAN_POINT('Ctrl Pts',(28.2721028283307,586.322952865215,-49.5221601717528)) ;
#68614=CARTESIAN_POINT('Ctrl Pts',(28.2592041019405,586.296843425323,-49.5221601717528)) ;
#68615=CARTESIAN_POINT('Ctrl Pts',(28.2469304374914,586.270393277738,-49.5221601717528)) ;
#68616=CARTESIAN_POINT('Ctrl Pts',(28.2413787772024,586.25842926857,-49.5221601717528)) ;
#68617=CARTESIAN_POINT('Ctrl Pts',(28.2359545091969,586.246394057129,-49.5221601717529)) ;
#68618=CARTESIAN_POINT('Ctrl Pts',(28.2306666151602,586.234309569701,-49.5221601717529)) ;
#68619=CARTESIAN_POINT('Ctrl Pts',(28.2038251620089,586.172968476081,-49.5221601717528)) ;
#68620=CARTESIAN_POINT('Ctrl Pts',(28.1804420988066,586.11025046575,-49.5221601717529)) ;
#68621=CARTESIAN_POINT('Ctrl Pts',(28.1605384877892,586.046514903665,-49.5221601717529)) ;
#68622=CARTESIAN_POINT('Ctrl Pts',(28.1402140591507,585.981431794767,-49.5221601717529)) ;
#68623=CARTESIAN_POINT('Ctrl Pts',(28.123517190455,585.915286818455,-49.5221601717529)) ;
#68624=CARTESIAN_POINT('Ctrl Pts',(28.1105100613261,585.848425691796,-49.5221601717529)) ;
#68625=CARTESIAN_POINT('Ctrl Pts',(28.099669740957,585.792702708959,-49.5221601717529)) ;
#68626=CARTESIAN_POINT('Ctrl Pts',(28.0913928086545,585.736481350659,-49.5221601717529)) ;
#68627=CARTESIAN_POINT('Ctrl Pts',(28.0857400408894,585.679949476623,-49.5221601717529)) ;
#68628=CARTESIAN_POINT('Ctrl Pts',(28.0831191304622,585.653738426693,-49.5221601717529)) ;
#68629=CARTESIAN_POINT('Ctrl Pts',(28.0810626789015,585.627460510806,-49.5221601717529)) ;
#68630=CARTESIAN_POINT('Ctrl Pts',(28.0795785764974,585.601134047563,-49.5221601717529)) ;
#68631=CARTESIAN_POINT('Ctrl Pts',(28.078939400595,585.58979571885,-49.5221601717529)) ;
#68632=CARTESIAN_POINT('Ctrl Pts',(28.0784065214721,585.578448977045,-49.5221601717529)) ;
#68633=CARTESIAN_POINT('Ctrl Pts',(28.077980858293,585.567108767372,-49.5221601717529)) ;
#68634=CARTESIAN_POINT('Ctrl Pts',(28.0753463536225,585.496922204811,-49.5221601717529)) ;
#68635=CARTESIAN_POINT('Ctrl Pts',(28.0768069816538,585.426855163324,-49.5221601717529)) ;
#68636=CARTESIAN_POINT('Ctrl Pts',(28.0824149563513,585.357271018537,-49.5221601717529)) ;
#68637=CARTESIAN_POINT('Ctrl Pts',(28.0874572060543,585.294706429303,-49.5221601717529)) ;
#68638=CARTESIAN_POINT('Ctrl Pts',(28.0958525755181,585.232531249517,-49.5221601717529)) ;
#68639=CARTESIAN_POINT('Ctrl Pts',(28.107672820771,585.170997260696,-49.5221601717529)) ;
#68640=CARTESIAN_POINT('Ctrl Pts',(28.1204848067534,585.10430045489,-49.5221601717529)) ;
#68641=CARTESIAN_POINT('Ctrl Pts',(28.1373194403939,585.038356097394,-49.522160171753)) ;
#68642=CARTESIAN_POINT('Ctrl Pts',(28.1579325844387,584.973376371762,-49.522160171753)) ;
#68643=CARTESIAN_POINT('Ctrl Pts',(28.1658012165057,584.948571734891,-49.522160171753)) ;
#68644=CARTESIAN_POINT('Ctrl Pts',(28.1742209850587,584.923907710175,-49.5221601717529)) ;
#68645=CARTESIAN_POINT('Ctrl Pts',(28.1831802469027,584.899396416888,-49.5221601717529)) ;
#68646=CARTESIAN_POINT('Ctrl Pts',(28.1871260725044,584.888601187295,-49.5221601717529)) ;
#68647=CARTESIAN_POINT('Ctrl Pts',(28.1911762786592,584.877836578581,-49.5221601717529)) ;
#68648=CARTESIAN_POINT('Ctrl Pts',(28.195325017675,584.867115518396,-49.5221601717529)) ;
#68649=CARTESIAN_POINT('Ctrl Pts',(28.2208657004741,584.801113970358,-49.5221601717529)) ;
#68650=CARTESIAN_POINT('Ctrl Pts',(28.2501794469246,584.736642414895,-49.522160171753)) ;
#68651=CARTESIAN_POINT('Ctrl Pts',(28.2829439666236,584.673925582888,-49.522160171753)) ;
#68652=CARTESIAN_POINT('Ctrl Pts',(28.3157084863227,584.611208750882,-49.522160171753)) ;
#68653=CARTESIAN_POINT('Ctrl Pts',(28.351924280498,584.550245857175,-49.5221601717529)) ;
#68654=CARTESIAN_POINT('Ctrl Pts',(28.3913232488784,584.491265452053,-49.5221601717529)) ;
#68655=CARTESIAN_POINT('Ctrl Pts',(28.4214332043401,584.446190734508,-49.5221601717529)) ;
#68656=CARTESIAN_POINT('Ctrl Pts',(28.4534034533065,584.402273869669,-49.5221601717529)) ;
#68657=CARTESIAN_POINT('Ctrl Pts',(28.4871328972782,584.359622730065,-49.5221601717528)) ;
#68658=CARTESIAN_POINT('Ctrl Pts',(28.5080342503109,584.333192809463,-49.5221601717528)) ;
#68659=CARTESIAN_POINT('Ctrl Pts',(28.5296114389798,584.307249043923,-49.522160171753)) ;
#68660=CARTESIAN_POINT('Ctrl Pts',(28.5518431286008,584.28181868143,-49.522160171753)) ;
#68661=CARTESIAN_POINT('Ctrl Pts',(28.5603428315767,584.272096049842,-49.522160171753)) ;
#68662=CARTESIAN_POINT('Ctrl Pts',(28.5689397661541,584.262446785189,-49.522160171753)) ;
#68663=CARTESIAN_POINT('Ctrl Pts',(28.577627784156,584.252877990672,-49.522160171753)) ;
#68664=CARTESIAN_POINT('Ctrl Pts',(28.6292044653751,584.196072553074,-49.5221601717531)) ;
#68665=CARTESIAN_POINT('Ctrl Pts',(28.6838606950433,584.142237698305,-49.5221601717529)) ;
#68666=CARTESIAN_POINT('Ctrl Pts',(28.7412855049599,584.091654439445,-49.5221601717529)) ;
#68667=CARTESIAN_POINT('Ctrl Pts',(28.7843541123974,584.0537169953,-49.522160171753)) ;
#68668=CARTESIAN_POINT('Ctrl Pts',(28.8289813491942,584.017608759369,-49.522160171753)) ;
#68669=CARTESIAN_POINT('Ctrl Pts',(28.8750546423904,583.983458791694,-49.522160171753)) ;
#68670=CARTESIAN_POINT('Ctrl Pts',(28.8914058161742,583.971339144553,-49.522160171753)) ;
#68671=CARTESIAN_POINT('Ctrl Pts',(28.9079392531401,583.959466246145,-49.5221601717529)) ;
#68672=CARTESIAN_POINT('Ctrl Pts',(28.9246503345323,583.947846242436,-49.5221601717531)) ;
#68673=CARTESIAN_POINT('Ctrl Pts',(28.9373060740742,583.939046109341,-49.5221601717531)) ;
#68674=CARTESIAN_POINT('Ctrl Pts',(28.9500595592467,583.93039398515,-49.5221601717528)) ;
#68675=CARTESIAN_POINT('Ctrl Pts',(28.9629018175317,583.921896637889,-49.5221601717528)) ;
#68676=CARTESIAN_POINT('Ctrl Pts',(29.0257081415723,583.880339527472,-49.5221601717527)) ;
#68677=CARTESIAN_POINT('Ctrl Pts',(29.0906820453539,583.842448662337,-49.5221601717529)) ;
#68678=CARTESIAN_POINT('Ctrl Pts',(29.1575622067351,583.808500383244,-49.522160171753)) ;
#68679=CARTESIAN_POINT('Ctrl Pts',(29.2115914739247,583.78107520059,-49.522160171753)) ;
#68680=CARTESIAN_POINT('Ctrl Pts',(29.2668657935751,583.756223325128,-49.522160171753)) ;
#68681=CARTESIAN_POINT('Ctrl Pts',(29.3232642411662,583.734108789472,-49.5221601717531)) ;
#68682=CARTESIAN_POINT('Ctrl Pts',(29.3337596629877,583.729993403499,-49.5221601717531)) ;
#68683=CARTESIAN_POINT('Ctrl Pts',(29.3442940503372,583.725972868921,-49.522160171753)) ;
#68684=CARTESIAN_POINT('Ctrl Pts',(29.3548662403592,583.722046833005,-49.5221601717529)) ;
#68685=CARTESIAN_POINT('Ctrl Pts',(29.9416432077809,587.375718227073,-47.5212921527489)) ;
#68686=CARTESIAN_POINT('Ctrl Pts',(29.9492394590292,587.375475919433,-47.5215814924169)) ;
#68687=CARTESIAN_POINT('Ctrl Pts',(29.9568340521747,587.375181631047,-47.521870832085)) ;
#68688=CARTESIAN_POINT('Ctrl Pts',(29.9644262760118,587.374835389473,-47.522160171753)) ;
#68689=CARTESIAN_POINT('Origin',(212.388527625401,504.21056516053,-49.5221601717613)) ;
#68690=CARTESIAN_POINT('',(184.88852762542,611.385991641078,-49.52216017176)) ;
#68691=CARTESIAN_POINT('',(182.13852762542,609.798278400806,-49.5221601717599)) ;
#68692=CARTESIAN_POINT('',(171.996867127016,603.942987982024,-49.5221601717594)) ;
#68693=CARTESIAN_POINT('',(182.13852762542,606.622851920264,-49.5221601717599)) ;
#68694=CARTESIAN_POINT('',(182.13852762542,557.004421780668,-49.5221601717599)) ;
#68695=CARTESIAN_POINT('',(184.88852762542,605.035138679992,-49.52216017176)) ;
#68696=CARTESIAN_POINT('',(215.655188123809,587.271998959181,-49.5221601717614)) ;
#68697=CARTESIAN_POINT('',(187.63852762542,606.622851920264,-49.5221601717601)) ;
#68698=CARTESIAN_POINT('',(173.371867127016,598.385991641073,-49.5221601717595)) ;
#68699=CARTESIAN_POINT('',(187.63852762542,609.798278400806,-49.5221601717601)) ;
#68700=CARTESIAN_POINT('',(187.63852762542,555.416708540397,-49.5221601717601)) ;
#68701=CARTESIAN_POINT('',(219.780188123809,591.24128205986,-49.5221601717616)) ;
#68702=CARTESIAN_POINT('',(7.38852762541949,611.385991641109,-49.5221601717519)) ;
#68703=CARTESIAN_POINT('',(4.63852762541949,609.798278400838,-49.5221601717518)) ;
#68704=CARTESIAN_POINT('',(61.0593671270093,642.372865274985,-49.5221601717544)) ;
#68705=CARTESIAN_POINT('',(4.63852762541949,606.622851920295,-49.5221601717518)) ;
#68706=CARTESIAN_POINT('',(4.63852762541951,557.004421780684,-49.5221601717518)) ;
#68707=CARTESIAN_POINT('',(7.38852762541949,605.035138680023,-49.5221601717519)) ;
#68708=CARTESIAN_POINT('',(104.717688123816,548.842121666274,-49.5221601717564)) ;
#68709=CARTESIAN_POINT('',(10.1385276254195,606.622851920295,-49.522160171752)) ;
#68710=CARTESIAN_POINT('',(62.4343671270093,636.815868934035,-49.5221601717544)) ;
#68711=CARTESIAN_POINT('',(10.1385276254195,609.798278400838,-49.522160171752)) ;
#68712=CARTESIAN_POINT('',(10.1385276254195,555.416708540412,-49.5221601717521)) ;
#68713=CARTESIAN_POINT('',(108.842688123816,552.811404766952,-49.5221601717565)) ;
#68714=CARTESIAN_POINT('',(7.38852762540283,516.385991641109,-49.5221601717519)) ;
#68715=CARTESIAN_POINT('',(4.63852762540283,514.798278400837,-49.5221601717518)) ;
#68716=CARTESIAN_POINT('',(81.6274704668794,559.247865274989,-49.5221601717553)) ;
#68717=CARTESIAN_POINT('',(4.63852762540283,511.622851920295,-49.5221601717518)) ;
#68718=CARTESIAN_POINT('',(4.63852762540284,509.504421780684,-49.5221601717518)) ;
#68719=CARTESIAN_POINT('',(7.38852762540283,510.035138680023,-49.5221601717519)) ;
#68720=CARTESIAN_POINT('',(84.149584783925,465.71712166627,-49.5221601717554)) ;
#68721=CARTESIAN_POINT('',(10.1385276254028,511.622851920295,-49.5221601717521)) ;
#68722=CARTESIAN_POINT('',(83.0024704668793,553.690868934039,-49.5221601717554)) ;
#68723=CARTESIAN_POINT('',(10.1385276254028,514.798278400837,-49.5221601717521)) ;
#68724=CARTESIAN_POINT('',(10.1385276254028,507.916708540412,-49.5221601717521)) ;
#68725=CARTESIAN_POINT('',(88.274584783925,469.686404766949,-49.5221601717556)) ;
#68726=CARTESIAN_POINT('Ctrl Pts',(178.619456745563,586.789923813584,-49.5221601717599)) ;
#68727=CARTESIAN_POINT('Ctrl Pts',(178.574188300298,586.747693158636,-49.5221601717599)) ;
#68728=CARTESIAN_POINT('Ctrl Pts',(178.531653457537,586.702888053417,-49.5221601717598)) ;
#68729=CARTESIAN_POINT('Ctrl Pts',(178.491848419612,586.655854613672,-49.5221601717598)) ;
#68730=CARTESIAN_POINT('Ctrl Pts',(178.449312342082,586.605594190776,-49.5221601717598)) ;
#68731=CARTESIAN_POINT('Ctrl Pts',(178.409892770719,586.552788955222,-49.5221601717599)) ;
#68732=CARTESIAN_POINT('Ctrl Pts',(178.373614216098,586.497806119515,-49.5221601717597)) ;
#68733=CARTESIAN_POINT('Ctrl Pts',(178.341870480804,586.449696138271,-49.5221601717596)) ;
#68734=CARTESIAN_POINT('Ctrl Pts',(178.312531836416,586.399917693953,-49.5221601717595)) ;
#68735=CARTESIAN_POINT('Ctrl Pts',(178.285637791918,586.348689004949,-49.5221601717596)) ;
#68736=CARTESIAN_POINT('Ctrl Pts',(178.272123794534,586.322947083936,-49.5221601717597)) ;
#68737=CARTESIAN_POINT('Ctrl Pts',(178.259227414255,586.296838621709,-49.5221601717596)) ;
#68738=CARTESIAN_POINT('Ctrl Pts',(178.246956033732,586.27038944072,-49.5221601717597)) ;
#68739=CARTESIAN_POINT('Ctrl Pts',(178.241402994952,586.258420670992,-49.5221601717597)) ;
#68740=CARTESIAN_POINT('Ctrl Pts',(178.235977443094,586.246380627231,-49.5221601717596)) ;
#68741=CARTESIAN_POINT('Ctrl Pts',(178.230688367278,586.234291259783,-49.5221601717597)) ;
#68742=CARTESIAN_POINT('Ctrl Pts',(178.203851554736,586.172949713692,-49.5221601717599)) ;
#68743=CARTESIAN_POINT('Ctrl Pts',(178.180473003136,586.11023107781,-49.5221601717597)) ;
#68744=CARTESIAN_POINT('Ctrl Pts',(178.160573650426,586.046494799319,-49.5221601717599)) ;
#68745=CARTESIAN_POINT('Ctrl Pts',(178.140312058258,585.98159829239,-49.52216017176)) ;
#68746=CARTESIAN_POINT('Ctrl Pts',(178.123656932244,585.915645914293,-49.52216017176)) ;
#68747=CARTESIAN_POINT('Ctrl Pts',(178.110669719504,585.848980531874,-49.5221601717598)) ;
#68748=CARTESIAN_POINT('Ctrl Pts',(178.099775969142,585.793061217362,-49.5221601717596)) ;
#68749=CARTESIAN_POINT('Ctrl Pts',(178.091463494471,585.736639290757,-49.5221601717596)) ;
#68750=CARTESIAN_POINT('Ctrl Pts',(178.085793601831,585.679904697295,-49.5221601717596)) ;
#68751=CARTESIAN_POINT('Ctrl Pts',(178.083174326351,585.653695465663,-49.5221601717595)) ;
#68752=CARTESIAN_POINT('Ctrl Pts',(178.081119341285,585.627419393335,-49.5221601717596)) ;
#68753=CARTESIAN_POINT('Ctrl Pts',(178.079636526497,585.601094799355,-49.5221601717597)) ;
#68754=CARTESIAN_POINT('Ctrl Pts',(178.078997639764,585.589752564316,-49.5221601717597)) ;
#68755=CARTESIAN_POINT('Ctrl Pts',(178.078465104061,585.578401896586,-49.5221601717596)) ;
#68756=CARTESIAN_POINT('Ctrl Pts',(178.078039839316,585.567057770085,-49.5221601717596)) ;
#68757=CARTESIAN_POINT('Ctrl Pts',(178.075408552685,585.496867027165,-49.5221601717596)) ;
#68758=CARTESIAN_POINT('Ctrl Pts',(178.076872157339,585.426795955192,-49.5221601717597)) ;
#68759=CARTESIAN_POINT('Ctrl Pts',(178.082482737992,585.357208068564,-49.5221601717599)) ;
#68760=CARTESIAN_POINT('Ctrl Pts',(178.087527938951,585.294632571642,-49.52216017176)) ;
#68761=CARTESIAN_POINT('Ctrl Pts',(178.095926768028,585.232446811339,-49.5221601717598)) ;
#68762=CARTESIAN_POINT('Ctrl Pts',(178.107750914516,585.170902758999,-49.5221601717598)) ;
#68763=CARTESIAN_POINT('Ctrl Pts',(178.120565934992,585.104201260358,-49.5221601717598)) ;
#68764=CARTESIAN_POINT('Ctrl Pts',(178.137403372988,585.03825267637,-49.5221601717599)) ;
#68765=CARTESIAN_POINT('Ctrl Pts',(178.158019131495,584.973269147845,-49.5221601717598)) ;
#68766=CARTESIAN_POINT('Ctrl Pts',(178.165888242172,584.948464696534,-49.5221601717597)) ;
#68767=CARTESIAN_POINT('Ctrl Pts',(178.174308388922,584.923800900598,-49.5221601717596)) ;
#68768=CARTESIAN_POINT('Ctrl Pts',(178.18326793304,584.89928987474,-49.5221601717596)) ;
#68769=CARTESIAN_POINT('Ctrl Pts',(178.187213992827,584.888494462361,-49.5221601717596)) ;
#68770=CARTESIAN_POINT('Ctrl Pts',(178.191264420398,584.877729679907,-49.52216017176)) ;
#68771=CARTESIAN_POINT('Ctrl Pts',(178.19541336821,584.86700845477,-49.52216017176)) ;
#68772=CARTESIAN_POINT('Ctrl Pts',(178.220666969342,584.801751055667,-49.5221601717596)) ;
#68773=CARTESIAN_POINT('Ctrl Pts',(178.249608559619,584.737989620282,-49.5221601717598)) ;
#68774=CARTESIAN_POINT('Ctrl Pts',(178.28192640687,584.67594128411,-49.5221601717598)) ;
#68775=CARTESIAN_POINT('Ctrl Pts',(178.314984652773,584.612471426755,-49.5221601717598)) ;
#68776=CARTESIAN_POINT('Ctrl Pts',(178.351575930346,584.550793244105,-49.5221601717599)) ;
#68777=CARTESIAN_POINT('Ctrl Pts',(178.39142267349,584.491143041426,-49.5221601717599)) ;
#68778=CARTESIAN_POINT('Ctrl Pts',(178.421531675276,584.446070146698,-49.5221601717599)) ;
#68779=CARTESIAN_POINT('Ctrl Pts',(178.453500638765,584.40215513963,-49.5221601717599)) ;
#68780=CARTESIAN_POINT('Ctrl Pts',(178.487228506351,584.359505850618,-49.5221601717599)) ;
#68781=CARTESIAN_POINT('Ctrl Pts',(178.508128949918,584.333076991578,-49.5221601717599)) ;
#68782=CARTESIAN_POINT('Ctrl Pts',(178.529705121679,584.30713428798,-49.5221601717597)) ;
#68783=CARTESIAN_POINT('Ctrl Pts',(178.551935695738,584.281704977885,-49.5221601717598)) ;
#68784=CARTESIAN_POINT('Ctrl Pts',(178.560436077436,584.271981484396,-49.5221601717599)) ;
#68785=CARTESIAN_POINT('Ctrl Pts',(178.569033700254,584.262331376981,-49.5221601717599)) ;
#68786=CARTESIAN_POINT('Ctrl Pts',(178.577722419645,584.252761755006,-49.5221601717599)) ;
#68787=CARTESIAN_POINT('Ctrl Pts',(178.629299529824,584.195955518691,-49.52216017176)) ;
#68788=CARTESIAN_POINT('Ctrl Pts',(178.683956074342,584.142120120314,-49.52216017176)) ;
#68789=CARTESIAN_POINT('Ctrl Pts',(178.741381145388,584.091536509087,-49.5221601717598)) ;
#68790=CARTESIAN_POINT('Ctrl Pts',(178.784449948673,584.053598800666,-49.5221601717597)) ;
#68791=CARTESIAN_POINT('Ctrl Pts',(178.829077351025,584.017490408156,-49.5221601717598)) ;
#68792=CARTESIAN_POINT('Ctrl Pts',(178.875150804438,583.983340366146,-49.5221601717598)) ;
#68793=CARTESIAN_POINT('Ctrl Pts',(178.891493617505,583.971226931804,-49.5221601717598)) ;
#68794=CARTESIAN_POINT('Ctrl Pts',(178.908018505489,583.959360002586,-49.5221601717597)) ;
#68795=CARTESIAN_POINT('Ctrl Pts',(178.924720857825,583.947745713805,-49.5221601717597)) ;
#68796=CARTESIAN_POINT('Ctrl Pts',(178.937371839859,583.938948620093,-49.5221601717597)) ;
#68797=CARTESIAN_POINT('Ctrl Pts',(178.950120518772,583.930299415061,-49.5221601717595)) ;
#68798=CARTESIAN_POINT('Ctrl Pts',(178.962957900953,583.921804880912,-49.5221601717595)) ;
#68799=CARTESIAN_POINT('Ctrl Pts',(179.025763082393,583.880246504684,-49.5221601717595)) ;
#68800=CARTESIAN_POINT('Ctrl Pts',(179.090735890326,583.842354383869,-49.5221601717597)) ;
#68801=CARTESIAN_POINT('Ctrl Pts',(179.157615054692,583.808404790033,-49.5221601717597)) ;
#68802=CARTESIAN_POINT('Ctrl Pts',(179.211658678873,583.78097084842,-49.5221601717596)) ;
#68803=CARTESIAN_POINT('Ctrl Pts',(179.266948118332,583.75611161908,-49.5221601717595)) ;
#68804=CARTESIAN_POINT('Ctrl Pts',(179.32336237667,583.733991238111,-49.5221601717598)) ;
#68805=CARTESIAN_POINT('Ctrl Pts',(179.333841264731,583.729882401039,-49.5221601717599)) ;
#68806=CARTESIAN_POINT('Ctrl Pts',(179.344358997566,583.725868115481,-49.5221601717977)) ;
#68807=CARTESIAN_POINT('Ctrl Pts',(179.354914418328,583.721948031586,-49.5221601717676)) ;
#68808=CARTESIAN_POINT('',(181.158603910567,586.791560837527,-49.5230454887661)) ;
#68809=CARTESIAN_POINT('Ctrl Pts',(180.418697842604,583.725390834864,-49.5221601717597)) ;
#68810=CARTESIAN_POINT('Ctrl Pts',(180.487296450736,583.750790356198,-49.5221601717599)) ;
#68811=CARTESIAN_POINT('Ctrl Pts',(180.554192682413,583.780090567917,-49.5221601717597)) ;
#68812=CARTESIAN_POINT('Ctrl Pts',(180.619198732011,583.812994518591,-49.5221601717598)) ;
#68813=CARTESIAN_POINT('Ctrl Pts',(180.686069299032,583.846842227418,-49.52216017176)) ;
#68814=CARTESIAN_POINT('Ctrl Pts',(180.750940472857,583.884504055634,-49.5221601717598)) ;
#68815=CARTESIAN_POINT('Ctrl Pts',(180.813576621044,583.925701550019,-49.5221601717597)) ;
#68816=CARTESIAN_POINT('Ctrl Pts',(180.866567999829,583.960555417843,-49.5221601717596)) ;
#68817=CARTESIAN_POINT('Ctrl Pts',(180.917959332204,583.997940989355,-49.5221601717597)) ;
#68818=CARTESIAN_POINT('Ctrl Pts',(180.967585109464,584.037707766149,-49.5221601717599)) ;
#68819=CARTESIAN_POINT('Ctrl Pts',(180.989595033746,584.0553450465,-49.5221601717599)) ;
#68820=CARTESIAN_POINT('Ctrl Pts',(181.011257355173,584.073450908606,-49.5221601717598)) ;
#68821=CARTESIAN_POINT('Ctrl Pts',(181.03255608396,584.092012943614,-49.5221601717598)) ;
#68822=CARTESIAN_POINT('Ctrl Pts',(181.044224754291,584.102182295473,-49.5221601717598)) ;
#68823=CARTESIAN_POINT('Ctrl Pts',(181.055784275477,584.112488573221,-49.5221601717599)) ;
#68824=CARTESIAN_POINT('Ctrl Pts',(181.067231885704,584.122929777226,-49.5221601717597)) ;
#68825=CARTESIAN_POINT('Ctrl Pts',(181.077873257536,584.132635622549,-49.5221601717596)) ;
#68826=CARTESIAN_POINT('Ctrl Pts',(181.08841944345,584.142459654982,-49.5221601717598)) ;
#68827=CARTESIAN_POINT('Ctrl Pts',(181.098852143756,584.152384601306,-49.5221601717598)) ;
#68828=CARTESIAN_POINT('Ctrl Pts',(181.151927496952,584.202876805252,-49.5221601717598)) ;
#68829=CARTESIAN_POINT('Ctrl Pts',(181.202162899846,584.25606195107,-49.52216017176)) ;
#68830=CARTESIAN_POINT('Ctrl Pts',(181.249340293922,584.311676856567,-49.5221601717599)) ;
#68831=CARTESIAN_POINT('Ctrl Pts',(181.296163855244,584.366874647563,-49.5221601717598)) ;
#68832=CARTESIAN_POINT('Ctrl Pts',(181.339975615632,584.424466779741,-49.5221601717597)) ;
#68833=CARTESIAN_POINT('Ctrl Pts',(181.380517571197,584.484220184186,-49.5221601717597)) ;
#68834=CARTESIAN_POINT('Ctrl Pts',(181.414270877463,584.533968030153,-49.5221601717597)) ;
#68835=CARTESIAN_POINT('Ctrl Pts',(181.445757100861,584.585214604105,-49.5221601717599)) ;
#68836=CARTESIAN_POINT('Ctrl Pts',(181.474799558564,584.637831851519,-49.52216017176)) ;
#68837=CARTESIAN_POINT('Ctrl Pts',(181.486860259247,584.659682649351,-49.52216017176)) ;
#68838=CARTESIAN_POINT('Ctrl Pts',(181.498499196222,584.681769865865,-49.5221601717599)) ;
#68839=CARTESIAN_POINT('Ctrl Pts',(181.509702288582,584.704084406422,-49.52216017176)) ;
#68840=CARTESIAN_POINT('Ctrl Pts',(181.514927026246,584.714491142058,-49.52216017176)) ;
#68841=CARTESIAN_POINT('Ctrl Pts',(181.520056956668,584.724947319877,-49.5221601717599)) ;
#68842=CARTESIAN_POINT('Ctrl Pts',(181.525090585488,584.735452015056,-49.5221601717597)) ;
#68843=CARTESIAN_POINT('Ctrl Pts',(181.530284200014,584.746290584888,-49.5221601717596)) ;
#68844=CARTESIAN_POINT('Ctrl Pts',(181.535371608344,584.757173173073,-49.5221601717597)) ;
#68845=CARTESIAN_POINT('Ctrl Pts',(181.540349993555,584.768094923541,-49.5221601717597)) ;
#68846=CARTESIAN_POINT('Ctrl Pts',(181.568890832369,584.830708784548,-49.5221601717597)) ;
#68847=CARTESIAN_POINT('Ctrl Pts',(181.593871140868,584.894647947158,-49.52216017176)) ;
#68848=CARTESIAN_POINT('Ctrl Pts',(181.615067844391,584.959704548492,-49.52216017176)) ;
#68849=CARTESIAN_POINT('Ctrl Pts',(181.634414752743,585.019083786513,-49.52216017176)) ;
#68850=CARTESIAN_POINT('Ctrl Pts',(181.650609336792,585.079394549769,-49.5221601717599)) ;
#68851=CARTESIAN_POINT('Ctrl Pts',(181.663444305221,585.140483589067,-49.5221601717599)) ;
#68852=CARTESIAN_POINT('Ctrl Pts',(181.678529682811,585.212283627337,-49.5221601717598)) ;
#68853=CARTESIAN_POINT('Ctrl Pts',(181.688974591945,585.285160304771,-49.5221601717599)) ;
#68854=CARTESIAN_POINT('Ctrl Pts',(181.69485402845,585.358692290302,-49.5221601717597)) ;
#68855=CARTESIAN_POINT('Ctrl Pts',(181.696158240314,585.375003596294,-49.5221601717597)) ;
#68856=CARTESIAN_POINT('Ctrl Pts',(181.697237572428,585.391347063828,-49.5221601717598)) ;
#68857=CARTESIAN_POINT('Ctrl Pts',(181.698092464185,585.407717923508,-49.5221601717599)) ;
#68858=CARTESIAN_POINT('Ctrl Pts',(181.698929390057,585.42374474318,-49.5221601717599)) ;
#68859=CARTESIAN_POINT('Ctrl Pts',(181.699551206998,585.439803114389,-49.5221601717596)) ;
#68860=CARTESIAN_POINT('Ctrl Pts',(181.699957827124,585.455857315496,-49.5221601717596)) ;
#68861=CARTESIAN_POINT('Ctrl Pts',(181.701693898361,585.524400987964,-49.5221601717595)) ;
#68862=CARTESIAN_POINT('Ctrl Pts',(181.699518932262,585.592962618904,-49.5221601717596)) ;
#68863=CARTESIAN_POINT('Ctrl Pts',(181.69355365263,585.661206408135,-49.5221601717596)) ;
#68864=CARTESIAN_POINT('Ctrl Pts',(181.687589105054,585.72944182252,-49.5221601717596)) ;
#68865=CARTESIAN_POINT('Ctrl Pts',(181.677834721031,585.797360538863,-49.5221601717599)) ;
#68866=CARTESIAN_POINT('Ctrl Pts',(181.664361571398,585.864611794249,-49.5221601717597)) ;
#68867=CARTESIAN_POINT('Ctrl Pts',(181.654511676375,585.913777566451,-49.5221601717596)) ;
#68868=CARTESIAN_POINT('Ctrl Pts',(181.642673152834,585.962586345324,-49.5221601717598)) ;
#68869=CARTESIAN_POINT('Ctrl Pts',(181.6288590601,586.010891074006,-49.5221601717596)) ;
#68870=CARTESIAN_POINT('Ctrl Pts',(181.623146758882,586.03086568731,-49.5221601717596)) ;
#68871=CARTESIAN_POINT('Ctrl Pts',(181.617096512571,586.050753989256,-49.5221601717595)) ;
#68872=CARTESIAN_POINT('Ctrl Pts',(181.610708686729,586.07054500919,-49.5221601717596)) ;
#68873=CARTESIAN_POINT('Ctrl Pts',(181.605967464192,586.085234456283,-49.5221601717597)) ;
#68874=CARTESIAN_POINT('Ctrl Pts',(181.60104026166,586.099870303452,-49.5221601717596)) ;
#68875=CARTESIAN_POINT('Ctrl Pts',(181.595927120135,586.114447926979,-49.5221601717595)) ;
#68876=CARTESIAN_POINT('Ctrl Pts',(181.591624798445,586.126713894112,-49.5221601717595)) ;
#68877=CARTESIAN_POINT('Ctrl Pts',(181.587193599639,586.138930667478,-49.5221601717596)) ;
#68878=CARTESIAN_POINT('Ctrl Pts',(181.582635315551,586.151092329678,-49.5221601717596)) ;
#68879=CARTESIAN_POINT('Ctrl Pts',(181.559525016203,586.212751420818,-49.5221601717596)) ;
#68880=CARTESIAN_POINT('Ctrl Pts',(181.533140942791,586.273025515692,-49.5221601717595)) ;
#68881=CARTESIAN_POINT('Ctrl Pts',(181.503533287679,586.331582535562,-49.5221601717596)) ;
#68882=CARTESIAN_POINT('Ctrl Pts',(181.482570051262,586.373042916223,-49.5221601717597)) ;
#68883=CARTESIAN_POINT('Ctrl Pts',(181.459989934264,586.413641981649,-49.5221601717594)) ;
#68884=CARTESIAN_POINT('Ctrl Pts',(181.435800104679,586.453250265223,-49.5221601717596)) ;
#68885=CARTESIAN_POINT('Ctrl Pts',(181.428072880055,586.465902777017,-49.5221601717596)) ;
#68886=CARTESIAN_POINT('Ctrl Pts',(181.420180103468,586.478455995157,-49.5221601717599)) ;
#68887=CARTESIAN_POINT('Ctrl Pts',(181.41212580138,586.490899350876,-49.5221601717598)) ;
#68888=CARTESIAN_POINT('Ctrl Pts',(181.377861739762,586.543835024558,-49.5221601717596)) ;
#68889=CARTESIAN_POINT('Ctrl Pts',(181.340741511594,586.594687784843,-49.5221601717595)) ;
#68890=CARTESIAN_POINT('Ctrl Pts',(181.300799349475,586.643144100953,-49.5221601717596)) ;
#68891=CARTESIAN_POINT('Ctrl Pts',(181.263590552905,586.688284401652,-49.5221601717596)) ;
#68892=CARTESIAN_POINT('Ctrl Pts',(181.223932268822,586.731345188883,-49.5221601717599)) ;
#68893=CARTESIAN_POINT('Ctrl Pts',(181.181829923378,586.772038827239,-49.5221601717597)) ;
#68894=CARTESIAN_POINT('Ctrl Pts',(181.174641042286,586.778987174755,-49.5221601717596)) ;
#68895=CARTESIAN_POINT('Ctrl Pts',(181.16738085938,586.785866419088,-49.5221601717594)) ;
#68896=CARTESIAN_POINT('Ctrl Pts',(181.160050608476,586.792676042491,-49.5221601717598)) ;
#68897=CARTESIAN_POINT('Ctrl Pts',(181.157212958645,586.790376961384,-49.5230454887661)) ;
#68898=CARTESIAN_POINT('Ctrl Pts',(181.15218800891,586.796280842063,-49.5227503830974)) ;
#68899=CARTESIAN_POINT('Ctrl Pts',(181.147121847573,586.802149646446,-49.5224552774286)) ;
#68900=CARTESIAN_POINT('Ctrl Pts',(181.142014968315,586.807982802636,-49.5221601717599)) ;
#68901=CARTESIAN_POINT('Ctrl Pts',(180.419233204836,583.719736168872,-49.5189770331172)) ;
#68902=CARTESIAN_POINT('Ctrl Pts',(181.082048866651,583.896399029745,-49.4818859761884)) ;
#68903=CARTESIAN_POINT('Ctrl Pts',(182.205022110371,584.964384226175,-49.4077208373071)) ;
#68904=CARTESIAN_POINT('Ctrl Pts',(181.773244511485,587.256847446489,-49.2964816164732)) ;
#68905=CARTESIAN_POINT('Ctrl Pts',(179.609919830324,588.131303024858,-49.1852593706157)) ;
#68906=CARTESIAN_POINT('Ctrl Pts',(177.703480010983,586.788368782476,-49.0740371247583)) ;
#68907=CARTESIAN_POINT('Ctrl Pts',(177.798971922146,584.457519353846,-48.9628148789009)) ;
#68908=CARTESIAN_POINT('Ctrl Pts',(179.810018459729,583.275506361501,-48.8515926330436)) ;
#68909=CARTESIAN_POINT('Ctrl Pts',(181.892849241664,584.325438807312,-48.7403703871863)) ;
#68910=CARTESIAN_POINT('Ctrl Pts',(182.138609898212,586.645025743417,-48.629148141329)) ;
#68911=CARTESIAN_POINT('Ctrl Pts',(180.321944045418,588.108107728139,-48.5179258954715)) ;
#68912=CARTESIAN_POINT('Ctrl Pts',(178.108023948598,587.373654057886,-48.406703649614)) ;
#68913=CARTESIAN_POINT('Ctrl Pts',(177.52607497017,585.114849113815,-48.2954814037566)) ;
#68914=CARTESIAN_POINT('Ctrl Pts',(179.109499392003,583.402058754468,-48.1842591578995)) ;
#68915=CARTESIAN_POINT('Ctrl Pts',(181.406959449108,583.805244989922,-48.0730369120422)) ;
#68916=CARTESIAN_POINT('Ctrl Pts',(182.312583535423,585.954753589864,-47.9618146661847)) ;
#68917=CARTESIAN_POINT('Ctrl Pts',(180.996335289573,587.880617927167,-47.8505924203273)) ;
#68918=CARTESIAN_POINT('Ctrl Pts',(178.664394818812,587.817124582104,-47.7393701744699)) ;
#68919=CARTESIAN_POINT('Ctrl Pts',(177.454434725336,585.823639759907,-47.6281479286125)) ;
#68920=CARTESIAN_POINT('Ctrl Pts',(178.474212119244,583.724901972206,-47.5169256827551)) ;
#68921=CARTESIAN_POINT('Ctrl Pts',(180.790706847517,583.45028245465,-47.4056890764861)) ;
#68922=CARTESIAN_POINT('Ctrl Pts',(181.779706210552,584.643301812666,-47.3315265521695)) ;
#68923=CARTESIAN_POINT('Ctrl Pts',(181.91085375533,585.316553064795,-47.2944381098053)) ;
#68924=CARTESIAN_POINT('Ctrl Pts',(180.385086629763,583.847829775303,-49.5955145204618)) ;
#68925=CARTESIAN_POINT('Ctrl Pts',(181.005255510324,584.013125822117,-49.5584234635329)) ;
#68926=CARTESIAN_POINT('Ctrl Pts',(182.055974585899,585.012394882708,-49.4842583246516)) ;
#68927=CARTESIAN_POINT('Ctrl Pts',(181.651978353492,587.157356794404,-49.3730191038177)) ;
#68928=CARTESIAN_POINT('Ctrl Pts',(179.627845969337,587.975548289235,-49.2617968579602)) ;
#68929=CARTESIAN_POINT('Ctrl Pts',(177.844070001549,586.719020911042,-49.1505746121029)) ;
#68930=CARTESIAN_POINT('Ctrl Pts',(177.933417787156,584.538142630417,-49.0393523662454)) ;
#68931=CARTESIAN_POINT('Ctrl Pts',(179.815069884142,583.432182532455,-48.9281301203881)) ;
#68932=CARTESIAN_POINT('Ctrl Pts',(181.763887494898,584.414560389673,-48.8169078745308)) ;
#68933=CARTESIAN_POINT('Ctrl Pts',(181.993835457868,586.584900827298,-48.7056856286735)) ;
#68934=CARTESIAN_POINT('Ctrl Pts',(180.294057234166,587.953845420656,-48.594463382816)) ;
#68935=CARTESIAN_POINT('Ctrl Pts',(178.222584836642,587.266647853149,-48.4832411369586)) ;
#68936=CARTESIAN_POINT('Ctrl Pts',(177.67807952802,585.153178582169,-48.3720188911011)) ;
#68937=CARTESIAN_POINT('Ctrl Pts',(179.159623504295,583.550592311223,-48.2607966452439)) ;
#68938=CARTESIAN_POINT('Ctrl Pts',(181.309260747095,583.927836801213,-48.1495743993865)) ;
#68939=CARTESIAN_POINT('Ctrl Pts',(182.156615310626,585.939042056281,-48.0383521535292)) ;
#68940=CARTESIAN_POINT('Ctrl Pts',(180.925056902766,587.740992732744,-47.9271299076718)) ;
#68941=CARTESIAN_POINT('Ctrl Pts',(178.743157779671,587.681584666521,-47.8159076618144)) ;
#68942=CARTESIAN_POINT('Ctrl Pts',(177.611048748572,585.816364331787,-47.7046854159569)) ;
#68943=CARTESIAN_POINT('Ctrl Pts',(178.565211785502,583.85266320133,-47.5934631700996)) ;
#68944=CARTESIAN_POINT('Ctrl Pts',(180.732658973646,583.595713209658,-47.4822265638306)) ;
#68945=CARTESIAN_POINT('Ctrl Pts',(181.658024294933,584.711971503438,-47.408064039514)) ;
#68946=CARTESIAN_POINT('Ctrl Pts',(181.780733564974,585.341904529203,-47.3709755971498)) ;
#68947=CARTESIAN_POINT('Ctrl Pts',(180.35094005469,583.975923381734,-49.6720520078063)) ;
#68948=CARTESIAN_POINT('Ctrl Pts',(180.928462153998,584.12985261449,-49.6349609508773)) ;
#68949=CARTESIAN_POINT('Ctrl Pts',(181.906927061425,585.060405539239,-49.5607958119961)) ;
#68950=CARTESIAN_POINT('Ctrl Pts',(181.530712195499,587.05786614232,-49.4495565911623)) ;
#68951=CARTESIAN_POINT('Ctrl Pts',(179.645772108348,587.819793553612,-49.3383343453048)) ;
#68952=CARTESIAN_POINT('Ctrl Pts',(177.984659992115,586.64967303961,-49.2271120994473)) ;
#68953=CARTESIAN_POINT('Ctrl Pts',(178.067863652165,584.61876590699,-49.11588985359)) ;
#68954=CARTESIAN_POINT('Ctrl Pts',(179.820121308555,583.58885870341,-49.0046676077327)) ;
#68955=CARTESIAN_POINT('Ctrl Pts',(181.634925748135,584.503681972034,-48.8934453618754)) ;
#68956=CARTESIAN_POINT('Ctrl Pts',(181.849061017523,586.52477591118,-48.782223116018)) ;
#68957=CARTESIAN_POINT('Ctrl Pts',(180.266170422915,587.799583113174,-48.6710008701606)) ;
#68958=CARTESIAN_POINT('Ctrl Pts',(178.337145724684,587.159641648412,-48.5597786243031)) ;
#68959=CARTESIAN_POINT('Ctrl Pts',(177.830084085871,585.191508050522,-48.4485563784457)) ;
#68960=CARTESIAN_POINT('Ctrl Pts',(179.209747616584,583.699125867978,-48.3373341325884)) ;
#68961=CARTESIAN_POINT('Ctrl Pts',(181.211562045081,584.050428612505,-48.2261118867311)) ;
#68962=CARTESIAN_POINT('Ctrl Pts',(182.000647085828,585.923330522697,-48.1148896408738)) ;
#68963=CARTESIAN_POINT('Ctrl Pts',(180.853778515959,587.601367538321,-48.0036673950164)) ;
#68964=CARTESIAN_POINT('Ctrl Pts',(178.82192074053,587.546044750939,-47.8924451491589)) ;
#68965=CARTESIAN_POINT('Ctrl Pts',(177.767662771809,585.809088903666,-47.7812229033014)) ;
#68966=CARTESIAN_POINT('Ctrl Pts',(178.65621145176,583.980424430455,-47.6700006574441)) ;
#68967=CARTESIAN_POINT('Ctrl Pts',(180.674611099775,583.741143964668,-47.5587640511751)) ;
#68968=CARTESIAN_POINT('Ctrl Pts',(181.536342379315,584.780641194212,-47.4846015268585)) ;
#68969=CARTESIAN_POINT('Ctrl Pts',(181.650613374619,585.367255993608,-47.4475130844944)) ;
#68970=CARTESIAN_POINT('Ctrl Pts',(180.316793479617,584.104016988166,-49.7485894951507)) ;
#68971=CARTESIAN_POINT('Ctrl Pts',(180.851668797671,584.246579406862,-49.7114984382218)) ;
#68972=CARTESIAN_POINT('Ctrl Pts',(181.757879536953,585.108416195771,-49.6373332993405)) ;
#68973=CARTESIAN_POINT('Ctrl Pts',(181.409446037507,586.958375490236,-49.5260940785067)) ;
#68974=CARTESIAN_POINT('Ctrl Pts',(179.66369824736,587.664038817989,-49.4148718326492)) ;
#68975=CARTESIAN_POINT('Ctrl Pts',(178.125249982681,586.580325168177,-49.3036495867918)) ;
#68976=CARTESIAN_POINT('Ctrl Pts',(178.202309517176,584.699389183561,-49.1924273409344)) ;
#68977=CARTESIAN_POINT('Ctrl Pts',(179.825172732969,583.745534874366,-49.0812050950771)) ;
#68978=CARTESIAN_POINT('Ctrl Pts',(181.505964001371,584.592803554395,-48.9699828492198)) ;
#68979=CARTESIAN_POINT('Ctrl Pts',(181.704286577179,586.464650995062,-48.8587606033624)) ;
#68980=CARTESIAN_POINT('Ctrl Pts',(180.238283611663,587.645320805693,-48.747538357505)) ;
#68981=CARTESIAN_POINT('Ctrl Pts',(178.451706612729,587.052635443676,-48.6363161116476)) ;
#68982=CARTESIAN_POINT('Ctrl Pts',(177.982088643721,585.229837518876,-48.5250938657901)) ;
#68983=CARTESIAN_POINT('Ctrl Pts',(179.259871728876,583.847659424733,-48.4138716199328)) ;
#68984=CARTESIAN_POINT('Ctrl Pts',(181.113863343068,584.173020423797,-48.3026493740755)) ;
#68985=CARTESIAN_POINT('Ctrl Pts',(181.844678861032,585.907618989114,-48.1914271282182)) ;
#68986=CARTESIAN_POINT('Ctrl Pts',(180.782500129152,587.461742343898,-48.0802048823608)) ;
#68987=CARTESIAN_POINT('Ctrl Pts',(178.90068370139,587.410504835355,-47.9689826365033)) ;
#68988=CARTESIAN_POINT('Ctrl Pts',(177.924276795045,585.801813475545,-47.8577603906459)) ;
#68989=CARTESIAN_POINT('Ctrl Pts',(178.747211118018,584.108185659579,-47.7465381447886)) ;
#68990=CARTESIAN_POINT('Ctrl Pts',(180.616563225904,583.886574719676,-47.6353015385195)) ;
#68991=CARTESIAN_POINT('Ctrl Pts',(181.414660463695,584.849310884986,-47.561139014203)) ;
#68992=CARTESIAN_POINT('Ctrl Pts',(181.520493184263,585.392607458014,-47.5240505718387)) ;
#68993=CARTESIAN_POINT('Ctrl Pts',(181.523656952667,585.391334705907,-47.52216017176)) ;
#68994=CARTESIAN_POINT('Ctrl Pts',(181.518864111216,585.329612029403,-47.5221601717599)) ;
#68995=CARTESIAN_POINT('Ctrl Pts',(181.510354110053,585.268421425887,-47.5221601717598)) ;
#68996=CARTESIAN_POINT('Ctrl Pts',(181.498399921215,585.207975725837,-47.5221601717598)) ;
#68997=CARTESIAN_POINT('Ctrl Pts',(181.485625550261,585.143382819915,-47.5221601717598)) ;
#68998=CARTESIAN_POINT('Ctrl Pts',(181.468918454449,585.079639831897,-47.5221601717598)) ;
#68999=CARTESIAN_POINT('Ctrl Pts',(181.448550450063,585.016994878175,-47.5221601717598)) ;
#69000=CARTESIAN_POINT('Ctrl Pts',(181.430728446226,584.962180543669,-47.5221601717598)) ;
#69001=CARTESIAN_POINT('Ctrl Pts',(181.410102435538,584.908206315245,-47.5221601717598)) ;
#69002=CARTESIAN_POINT('Ctrl Pts',(181.386818394606,584.855239139212,-47.5221601717598)) ;
#69003=CARTESIAN_POINT('Ctrl Pts',(181.375118389598,584.828623646365,-47.5221601717598)) ;
#69004=CARTESIAN_POINT('Ctrl Pts',(181.36274673317,584.802262491287,-47.5221601717597)) ;
#69005=CARTESIAN_POINT('Ctrl Pts',(181.349719011124,584.776177545999,-47.5221601717597)) ;
#69006=CARTESIAN_POINT('Ctrl Pts',(181.343823711948,584.764373597778,-47.5221601717597)) ;
#69007=CARTESIAN_POINT('Ctrl Pts',(181.337793201643,584.752624884227,-47.5221601717598)) ;
#69008=CARTESIAN_POINT('Ctrl Pts',(181.331639037062,584.740952119149,-47.5221601717598)) ;
#69009=CARTESIAN_POINT('Ctrl Pts',(181.300412762748,584.681724427155,-47.5221601717601)) ;
#69010=CARTESIAN_POINT('Ctrl Pts',(181.265953645831,584.624341910917,-47.5221601717599)) ;
#69011=CARTESIAN_POINT('Ctrl Pts',(181.22852965889,584.569045052016,-47.5221601717601)) ;
#69012=CARTESIAN_POINT('Ctrl Pts',(181.19042442106,584.512741591806,-47.5221601717603)) ;
#69013=CARTESIAN_POINT('Ctrl Pts',(181.14924507502,584.458599455405,-47.52216017176)) ;
#69014=CARTESIAN_POINT('Ctrl Pts',(181.105221373277,584.406880458077,-47.52216017176)) ;
#69015=CARTESIAN_POINT('Ctrl Pts',(181.068294032599,584.363498258075,-47.5221601717601)) ;
#69016=CARTESIAN_POINT('Ctrl Pts',(181.029364334819,584.321820807193,-47.5221601717601)) ;
#69017=CARTESIAN_POINT('Ctrl Pts',(180.988542561273,584.28201446558,-47.52216017176)) ;
#69018=CARTESIAN_POINT('Ctrl Pts',(180.969684450482,584.263625445822,-47.5221601717599)) ;
#69019=CARTESIAN_POINT('Ctrl Pts',(180.95042225226,584.24563593154,-47.5221601717597)) ;
#69020=CARTESIAN_POINT('Ctrl Pts',(180.930765375998,584.228063505193,-47.5221601717599)) ;
#69021=CARTESIAN_POINT('Ctrl Pts',(180.922295997763,584.220492234801,-47.5221601717599)) ;
#69022=CARTESIAN_POINT('Ctrl Pts',(180.913753717785,584.212998855305,-47.52216017176)) ;
#69023=CARTESIAN_POINT('Ctrl Pts',(180.905149669589,584.205593422028,-47.52216017176)) ;
#69024=CARTESIAN_POINT('Ctrl Pts',(180.851912915241,584.159772986898,-47.5221601717599)) ;
#69025=CARTESIAN_POINT('Ctrl Pts',(180.796216600555,584.117228680269,-47.5221601717599)) ;
#69026=CARTESIAN_POINT('Ctrl Pts',(180.738312458319,584.078227871123,-47.5221601717597)) ;
#69027=CARTESIAN_POINT('Ctrl Pts',(180.68624332931,584.043157182146,-47.5221601717596)) ;
#69028=CARTESIAN_POINT('Ctrl Pts',(180.632387955704,584.010951462255,-47.5221601717599)) ;
#69029=CARTESIAN_POINT('Ctrl Pts',(180.576898639163,583.981823861986,-47.5221601717599)) ;
#69030=CARTESIAN_POINT('Ctrl Pts',(180.516759270754,583.950255344068,-47.5221601717598)) ;
#69031=CARTESIAN_POINT('Ctrl Pts',(180.45470061862,583.922301113456,-47.52216017176)) ;
#69032=CARTESIAN_POINT('Ctrl Pts',(180.391040733099,583.897902595055,-47.5221601717598)) ;
#69033=CARTESIAN_POINT('Ctrl Pts',(180.366741521824,583.888589591291,-47.5221601717597)) ;
#69034=CARTESIAN_POINT('Ctrl Pts',(180.342208714014,583.879795102048,-47.5221601717597)) ;
#69035=CARTESIAN_POINT('Ctrl Pts',(180.317459037939,583.871517581215,-47.5221601717597)) ;
#69036=CARTESIAN_POINT('Ctrl Pts',(180.306558516397,583.867871905454,-47.5221601717597)) ;
#69037=CARTESIAN_POINT('Ctrl Pts',(180.295616870051,583.864326925159,-47.5221601717597)) ;
#69038=CARTESIAN_POINT('Ctrl Pts',(180.284647851826,583.860886128633,-47.5221601717597)) ;
#69039=CARTESIAN_POINT('Ctrl Pts',(180.217882198215,583.839942866049,-47.5221601717599)) ;
#69040=CARTESIAN_POINT('Ctrl Pts',(180.149986712694,583.822815707665,-47.5221601717597)) ;
#69041=CARTESIAN_POINT('Ctrl Pts',(180.081325520431,583.809396313223,-47.5221601717599)) ;
#69042=CARTESIAN_POINT('Ctrl Pts',(180.011091307362,583.795669481843,-47.52216017176)) ;
#69043=CARTESIAN_POINT('Ctrl Pts',(179.940055072934,583.785821976791,-47.5221601717599)) ;
#69044=CARTESIAN_POINT('Ctrl Pts',(179.868574627648,583.779784122078,-47.5221601717597)) ;
#69045=CARTESIAN_POINT('Ctrl Pts',(179.814562564869,583.775221797564,-47.5221601717595)) ;
#69046=CARTESIAN_POINT('Ctrl Pts',(179.760296108056,583.772835580708,-47.5221601717598)) ;
#69047=CARTESIAN_POINT('Ctrl Pts',(179.70592257077,583.772613692646,-47.5221601717599)) ;
#69048=CARTESIAN_POINT('Ctrl Pts',(179.672228443948,583.772476193324,-47.52216017176)) ;
#69049=CARTESIAN_POINT('Ctrl Pts',(179.638493099144,583.773170112498,-47.5221601717597)) ;
#69050=CARTESIAN_POINT('Ctrl Pts',(179.604751128406,583.774695759566,-47.5221601717598)) ;
#69051=CARTESIAN_POINT('Ctrl Pts',(179.591849093273,583.775279126561,-47.5221601717598)) ;
#69052=CARTESIAN_POINT('Ctrl Pts',(179.578943804841,583.775984275203,-47.52216017176)) ;
#69053=CARTESIAN_POINT('Ctrl Pts',(179.566044644676,583.776810827873,-47.5221601717599)) ;
#69054=CARTESIAN_POINT('Ctrl Pts',(179.489473938043,583.781717327302,-47.5221601717596)) ;
#69055=CARTESIAN_POINT('Ctrl Pts',(179.413305930242,583.790883712635,-47.5221601717601)) ;
#69056=CARTESIAN_POINT('Ctrl Pts',(179.337954124025,583.804242075326,-47.5221601717598)) ;
#69057=CARTESIAN_POINT('Ctrl Pts',(179.281440269363,583.814260847344,-47.5221601717596)) ;
#69058=CARTESIAN_POINT('Ctrl Pts',(179.22538486089,583.826638741016,-47.5221601717598)) ;
#69059=CARTESIAN_POINT('Ctrl Pts',(179.16995895443,583.841368214518,-47.5221601717597)) ;
#69060=CARTESIAN_POINT('Ctrl Pts',(179.150298717127,583.846592936365,-47.5221601717597)) ;
#69061=CARTESIAN_POINT('Ctrl Pts',(179.130717683404,583.852113703417,-47.52216017176)) ;
#69062=CARTESIAN_POINT('Ctrl Pts',(179.111223524679,583.857930736292,-47.5221601717599)) ;
#69063=CARTESIAN_POINT('Ctrl Pts',(179.096457923615,583.862336773405,-47.5221601717599)) ;
#69064=CARTESIAN_POINT('Ctrl Pts',(179.081747033544,583.866911400053,-47.5221601717598)) ;
#69065=CARTESIAN_POINT('Ctrl Pts',(179.067101764441,583.871651813381,-47.5221601717598)) ;
#69066=CARTESIAN_POINT('Ctrl Pts',(178.995451726963,583.894843657125,-47.5221601717601)) ;
#69067=CARTESIAN_POINT('Ctrl Pts',(178.925316590381,583.922016092408,-47.5221601717601)) ;
#69068=CARTESIAN_POINT('Ctrl Pts',(178.85707525169,583.953137102575,-47.52216017176)) ;
#69069=CARTESIAN_POINT('Ctrl Pts',(178.801930877505,583.978285328893,-47.52216017176)) ;
#69070=CARTESIAN_POINT('Ctrl Pts',(178.748022741564,584.006012880253,-47.5221601717596)) ;
#69071=CARTESIAN_POINT('Ctrl Pts',(178.695554610711,584.036327495048,-47.5221601717598)) ;
#69072=CARTESIAN_POINT('Ctrl Pts',(178.68521642417,584.042300609348,-47.5221601717598)) ;
#69073=CARTESIAN_POINT('Ctrl Pts',(178.6749341666,584.048374232336,-47.5221601717599)) ;
#69074=CARTESIAN_POINT('Ctrl Pts',(178.664708372347,584.054547023819,-47.5221601717602)) ;
#69075=CARTESIAN_POINT('Ctrl Pts',(178.622424393781,586.788243831647,-49.5202697760045)) ;
#69076=CARTESIAN_POINT('Ctrl Pts',(178.263643649736,586.36676060424,-49.4831813336731)) ;
#69077=CARTESIAN_POINT('Ctrl Pts',(178.008551654752,585.142526919038,-49.4090188093893)) ;
#69078=CARTESIAN_POINT('Ctrl Pts',(179.347336054222,583.819180735871,-49.2977822031531)) ;
#69079=CARTESIAN_POINT('Ctrl Pts',(181.184558760889,584.231744443467,-49.1865599572958)) ;
#69080=CARTESIAN_POINT('Ctrl Pts',(181.833504573659,585.99813274514,-49.0753377114385)) ;
#69081=CARTESIAN_POINT('Ctrl Pts',(180.700270327141,587.501342130218,-48.9641154655811)) ;
#69082=CARTESIAN_POINT('Ctrl Pts',(178.822950161505,587.362806835846,-48.8528932197236)) ;
#69083=CARTESIAN_POINT('Ctrl Pts',(177.9224424202,585.7099277411,-48.7416709738662)) ;
#69084=CARTESIAN_POINT('Ctrl Pts',(178.824009812191,584.057559465188,-48.6304487280089)) ;
#69085=CARTESIAN_POINT('Ctrl Pts',(180.701324880746,583.920322366968,-48.5192264821516)) ;
#69086=CARTESIAN_POINT('Ctrl Pts',(181.833643668398,585.423980393734,-48.4080042362942)) ;
#69087=CARTESIAN_POINT('Ctrl Pts',(181.183111205273,587.190315812827,-48.2967819904368)) ;
#69088=CARTESIAN_POINT('Ctrl Pts',(179.345988480579,587.600347497167,-48.1855597445794)) ;
#69089=CARTESIAN_POINT('Ctrl Pts',(178.006171324865,586.278214874925,-48.0743374987219)) ;
#69090=CARTESIAN_POINT('Ctrl Pts',(178.391706208018,584.435855966388,-47.9631152528646)) ;
#69091=CARTESIAN_POINT('Ctrl Pts',(180.149298192699,583.761768844811,-47.8518930070073)) ;
#69092=CARTESIAN_POINT('Ctrl Pts',(181.667918986456,584.874265675204,-47.74067076115)) ;
#69093=CARTESIAN_POINT('Ctrl Pts',(181.555993617726,586.752757360581,-47.6294485152926)) ;
#69094=CARTESIAN_POINT('Ctrl Pts',(179.915827865207,587.677664053704,-47.5182262694351)) ;
#69095=CARTESIAN_POINT('Ctrl Pts',(178.252238680771,586.796655916462,-47.4069878500146)) ;
#69096=CARTESIAN_POINT('Ctrl Pts',(178.143431118054,585.550825987599,-47.3328235125465)) ;
#69097=CARTESIAN_POINT('Ctrl Pts',(178.365443895008,585.043763351793,-47.2957332570309)) ;
#69098=CARTESIAN_POINT('Ctrl Pts',(178.52085580834,586.874696733313,-49.5972768795265)) ;
#69099=CARTESIAN_POINT('Ctrl Pts',(178.133293167415,586.419401527445,-49.5601884371951)) ;
#69100=CARTESIAN_POINT('Ctrl Pts',(177.857737333116,585.096958090823,-49.4860259129113)) ;
#69101=CARTESIAN_POINT('Ctrl Pts',(179.303920903732,583.667451211978,-49.3747893066751)) ;
#69102=CARTESIAN_POINT('Ctrl Pts',(181.288528204949,584.113111361584,-49.2635670608178)) ;
#69103=CARTESIAN_POINT('Ctrl Pts',(181.989533365316,586.021201822019,-49.1523448149605)) ;
#69104=CARTESIAN_POINT('Ctrl Pts',(180.765389470584,587.645000782295,-49.0411225691031)) ;
#69105=CARTESIAN_POINT('Ctrl Pts',(178.737468035733,587.495351991384,-48.9299003232456)) ;
#69106=CARTESIAN_POINT('Ctrl Pts',(177.764720294423,585.709876606414,-48.8186780773881)) ;
#69107=CARTESIAN_POINT('Ctrl Pts',(178.738612693092,583.924953018886,-48.7074558315308)) ;
#69108=CARTESIAN_POINT('Ctrl Pts',(180.766528621966,583.776706567251,-48.5962335856736)) ;
#69109=CARTESIAN_POINT('Ctrl Pts',(181.989683618431,585.400990159884,-48.4850113398162)) ;
#69110=CARTESIAN_POINT('Ctrl Pts',(181.286964524382,587.309023495424,-48.3737890939588)) ;
#69111=CARTESIAN_POINT('Ctrl Pts',(179.302465225832,587.751948499301,-48.2625668481014)) ;
#69112=CARTESIAN_POINT('Ctrl Pts',(177.855166049811,586.323752534949,-48.1513446022439)) ;
#69113=CARTESIAN_POINT('Ctrl Pts',(178.271629084588,584.333596998508,-48.0401223563866)) ;
#69114=CARTESIAN_POINT('Ctrl Pts',(180.170217575085,583.605433658112,-47.9289001105293)) ;
#69115=CARTESIAN_POINT('Ctrl Pts',(181.810664268964,584.807176551974,-47.817677864672)) ;
#69116=CARTESIAN_POINT('Ctrl Pts',(181.689760089429,586.836363487529,-47.7064556188146)) ;
#69117=CARTESIAN_POINT('Ctrl Pts',(179.918017928915,587.835467498957,-47.5952333729571)) ;
#69118=CARTESIAN_POINT('Ctrl Pts',(178.120973275767,586.883783647426,-47.4839949535366)) ;
#69119=CARTESIAN_POINT('Ctrl Pts',(178.003437017037,585.538011486041,-47.4098306160686)) ;
#69120=CARTESIAN_POINT('Ctrl Pts',(178.243259971819,584.990271571035,-47.3727403605529)) ;
#69121=CARTESIAN_POINT('Ctrl Pts',(178.419287222901,586.961149634978,-49.6742839830486)) ;
#69122=CARTESIAN_POINT('Ctrl Pts',(178.002942685092,586.472042450653,-49.6371955407171)) ;
#69123=CARTESIAN_POINT('Ctrl Pts',(177.706923011481,585.051389262609,-49.5630330164334)) ;
#69124=CARTESIAN_POINT('Ctrl Pts',(179.260505753241,583.515721688086,-49.4517964101971)) ;
#69125=CARTESIAN_POINT('Ctrl Pts',(181.39249764901,583.994478279701,-49.3405741643399)) ;
#69126=CARTESIAN_POINT('Ctrl Pts',(182.145562156973,586.044270898896,-49.2293519184826)) ;
#69127=CARTESIAN_POINT('Ctrl Pts',(180.830508614027,587.788659434373,-49.1181296726251)) ;
#69128=CARTESIAN_POINT('Ctrl Pts',(178.651985909963,587.627897146924,-49.0069074267677)) ;
#69129=CARTESIAN_POINT('Ctrl Pts',(177.606998168646,585.70982547173,-48.8956851809102)) ;
#69130=CARTESIAN_POINT('Ctrl Pts',(178.653215573992,583.792346572583,-48.7844629350528)) ;
#69131=CARTESIAN_POINT('Ctrl Pts',(180.831732363186,583.633090767534,-48.6732406891957)) ;
#69132=CARTESIAN_POINT('Ctrl Pts',(182.145723568463,585.377999926036,-48.5620184433382)) ;
#69133=CARTESIAN_POINT('Ctrl Pts',(181.39081784349,587.427731178022,-48.4507961974808)) ;
#69134=CARTESIAN_POINT('Ctrl Pts',(179.258941971085,587.903549501434,-48.3395739516234)) ;
#69135=CARTESIAN_POINT('Ctrl Pts',(177.704160774758,586.369290194971,-48.228351705766)) ;
#69136=CARTESIAN_POINT('Ctrl Pts',(178.151551961158,584.231338030628,-48.1171294599086)) ;
#69137=CARTESIAN_POINT('Ctrl Pts',(180.191136957471,583.449098471413,-48.0059072140514)) ;
#69138=CARTESIAN_POINT('Ctrl Pts',(181.953409551472,584.740087428744,-47.8946849681939)) ;
#69139=CARTESIAN_POINT('Ctrl Pts',(181.823526561132,586.919969614479,-47.7834627223367)) ;
#69140=CARTESIAN_POINT('Ctrl Pts',(179.920207992622,587.99327094421,-47.6722404764791)) ;
#69141=CARTESIAN_POINT('Ctrl Pts',(177.989707870763,586.970911378389,-47.5610020570586)) ;
#69142=CARTESIAN_POINT('Ctrl Pts',(177.863442916019,585.525196984482,-47.4868377195905)) ;
#69143=CARTESIAN_POINT('Ctrl Pts',(178.12107604863,584.936779790278,-47.449747464075)) ;
#69144=CARTESIAN_POINT('Ctrl Pts',(178.317718637461,587.047602536644,-49.7512910865705)) ;
#69145=CARTESIAN_POINT('Ctrl Pts',(177.87259220277,586.52468337386,-49.7142026442391)) ;
#69146=CARTESIAN_POINT('Ctrl Pts',(177.556108689845,585.005820434396,-49.6400401199553)) ;
#69147=CARTESIAN_POINT('Ctrl Pts',(179.217090602751,583.363992164192,-49.5288035137192)) ;
#69148=CARTESIAN_POINT('Ctrl Pts',(181.496467093069,583.875845197818,-49.4175812678619)) ;
#69149=CARTESIAN_POINT('Ctrl Pts',(182.301590948631,586.067339975775,-49.3063590220046)) ;
#69150=CARTESIAN_POINT('Ctrl Pts',(180.89562775747,587.932318086451,-49.1951367761471)) ;
#69151=CARTESIAN_POINT('Ctrl Pts',(178.566503784192,587.760442302463,-49.0839145302897)) ;
#69152=CARTESIAN_POINT('Ctrl Pts',(177.44927604287,585.709774337044,-48.9726922844322)) ;
#69153=CARTESIAN_POINT('Ctrl Pts',(178.567818454894,583.65974012628,-48.8614700385749)) ;
#69154=CARTESIAN_POINT('Ctrl Pts',(180.896936104404,583.489474967817,-48.7502477927177)) ;
#69155=CARTESIAN_POINT('Ctrl Pts',(182.301763518496,585.355009692186,-48.6390255468602)) ;
#69156=CARTESIAN_POINT('Ctrl Pts',(181.494671162598,587.546438860619,-48.5278033010028)) ;
#69157=CARTESIAN_POINT('Ctrl Pts',(179.215418716338,588.055150503567,-48.4165810551454)) ;
#69158=CARTESIAN_POINT('Ctrl Pts',(177.553155499703,586.414827854993,-48.305358809288)) ;
#69159=CARTESIAN_POINT('Ctrl Pts',(178.031474837727,584.129079062749,-48.1941365634305)) ;
#69160=CARTESIAN_POINT('Ctrl Pts',(180.212056339858,583.292763284713,-48.0829143175733)) ;
#69161=CARTESIAN_POINT('Ctrl Pts',(182.096154833979,584.672998305515,-47.971692071716)) ;
#69162=CARTESIAN_POINT('Ctrl Pts',(181.957293032835,587.003575741428,-47.8604698258587)) ;
#69163=CARTESIAN_POINT('Ctrl Pts',(179.922398056331,588.151074389465,-47.7492475800012)) ;
#69164=CARTESIAN_POINT('Ctrl Pts',(177.858442465759,587.058039109354,-47.6380091605806)) ;
#69165=CARTESIAN_POINT('Ctrl Pts',(177.723448815003,585.512382482924,-47.5638448231125)) ;
#69166=CARTESIAN_POINT('Ctrl Pts',(177.998892125441,584.883288009522,-47.526754567597)) ;
#69167=CARTESIAN_POINT('',(179.941804423115,587.377540552573,-47.5212748618547)) ;
#69168=CARTESIAN_POINT('Ctrl Pts',(178.005900115752,584.887332980433,-47.5221601717599)) ;
#69169=CARTESIAN_POINT('Ctrl Pts',(177.982987728062,584.956801876012,-47.52216017176)) ;
#69170=CARTESIAN_POINT('Ctrl Pts',(177.964186437101,585.027371840573,-47.52216017176)) ;
#69171=CARTESIAN_POINT('Ctrl Pts',(177.94938117184,585.098710895595,-47.5221601717598)) ;
#69172=CARTESIAN_POINT('Ctrl Pts',(177.934151259053,585.172096111404,-47.5221601717596)) ;
#69173=CARTESIAN_POINT('Ctrl Pts',(177.923149945878,585.246296203004,-47.52216017176)) ;
#69174=CARTESIAN_POINT('Ctrl Pts',(177.916306443315,585.320953332826,-47.5221601717598)) ;
#69175=CARTESIAN_POINT('Ctrl Pts',(177.910516709373,585.384114691281,-47.5221601717596)) ;
#69176=CARTESIAN_POINT('Ctrl Pts',(177.907703953494,585.447603574384,-47.5221601717599)) ;
#69177=CARTESIAN_POINT('Ctrl Pts',(177.907853704318,585.511196748025,-47.5221601717599)) ;
#69178=CARTESIAN_POINT('Ctrl Pts',(177.907920121497,585.539401462535,-47.5221601717599)) ;
#69179=CARTESIAN_POINT('Ctrl Pts',(177.908569617401,585.567626566114,-47.52216017176)) ;
#69180=CARTESIAN_POINT('Ctrl Pts',(177.909802459868,585.595851820656,-47.52216017176)) ;
#69181=CARTESIAN_POINT('Ctrl Pts',(177.910477882035,585.611315242044,-47.52216017176)) ;
#69182=CARTESIAN_POINT('Ctrl Pts',(177.911328410559,585.626778699084,-47.5221601717596)) ;
#69183=CARTESIAN_POINT('Ctrl Pts',(177.912354204027,585.642238785753,-47.5221601717597)) ;
#69184=CARTESIAN_POINT('Ctrl Pts',(177.913307752249,585.656610039442,-47.5221601717597)) ;
#69185=CARTESIAN_POINT('Ctrl Pts',(177.914413050293,585.670980562236,-47.5221601717595)) ;
#69186=CARTESIAN_POINT('Ctrl Pts',(177.915668003083,585.685325277191,-47.5221601717596)) ;
#69187=CARTESIAN_POINT('Ctrl Pts',(177.922052454499,585.758302632532,-47.5221601717599)) ;
#69188=CARTESIAN_POINT('Ctrl Pts',(177.932313012602,585.830738647026,-47.5221601717598)) ;
#69189=CARTESIAN_POINT('Ctrl Pts',(177.946379870592,585.902298744286,-47.5221601717596)) ;
#69190=CARTESIAN_POINT('Ctrl Pts',(177.96034122638,585.97332213691,-47.5221601717594)) ;
#69191=CARTESIAN_POINT('Ctrl Pts',(177.978052380569,586.043483656018,-47.5221601717599)) ;
#69192=CARTESIAN_POINT('Ctrl Pts',(177.999491975402,586.112436269997,-47.5221601717598)) ;
#69193=CARTESIAN_POINT('Ctrl Pts',(178.017341563624,586.16984294097,-47.5221601717597)) ;
#69194=CARTESIAN_POINT('Ctrl Pts',(178.037776407616,586.226411576796,-47.5221601717598)) ;
#69195=CARTESIAN_POINT('Ctrl Pts',(178.060806550301,586.281924200616,-47.5221601717596)) ;
#69196=CARTESIAN_POINT('Ctrl Pts',(178.070370467521,586.304977385573,-47.5221601717596)) ;
#69197=CARTESIAN_POINT('Ctrl Pts',(178.080382189699,586.327848227021,-47.5221601717595)) ;
#69198=CARTESIAN_POINT('Ctrl Pts',(178.090843385664,586.350520045651,-47.5221601717597)) ;
#69199=CARTESIAN_POINT('Ctrl Pts',(178.095722128577,586.361093404073,-47.5221601717597)) ;
#69200=CARTESIAN_POINT('Ctrl Pts',(178.100698638309,586.371623465901,-47.5221601717597)) ;
#69201=CARTESIAN_POINT('Ctrl Pts',(178.105773123522,586.382108486179,-47.5221601717598)) ;
#69202=CARTESIAN_POINT('Ctrl Pts',(178.111008892306,586.39292675435,-47.5221601717599)) ;
#69203=CARTESIAN_POINT('Ctrl Pts',(178.116345294491,586.403689432172,-47.5221601717598)) ;
#69204=CARTESIAN_POINT('Ctrl Pts',(178.121780289776,586.414391289583,-47.5221601717598)) ;
#69205=CARTESIAN_POINT('Ctrl Pts',(178.152938853733,586.475744518271,-47.5221601717595)) ;
#69206=CARTESIAN_POINT('Ctrl Pts',(178.187353534623,586.535140324373,-47.5221601717597)) ;
#69207=CARTESIAN_POINT('Ctrl Pts',(178.225000903539,586.59227470075,-47.5221601717595)) ;
#69208=CARTESIAN_POINT('Ctrl Pts',(178.259362859716,586.644423071108,-47.5221601717594)) ;
#69209=CARTESIAN_POINT('Ctrl Pts',(178.296418553824,586.694687651655,-47.5221601717597)) ;
#69210=CARTESIAN_POINT('Ctrl Pts',(178.336177414887,586.742810826234,-47.5221601717597)) ;
#69211=CARTESIAN_POINT('Ctrl Pts',(178.382907364859,586.799371640113,-47.5221601717598)) ;
#69212=CARTESIAN_POINT('Ctrl Pts',(178.433372350224,586.852975663353,-47.5221601717595)) ;
#69213=CARTESIAN_POINT('Ctrl Pts',(178.487196201923,586.903418834412,-47.5221601717596)) ;
#69214=CARTESIAN_POINT('Ctrl Pts',(178.499135731636,586.914608441262,-47.5221601717596)) ;
#69215=CARTESIAN_POINT('Ctrl Pts',(178.5112406165,586.92564228244,-47.5221601717595)) ;
#69216=CARTESIAN_POINT('Ctrl Pts',(178.523506853694,586.936517727807,-47.5221601717595)) ;
#69217=CARTESIAN_POINT('Ctrl Pts',(178.535515310811,586.947164621165,-47.5221601717595)) ;
#69218=CARTESIAN_POINT('Ctrl Pts',(178.547682554143,586.95766300766,-47.5221601717598)) ;
#69219=CARTESIAN_POINT('Ctrl Pts',(178.559980710183,586.967990546505,-47.5221601717598)) ;
#69220=CARTESIAN_POINT('Ctrl Pts',(178.612487888008,587.01208414207,-47.5221601717597)) ;
#69221=CARTESIAN_POINT('Ctrl Pts',(178.667447598405,587.053131162542,-47.5221601717596)) ;
#69222=CARTESIAN_POINT('Ctrl Pts',(178.72452203213,587.091016625585,-47.5221601717597)) ;
#69223=CARTESIAN_POINT('Ctrl Pts',(178.781589461753,587.128897439372,-47.5221601717597)) ;
#69224=CARTESIAN_POINT('Ctrl Pts',(178.840772211404,587.163617781791,-47.5221601717597)) ;
#69225=CARTESIAN_POINT('Ctrl Pts',(178.901751731621,587.195014521141,-47.5221601717596)) ;
#69226=CARTESIAN_POINT('Ctrl Pts',(178.946332389148,587.217967920568,-47.5221601717595)) ;
#69227=CARTESIAN_POINT('Ctrl Pts',(178.991873827707,587.239143965964,-47.5221601717594)) ;
#69228=CARTESIAN_POINT('Ctrl Pts',(179.038252931247,587.258461179061,-47.5221601717596)) ;
#69229=CARTESIAN_POINT('Ctrl Pts',(179.057431274439,587.266449089866,-47.5221601717597)) ;
#69230=CARTESIAN_POINT('Ctrl Pts',(179.076752842022,587.27411897031,-47.5221601717596)) ;
#69231=CARTESIAN_POINT('Ctrl Pts',(179.09620882887,587.281464266111,-47.5221601717597)) ;
#69232=CARTESIAN_POINT('Ctrl Pts',(179.110649603242,587.286916148875,-47.5221601717598)) ;
#69233=CARTESIAN_POINT('Ctrl Pts',(179.125164428122,587.292189207664,-47.5221601717596)) ;
#69234=CARTESIAN_POINT('Ctrl Pts',(179.139749662979,587.297280591696,-47.5221601717598)) ;
#69235=CARTESIAN_POINT('Ctrl Pts',(179.152022037213,587.30156460706,-47.5221601717599)) ;
#69236=CARTESIAN_POINT('Ctrl Pts',(179.164336303796,587.305717190402,-47.5221601717595)) ;
#69237=CARTESIAN_POINT('Ctrl Pts',(179.176686719118,587.309736053194,-47.5221601717595)) ;
#69238=CARTESIAN_POINT('Ctrl Pts',(179.239458582398,587.330162208845,-47.5221601717595)) ;
#69239=CARTESIAN_POINT('Ctrl Pts',(179.30319355351,587.347148258287,-47.5221601717595)) ;
#69240=CARTESIAN_POINT('Ctrl Pts',(179.367598526706,587.36052507701,-47.5221601717595)) ;
#69241=CARTESIAN_POINT('Ctrl Pts',(179.412926408987,587.369939611855,-47.5221601717596)) ;
#69242=CARTESIAN_POINT('Ctrl Pts',(179.458586283043,587.377565388163,-47.5221601717598)) ;
#69243=CARTESIAN_POINT('Ctrl Pts',(179.50447356325,587.383328055194,-47.5221601717595)) ;
#69244=CARTESIAN_POINT('Ctrl Pts',(179.519183541229,587.385175379872,-47.5221601717594)) ;
#69245=CARTESIAN_POINT('Ctrl Pts',(179.533919108266,587.386831362232,-47.5221601717596)) ;
#69246=CARTESIAN_POINT('Ctrl Pts',(179.548669490907,587.388292560769,-47.5221601717596)) ;
#69247=CARTESIAN_POINT('Ctrl Pts',(179.611419560358,587.394508691691,-47.5221601717596)) ;
#69248=CARTESIAN_POINT('Ctrl Pts',(179.674321933271,587.397193106461,-47.5221601717594)) ;
#69249=CARTESIAN_POINT('Ctrl Pts',(179.737110137716,587.396177085949,-47.5221601717594)) ;
#69250=CARTESIAN_POINT('Ctrl Pts',(179.795601551891,587.39523059485,-47.5221601717594)) ;
#69251=CARTESIAN_POINT('Ctrl Pts',(179.853994367444,587.391072461822,-47.5221601717598)) ;
#69252=CARTESIAN_POINT('Ctrl Pts',(179.912060318785,587.383527591442,-47.5221601717599)) ;
#69253=CARTESIAN_POINT('Ctrl Pts',(179.921974949721,587.382239321749,-47.5221601717599)) ;
#69254=CARTESIAN_POINT('Ctrl Pts',(179.931880009566,587.380852220923,-47.5221601717594)) ;
#69255=CARTESIAN_POINT('Ctrl Pts',(179.941774324258,587.379366930793,-47.5221601717597)) ;
#69256=CARTESIAN_POINT('Ctrl Pts',(179.941746076329,587.375714942532,-47.5212748618547)) ;
#69257=CARTESIAN_POINT('Ctrl Pts',(179.949494858334,587.375467290232,-47.5215699651564)) ;
#69258=CARTESIAN_POINT('Ctrl Pts',(179.95724191163,587.375165548564,-47.5218650684581)) ;
#69259=CARTESIAN_POINT('Ctrl Pts',(179.964986481303,587.374809746934,-47.5221601717598)) ;
#69260=CARTESIAN_POINT('Origin',(10.1385276254028,514.798278400837,-46.5221601717518)) ;
#69261=CARTESIAN_POINT('',(7.38852762540283,516.385991641109,-47.5221601717519)) ;
#69262=CARTESIAN_POINT('',(10.1385276254028,514.798278400837,-47.5221601717521)) ;
#69263=CARTESIAN_POINT('',(88.274584783925,469.686404766948,-47.5221601717556)) ;
#69264=CARTESIAN_POINT('',(7.38852762540283,516.385991641109,-46.5221601717517)) ;
#69265=CARTESIAN_POINT('',(10.1385276254028,514.798278400837,-46.7721601717518)) ;
#69266=CARTESIAN_POINT('Origin',(10.1385276254028,511.622851920294,-46.5221601717521)) ;
#69267=CARTESIAN_POINT('',(10.1385276254028,511.622851920294,-47.5221601717521)) ;
#69268=CARTESIAN_POINT('',(10.1385276254028,507.916708540412,-47.5221601717521)) ;
#69269=CARTESIAN_POINT('',(10.1385276254028,511.622851920294,-46.7721601717521)) ;
#69270=CARTESIAN_POINT('Origin',(7.38852762540283,516.385991641109,-46.5221601717517)) ;
#69271=CARTESIAN_POINT('',(4.63852762540283,514.798278400837,-47.5221601717518)) ;
#69272=CARTESIAN_POINT('',(81.6274704668795,559.247865274989,-47.5221601717553)) ;
#69273=CARTESIAN_POINT('',(4.63852762540283,514.798278400837,-46.7721601717518)) ;
#69274=CARTESIAN_POINT('Origin',(4.63852762540283,514.798278400837,-46.5221601717518)) ;
#69275=CARTESIAN_POINT('',(4.63852762540283,511.622851920294,-47.5221601717518)) ;
#69276=CARTESIAN_POINT('',(4.63852762540284,509.504421780684,-47.5221601717518)) ;
#69277=CARTESIAN_POINT('',(4.63852762540283,511.622851920294,-46.7721601717521)) ;
#69278=CARTESIAN_POINT('Origin',(4.63852762540283,511.622851920294,-46.5221601717521)) ;
#69279=CARTESIAN_POINT('',(7.38852762540283,510.035138680023,-47.5221601717519)) ;
#69280=CARTESIAN_POINT('',(84.149584783925,465.71712166627,-47.5221601717554)) ;
#69281=CARTESIAN_POINT('',(7.38852762540283,510.035138680023,-46.5221601717522)) ;
#69282=CARTESIAN_POINT('Origin',(7.38852762540283,510.035138680023,-46.5221601717522)) ;
#69283=CARTESIAN_POINT('',(83.0024704668795,553.690868934038,-47.5221601717554)) ;
#69284=CARTESIAN_POINT('Origin',(187.63852762542,609.798278400806,-46.5221601717598)) ;
#69285=CARTESIAN_POINT('',(184.88852762542,611.385991641078,-47.52216017176)) ;
#69286=CARTESIAN_POINT('',(187.63852762542,609.798278400806,-47.5221601717601)) ;
#69287=CARTESIAN_POINT('',(219.780188123809,591.241282059859,-47.5221601717616)) ;
#69288=CARTESIAN_POINT('',(184.88852762542,611.385991641078,-46.5221601717597)) ;
#69289=CARTESIAN_POINT('',(187.63852762542,609.798278400806,-46.7721601717598)) ;
#69290=CARTESIAN_POINT('Origin',(187.63852762542,606.622851920263,-46.5221601717601)) ;
#69291=CARTESIAN_POINT('',(187.63852762542,606.622851920263,-47.5221601717601)) ;
#69292=CARTESIAN_POINT('',(187.63852762542,555.416708540397,-47.5221601717601)) ;
#69293=CARTESIAN_POINT('',(187.63852762542,606.622851920263,-46.7721601717601)) ;
#69294=CARTESIAN_POINT('Origin',(184.88852762542,611.385991641078,-46.5221601717597)) ;
#69295=CARTESIAN_POINT('',(182.13852762542,609.798278400806,-47.5221601717599)) ;
#69296=CARTESIAN_POINT('',(171.996867127016,603.942987982023,-47.5221601717594)) ;
#69297=CARTESIAN_POINT('',(182.13852762542,609.798278400806,-46.7721601717598)) ;
#69298=CARTESIAN_POINT('Origin',(182.13852762542,609.798278400806,-46.5221601717598)) ;
#69299=CARTESIAN_POINT('',(182.13852762542,606.622851920263,-47.5221601717599)) ;
#69300=CARTESIAN_POINT('',(182.13852762542,557.004421780668,-47.5221601717599)) ;
#69301=CARTESIAN_POINT('',(182.13852762542,606.622851920263,-46.7721601717601)) ;
#69302=CARTESIAN_POINT('Origin',(182.13852762542,606.622851920263,-46.5221601717601)) ;
#69303=CARTESIAN_POINT('',(184.88852762542,605.035138679992,-47.52216017176)) ;
#69304=CARTESIAN_POINT('',(215.655188123809,587.271998959181,-47.5221601717614)) ;
#69305=CARTESIAN_POINT('',(184.88852762542,605.035138679992,-46.5221601717602)) ;
#69306=CARTESIAN_POINT('Origin',(184.88852762542,605.035138679992,-46.5221601717602)) ;
#69307=CARTESIAN_POINT('',(173.371867127016,598.385991641073,-47.5221601717595)) ;
#69308=CARTESIAN_POINT('Origin',(212.388527625401,504.21056516053,-47.5221601717613)) ;
#69309=CARTESIAN_POINT('',(4.63852762541949,609.798278400837,-47.5221601717518)) ;
#69310=CARTESIAN_POINT('',(7.38852762541949,611.385991641109,-47.5221601717519)) ;
#69311=CARTESIAN_POINT('',(61.0593671270094,642.372865274985,-47.5221601717544)) ;
#69312=CARTESIAN_POINT('',(10.1385276254195,609.798278400837,-47.5221601717521)) ;
#69313=CARTESIAN_POINT('',(108.842688123816,552.811404766952,-47.5221601717566)) ;
#69314=CARTESIAN_POINT('',(10.1385276254195,606.622851920294,-47.5221601717521)) ;
#69315=CARTESIAN_POINT('',(10.1385276254195,555.416708540412,-47.5221601717521)) ;
#69316=CARTESIAN_POINT('',(7.38852762541949,605.035138680023,-47.5221601717519)) ;
#69317=CARTESIAN_POINT('',(62.4343671270094,636.815868934035,-47.5221601717544)) ;
#69318=CARTESIAN_POINT('',(4.63852762541949,606.622851920294,-47.5221601717518)) ;
#69319=CARTESIAN_POINT('',(104.717688123816,548.842121666274,-47.5221601717564)) ;
#69320=CARTESIAN_POINT('',(4.63852762541951,557.004421780684,-47.5221601717518)) ;
#69321=CARTESIAN_POINT('Origin',(10.1385276254195,609.798278400837,-46.5221601717518)) ;
#69322=CARTESIAN_POINT('',(7.38852762541949,611.385991641109,-46.5221601717516)) ;
#69323=CARTESIAN_POINT('',(10.1385276254195,609.798278400837,-46.7721601717518)) ;
#69324=CARTESIAN_POINT('Origin',(10.1385276254195,606.622851920294,-46.522160171752)) ;
#69325=CARTESIAN_POINT('',(10.1385276254195,606.622851920294,-46.772160171752)) ;
#69326=CARTESIAN_POINT('Origin',(7.38852762541949,611.385991641109,-46.5221601717516)) ;
#69327=CARTESIAN_POINT('',(4.63852762541949,609.798278400837,-46.7721601717518)) ;
#69328=CARTESIAN_POINT('Origin',(4.63852762541949,609.798278400837,-46.5221601717518)) ;
#69329=CARTESIAN_POINT('',(4.63852762541949,606.622851920294,-46.772160171752)) ;
#69330=CARTESIAN_POINT('Origin',(4.63852762541949,606.622851920294,-46.522160171752)) ;
#69331=CARTESIAN_POINT('',(7.38852762541949,605.035138680023,-46.5221601717522)) ;
#69332=CARTESIAN_POINT('Origin',(7.38852762541949,605.035138680023,-46.5221601717522)) ;
#69333=CARTESIAN_POINT('',(0.,0.,0.)) ;
#69334=CARTESIAN_POINT('',(0.,0.,0.)) ;
#86282=UNCERTAINTY_MEASURE_WITH_UNIT(LENGTH_MEASURE(0.01),#86331,
'DISTANCE_ACCURACY_VALUE',
'Maximum model space distance between geometric entities at asserted c
onnectivities') ;
#86304=UNCERTAINTY_MEASURE_WITH_UNIT(LENGTH_MEASURE(0.01),#86331,
'DISTANCE_ACCURACY_VALUE',
'Maximum model space distance between geometric entities at asserted c
onnectivities') ;
#86308=(
GEOMETRIC_REPRESENTATION_CONTEXT(3)
GLOBAL_UNCERTAINTY_ASSIGNED_CONTEXT((#86282))
GLOBAL_UNIT_ASSIGNED_CONTEXT((#86331,#86333,#86334))
REPRESENTATION_CONTEXT('','3D')
) ;
#86330=(
GEOMETRIC_REPRESENTATION_CONTEXT(3)
GLOBAL_UNCERTAINTY_ASSIGNED_CONTEXT((#86304))
GLOBAL_UNIT_ASSIGNED_CONTEXT((#86331,#86333,#86334))
REPRESENTATION_CONTEXT('','3D')
) ;
#86331=(
LENGTH_UNIT()
NAMED_UNIT(*)
SI_UNIT(.MILLI.,.METRE.)
) ;
#86333=(
NAMED_UNIT(*)
PLANE_ANGLE_UNIT()
SI_UNIT($,.RADIAN.)
) ;
#86334=(
NAMED_UNIT(*)
SI_UNIT($,.STERADIAN.)
SOLID_ANGLE_UNIT()
) ;
#86338=SHAPE_DEFINITION_REPRESENTATION(#86363,#86454) ;
#86363=PRODUCT_DEFINITION_SHAPE('',$,#86480) ;
#86454=SHAPE_REPRESENTATION('',(#33060,#33712,#33713),#86308) ;
#86476=PRODUCT_DEFINITION_CONTEXT('part definition',#86553,'design') ;
#86480=PRODUCT_DEFINITION('Box','Box',#86505,#86476) ;
#86505=PRODUCT_DEFINITION_FORMATION('',$,#86558) ;
#86553=APPLICATION_CONTEXT(
'Core Data for Automotive Mechanical Design Process') ;
#86554=PRODUCT_CONTEXT('part definition',#86553,'mechanical') ;
#86558=PRODUCT('Box','Box',$,(#86554)) ;
#86581=PRESENTATION_STYLE_ASSIGNMENT((#86586)) ;
#86586=SURFACE_STYLE_USAGE(.BOTH.,#86591) ;
#86591=SURFACE_SIDE_STYLE('',(#86596)) ;
#86596=SURFACE_STYLE_FILL_AREA(#86601) ;
#86601=FILL_AREA_STYLE('Opaque(228,229,230)',(#86606)) ;
#86606=FILL_AREA_STYLE_COLOUR('Opaque(228,229,230)',#86611) ;
#86611=COLOUR_RGB('Opaque(228,229,230)', 0.09019608, 0.27058824, 0.51372549) ;
ENDSEC;
END-ISO-10303-21;
